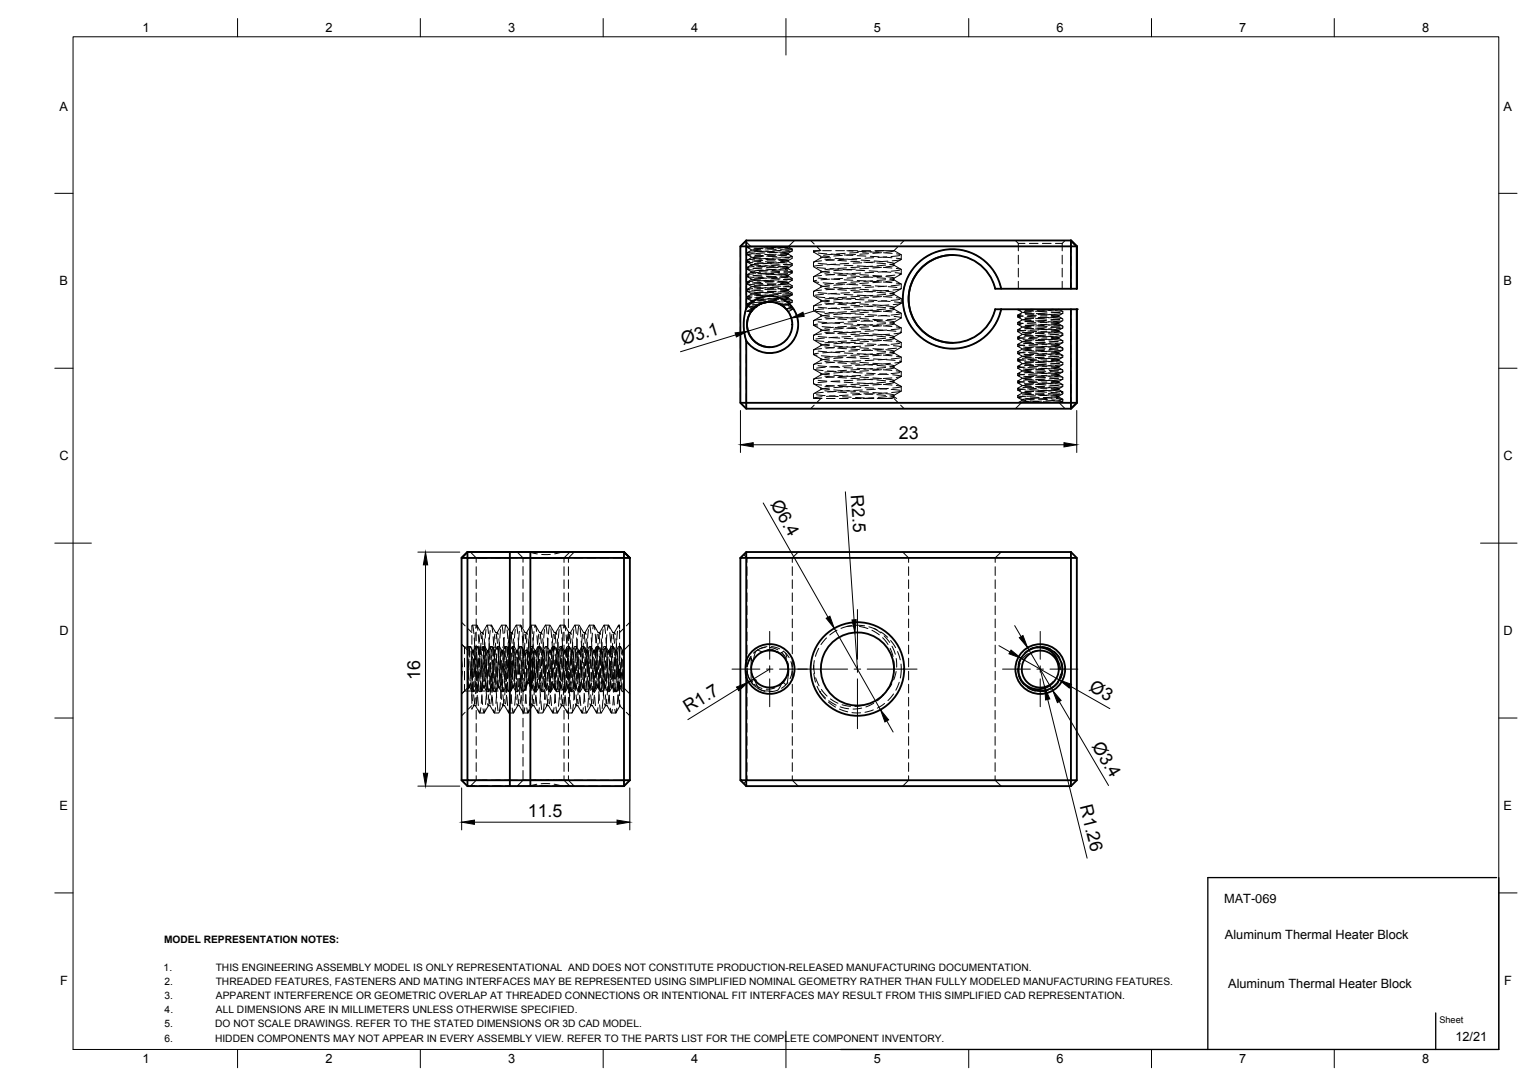
ISO-10303-21;
HEADER;
/* Generated by software containing ST-Developer
 * from STEP Tools, Inc. (www.steptools.com) 
 */

FILE_DESCRIPTION(
/* description */ ('CAx-IF Rec.Pracs.---Representation and Presentation of Product Manufa
cturing Information (PMI)---4.0---2014-10-13'),
/* implementation_level */ '2;1');

FILE_NAME(
/* name */ 'Aluminum Thermal Heater Block.step',
/* time_stamp */ '2026-10-24T15:08:39-07:00',
/* author */ (''),
/* organization */ (''),
/* preprocessor_version */ 'ST-DEVELOPER v20.2',
/* originating_system */ 'Autodesk Translation Framework v15.17.0.0',
/* authorisation */ '');

FILE_SCHEMA (('AP242_MANAGED_MODEL_BASED_3D_ENGINEERING_MIM_LF { 1 0 10303 442 2 1 4 }'));
ENDSEC;

DATA;
#10=MECHANICAL_DESIGN_GEOMETRIC_PRESENTATION_REPRESENTATION('',(#829),#50081);
#96=B_SPLINE_SURFACE_WITH_KNOTS('',3,3,((#29778,#29779,#29780,#29781,#29782,
#29783,#29784,#29785,#29786,#29787,#29788,#29789,#29790,#29791,#29792,#29793,
#29794,#29795,#29796,#29797,#29798,#29799,#29800,#29801,#29802,#29803,#29804,
#29805,#29806,#29807,#29808,#29809,#29810,#29811,#29812,#29813,#29814,#29815,
#29816,#29817,#29818,#29819,#29820,#29821,#29822,#29823,#29824,#29825,#29826,
#29827,#29828,#29829,#29830,#29831,#29832,#29833,#29834,#29835,#29836,#29837,
#29838,#29839,#29840,#29841,#29842,#29843,#29844,#29845,#29846,#29847,#29848,
#29849,#29850,#29851,#29852,#29853,#29854,#29855,#29856,#29857,#29858,#29859,
#29860,#29861,#29862),(#29863,#29864,#29865,#29866,#29867,#29868,#29869,
#29870,#29871,#29872,#29873,#29874,#29875,#29876,#29877,#29878,#29879,#29880,
#29881,#29882,#29883,#29884,#29885,#29886,#29887,#29888,#29889,#29890,#29891,
#29892,#29893,#29894,#29895,#29896,#29897,#29898,#29899,#29900,#29901,#29902,
#29903,#29904,#29905,#29906,#29907,#29908,#29909,#29910,#29911,#29912,#29913,
#29914,#29915,#29916,#29917,#29918,#29919,#29920,#29921,#29922,#29923,#29924,
#29925,#29926,#29927,#29928,#29929,#29930,#29931,#29932,#29933,#29934,#29935,
#29936,#29937,#29938,#29939,#29940,#29941,#29942,#29943,#29944,#29945,#29946,
#29947),(#29948,#29949,#29950,#29951,#29952,#29953,#29954,#29955,#29956,
#29957,#29958,#29959,#29960,#29961,#29962,#29963,#29964,#29965,#29966,#29967,
#29968,#29969,#29970,#29971,#29972,#29973,#29974,#29975,#29976,#29977,#29978,
#29979,#29980,#29981,#29982,#29983,#29984,#29985,#29986,#29987,#29988,#29989,
#29990,#29991,#29992,#29993,#29994,#29995,#29996,#29997,#29998,#29999,#30000,
#30001,#30002,#30003,#30004,#30005,#30006,#30007,#30008,#30009,#30010,#30011,
#30012,#30013,#30014,#30015,#30016,#30017,#30018,#30019,#30020,#30021,#30022,
#30023,#30024,#30025,#30026,#30027,#30028,#30029,#30030,#30031,#30032),
(#30033,#30034,#30035,#30036,#30037,#30038,#30039,#30040,#30041,#30042,
#30043,#30044,#30045,#30046,#30047,#30048,#30049,#30050,#30051,#30052,#30053,
#30054,#30055,#30056,#30057,#30058,#30059,#30060,#30061,#30062,#30063,#30064,
#30065,#30066,#30067,#30068,#30069,#30070,#30071,#30072,#30073,#30074,#30075,
#30076,#30077,#30078,#30079,#30080,#30081,#30082,#30083,#30084,#30085,#30086,
#30087,#30088,#30089,#30090,#30091,#30092,#30093,#30094,#30095,#30096,#30097,
#30098,#30099,#30100,#30101,#30102,#30103,#30104,#30105,#30106,#30107,#30108,
#30109,#30110,#30111,#30112,#30113,#30114,#30115,#30116,#30117)),
 .UNSPECIFIED.,.F.,.F.,.F.,(4,4),(4,1,1,1,1,1,1,1,1,1,1,1,1,1,1,1,1,1,1,
1,1,1,1,1,1,1,1,1,1,1,1,1,1,1,1,1,1,1,1,1,1,1,1,1,1,1,1,1,1,1,1,1,1,1,1,
1,1,1,1,1,1,1,1,1,1,1,1,1,1,1,1,1,1,1,1,1,1,1,1,1,1,1,4),(-0.000229032876373949,
0.0325052131810458),(10.2100639933856,11.2101668347381,12.2101575453093,
13.2101482558806,14.2101389664519,15.2101296770232,16.2101203875945,17.2101110981658,
18.2101018087371,19.2100925193084,20.2100832298797,21.210073940451,22.2100646510223,
23.2100553615935,24.2100460721648,25.2100367827361,26.2100274933074,27.2100182038787,
28.21000891445,29.2099996250213,30.2099903355926,31.2099810461639,32.2099717567352,
33.2099624673065,34.2099531778778,35.209943888449,36.2099345990203,37.2099253095916,
38.2099160201629,39.2099067307342,40.2098974413055,41.2098881518768,42.2098788624481,
43.2098695730194,44.2098602835907,45.209850994162,46.2098417047333,47.2098324153045,
48.2098231258758,49.2098138364471,50.2098045470184,51.2097952575897,52.209785968161,
53.2097766787323,54.2097673893036,55.2097580998749,56.2097488104462,57.2097395210175,
58.2097302315887,59.20972094216,60.2097116527313,61.2097023633026,62.2096930738739,
63.2096837844452,64.2096744950165,65.2096652055878,66.2096559161591,67.2096466267304,
68.2096373373017,69.209628047873,70.2096187584443,71.2096094690155,72.2096001795868,
73.2095908901581,74.2095816007294,75.2095723113007,76.209563021872,77.2095537324433,
78.2095444430146,79.2095351535859,80.2095258641572,81.2095165747285,82.2095072852998,
83.209497995871,84.2094887064423,85.2094794170136,86.2094701275849,87.2094608381562,
88.2094515487275,89.2094422592988,90.2094329698701,91.2094236804414,92.2094929101791),
 .UNSPECIFIED.);
#97=B_SPLINE_SURFACE_WITH_KNOTS('',3,3,((#30146,#30147,#30148,#30149,#30150,
#30151,#30152,#30153,#30154,#30155,#30156,#30157,#30158,#30159,#30160,#30161,
#30162,#30163,#30164,#30165,#30166,#30167,#30168,#30169,#30170,#30171,#30172,
#30173,#30174,#30175,#30176,#30177,#30178,#30179,#30180,#30181,#30182,#30183,
#30184,#30185,#30186,#30187,#30188,#30189,#30190,#30191,#30192,#30193,#30194,
#30195,#30196,#30197,#30198,#30199,#30200,#30201,#30202,#30203,#30204,#30205,
#30206,#30207,#30208,#30209,#30210,#30211,#30212,#30213,#30214,#30215,#30216,
#30217,#30218,#30219,#30220,#30221,#30222,#30223,#30224,#30225,#30226,#30227,
#30228,#30229,#30230),(#30231,#30232,#30233,#30234,#30235,#30236,#30237,
#30238,#30239,#30240,#30241,#30242,#30243,#30244,#30245,#30246,#30247,#30248,
#30249,#30250,#30251,#30252,#30253,#30254,#30255,#30256,#30257,#30258,#30259,
#30260,#30261,#30262,#30263,#30264,#30265,#30266,#30267,#30268,#30269,#30270,
#30271,#30272,#30273,#30274,#30275,#30276,#30277,#30278,#30279,#30280,#30281,
#30282,#30283,#30284,#30285,#30286,#30287,#30288,#30289,#30290,#30291,#30292,
#30293,#30294,#30295,#30296,#30297,#30298,#30299,#30300,#30301,#30302,#30303,
#30304,#30305,#30306,#30307,#30308,#30309,#30310,#30311,#30312,#30313,#30314,
#30315),(#30316,#30317,#30318,#30319,#30320,#30321,#30322,#30323,#30324,
#30325,#30326,#30327,#30328,#30329,#30330,#30331,#30332,#30333,#30334,#30335,
#30336,#30337,#30338,#30339,#30340,#30341,#30342,#30343,#30344,#30345,#30346,
#30347,#30348,#30349,#30350,#30351,#30352,#30353,#30354,#30355,#30356,#30357,
#30358,#30359,#30360,#30361,#30362,#30363,#30364,#30365,#30366,#30367,#30368,
#30369,#30370,#30371,#30372,#30373,#30374,#30375,#30376,#30377,#30378,#30379,
#30380,#30381,#30382,#30383,#30384,#30385,#30386,#30387,#30388,#30389,#30390,
#30391,#30392,#30393,#30394,#30395,#30396,#30397,#30398,#30399,#30400),
(#30401,#30402,#30403,#30404,#30405,#30406,#30407,#30408,#30409,#30410,
#30411,#30412,#30413,#30414,#30415,#30416,#30417,#30418,#30419,#30420,#30421,
#30422,#30423,#30424,#30425,#30426,#30427,#30428,#30429,#30430,#30431,#30432,
#30433,#30434,#30435,#30436,#30437,#30438,#30439,#30440,#30441,#30442,#30443,
#30444,#30445,#30446,#30447,#30448,#30449,#30450,#30451,#30452,#30453,#30454,
#30455,#30456,#30457,#30458,#30459,#30460,#30461,#30462,#30463,#30464,#30465,
#30466,#30467,#30468,#30469,#30470,#30471,#30472,#30473,#30474,#30475,#30476,
#30477,#30478,#30479,#30480,#30481,#30482,#30483,#30484,#30485)),
 .UNSPECIFIED.,.F.,.F.,.F.,(4,4),(4,1,1,1,1,1,1,1,1,1,1,1,1,1,1,1,1,1,1,
1,1,1,1,1,1,1,1,1,1,1,1,1,1,1,1,1,1,1,1,1,1,1,1,1,1,1,1,1,1,1,1,1,1,1,1,
1,1,1,1,1,1,1,1,1,1,1,1,1,1,1,1,1,1,1,1,1,1,1,1,1,1,1,4),(-0.000337093536336005,
0.0325391625776436),(13.6871942222869,14.6873814867633,15.6873721973346,
16.6873629079059,17.6873536184772,18.6873443290484,19.6873350396197,20.687325750191,
21.6873164607623,22.6873071713336,23.6872978819049,24.6872885924762,25.6872793030475,
26.6872700136188,27.6872607241901,28.6872514347614,29.6872421453326,30.6872328559039,
31.6872235664752,32.6872142770465,33.6872049876178,34.6871956981891,35.6871864087604,
36.6871771193317,37.687167829903,38.6871585404743,39.6871492510456,40.6871399616169,
41.6871306721881,42.6871213827594,43.6871120933307,44.687102803902,45.6870935144733,
46.6870842250446,47.6870749356159,48.6870656461872,49.6870563567585,50.6870470673298,
51.6870377779011,52.6870284884724,53.6870191990436,54.6870099096149,55.6870006201862,
56.6869913307575,57.6869820413288,58.6869727519001,59.6869634624714,60.6869541730427,
61.686944883614,62.6869355941853,63.6869263047566,64.6869170153279,65.6869077258991,
66.6868984364704,67.6868891470417,68.686879857613,69.6868705681843,70.6868612787556,
71.6868519893269,72.6868426998982,73.6868334104695,74.6868241210408,75.6868148316121,
76.6868055421834,77.6867962527546,78.6867869633259,79.6867776738972,80.6867683844685,
81.6867590950398,82.6867498056111,83.6867405161824,84.6867312267537,85.686721937325,
86.6867126478963,87.6867033584676,88.6866940690389,89.6866847796101,90.6866754901814,
91.6866662007527,92.686656911324,93.6866476218953,94.6866383324666,95.6868551020536),
 .UNSPECIFIED.);
#98=B_SPLINE_SURFACE_WITH_KNOTS('',3,3,((#30688,#30689,#30690,#30691,#30692,
#30693,#30694,#30695,#30696,#30697,#30698,#30699,#30700,#30701,#30702,#30703,
#30704,#30705,#30706,#30707,#30708,#30709,#30710,#30711,#30712,#30713,#30714,
#30715,#30716,#30717,#30718,#30719,#30720,#30721,#30722,#30723,#30724,#30725,
#30726,#30727,#30728,#30729,#30730,#30731,#30732,#30733,#30734,#30735,#30736,
#30737,#30738,#30739,#30740,#30741,#30742,#30743,#30744,#30745,#30746,#30747,
#30748,#30749,#30750,#30751,#30752,#30753,#30754,#30755,#30756),(#30757,
#30758,#30759,#30760,#30761,#30762,#30763,#30764,#30765,#30766,#30767,#30768,
#30769,#30770,#30771,#30772,#30773,#30774,#30775,#30776,#30777,#30778,#30779,
#30780,#30781,#30782,#30783,#30784,#30785,#30786,#30787,#30788,#30789,#30790,
#30791,#30792,#30793,#30794,#30795,#30796,#30797,#30798,#30799,#30800,#30801,
#30802,#30803,#30804,#30805,#30806,#30807,#30808,#30809,#30810,#30811,#30812,
#30813,#30814,#30815,#30816,#30817,#30818,#30819,#30820,#30821,#30822,#30823,
#30824,#30825),(#30826,#30827,#30828,#30829,#30830,#30831,#30832,#30833,
#30834,#30835,#30836,#30837,#30838,#30839,#30840,#30841,#30842,#30843,#30844,
#30845,#30846,#30847,#30848,#30849,#30850,#30851,#30852,#30853,#30854,#30855,
#30856,#30857,#30858,#30859,#30860,#30861,#30862,#30863,#30864,#30865,#30866,
#30867,#30868,#30869,#30870,#30871,#30872,#30873,#30874,#30875,#30876,#30877,
#30878,#30879,#30880,#30881,#30882,#30883,#30884,#30885,#30886,#30887,#30888,
#30889,#30890,#30891,#30892,#30893,#30894),(#30895,#30896,#30897,#30898,
#30899,#30900,#30901,#30902,#30903,#30904,#30905,#30906,#30907,#30908,#30909,
#30910,#30911,#30912,#30913,#30914,#30915,#30916,#30917,#30918,#30919,#30920,
#30921,#30922,#30923,#30924,#30925,#30926,#30927,#30928,#30929,#30930,#30931,
#30932,#30933,#30934,#30935,#30936,#30937,#30938,#30939,#30940,#30941,#30942,
#30943,#30944,#30945,#30946,#30947,#30948,#30949,#30950,#30951,#30952,#30953,
#30954,#30955,#30956,#30957,#30958,#30959,#30960,#30961,#30962,#30963)),
 .UNSPECIFIED.,.F.,.F.,.F.,(4,4),(4,1,1,1,1,1,1,1,1,1,1,1,1,1,1,1,1,1,1,
1,1,1,1,1,1,1,1,1,1,1,1,1,1,1,1,1,1,1,1,1,1,1,1,1,1,1,1,1,1,1,1,1,1,1,1,
1,1,1,1,1,1,1,1,1,1,1,4),(-0.000882682909917588,0.0581163152088491),(13.8937860366664,
14.8831634638169,15.8721630239192,16.8611625840214,17.8501621441237,18.8391617042259,
19.8281612643282,20.8171608244304,21.8061603845326,22.7951599446349,23.7841595047371,
24.7731590648394,25.7621586249416,26.7511581850439,27.7401577451461,28.7291573052483,
29.7181568653506,30.7071564254528,31.6961559855551,32.6851555456573,33.6741551057596,
34.6631546658618,35.652154225964,36.6411537860663,37.6301533461685,38.6191529062708,
39.608152466373,40.5971520264753,41.5861515865775,42.5751511466798,43.564150706782,
44.5531502668842,45.5421498269865,46.5311493870887,47.520148947191,48.5091485072932,
49.4981480673955,50.4871476274977,51.4761471875999,52.4651467477022,53.4541463078044,
54.4431458679067,55.4321454280089,56.4211449881112,57.4101445482134,58.3991441083156,
59.3881436684179,60.3771432285201,61.3661427886224,62.3551423487246,63.3441419088269,
64.3331414689291,65.3221410290313,66.3111405891336,67.3001401492358,68.2891397093381,
69.2781392694403,70.2671388295426,71.2561383896448,72.245137949747,73.2341375098493,
74.2231370699515,75.2121366300538,76.201136190156,77.1901357502583,78.1791353103605,
79.1681348704628),.UNSPECIFIED.);
#99=B_SPLINE_SURFACE_WITH_KNOTS('',3,3,((#31557,#31558,#31559,#31560,#31561,
#31562,#31563,#31564,#31565,#31566,#31567,#31568,#31569,#31570,#31571,#31572,
#31573,#31574,#31575,#31576,#31577,#31578,#31579,#31580,#31581,#31582,#31583,
#31584,#31585,#31586,#31587,#31588,#31589,#31590,#31591,#31592,#31593,#31594,
#31595,#31596,#31597,#31598,#31599,#31600,#31601,#31602,#31603,#31604,#31605,
#31606,#31607,#31608,#31609,#31610,#31611,#31612,#31613,#31614,#31615,#31616,
#31617,#31618,#31619,#31620,#31621,#31622,#31623,#31624,#31625),(#31626,
#31627,#31628,#31629,#31630,#31631,#31632,#31633,#31634,#31635,#31636,#31637,
#31638,#31639,#31640,#31641,#31642,#31643,#31644,#31645,#31646,#31647,#31648,
#31649,#31650,#31651,#31652,#31653,#31654,#31655,#31656,#31657,#31658,#31659,
#31660,#31661,#31662,#31663,#31664,#31665,#31666,#31667,#31668,#31669,#31670,
#31671,#31672,#31673,#31674,#31675,#31676,#31677,#31678,#31679,#31680,#31681,
#31682,#31683,#31684,#31685,#31686,#31687,#31688,#31689,#31690,#31691,#31692,
#31693,#31694),(#31695,#31696,#31697,#31698,#31699,#31700,#31701,#31702,
#31703,#31704,#31705,#31706,#31707,#31708,#31709,#31710,#31711,#31712,#31713,
#31714,#31715,#31716,#31717,#31718,#31719,#31720,#31721,#31722,#31723,#31724,
#31725,#31726,#31727,#31728,#31729,#31730,#31731,#31732,#31733,#31734,#31735,
#31736,#31737,#31738,#31739,#31740,#31741,#31742,#31743,#31744,#31745,#31746,
#31747,#31748,#31749,#31750,#31751,#31752,#31753,#31754,#31755,#31756,#31757,
#31758,#31759,#31760,#31761,#31762,#31763),(#31764,#31765,#31766,#31767,
#31768,#31769,#31770,#31771,#31772,#31773,#31774,#31775,#31776,#31777,#31778,
#31779,#31780,#31781,#31782,#31783,#31784,#31785,#31786,#31787,#31788,#31789,
#31790,#31791,#31792,#31793,#31794,#31795,#31796,#31797,#31798,#31799,#31800,
#31801,#31802,#31803,#31804,#31805,#31806,#31807,#31808,#31809,#31810,#31811,
#31812,#31813,#31814,#31815,#31816,#31817,#31818,#31819,#31820,#31821,#31822,
#31823,#31824,#31825,#31826,#31827,#31828,#31829,#31830,#31831,#31832)),
 .UNSPECIFIED.,.F.,.F.,.F.,(4,4),(4,1,1,1,1,1,1,1,1,1,1,1,1,1,1,1,1,1,1,
1,1,1,1,1,1,1,1,1,1,1,1,1,1,1,1,1,1,1,1,1,1,1,1,1,1,1,1,1,1,1,1,1,1,1,1,
1,1,1,1,1,1,1,1,1,1,1,4),(-0.000390001319482014,0.0587333122782212),(10.2099729995397,
11.199175684269,12.1881752443713,13.1771748044735,14.1661743645758,15.155173924678,
16.1441734847802,17.1331730448825,18.1221726049847,19.111172165087,20.1001717251892,
21.0891712852915,22.0781708453937,23.0671704054959,24.0561699655982,25.0451695257004,
26.0341690858027,27.0231686459049,28.0121682060072,29.0011677661094,29.9901673262116,
30.9791668863139,31.9681664464161,32.9571660065184,33.9461655666206,34.9351651267229,
35.9241646868251,36.9131642469273,37.9021638070296,38.8911633671318,39.8801629272341,
40.8691624873363,41.8581620474386,42.8471616075408,43.836161167643,44.8251607277453,
45.8141602878475,46.8031598479498,47.792159408052,48.7811589681543,49.7701585282565,
50.7591580883588,51.748157648461,52.7371572085632,53.7261567686655,54.7151563287677,
55.70415588887,56.6931554489722,57.6821550090744,58.6711545691767,59.6601541292789,
60.6491536893812,61.6381532494834,62.6271528095857,63.6161523696879,64.6051519297902,
65.5941514898924,66.5831510499946,67.5721506100969,68.5611501701991,69.5501497303014,
70.5391492904036,71.5281488505059,72.5171484106081,73.5061479707103,74.4951475308126,
75.484582158383),.UNSPECIFIED.);
#100=B_SPLINE_SURFACE_WITH_KNOTS('',3,3,((#33783,#33784,#33785,#33786,#33787,
#33788,#33789,#33790,#33791,#33792,#33793,#33794,#33795,#33796,#33797,#33798,
#33799,#33800,#33801,#33802,#33803,#33804,#33805,#33806,#33807,#33808,#33809,
#33810,#33811,#33812,#33813,#33814,#33815,#33816,#33817,#33818,#33819,#33820,
#33821,#33822,#33823,#33824,#33825,#33826,#33827,#33828,#33829,#33830,#33831,
#33832,#33833,#33834,#33835,#33836),(#33837,#33838,#33839,#33840,#33841,
#33842,#33843,#33844,#33845,#33846,#33847,#33848,#33849,#33850,#33851,#33852,
#33853,#33854,#33855,#33856,#33857,#33858,#33859,#33860,#33861,#33862,#33863,
#33864,#33865,#33866,#33867,#33868,#33869,#33870,#33871,#33872,#33873,#33874,
#33875,#33876,#33877,#33878,#33879,#33880,#33881,#33882,#33883,#33884,#33885,
#33886,#33887,#33888,#33889,#33890),(#33891,#33892,#33893,#33894,#33895,
#33896,#33897,#33898,#33899,#33900,#33901,#33902,#33903,#33904,#33905,#33906,
#33907,#33908,#33909,#33910,#33911,#33912,#33913,#33914,#33915,#33916,#33917,
#33918,#33919,#33920,#33921,#33922,#33923,#33924,#33925,#33926,#33927,#33928,
#33929,#33930,#33931,#33932,#33933,#33934,#33935,#33936,#33937,#33938,#33939,
#33940,#33941,#33942,#33943,#33944),(#33945,#33946,#33947,#33948,#33949,
#33950,#33951,#33952,#33953,#33954,#33955,#33956,#33957,#33958,#33959,#33960,
#33961,#33962,#33963,#33964,#33965,#33966,#33967,#33968,#33969,#33970,#33971,
#33972,#33973,#33974,#33975,#33976,#33977,#33978,#33979,#33980,#33981,#33982,
#33983,#33984,#33985,#33986,#33987,#33988,#33989,#33990,#33991,#33992,#33993,
#33994,#33995,#33996,#33997,#33998)),.UNSPECIFIED.,.F.,.F.,.F.,(4,4),(4,
1,1,1,1,1,1,1,1,1,1,1,1,1,1,1,1,1,1,1,1,1,1,1,1,1,1,1,1,1,1,1,1,1,1,1,1,
1,1,1,1,1,1,1,1,1,1,1,1,1,1,4),(-0.000427176962040987,0.0325519917386635),
(13.6872368315967,14.6740326940116,15.6606746118312,16.6473165296507,17.6339584474703,
18.6206003652899,19.6072422831094,20.593884200929,21.5805261187486,22.5671680365682,
23.5538099543877,24.5404518722073,25.5270937900269,26.5137357078464,27.500377625666,
28.4870195434856,29.4736614613051,30.4603033791247,31.4469452969443,32.4335872147639,
33.4202291325834,34.406871050403,35.3935129682226,36.3801548860421,37.3667968038617,
38.3534387216813,39.3400806395008,40.3267225573204,41.31336447514,42.3000063929596,
43.2866483107791,44.2732902285987,45.2599321464183,46.2465740642378,47.2332159820574,
48.219857899877,49.2064998176965,50.1931417355161,51.1797836533357,52.1664255711553,
53.1530674889748,54.1397094067944,55.126351324614,56.1129932424335,57.0996351602531,
58.0862770780727,59.0729189958922,60.0595609137118,61.0462028315314,62.032844749351,
63.0194866671705,64.0063577917107),.UNSPECIFIED.);
#101=B_SPLINE_SURFACE_WITH_KNOTS('',3,3,((#34172,#34173,#34174,#34175,#34176,
#34177,#34178,#34179,#34180,#34181,#34182,#34183,#34184,#34185,#34186,#34187,
#34188,#34189,#34190,#34191,#34192,#34193,#34194,#34195,#34196,#34197,#34198,
#34199,#34200,#34201,#34202,#34203,#34204,#34205,#34206,#34207,#34208,#34209,
#34210,#34211,#34212,#34213,#34214,#34215,#34216,#34217,#34218,#34219,#34220,
#34221,#34222,#34223,#34224,#34225),(#34226,#34227,#34228,#34229,#34230,
#34231,#34232,#34233,#34234,#34235,#34236,#34237,#34238,#34239,#34240,#34241,
#34242,#34243,#34244,#34245,#34246,#34247,#34248,#34249,#34250,#34251,#34252,
#34253,#34254,#34255,#34256,#34257,#34258,#34259,#34260,#34261,#34262,#34263,
#34264,#34265,#34266,#34267,#34268,#34269,#34270,#34271,#34272,#34273,#34274,
#34275,#34276,#34277,#34278,#34279),(#34280,#34281,#34282,#34283,#34284,
#34285,#34286,#34287,#34288,#34289,#34290,#34291,#34292,#34293,#34294,#34295,
#34296,#34297,#34298,#34299,#34300,#34301,#34302,#34303,#34304,#34305,#34306,
#34307,#34308,#34309,#34310,#34311,#34312,#34313,#34314,#34315,#34316,#34317,
#34318,#34319,#34320,#34321,#34322,#34323,#34324,#34325,#34326,#34327,#34328,
#34329,#34330,#34331,#34332,#34333),(#34334,#34335,#34336,#34337,#34338,
#34339,#34340,#34341,#34342,#34343,#34344,#34345,#34346,#34347,#34348,#34349,
#34350,#34351,#34352,#34353,#34354,#34355,#34356,#34357,#34358,#34359,#34360,
#34361,#34362,#34363,#34364,#34365,#34366,#34367,#34368,#34369,#34370,#34371,
#34372,#34373,#34374,#34375,#34376,#34377,#34378,#34379,#34380,#34381,#34382,
#34383,#34384,#34385,#34386,#34387)),.UNSPECIFIED.,.F.,.F.,.F.,(4,4),(4,
1,1,1,1,1,1,1,1,1,1,1,1,1,1,1,1,1,1,1,1,1,1,1,1,1,1,1,1,1,1,1,1,1,1,1,1,
1,1,1,1,1,1,1,1,1,1,1,1,1,1,4),(-0.000290371553175226,0.0325162600682668),
(10.2100759344954,11.2038007070197,12.1974252898726,13.1910498727256,14.1846744555785,
15.1782990384314,16.1719236212843,17.1655482041372,18.1591727869901,19.152797369843,
20.146421952696,21.1400465355489,22.1336711184018,23.1272957012547,24.1209202841076,
25.1145448669605,26.1081694498134,27.1017940326664,28.0954186155193,29.0890431983722,
30.0826677812251,31.076292364078,32.0699169469309,33.0635415297839,34.0571661126368,
35.0507906954897,36.0444152783426,37.0380398611955,38.0316644440484,39.0252890269013,
40.0189136097543,41.0125381926072,42.0061627754601,42.999787358313,43.9934119411659,
44.9870365240188,45.9806611068718,46.9742856897247,47.9679102725776,48.9615348554305,
49.9551594382834,50.9487840211363,51.9424086039892,52.9360331868422,53.9296577696951,
54.923282352548,55.9169069354009,56.9105315182538,57.9041561011067,58.8977806839596,
59.8914052668126,60.8850348774998),.UNSPECIFIED.);
#102=B_SPLINE_SURFACE_WITH_KNOTS('',3,3,((#34609,#34610,#34611,#34612,#34613),
(#34614,#34615,#34616,#34617,#34618),(#34619,#34620,#34621,#34622,#34623),
(#34624,#34625,#34626,#34627,#34628)),.UNSPECIFIED.,.F.,.F.,.F.,(4,4),(4,
1,4),(0.,0.032160890827504),(68.4560911973857,69.0589356637105,69.6617801300352),
 .UNSPECIFIED.);
#103=B_SPLINE_SURFACE_WITH_KNOTS('',3,3,((#34647,#34648,#34649,#34650,#34651),
(#34652,#34653,#34654,#34655,#34656),(#34657,#34658,#34659,#34660,#34661),
(#34662,#34663,#34664,#34665,#34666)),.UNSPECIFIED.,.F.,.F.,.F.,(4,4),(4,
1,4),(-9.07170059861442E-6,0.0322908342399317),(61.7440410216514,62.7372907531955,
63.7305404920565),.UNSPECIFIED.);
#104=B_SPLINE_SURFACE_WITH_KNOTS('',3,3,((#34693,#34694,#34695,#34696,#34697),
(#34698,#34699,#34700,#34701,#34702),(#34703,#34704,#34705,#34706,#34707),
(#34708,#34709,#34710,#34711,#34712)),.UNSPECIFIED.,.F.,.F.,.F.,(4,4),(4,
1,4),(-0.000103109978180118,0.0323481470425964),(64.9669593015238,65.8588193203942,
66.7505475116691),.UNSPECIFIED.);
#105=B_SPLINE_SURFACE_WITH_KNOTS('',3,3,((#34737,#34738,#34739,#34740,#34741),
(#34742,#34743,#34744,#34745,#34746),(#34747,#34748,#34749,#34750,#34751),
(#34752,#34753,#34754,#34755,#34756)),.UNSPECIFIED.,.F.,.F.,.F.,(4,4),(4,
1,4),(0.00156261713707751,0.032191282069214),(65.1886793093356,65.9220033054732,
66.6553273016042),.UNSPECIFIED.);
#204=B_SPLINE_CURVE_WITH_KNOTS('',3,(#18145,#18146,#18147,#18148),
 .UNSPECIFIED.,.F.,.F.,(4,4),(0.971412745929808,0.971526261856752),
 .UNSPECIFIED.);
#205=B_SPLINE_CURVE_WITH_KNOTS('',3,(#18150,#18151,#18152,#18153,#18154,
#18155,#18156,#18157,#18158,#18159),.UNSPECIFIED.,.F.,.F.,(4,3,3,4),(0.,
0.167901694834844,0.56724113492481,0.999999992512719),.UNSPECIFIED.);
#206=B_SPLINE_CURVE_WITH_KNOTS('',3,(#18161,#18162,#18163,#18164,#18165,
#18166),.UNSPECIFIED.,.F.,.F.,(4,2,4),(0.315127929368065,0.328175365228812,
0.354466558811423),.UNSPECIFIED.);
#207=B_SPLINE_CURVE_WITH_KNOTS('',3,(#18168,#18169,#18170,#18171,#18172,
#18173,#18174,#18175,#18176,#18177,#18178,#18179,#18180,#18181,#18182,#18183,
#18184,#18185,#18186,#18187,#18188,#18189,#18190,#18191,#18192,#18193,#18194,
#18195,#18196,#18197,#18198,#18199,#18200,#18201,#18202,#18203,#18204,#18205,
#18206,#18207,#18208,#18209,#18210,#18211,#18212,#18213,#18214,#18215),
 .UNSPECIFIED.,.F.,.F.,(4,2,2,2,2,2,2,2,2,2,2,2,2,2,2,2,2,2,2,2,2,2,2,4),
(0.000119713185355978,0.00575344874658494,0.00971112169393152,0.0122781598323848,
0.0146592854190729,0.0174902469786257,0.0227397139191457,0.0430245441916241,
0.0660773827934058,0.0761631161494674,0.0842516350753493,0.0890477968215787,
0.0934275126674497,0.0991547350761513,0.111968591580187,0.132666811210395,
0.158224662764418,0.163318033350428,0.166132967630979,0.16860703948596,
0.172184160315179,0.182361036453311,0.201361583255606,0.223791868919182),
 .UNSPECIFIED.);
#208=B_SPLINE_CURVE_WITH_KNOTS('',3,(#18216,#18217,#18218,#18219),
 .UNSPECIFIED.,.F.,.F.,(4,4),(-9.40886979550022E-5,-9.99998847734106E-7),
 .UNSPECIFIED.);
#209=B_SPLINE_CURVE_WITH_KNOTS('',3,(#18225,#18226,#18227,#18228),
 .UNSPECIFIED.,.F.,.F.,(4,4),(-4.85633810213992,-4.85633121754184),
 .UNSPECIFIED.);
#210=B_SPLINE_CURVE_WITH_KNOTS('',3,(#18229,#18230,#18231,#18232,#18233,
#18234,#18235,#18236,#18237,#18238,#18239,#18240,#18241,#18242,#18243,#18244,
#18245,#18246,#18247,#18248,#18249,#18250,#18251,#18252,#18253,#18254,#18255,
#18256,#18257,#18258,#18259,#18260,#18261,#18262,#18263,#18264,#18265,#18266,
#18267,#18268,#18269,#18270,#18271,#18272,#18273,#18274,#18275,#18276,#18277,
#18278,#18279,#18280,#18281,#18282,#18283,#18284,#18285,#18286,#18287,#18288,
#18289,#18290,#18291,#18292,#18293,#18294,#18295,#18296,#18297,#18298,#18299,
#18300,#18301,#18302,#18303,#18304,#18305,#18306,#18307,#18308,#18309,#18310,
#18311,#18312,#18313,#18314,#18315,#18316,#18317,#18318,#18319,#18320,#18321,
#18322,#18323,#18324,#18325,#18326,#18327,#18328,#18329,#18330,#18331,#18332,
#18333,#18334,#18335,#18336,#18337,#18338,#18339,#18340,#18341,#18342,#18343,
#18344,#18345,#18346,#18347,#18348,#18349,#18350,#18351,#18352,#18353,#18354,
#18355,#18356,#18357,#18358,#18359,#18360,#18361,#18362,#18363,#18364,#18365,
#18366,#18367,#18368,#18369,#18370,#18371,#18372,#18373,#18374,#18375,#18376,
#18377,#18378,#18379,#18380,#18381,#18382,#18383,#18384,#18385,#18386,#18387,
#18388,#18389,#18390,#18391,#18392,#18393,#18394,#18395,#18396,#18397,#18398,
#18399,#18400,#18401,#18402,#18403,#18404,#18405,#18406),.UNSPECIFIED.,
 .F.,.F.,(4,2,2,2,2,2,2,2,2,2,2,2,2,2,2,2,2,2,2,2,2,2,2,2,2,2,2,2,2,2,2,
2,2,2,2,2,2,2,2,2,2,2,2,2,2,2,2,2,2,2,2,2,2,2,2,2,2,2,2,2,2,2,2,2,2,2,2,
2,2,2,2,2,2,2,2,2,2,2,2,2,2,2,2,2,2,2,2,2,4),(0.000141208970641106,0.00260421869732101,
0.0052276655840623,0.0097768460544778,0.0172305119182923,0.0501220173560818,
0.0664236905796941,0.0757300526936879,0.0791631109294421,0.0815747821003626,
0.0843414713693197,0.0894007964463044,0.122158036354821,0.138557390784882,
0.149876449259462,0.155175782700374,0.159350568636847,0.164184987943546,
0.172678480141147,0.210890365945431,0.227969106547551,0.232065738371256,
0.234603525100323,0.23716172683167,0.241335891636054,0.25882343157927,0.286510199887536,
0.301740206595418,0.307600734640189,0.311888589272734,0.316468780859696,
0.323892113808258,0.358076836795881,0.373771160545672,0.382869904577255,
0.386278215195521,0.388683195388731,0.391441676684064,0.396518214189327,
0.426670009264769,0.451576415664413,0.459372629966599,0.464001457786102,
0.468219921708977,0.473710730334942,0.485788376105022,0.504690750023019,
0.533932313828317,0.53873116378046,0.541406392559831,0.543848174084512,
0.547461433203641,0.558234193736316,0.579315768765851,0.605461131396945,
0.613275807184344,0.617943501828802,0.622217509627598,0.627912405532227,
0.641771644016302,0.664748194881735,0.686924115465114,0.692149336246089,
0.694936696052987,0.697413109346304,0.700989607490205,0.711057887758149,
0.72977222339771,0.757407061188366,0.76510902159049,0.769781938977176,0.77411278768263,
0.779969035677471,0.794784284402865,0.820580861292412,0.8410739972508,0.845308006048228,
0.847872631386642,0.850264924059376,0.853976226329157,0.867138706639604,
0.899855434061717,0.916853095757379,0.922877344557088,0.926610466523709,
0.930734370267285,0.936631753567681,0.953829720348217,0.971412745929808),
 .UNSPECIFIED.);
#211=B_SPLINE_CURVE_WITH_KNOTS('',3,(#18407,#18408,#18409,#18410,#18411,
#18412,#18413,#18414,#18415,#18416,#18417,#18418,#18419,#18420,#18421,#18422,
#18423,#18424,#18425,#18426,#18427,#18428,#18429,#18430,#18431,#18432,#18433,
#18434,#18435,#18436,#18437,#18438,#18439,#18440,#18441,#18442,#18443,#18444,
#18445,#18446,#18447,#18448,#18449,#18450,#18451,#18452,#18453,#18454,#18455,
#18456,#18457,#18458,#18459,#18460,#18461,#18462,#18463,#18464,#18465,#18466,
#18467,#18468,#18469,#18470,#18471,#18472,#18473,#18474,#18475,#18476,#18477,
#18478,#18479,#18480,#18481,#18482,#18483,#18484,#18485,#18486,#18487,#18488,
#18489,#18490,#18491,#18492,#18493,#18494,#18495,#18496,#18497,#18498,#18499,
#18500,#18501,#18502,#18503,#18504,#18505,#18506,#18507,#18508,#18509,#18510,
#18511,#18512,#18513,#18514,#18515,#18516,#18517,#18518,#18519,#18520,#18521,
#18522,#18523,#18524,#18525,#18526,#18527,#18528,#18529,#18530,#18531,#18532,
#18533,#18534,#18535,#18536,#18537,#18538,#18539,#18540,#18541,#18542,#18543,
#18544,#18545,#18546,#18547,#18548,#18549,#18550,#18551,#18552,#18553,#18554,
#18555,#18556,#18557,#18558,#18559,#18560,#18561,#18562,#18563,#18564,#18565,
#18566,#18567,#18568,#18569,#18570,#18571,#18572,#18573,#18574,#18575,#18576,
#18577,#18578,#18579,#18580,#18581,#18582,#18583,#18584,#18585,#18586,#18587,
#18588),.UNSPECIFIED.,.F.,.F.,(4,2,2,2,2,2,2,2,2,2,2,2,2,2,2,2,2,2,2,2,
2,2,2,2,2,2,2,2,2,2,2,2,2,2,2,2,2,2,2,2,2,2,2,2,2,2,2,2,2,2,2,2,2,2,2,2,
2,2,2,2,2,2,2,2,2,2,2,2,2,2,2,2,2,2,2,2,2,2,2,2,2,2,2,2,2,2,2,2,2,2,4),
(-0.971391456537255,-0.971350475017715,-0.94591226166657,-0.939055866602481,
-0.934491943525297,-0.929966522537624,-0.923315457172628,-0.900084828443717,
-0.866675788733297,-0.861483715642629,-0.858667284068134,-0.856156444610882,
-0.852480155304097,-0.841678563536531,-0.82054319420312,-0.79533261802684,
-0.787491045820371,-0.782733466408728,-0.77832103124467,-0.772342363335511,
-0.75698856882546,-0.728964770759938,-0.712339354105396,-0.708142242501503,
-0.705532704686271,-0.702880771961631,-0.698485355783003,-0.674022702995305,
-0.642599533278312,-0.634880128685733,-0.630145861839832,-0.625722256150309,
-0.619676109637291,-0.603761730423759,-0.5733448179666,-0.564910522641159,
-0.557601689880697,-0.55443107439597,-0.551970146896551,-0.548875717294742,
-0.542206024288379,-0.532494999382091,-0.489582880438121,-0.482087767216936,
-0.477401905795565,-0.472964832662002,-0.466804632427164,-0.449814264601177,
-0.413424403576693,-0.405535496779586,-0.402459473341899,-0.399951900345286,
-0.397132042878921,-0.391921343895885,-0.372654164363047,-0.336263006736024,
-0.329122575864086,-0.324502881571398,-0.320018727171346,-0.313602331443732,
-0.29388634728559,-0.276304617435784,-0.256570434034097,-0.251340125257597,
-0.24851417463144,-0.245996946416581,-0.242316540835892,-0.231540604020166,
-0.210486510775074,-0.185387242102097,-0.177555587523125,-0.172793530995205,
-0.16836913555747,-0.162360818143053,-0.146824797563933,-0.118104728439308,
-0.102309888146275,-0.098139487777396,-0.0955356246830923,-0.0929006792526596,
-0.088522539861798,-0.0830553365089054,-0.070707876555459,-0.0556129729315022,
-0.0325113603607354,-0.0247369510017717,-0.0200127871468392,-0.0158546275414271,
-0.0115824295604963,-0.00654733946174566,-9.40886979550022E-5),
 .UNSPECIFIED.);
#212=B_SPLINE_CURVE_WITH_KNOTS('',3,(#18593,#18594,#18595,#18596,#18597,
#18598,#18599,#18600,#18601,#18602,#18603,#18604,#18605,#18606,#18607,#18608,
#18609,#18610,#18611,#18612,#18613,#18614,#18615,#18616,#18617,#18618,#18619,
#18620,#18621,#18622,#18623,#18624,#18625,#18626,#18627,#18628,#18629,#18630,
#18631,#18632,#18633,#18634,#18635,#18636,#18637,#18638,#18639,#18640,#18641,
#18642,#18643,#18644,#18645,#18646,#18647,#18648,#18649,#18650,#18651,#18652,
#18653,#18654,#18655,#18656,#18657,#18658,#18659,#18660,#18661,#18662,#18663,
#18664,#18665,#18666,#18667,#18668,#18669,#18670,#18671,#18672,#18673,#18674,
#18675,#18676,#18677,#18678,#18679,#18680,#18681,#18682,#18683,#18684,#18685,
#18686,#18687,#18688,#18689,#18690,#18691,#18692,#18693,#18694,#18695,#18696,
#18697,#18698,#18699,#18700,#18701,#18702,#18703,#18704,#18705,#18706,#18707,
#18708,#18709,#18710,#18711,#18712,#18713,#18714,#18715,#18716,#18717,#18718,
#18719,#18720,#18721,#18722,#18723,#18724,#18725,#18726,#18727,#18728,#18729,
#18730,#18731,#18732,#18733,#18734,#18735,#18736,#18737,#18738,#18739,#18740,
#18741,#18742,#18743,#18744,#18745,#18746,#18747,#18748,#18749,#18750,#18751,
#18752,#18753,#18754,#18755,#18756,#18757,#18758,#18759,#18760,#18761,#18762,
#18763,#18764,#18765,#18766,#18767,#18768),.UNSPECIFIED.,.F.,.F.,(4,2,2,
2,2,2,2,2,2,2,2,2,2,2,2,2,2,2,2,2,2,2,2,2,2,2,2,2,2,2,2,2,2,2,2,2,2,2,2,
2,2,2,2,2,2,2,2,2,2,2,2,2,2,2,2,2,2,2,2,2,2,2,2,2,2,2,2,2,2,2,2,2,2,2,2,
2,2,2,2,2,2,2,2,2,2,2,2,4),(-4.85633121754184,-4.85213065139609,-4.84647712007667,
-4.81509163858284,-4.79825979897682,-4.78876865709538,-4.78530539628214,
-4.78288273583215,-4.78011349846824,-4.7750701610028,-4.74952354545192,
-4.72855908723541,-4.71538188389384,-4.70978571060111,-4.70552965445536,
-4.70082677238956,-4.69281250170212,-4.65374878230526,-4.63651598370295,
-4.63240505707741,-4.62985974897014,-4.62730253249263,-4.62313232718254,
-4.60581215907345,-4.57782671807124,-4.56249583090281,-4.55661704711339,
-4.55232213524437,-4.54774021309657,-4.54032700092237,-4.50611548905706,
-4.4904787062145,-4.48139560604128,-4.47798324594874,-4.47556663890993,
-4.47276988568106,-4.46759538793662,-4.4469975552687,-4.42839427299879,
-4.41579147273591,-4.40632672287472,-4.40134419610195,-4.39712653939579,
-4.39196322116091,-4.38149899293316,-4.34576805751086,-4.3291871500724,
-4.32511116833149,-4.32257420413104,-4.32001020944753,-4.3158074141098,
-4.29765351873152,-4.27033522323949,-4.2551758391028,-4.24931760071498,
-4.24502565608104,-4.24043587806352,-4.23298424974857,-4.1991058388011,
-4.18330012692505,-4.17699819205573,-4.17214266234621,-4.16944123140104,
-4.1670201152808,-4.1640022471072,-4.15612700531233,-4.11979209381665,-4.10217771943166,
-4.0960492225731,-4.09171332297588,-4.08774491599307,-4.08121543145688,
-4.06038638190995,-4.03660661272028,-4.0217184107034,-4.01774498588615,
-4.01522918083307,-4.01264060239549,-4.00832142166615,-3.98491873872065,
-3.96283719571124,-3.94786173772201,-3.94202651256228,-3.93773842295176,
-3.93314082421309,-3.92564856185857,-3.89212701756681,-3.88485527042599),
 .UNSPECIFIED.);
#213=B_SPLINE_CURVE_WITH_KNOTS('',3,(#18770,#18771,#18772,#18773,#18774,
#18775,#18776,#18777,#18778,#18779,#18780,#18781,#18782,#18783,#18784,#18785,
#18786,#18787,#18788,#18789,#18790,#18791,#18792,#18793,#18794,#18795,#18796,
#18797,#18798,#18799,#18800,#18801,#18802,#18803,#18804,#18805,#18806,#18807,
#18808,#18809,#18810,#18811,#18812,#18813,#18814,#18815,#18816,#18817,#18818,
#18819,#18820,#18821,#18822,#18823,#18824,#18825,#18826,#18827,#18828,#18829,
#18830,#18831,#18832,#18833,#18834,#18835,#18836,#18837,#18838,#18839,#18840,
#18841,#18842,#18843,#18844,#18845,#18846,#18847,#18848,#18849,#18850,#18851,
#18852,#18853,#18854,#18855,#18856,#18857,#18858,#18859,#18860,#18861,#18862,
#18863,#18864,#18865,#18866,#18867,#18868,#18869,#18870,#18871,#18872,#18873,
#18874,#18875,#18876,#18877,#18878,#18879,#18880,#18881,#18882,#18883,#18884,
#18885,#18886,#18887,#18888,#18889,#18890,#18891,#18892,#18893,#18894,#18895,
#18896,#18897,#18898,#18899,#18900,#18901,#18902,#18903,#18904,#18905,#18906,
#18907,#18908,#18909,#18910,#18911,#18912,#18913,#18914,#18915,#18916,#18917,
#18918,#18919,#18920,#18921,#18922,#18923,#18924,#18925,#18926,#18927,#18928,
#18929,#18930,#18931,#18932,#18933,#18934,#18935,#18936,#18937,#18938,#18939,
#18940,#18941,#18942,#18943,#18944,#18945,#18946,#18947,#18948,#18949),
 .UNSPECIFIED.,.F.,.F.,(4,2,2,2,2,2,2,2,2,2,2,2,2,2,2,2,2,2,2,2,2,2,2,2,
2,2,2,2,2,2,2,2,2,2,2,2,2,2,2,2,2,2,2,2,2,2,2,2,2,2,2,2,2,2,2,2,2,2,2,2,
2,2,2,2,2,2,2,2,2,2,2,2,2,2,2,2,2,2,2,2,2,2,2,2,2,2,2,2,2,4),(-1.94269089166418,
-1.93517126631823,-1.93043333031223,-1.92786163297422,-1.92553536015628,
-1.92280532619892,-1.91803394431714,-1.89257796006248,-1.87521637487989,
-1.85925975941574,-1.85320984431279,-1.84878693253339,-1.84405669275704,
-1.83635192095474,-1.80474817087353,-1.78807814579666,-1.77861330164555,
-1.77509630832447,-1.77260867024126,-1.76971426813013,-1.76413130798493,
-1.72451055249351,-1.70709282269508,-1.70088554182812,-1.69643807008872,
-1.69176164519176,-1.6843267070496,-1.65018390868158,-1.6349011240992,-1.62868924094152,
-1.62386396573735,-1.62112286042163,-1.61860796391698,-1.61476212732756,
-1.60325377303154,-1.57221947927429,-1.55461691378427,-1.54839093462721,
-1.54394024355143,-1.5392693116814,-1.53186285436495,-1.4974924177766,-1.47704377309018,
-1.47170592584779,-1.46886008183724,-1.46635918549734,-1.46332036842669,
-1.45569326796168,-1.41897825334754,-1.40193593124306,-1.39576718039066,
-1.39132592330984,-1.38663716530924,-1.3791401304918,-1.34060260362163,
-1.32827031598642,-1.32279955547753,-1.31841370662874,-1.31576482604718,
-1.31315484570357,-1.30895356582117,-1.29223604561974,-1.26426876913352,
-1.24892766355139,-1.24295068925588,-1.23853883800795,-1.2337812834758,
-1.22593814368876,-1.20005736734272,-1.17945799774462,-1.16880260208862,
-1.16514274803746,-1.1626344563469,-1.15981042358652,-1.15458141811861,
-1.13486316357308,-1.11599121466708,-1.09728664369118,-1.09095635205127,
-1.08648786296795,-1.08184677873542,-1.07459311863954,-1.03907910966406,
-1.01933714810872,-1.01407451481946,-1.0112436859667,-1.00873791278509,
-1.00567541865444,-0.999413749447903,-0.971391456537255),.UNSPECIFIED.);
#214=B_SPLINE_CURVE_WITH_KNOTS('',3,(#18950,#18951,#18952,#18953),
 .UNSPECIFIED.,.F.,.F.,(4,4),(-5.03931041703063E-5,-9.99999999955958E-7),
 .UNSPECIFIED.);
#215=B_SPLINE_CURVE_WITH_KNOTS('',3,(#18958,#18959,#18960,#18961,#18962,
#18963,#18964,#18965,#18966,#18967,#18968,#18969,#18970,#18971,#18972,#18973,
#18974,#18975,#18976,#18977,#18978,#18979,#18980,#18981,#18982,#18983,#18984,
#18985,#18986,#18987,#18988,#18989,#18990,#18991,#18992,#18993,#18994,#18995,
#18996,#18997,#18998,#18999,#19000,#19001,#19002,#19003,#19004,#19005,#19006,
#19007,#19008,#19009,#19010,#19011,#19012,#19013,#19014,#19015,#19016,#19017,
#19018,#19019,#19020,#19021,#19022,#19023,#19024,#19025,#19026,#19027,#19028,
#19029,#19030,#19031,#19032,#19033,#19034,#19035,#19036,#19037,#19038,#19039,
#19040,#19041,#19042,#19043,#19044,#19045,#19046,#19047,#19048,#19049,#19050,
#19051,#19052,#19053,#19054,#19055,#19056,#19057,#19058,#19059,#19060,#19061,
#19062,#19063,#19064,#19065,#19066,#19067,#19068,#19069,#19070,#19071,#19072,
#19073,#19074,#19075,#19076,#19077,#19078,#19079,#19080,#19081,#19082,#19083,
#19084,#19085,#19086,#19087,#19088,#19089,#19090,#19091,#19092,#19093,#19094,
#19095,#19096,#19097,#19098,#19099,#19100,#19101,#19102,#19103,#19104,#19105,
#19106,#19107,#19108,#19109,#19110,#19111,#19112,#19113,#19114,#19115,#19116,
#19117,#19118,#19119,#19120,#19121,#19122,#19123,#19124,#19125,#19126,#19127,
#19128,#19129,#19130,#19131,#19132,#19133,#19134,#19135,#19136,#19137,#19138,
#19139,#19140,#19141),.UNSPECIFIED.,.F.,.F.,(4,2,2,2,2,2,2,2,2,2,2,2,2,
2,2,2,2,2,2,2,2,2,2,2,2,2,2,2,2,2,2,2,2,2,2,2,2,2,2,2,2,2,2,2,2,2,2,2,2,
2,2,2,2,2,2,2,2,2,2,2,2,2,2,2,2,2,2,2,2,2,2,2,2,2,2,2,2,2,2,2,2,2,2,2,2,
2,2,2,2,2,2,4),(-3.88485527042599,-3.87612942688473,-3.86692044470073,-3.86349153731901,
-3.86107257062718,-3.85828415396544,-3.85314986936548,-3.83333871713199,
-3.81620582124791,-3.79554569255171,-3.78915634087622,-3.78477394437684,
-3.78033504307713,-3.77364604115463,-3.74852033650871,-3.72943267851357,
-3.71450137835232,-3.71052510579754,-3.70800873290492,-3.70542091489492,
-3.70110519033777,-3.67776277543455,-3.65576783747023,-3.64067702214714,
-3.63482764500726,-3.6305374713829,-3.62594527333001,-3.61847969068087,
-3.58472537830717,-3.56885372918825,-3.55968859064669,-3.55626545207974,
-3.55384732491795,-3.55105601839559,-3.54590777953046,-3.52577729066484,
-3.50121160951107,-3.4868336778872,-3.48107453324816,-3.4767977861641,-3.47217062463026,
-3.464530214041,-3.4265206417358,-3.41369232636088,-3.40567341917178,-3.40241026570776,
-3.40001061219079,-3.39712333543128,-3.39133091879335,-3.35149730986139,
-3.3340332722328,-3.3279203483318,-3.32358760248186,-3.31961685512853,-3.31307117766192,
-3.29189576157376,-3.26853402696514,-3.25362519952796,-3.24965080394012,
-3.24713502918839,-3.2445471729515,-3.24023032986175,-3.216862172777,-3.19482835978413,
-3.17979514314729,-3.17395332523438,-3.16966470088453,-3.16507048997968,
-3.15759303466847,-3.12395452658673,-3.10802504654718,-3.09884021816107,
-3.09541476698086,-3.09299655139007,-3.09020699420807,-3.0850660896511,
-3.06508406113471,-3.04741826210348,-3.03394630531244,-3.0240292898885,
-3.01896370630131,-3.01474788399437,-3.00967462757103,-3.00003076781016,
-2.96340500896624,-2.94664413792194,-2.94255877751648,-2.94001993078873,
-2.93745851883094,-2.93326652107717,-2.91540016853139,-2.91349531428362),
 .UNSPECIFIED.);
#216=B_SPLINE_CURVE_WITH_KNOTS('',3,(#19142,#19143,#19144,#19145,#19146,
#19147,#19148,#19149,#19150,#19151,#19152,#19153,#19154,#19155,#19156,#19157,
#19158,#19159,#19160,#19161,#19162,#19163,#19164,#19165,#19166,#19167,#19168,
#19169,#19170,#19171,#19172,#19173,#19174,#19175,#19176,#19177,#19178,#19179,
#19180,#19181,#19182,#19183,#19184,#19185,#19186,#19187,#19188,#19189,#19190,
#19191,#19192,#19193,#19194,#19195,#19196,#19197,#19198,#19199,#19200,#19201,
#19202,#19203,#19204,#19205,#19206,#19207,#19208,#19209,#19210,#19211,#19212,
#19213,#19214,#19215,#19216,#19217,#19218,#19219,#19220,#19221,#19222,#19223,
#19224,#19225,#19226,#19227,#19228,#19229,#19230,#19231,#19232,#19233,#19234,
#19235,#19236,#19237,#19238,#19239,#19240,#19241,#19242,#19243,#19244,#19245,
#19246,#19247,#19248,#19249,#19250,#19251,#19252,#19253,#19254,#19255,#19256,
#19257,#19258,#19259,#19260,#19261,#19262,#19263,#19264,#19265,#19266,#19267,
#19268,#19269,#19270,#19271,#19272,#19273,#19274,#19275,#19276,#19277,#19278,
#19279,#19280,#19281,#19282,#19283,#19284,#19285,#19286,#19287,#19288,#19289,
#19290,#19291,#19292,#19293,#19294,#19295,#19296,#19297,#19298,#19299,#19300,
#19301,#19302,#19303,#19304,#19305,#19306,#19307,#19308,#19309,#19310,#19311,
#19312,#19313),.UNSPECIFIED.,.F.,.F.,(4,2,2,2,2,2,2,2,2,2,2,2,2,2,2,2,2,
2,2,2,2,2,2,2,2,2,2,2,2,2,2,2,2,2,2,2,2,2,2,2,2,2,2,2,2,2,2,2,2,2,2,2,2,
2,2,2,2,2,2,2,2,2,2,2,2,2,2,2,2,2,2,2,2,2,2,2,2,2,2,2,2,2,2,2,2,4),(-0.971153636545791,
-0.971008594948987,-0.965153140353171,-0.95076796891759,-0.926253312146383,
-0.90671530802577,-0.901494145309361,-0.89867202134374,-0.896163631368954,
-0.892501243608833,-0.881821284397918,-0.861131733116912,-0.835352323870838,
-0.827509082887044,-0.822751871248581,-0.818340630311989,-0.812364916031061,
-0.797028470229962,-0.769069200644485,-0.752372464055914,-0.748172865866162,
-0.745563418770317,-0.742914593343789,-0.738527914593733,-0.713956050207449,
-0.682628402926648,-0.674902030268896,-0.670168151700236,-0.665748074128256,
-0.659711984422174,-0.643865552001454,-0.613741869417596,-0.599615662445248,
-0.595543574305058,-0.593215185351513,-0.590611055995399,-0.586436796558227,
-0.569165018086564,-0.529000858285284,-0.52183672145698,-0.517213947677662,
-0.512735529760769,-0.506342893017696,-0.486899844471605,-0.462578022509873,
-0.447258910048538,-0.443111883548401,-0.440769822998353,-0.438181882272539,
-0.434086121713075,-0.418245765591886,-0.394401111842103,-0.375077375664371,
-0.368594007728611,-0.364144264275441,-0.359553818730779,-0.352556450278034,
-0.323932613112025,-0.296283664564022,-0.291322307551835,-0.288553280531884,
-0.286023139790771,-0.282230708438604,-0.27030305615395,-0.244409759413656,
-0.222958751252185,-0.216306730914958,-0.212233208575315,-0.207751323681161,
-0.201340042475556,-0.181673786527202,-0.164031378728836,-0.144274319040584,
-0.139042083772736,-0.136217773264899,-0.133710255969495,-0.130053059538382,
-0.119418783112649,-0.0988954692710536,-0.0728956763044899,-0.0650518898003542,
-0.0602946576044903,-0.0558835931377834,-0.0499084241794123,-0.0345755390114698,
-5.03931041703063E-5),.UNSPECIFIED.);
#217=B_SPLINE_CURVE_WITH_KNOTS('',3,(#19318,#19319,#19320,#19321,#19322,
#19323,#19324,#19325,#19326,#19327,#19328,#19329,#19330,#19331,#19332,#19333,
#19334,#19335,#19336,#19337,#19338,#19339,#19340,#19341,#19342,#19343,#19344,
#19345,#19346,#19347,#19348,#19349,#19350,#19351,#19352,#19353,#19354,#19355,
#19356,#19357,#19358,#19359,#19360,#19361,#19362,#19363,#19364,#19365,#19366,
#19367,#19368,#19369,#19370,#19371,#19372,#19373,#19374,#19375,#19376,#19377,
#19378,#19379,#19380,#19381,#19382,#19383,#19384,#19385,#19386,#19387,#19388,
#19389,#19390,#19391,#19392,#19393,#19394,#19395,#19396,#19397,#19398,#19399,
#19400,#19401,#19402,#19403,#19404,#19405,#19406,#19407,#19408,#19409,#19410,
#19411,#19412,#19413,#19414,#19415,#19416,#19417,#19418,#19419,#19420,#19421,
#19422,#19423,#19424,#19425,#19426,#19427,#19428,#19429,#19430,#19431,#19432,
#19433,#19434,#19435,#19436,#19437,#19438,#19439,#19440,#19441,#19442,#19443,
#19444,#19445,#19446,#19447,#19448,#19449,#19450,#19451,#19452,#19453,#19454,
#19455,#19456,#19457,#19458,#19459,#19460,#19461,#19462,#19463,#19464,#19465,
#19466,#19467,#19468,#19469,#19470,#19471,#19472,#19473,#19474,#19475,#19476,
#19477,#19478,#19479,#19480,#19481,#19482,#19483,#19484,#19485,#19486,#19487,
#19488,#19489,#19490,#19491,#19492,#19493,#19494,#19495,#19496,#19497,#19498,
#19499),.UNSPECIFIED.,.F.,.F.,(4,2,2,2,2,2,2,2,2,2,2,2,2,2,2,2,2,2,2,2,
2,2,2,2,2,2,2,2,2,2,2,2,2,2,2,2,2,2,2,2,2,2,2,2,2,2,2,2,2,2,2,2,2,2,2,2,
2,2,2,2,2,2,2,2,2,2,2,2,2,2,2,2,2,2,2,2,2,2,2,2,2,2,2,2,2,2,2,2,2,2,4),
(-2.91349531428362,-2.88785921300174,-2.8726430027449,-2.86677863205918,
-2.86248643922693,-2.85790029096159,-2.85046367156569,-2.81646981931229,
-2.8007280660255,-2.79160863757645,-2.78819166947628,-2.78577453314058,
-2.78298032492328,-2.7778177001423,-2.75740712949668,-2.73825152738121,
-2.72583812859598,-2.71647441260755,-2.71151088112635,-2.70729248773251,
-2.70210703845323,-2.69390586646746,-2.6591339369195,-2.64588606824007,
-2.63769869396671,-2.63441089253566,-2.63200904157476,-2.62913865956645,
-2.6234339484568,-2.58348277115152,-2.56600629696093,-2.55989253487532,
-2.55555995071342,-2.55158985421312,-2.54504643819555,-2.52390841910659,
-2.50029087033371,-2.49029362580967,-2.48351409579007,-2.480449193245,-2.4780605078139,
-2.47501214793163,-2.46832900078042,-2.45915292464736,-2.42810789893616,
-2.41232853260371,-2.40625822001906,-2.40197600471217,-2.39746852318833,
-2.39042469203808,-2.38200394689515,-2.36369363346378,-2.33336593040561,
-2.32867955052637,-2.32601391858675,-2.3235491164382,-2.31983572683312,
-2.30811366746104,-2.28309948628011,-2.2599663128295,-2.25335383883438,
-2.24893029326256,-2.24453614668166,-2.23807947644657,-2.21642727345666,
-2.19829989391596,-2.17894872278306,-2.17472001156547,-2.1721509942611,
-2.16961971164294,-2.16556936904969,-2.14944123261186,-2.12563610681186,
-2.10603499553312,-2.09958972783228,-2.09563623816902,-2.09128861274927,
-2.08508808823211,-2.06670303492164,-2.04752070148475,-2.027147259442,-2.02198742240317,
-2.01919398856709,-2.01677702398121,-2.01335958053459,-2.00423504373367,
-1.98847734663213,-1.95449285532475,-1.94705346079759,-1.94246711155014,
-1.94225105833858),.UNSPECIFIED.);
#218=B_SPLINE_CURVE_WITH_KNOTS('',3,(#19500,#19501,#19502,#19503,#19504,
#19505,#19506,#19507,#19508,#19509,#19510,#19511,#19512,#19513,#19514,#19515,
#19516,#19517,#19518,#19519,#19520,#19521,#19522,#19523,#19524,#19525,#19526,
#19527,#19528,#19529,#19530,#19531,#19532,#19533,#19534,#19535,#19536,#19537,
#19538,#19539,#19540,#19541,#19542,#19543,#19544,#19545,#19546,#19547,#19548,
#19549,#19550,#19551,#19552,#19553,#19554,#19555,#19556,#19557,#19558,#19559,
#19560,#19561,#19562,#19563,#19564,#19565,#19566,#19567,#19568,#19569,#19570,
#19571,#19572,#19573,#19574,#19575,#19576,#19577,#19578,#19579,#19580,#19581,
#19582,#19583,#19584,#19585,#19586,#19587,#19588,#19589,#19590,#19591,#19592,
#19593,#19594,#19595,#19596,#19597,#19598,#19599,#19600,#19601,#19602,#19603,
#19604,#19605,#19606,#19607,#19608,#19609,#19610,#19611,#19612,#19613,#19614,
#19615,#19616,#19617,#19618,#19619,#19620,#19621,#19622,#19623,#19624,#19625,
#19626,#19627,#19628,#19629,#19630,#19631,#19632,#19633,#19634,#19635,#19636,
#19637,#19638,#19639,#19640,#19641,#19642,#19643,#19644,#19645,#19646,#19647,
#19648,#19649,#19650,#19651,#19652,#19653,#19654,#19655,#19656,#19657,#19658,
#19659,#19660,#19661,#19662,#19663,#19664,#19665,#19666,#19667,#19668,#19669,
#19670,#19671,#19672,#19673),.UNSPECIFIED.,.F.,.F.,(4,2,2,2,2,2,2,2,2,2,
2,2,2,2,2,2,2,2,2,2,2,2,2,2,2,2,2,2,2,2,2,2,2,2,2,2,2,2,2,2,2,2,2,2,2,2,
2,2,2,2,2,2,2,2,2,2,2,2,2,2,2,2,2,2,2,2,2,2,2,2,2,2,2,2,2,2,2,2,2,2,2,2,
2,2,2,2,4),(-1.94245618738083,-1.93666604794167,-1.90204794308009,-1.89466971332662,
-1.89000414570624,-1.88555010505709,-1.87930511456366,-1.86150959565628,
-1.84248742044491,-1.82190397686627,-1.81663235642541,-1.81379978161942,
-1.8112944826846,-1.80765376515567,-1.79716872592755,-1.77718374838492,
-1.75044607779919,-1.74260114083196,-1.73784309629813,-1.73343120666949,
-1.72745480759043,-1.71211797648903,-1.68416231528133,-1.66745337302565,
-1.6632526590439,-1.6606427107058,-1.65799358232213,-1.65360673403587,-1.64813392266078,
-1.63579470820685,-1.59724524016339,-1.58974619776021,-1.58505694537765,
-1.58061575981501,-1.57444797141161,-1.55741343123057,-1.52073045017774,
-1.51309191974478,-1.51005139105216,-1.50755014135901,-1.50470548247491,
-1.49937336423293,-1.4789803418051,-1.44449618557995,-1.43710156101452,
-1.43243304053073,-1.42798123994456,-1.42174793734908,-1.40406750826335,
-1.38483827982886,-1.36431858492595,-1.35905146718736,-1.35621995243168,
-1.35371459476435,-1.35007240956499,-1.33957267411533,-1.31953415473493,
-1.29287412174753,-1.28502968466071,-1.28027201711475,-1.2758605236468,
-1.26988473431397,-1.25454998511729,-1.22659974312072,-1.20988862582101,
-1.20568810136917,-1.20307834315922,-1.20042948546114,-1.19604321065498,
-1.17138803697016,-1.14015161558894,-1.13241791790184,-1.12768236692295,
-1.12326253877635,-1.11722967994469,-1.10141348586324,-1.07142877420758,
-1.05714431415319,-1.05306015150634,-1.05072945077579,-1.048127766341,-1.04396593742351,
-1.02694592560699,-0.988307700660695,-0.980210340516297,-0.97540285891718,
-0.971153636545791),.UNSPECIFIED.);
#219=B_SPLINE_CURVE_WITH_KNOTS('',3,(#19678,#19679,#19680,#19681,#19682,
#19683,#19684,#19685,#19686,#19687,#19688,#19689,#19690,#19691,#19692,#19693,
#19694,#19695,#19696,#19697,#19698,#19699,#19700,#19701,#19702,#19703,#19704,
#19705,#19706,#19707,#19708,#19709,#19710,#19711,#19712,#19713,#19714,#19715,
#19716,#19717,#19718,#19719,#19720,#19721,#19722,#19723,#19724,#19725,#19726,
#19727,#19728,#19729,#19730,#19731,#19732,#19733,#19734,#19735,#19736,#19737,
#19738,#19739,#19740,#19741,#19742,#19743,#19744,#19745,#19746,#19747,#19748,
#19749,#19750,#19751,#19752,#19753,#19754,#19755,#19756,#19757,#19758,#19759,
#19760,#19761,#19762,#19763,#19764,#19765,#19766,#19767,#19768,#19769,#19770,
#19771,#19772,#19773,#19774,#19775,#19776,#19777,#19778,#19779,#19780,#19781,
#19782,#19783,#19784,#19785,#19786,#19787,#19788,#19789,#19790,#19791,#19792,
#19793,#19794,#19795,#19796,#19797,#19798,#19799,#19800,#19801,#19802,#19803,
#19804,#19805,#19806,#19807,#19808,#19809,#19810,#19811,#19812,#19813,#19814,
#19815,#19816,#19817,#19818,#19819,#19820,#19821,#19822,#19823,#19824,#19825,
#19826,#19827,#19828,#19829,#19830,#19831,#19832,#19833,#19834,#19835,#19836,
#19837,#19838,#19839,#19840,#19841,#19842,#19843,#19844,#19845,#19846,#19847,
#19848,#19849,#19850,#19851,#19852,#19853,#19854,#19855),.UNSPECIFIED.,
 .F.,.F.,(4,2,2,2,2,2,2,2,2,2,2,2,2,2,2,2,2,2,2,2,2,2,2,2,2,2,2,2,2,2,2,
2,2,2,2,2,2,2,2,2,2,2,2,2,2,2,2,2,2,2,2,2,2,2,2,2,2,2,2,2,2,2,2,2,2,2,2,
2,2,2,2,2,2,2,2,2,2,2,2,2,2,2,2,2,2,2,2,2,4),(-1.94225105833858,-1.93817574801027,
-1.93231411518889,-1.91711500751957,-1.88963102947338,-1.87172412036913,
-1.86753138927278,-1.8649700191301,-1.86243177847413,-1.8583481593741,-1.84161793735377,
-1.80515530132293,-1.795380257346,-1.79028208426469,-1.78606669827375,-1.78102681224781,
-1.77124795889596,-1.73973914369167,-1.719912592923,-1.71477931531364,-1.71199154432955,
-1.70957320869571,-1.70614527105133,-1.69693999447017,-1.68095029460128,
-1.64740248617903,-1.63991313286521,-1.6353168705613,-1.63102976626463,
-1.6251954438425,-1.61021784625178,-1.58816155316777,-1.56478150171211,
-1.56046398562556,-1.55787617832783,-1.55536095068415,-1.5513880750123,
-1.53649964166235,-1.51269756471832,-1.49188165487078,-1.48535372135347,
-1.48138635901469,-1.47705172621421,-1.47092519036825,-1.45331554879081,
-1.41749445323066,-1.40922488689507,-1.40584696409475,-1.40343514035856,
-1.400620134993,-1.39519912177293,-1.38788544959407,-1.3670881388276,-1.34080726817211,
-1.33301890460348,-1.32836274674951,-1.32409675309266,-1.31840930426554,
-1.30456333433945,-1.2816664608601,-1.25919555634037,-1.25404859301556,
-1.25125790778109,-1.24884029374826,-1.24541780555451,-1.23625448984316,
-1.22038566594815,-1.1866117703993,-1.17914796741874,-1.17455678542318,
-1.17026754163774,-1.1644193812063,-1.14932995360108,-1.12226165345558,
-1.10383073725108,-1.09962093371131,-1.09705596718609,-1.09452113217626,
-1.09045361213551,-1.07401965479348,-1.0457268751906,-1.0300686358062,-1.02400990891724,
-1.01972965461697,-1.01521888392003,-1.00815824775775,-0.98876999730182,
-0.971774429615847,-0.971085382281135),.UNSPECIFIED.);
#220=B_SPLINE_CURVE_WITH_KNOTS('',3,(#19856,#19857,#19858,#19859,#19860,
#19861,#19862,#19863,#19864,#19865,#19866,#19867,#19868,#19869,#19870,#19871,
#19872,#19873,#19874,#19875,#19876,#19877,#19878,#19879,#19880,#19881,#19882,
#19883,#19884,#19885,#19886,#19887,#19888,#19889,#19890,#19891,#19892,#19893,
#19894,#19895,#19896,#19897,#19898,#19899,#19900,#19901,#19902,#19903,#19904,
#19905,#19906,#19907,#19908,#19909,#19910,#19911,#19912,#19913,#19914,#19915,
#19916,#19917,#19918,#19919,#19920,#19921,#19922,#19923,#19924,#19925,#19926,
#19927,#19928,#19929,#19930,#19931,#19932,#19933,#19934,#19935,#19936,#19937,
#19938,#19939,#19940,#19941,#19942,#19943,#19944,#19945,#19946,#19947,#19948,
#19949,#19950,#19951,#19952,#19953,#19954,#19955,#19956,#19957,#19958,#19959,
#19960,#19961,#19962,#19963,#19964,#19965,#19966,#19967,#19968,#19969,#19970,
#19971,#19972,#19973,#19974,#19975,#19976,#19977,#19978,#19979,#19980,#19981,
#19982,#19983,#19984,#19985,#19986,#19987,#19988,#19989,#19990,#19991,#19992,
#19993,#19994,#19995,#19996,#19997,#19998,#19999,#20000,#20001,#20002,#20003,
#20004,#20005,#20006,#20007,#20008,#20009,#20010,#20011,#20012,#20013,#20014,
#20015,#20016,#20017,#20018,#20019,#20020,#20021,#20022,#20023,#20024,#20025,
#20026,#20027,#20028,#20029,#20030,#20031,#20032,#20033,#20034,#20035),
 .UNSPECIFIED.,.F.,.F.,(4,2,2,2,2,2,2,2,2,2,2,2,2,2,2,2,2,2,2,2,2,2,2,2,
2,2,2,2,2,2,2,2,2,2,2,2,2,2,2,2,2,2,2,2,2,2,2,2,2,2,2,2,2,2,2,2,2,2,2,2,
2,2,2,2,2,2,2,2,2,2,2,2,2,2,2,2,2,2,2,2,2,2,2,2,2,2,2,2,2,4),(-2.91390510725203,
-2.90506916989555,-2.88772673429663,-2.8835480860879,-2.8809423704627,-2.87861359182467,
-2.87454254971778,-2.86044734758774,-2.83026176834386,-2.81439641115966,
-2.80835642733313,-2.80393451095304,-2.79919960570182,-2.79147369713496,
-2.76012189440003,-2.73557156460837,-2.73118505816924,-2.72853566313497,
-2.7259250364792,-2.72172250438345,-2.70499398005282,-2.67702817031134,
-2.66168584902575,-2.65570787327748,-2.65129512960579,-2.64653646712782,
-2.63869114627471,-2.6126222420344,-2.59215471299504,-2.58153453166287,
-2.57787815246974,-2.5753700689154,-2.57254382937296,-2.56730509631592,
-2.54736467729883,-2.52861598188627,-2.50999173565466,-2.50366784824209,
-2.49919992865341,-2.49455609451121,-2.48729097506967,-2.45184326922799,
-2.4371964058279,-2.42844302550073,-2.42535639556814,-2.42284501514053,
-2.420028027468,-2.41483495373192,-2.3957295454715,-2.35910993658772,-2.35200981835196,
-2.34739843873784,-2.3429095787987,-2.33646386555045,-2.31638148401164,
-2.29909437824261,-2.27944481753455,-2.27421846504341,-2.27139486389236,
-2.26888614771493,-2.26522465745816,-2.25455806149966,-2.23392189313628,
-2.2080583944128,-2.20021292232938,-2.19545449055155,-2.19104220230369,
-2.18506520124496,-2.16972638699072,-2.14176573463677,-2.12505839436397,
-2.12085745960638,-2.11824731279366,-2.11559791678661,-2.11121051920109,
-2.10573695657757,-2.09339565663989,-2.05484541326446,-2.04734518869667,
-2.04265542025411,-2.03821389526489,-2.03204588294094,-2.01501288953075,
-1.97834784318526,-1.970691107395,-1.9676476134136,-1.96514559019334,-1.96230241920289,
-1.95697850885554,-1.94245618738083),.UNSPECIFIED.);
#221=B_SPLINE_CURVE_WITH_KNOTS('',3,(#20041,#20042,#20043,#20044),
 .UNSPECIFIED.,.F.,.F.,(4,4),(0.971411654023308,0.971463527532095),
 .UNSPECIFIED.);
#222=B_SPLINE_CURVE_WITH_KNOTS('',3,(#20045,#20046,#20047,#20048,#20049,
#20050,#20051,#20052,#20053,#20054,#20055,#20056,#20057,#20058,#20059,#20060,
#20061,#20062,#20063,#20064,#20065,#20066,#20067,#20068,#20069,#20070,#20071,
#20072,#20073,#20074,#20075,#20076,#20077,#20078,#20079,#20080,#20081,#20082,
#20083,#20084,#20085,#20086,#20087,#20088,#20089,#20090,#20091,#20092,#20093,
#20094,#20095,#20096,#20097,#20098,#20099,#20100,#20101,#20102,#20103,#20104,
#20105,#20106,#20107,#20108,#20109,#20110,#20111,#20112,#20113,#20114,#20115,
#20116,#20117,#20118,#20119,#20120,#20121,#20122,#20123,#20124,#20125,#20126,
#20127,#20128,#20129,#20130,#20131,#20132,#20133,#20134,#20135,#20136,#20137,
#20138,#20139,#20140,#20141,#20142,#20143,#20144,#20145,#20146,#20147,#20148,
#20149,#20150,#20151,#20152,#20153,#20154,#20155,#20156,#20157,#20158,#20159,
#20160,#20161,#20162,#20163,#20164,#20165,#20166,#20167,#20168,#20169,#20170,
#20171,#20172,#20173,#20174,#20175,#20176,#20177,#20178,#20179,#20180,#20181,
#20182,#20183,#20184,#20185,#20186,#20187,#20188,#20189,#20190,#20191,#20192,
#20193,#20194,#20195,#20196,#20197,#20198,#20199,#20200,#20201,#20202,#20203,
#20204,#20205,#20206,#20207,#20208,#20209,#20210,#20211,#20212,#20213,#20214,
#20215,#20216,#20217,#20218,#20219,#20220,#20221,#20222,#20223,#20224,#20225,
#20226,#20227,#20228),.UNSPECIFIED.,.F.,.F.,(4,2,2,2,2,2,2,2,2,2,2,2,2,
2,2,2,2,2,2,2,2,2,2,2,2,2,2,2,2,2,2,2,2,2,2,2,2,2,2,2,2,2,2,2,2,2,2,2,2,
2,2,2,2,2,2,2,2,2,2,2,2,2,2,2,2,2,2,2,2,2,2,2,2,2,2,2,2,2,2,2,2,2,2,2,2,
2,2,2,2,2,2,4),(-0.971085382281135,-0.952017792902401,-0.946887432167989,
-0.944100295124911,-0.941681821236157,-0.938252749983855,-0.929038611127879,
-0.913023210440452,-0.879523662738073,-0.872029045202164,-0.867431756175606,
-0.863145118166893,-0.857313684147572,-0.842359088763997,-0.820286139752394,
-0.796894438362392,-0.79257632409696,-0.789988405026593,-0.787473312643114,
-0.783501009954662,-0.768620603544608,-0.744673319203854,-0.723979872911306,
-0.717458520787705,-0.713492309834453,-0.709156757727181,-0.703024669862699,
-0.685358114282465,-0.65359169314679,-0.642232113050811,-0.638459384428977,
-0.636008118489447,-0.633371235784275,-0.628821535758767,-0.623041560473158,
-0.609403794671107,-0.573020454850763,-0.565176371485666,-0.560509312757121,
-0.556247032331601,-0.550585160075782,-0.536923941376815,-0.514576124664695,
-0.491216671566923,-0.486125177869648,-0.48334636199671,-0.48092577991027,
-0.477480959993249,-0.468144152881925,-0.451770477933558,-0.418925052205649,
-0.411361974473767,-0.406751108100979,-0.402470006324611,-0.396674683919592,
-0.382006200663234,-0.356452120365438,-0.336009594444376,-0.331774337944482,
-0.329204078843861,-0.326674365941362,-0.322630720333002,-0.306612701948914,
-0.280508397917966,-0.277886164043204,-0.262211200634713,-0.25615115654366,
-0.251870919348402,-0.247360986889347,-0.24030345927568,-0.209476177528243,
-0.183985304908225,-0.178943418322464,-0.176175112575443,-0.173751473514796,
-0.170285537214507,-0.160782937797474,-0.143915852684806,-0.111923197089701,
-0.104281902724935,-0.0996552709832551,-0.0953797221880297,-0.0896232712769271,
-0.0752578316239034,-0.0628013904956974,-0.0323914044481022,-0.0260414146726733,
-0.0230517243937155,-0.0206616239994298,-0.0183163031974911,-0.0151902078220476,
-1.00000003733225E-6),.UNSPECIFIED.);
#223=B_SPLINE_CURVE_WITH_KNOTS('',3,(#20229,#20230,#20231,#20232,#20233,
#20234,#20235,#20236,#20237,#20238,#20239,#20240,#20241,#20242,#20243,#20244,
#20245,#20246,#20247,#20248,#20249,#20250,#20251,#20252,#20253,#20254,#20255,
#20256,#20257,#20258,#20259,#20260,#20261,#20262,#20263,#20264,#20265,#20266,
#20267,#20268,#20269,#20270,#20271,#20272,#20273,#20274,#20275,#20276,#20277,
#20278,#20279,#20280,#20281,#20282,#20283,#20284,#20285,#20286,#20287,#20288,
#20289,#20290,#20291,#20292,#20293,#20294,#20295,#20296,#20297,#20298,#20299,
#20300,#20301,#20302,#20303,#20304,#20305,#20306,#20307,#20308,#20309,#20310,
#20311,#20312,#20313,#20314,#20315,#20316,#20317,#20318,#20319,#20320,#20321,
#20322,#20323,#20324,#20325,#20326,#20327,#20328,#20329,#20330,#20331,#20332,
#20333,#20334,#20335,#20336,#20337,#20338,#20339,#20340,#20341,#20342,#20343,
#20344,#20345,#20346,#20347,#20348,#20349,#20350,#20351,#20352,#20353,#20354,
#20355,#20356,#20357,#20358,#20359,#20360,#20361,#20362,#20363,#20364,#20365,
#20366,#20367,#20368,#20369,#20370,#20371,#20372,#20373,#20374,#20375,#20376,
#20377,#20378,#20379,#20380,#20381,#20382,#20383,#20384,#20385,#20386,#20387,
#20388,#20389,#20390,#20391,#20392,#20393,#20394,#20395,#20396,#20397,#20398,
#20399,#20400,#20401,#20402,#20403,#20404,#20405,#20406,#20407,#20408),
 .UNSPECIFIED.,.F.,.F.,(4,2,2,2,2,2,2,2,2,2,2,2,2,2,2,2,2,2,2,2,2,2,2,2,
2,2,2,2,2,2,2,2,2,2,2,2,2,2,2,2,2,2,2,2,2,2,2,2,2,2,2,2,2,2,2,2,2,2,2,2,
2,2,2,2,2,2,2,2,2,2,2,2,2,2,2,2,2,2,2,2,2,2,2,2,2,2,2,2,2,4),(-3.88535150283469,
-3.88206035453889,-3.87607707548919,-3.87166257690228,-3.86690391205419,
-3.85906272704095,-3.83357894725827,-3.8126953004503,-3.80533831202851,
-3.799868786755,-3.7969956088574,-3.79450114210205,-3.79149892792447,-3.78410652161969,
-3.74710213544244,-3.73001793708437,-3.72384423113077,-3.71940166878453,
-3.71471352987746,-3.70722203056161,-3.66863710155652,-3.65631546398605,
-3.65084729615386,-3.64646290060631,-3.64381421307235,-3.64120384542324,
-3.63700107334225,-3.62025719321828,-3.59230640344088,-3.57696863223177,
-3.57099186417255,-3.56657992282527,-3.56182207196605,-3.55397804374203,
-3.52719836237098,-3.50725743768062,-3.49678493994851,-3.49314572741337,
-3.4906405877451,-3.4878070449491,-3.4825315902463,-3.46189736598215,-3.44288580097196,
-3.42509991143467,-3.41885501071075,-3.41440051324379,-3.40973401626855,
-3.40235319539531,-3.36553066063845,-3.34709456543,-3.34197757082293,-3.33917592150492,
-3.33668712098327,-3.33359093629159,-3.32549151930023,-3.2986392514912,
-3.27555184356393,-3.2678827313774,-3.26315915128797,-3.2587326127178,-3.25266185931445,
-3.23774973729583,-3.23323840101226,-3.20883007852156,-3.19271533485041,
-3.18860248720295,-3.18601043490097,-3.18367043807317,-3.179537537448,-3.16449543019859,
-3.13514329638442,-3.11946714048323,-3.11344962767322,-3.10903138551789,
-3.10428867036823,-3.09652209350788,-3.06579020797141,-3.04160158508689,
-3.03672543278749,-3.03397344902604,-3.03146333981517,-3.02764630109747,
-3.01643596510118,-2.9869759230571,-2.96777260568876,-2.96139797963505,
-2.95692138561248,-2.95229144896243,-2.94509696895192,-2.91390510725203),
 .UNSPECIFIED.);
#224=B_SPLINE_CURVE_WITH_KNOTS('',3,(#20414,#20415,#20416,#20417,#20418,
#20419,#20420,#20421,#20422,#20423,#20424,#20425,#20426,#20427,#20428,#20429,
#20430,#20431,#20432),.UNSPECIFIED.,.F.,.F.,(4,3,3,3,3,3,4),(3.11344365898459E-7,
0.0233011787387913,0.320469476292411,0.5,0.51186353466473,0.820469476292293,
0.999999999999359),.UNSPECIFIED.);
#225=B_SPLINE_CURVE_WITH_KNOTS('',3,(#20435,#20436,#20437,#20438,#20439,
#20440,#20441,#20442,#20443,#20444,#20445,#20446,#20447,#20448,#20449,#20450,
#20451,#20452,#20453,#20454,#20455,#20456,#20457,#20458,#20459,#20460,#20461,
#20462,#20463,#20464,#20465,#20466,#20467,#20468,#20469,#20470,#20471,#20472,
#20473,#20474,#20475,#20476,#20477,#20478,#20479,#20480,#20481,#20482,#20483,
#20484,#20485,#20486,#20487,#20488,#20489,#20490,#20491,#20492,#20493,#20494,
#20495,#20496,#20497,#20498,#20499,#20500,#20501,#20502,#20503,#20504,#20505,
#20506,#20507,#20508,#20509,#20510,#20511,#20512,#20513,#20514,#20515,#20516,
#20517,#20518,#20519,#20520,#20521,#20522,#20523,#20524,#20525,#20526,#20527,
#20528,#20529,#20530,#20531,#20532),.UNSPECIFIED.,.F.,.F.,(4,2,2,2,2,2,
2,2,2,2,2,2,2,2,2,2,2,2,2,2,2,2,2,2,2,2,2,2,2,2,2,2,2,2,2,2,2,2,2,2,2,2,
2,2,2,2,2,2,4),(8.62633731758881E-5,0.00489546330344884,0.0142706318016333,
0.0445460973104298,0.0630467411669007,0.0693037770110129,0.0736989523517897,
0.0782406243222035,0.0852821894467348,0.124802990275626,0.141850628688387,
0.145989670920605,0.148576444505331,0.151175121296076,0.155488466861705,
0.178558908054217,0.202019090751898,0.216034749297213,0.221750471086131,
0.226027220615217,0.230685578642636,0.238453950532035,0.269014666080015,
0.293684353627655,0.298770656815782,0.301546549909239,0.303950704394756,
0.307358580056001,0.316538424984634,0.33249230058845,0.366143481626674,
0.373591277326783,0.378150253498505,0.38239241413236,0.388145658930972,
0.402721932626938,0.427956648573111,0.447476517083816,0.452584570366893,
0.455349803213659,0.457753117029615,0.46114906629338,0.470153889756483,
0.485582082471485,0.520062889397207,0.52737915856892,0.531908116637689,
0.534920387016673,0.537782073242468),.UNSPECIFIED.);
#226=B_SPLINE_CURVE_WITH_KNOTS('',3,(#20538,#20539,#20540,#20541),
 .UNSPECIFIED.,.F.,.F.,(4,4),(0.971382721880866,0.971517849456709),
 .UNSPECIFIED.);
#227=B_SPLINE_CURVE_WITH_KNOTS('',3,(#20543,#20544,#20545,#20546,#20547,
#20548,#20549,#20550,#20551,#20552),.UNSPECIFIED.,.F.,.F.,(4,3,3,4),(0.,
0.0931868878003157,0.613406353066145,0.999999999998996),.UNSPECIFIED.);
#228=B_SPLINE_CURVE_WITH_KNOTS('',3,(#20555,#20556,#20557,#20558,#20559,
#20560,#20561,#20562,#20563,#20564,#20565,#20566,#20567,#20568,#20569,#20570,
#20571,#20572,#20573,#20574,#20575,#20576,#20577,#20578,#20579,#20580,#20581,
#20582,#20583,#20584,#20585,#20586,#20587,#20588,#20589,#20590,#20591,#20592,
#20593,#20594,#20595,#20596,#20597,#20598,#20599,#20600,#20601,#20602,#20603,
#20604,#20605,#20606,#20607,#20608,#20609,#20610,#20611,#20612,#20613,#20614,
#20615,#20616,#20617,#20618,#20619,#20620,#20621,#20622,#20623,#20624,#20625,
#20626,#20627,#20628,#20629,#20630,#20631,#20632,#20633,#20634,#20635,#20636,
#20637,#20638,#20639,#20640,#20641,#20642),.UNSPECIFIED.,.F.,.F.,(4,2,2,
2,2,2,2,2,2,2,2,2,2,2,2,2,2,2,2,2,2,2,2,2,2,2,2,2,2,2,2,2,2,2,2,2,2,2,2,
2,2,2,2,4),(0.000234844493040472,0.00146418424371738,0.00341290155910423,
0.0105235842651047,0.0435947675953836,0.0652403380488386,0.0713326511653109,
0.074496898121553,0.0768442786627634,0.0797918452300767,0.0848443214240282,
0.108994234681365,0.135616401151146,0.143099789849741,0.148157384505868,
0.150240790666415,0.15174083621689,0.153383032157199,0.156222550817788,
0.167533662195587,0.198103239830759,0.219661864304074,0.224625012836271,
0.227533567510446,0.229855712185375,0.232992693500092,0.239052101197498,
0.260684547479627,0.281545102252944,0.300695542025709,0.30380988239119,
0.305520791106776,0.306959059118639,0.308816983437047,0.312803153697811,
0.329751614485091,0.363453134506496,0.376029122449674,0.380247298277758,
0.382972843708573,0.385398498336505,0.38792367207521,0.391442636254487,
0.395910794425901),.UNSPECIFIED.);
#229=B_SPLINE_CURVE_WITH_KNOTS('',3,(#20648,#20649,#20650,#20651),
 .UNSPECIFIED.,.F.,.F.,(4,4),(3.88500542880906,3.88507765274843),
 .UNSPECIFIED.);
#230=B_SPLINE_CURVE_WITH_KNOTS('',3,(#20652,#20653,#20654,#20655,#20656,
#20657,#20658,#20659,#20660,#20661,#20662,#20663,#20664,#20665,#20666,#20667,
#20668,#20669,#20670,#20671,#20672,#20673,#20674,#20675,#20676,#20677,#20678,
#20679,#20680,#20681,#20682,#20683,#20684,#20685,#20686,#20687,#20688,#20689,
#20690,#20691,#20692,#20693,#20694,#20695,#20696,#20697,#20698,#20699,#20700,
#20701,#20702,#20703,#20704,#20705,#20706,#20707,#20708,#20709,#20710,#20711,
#20712,#20713,#20714,#20715,#20716,#20717,#20718,#20719,#20720,#20721,#20722,
#20723,#20724,#20725,#20726,#20727,#20728,#20729,#20730,#20731,#20732,#20733,
#20734,#20735,#20736,#20737,#20738,#20739,#20740,#20741,#20742,#20743,#20744,
#20745,#20746,#20747,#20748,#20749,#20750,#20751,#20752,#20753,#20754,#20755,
#20756,#20757,#20758,#20759,#20760,#20761,#20762,#20763,#20764,#20765,#20766,
#20767,#20768,#20769,#20770,#20771,#20772,#20773,#20774,#20775,#20776,#20777,
#20778,#20779,#20780,#20781,#20782,#20783,#20784,#20785,#20786,#20787,#20788,
#20789,#20790,#20791,#20792,#20793,#20794,#20795,#20796,#20797,#20798,#20799,
#20800,#20801,#20802,#20803,#20804,#20805,#20806,#20807,#20808,#20809,#20810,
#20811,#20812,#20813,#20814,#20815,#20816,#20817,#20818,#20819,#20820,#20821,
#20822,#20823,#20824,#20825,#20826,#20827,#20828,#20829,#20830,#20831,#20832,
#20833,#20834,#20835,#20836,#20837,#20838,#20839,#20840,#20841,#20842,#20843),
 .UNSPECIFIED.,.F.,.F.,(4,2,2,2,2,2,2,2,2,2,2,2,2,2,2,2,2,2,2,2,2,2,2,2,
2,2,2,2,2,2,2,2,2,2,2,2,2,2,2,2,2,2,2,2,2,2,2,2,2,2,2,2,2,2,2,2,2,2,2,2,
2,2,2,2,2,2,2,2,2,2,2,2,2,2,2,2,2,2,2,2,2,2,2,2,2,2,2,2,2,2,2,2,2,2,2,4),
(0.00010723938499698,0.0325187247414615,0.0544725371139445,0.0575983339188545,
0.0592871541663569,0.0607260986265854,0.0625764159723312,0.0666114580245643,
0.0972489748726172,0.118039938923406,0.12618621984718,0.132455473259296,
0.135619249056975,0.138173003785047,0.141108191615718,0.146128011407001,
0.174150022420611,0.194280527218451,0.209426783900504,0.212355910959386,
0.214005042652508,0.21545781729891,0.217386535260743,0.221663145687393,
0.245868482680921,0.278894239275846,0.286186917169818,0.28954662742067,
0.292125179215272,0.294953054612662,0.299590347161342,0.316186033500614,
0.34553556872939,0.362165930058378,0.366122194262503,0.367978103843899,
0.369411413612714,0.371105569223375,0.37420224477463,0.393833070494413,
0.413307470118417,0.437728930353591,0.442639641342819,0.445508952404061,
0.448048188735129,0.451250327337316,0.45779269776308,0.485741215041162,
0.516986055850625,0.520572071624079,0.522376012929019,0.523836159716188,
0.525393711857864,0.527903595431521,0.536715860065318,0.553860138012039,
0.590528931316358,0.596098825485749,0.599429046958941,0.602017534001131,
0.604845373079938,0.609457924076973,0.62757698180739,0.648156752284447,
0.650779948621628,0.672976630071433,0.676122126760828,0.677846444242693,
0.679171577048668,0.681015609814576,0.6847506784207,0.70807317152071,0.743124756883826,
0.748635715824495,0.751966549153858,0.754578867291662,0.757457772803745,
0.762213915144583,0.781977740838373,0.801561242789734,0.824507170834108,
0.828405954858497,0.830497849884236,0.831950627934779,0.833445295207564,
0.835868352091489,0.844813610434875,0.86262868468981,0.900453538272329,
0.906603066920837,0.909641785046459,0.912060551520529,0.914800836309468,
0.919501233589327,0.942373104456299,0.971382721880866),.UNSPECIFIED.);
#231=B_SPLINE_CURVE_WITH_KNOTS('',3,(#20845,#20846,#20847,#20848),
 .UNSPECIFIED.,.F.,.F.,(4,4),(0.395910794425901,0.395980603577569),
 .UNSPECIFIED.);
#232=B_SPLINE_CURVE_WITH_KNOTS('',3,(#20849,#20850,#20851,#20852,#20853,
#20854,#20855,#20856,#20857,#20858,#20859,#20860,#20861,#20862,#20863,#20864,
#20865,#20866,#20867,#20868,#20869,#20870,#20871,#20872,#20873,#20874,#20875,
#20876,#20877,#20878,#20879,#20880,#20881,#20882,#20883,#20884,#20885,#20886,
#20887,#20888,#20889,#20890,#20891,#20892,#20893,#20894,#20895,#20896,#20897,
#20898,#20899,#20900,#20901,#20902,#20903,#20904,#20905,#20906,#20907,#20908,
#20909,#20910,#20911,#20912,#20913,#20914,#20915,#20916,#20917,#20918,#20919,
#20920,#20921,#20922,#20923,#20924,#20925,#20926,#20927,#20928,#20929,#20930,
#20931,#20932,#20933,#20934,#20935,#20936,#20937,#20938,#20939,#20940,#20941,
#20942,#20943,#20944,#20945,#20946,#20947,#20948,#20949,#20950,#20951,#20952,
#20953,#20954,#20955,#20956,#20957,#20958,#20959,#20960,#20961,#20962,#20963,
#20964,#20965,#20966,#20967,#20968,#20969,#20970,#20971,#20972,#20973,#20974,
#20975,#20976,#20977,#20978,#20979,#20980,#20981,#20982,#20983,#20984,#20985,
#20986,#20987,#20988,#20989,#20990,#20991,#20992,#20993,#20994,#20995,#20996,
#20997,#20998,#20999,#21000,#21001,#21002,#21003,#21004,#21005,#21006,#21007,
#21008,#21009,#21010,#21011,#21012,#21013,#21014,#21015,#21016,#21017,#21018,
#21019,#21020,#21021,#21022,#21023,#21024,#21025,#21026,#21027,#21028,#21029,
#21030,#21031,#21032,#21033,#21034,#21035,#21036,#21037,#21038,#21039,#21040),
 .UNSPECIFIED.,.F.,.F.,(4,2,2,2,2,2,2,2,2,2,2,2,2,2,2,2,2,2,2,2,2,2,2,2,
2,2,2,2,2,2,2,2,2,2,2,2,2,2,2,2,2,2,2,2,2,2,2,2,2,2,2,2,2,2,2,2,2,2,2,2,
2,2,2,2,2,2,2,2,2,2,2,2,2,2,2,2,2,2,2,2,2,2,2,2,2,2,2,2,2,2,2,2,2,2,2,4),
(9.9999999796755E-7,0.02519092473315,0.0564025880721698,0.0616559800192072,
0.0637316023650858,0.0651999446191349,0.0668019206662103,0.0694848898638641,
0.0790681216699718,0.106175768478792,0.133394245650913,0.138446429899689,
0.141377475176916,0.143960024998273,0.147202921781375,0.153568097338929,
0.186356224183761,0.205581266730133,0.21191672535024,0.216378598227054,
0.218339147871063,0.21980092101262,0.221473877686754,0.224398440116991,
0.237776146358797,0.262138962502371,0.285564999976058,0.291850582258868,
0.295032065258697,0.297605155500909,0.300568549248421,0.305652693250769,
0.333568857700026,0.365169152721188,0.37060678651047,0.372720564963444,
0.374201757311434,0.37579470633124,0.378441810170241,0.387657508910769,
0.415010559853812,0.442351829245785,0.447395093832823,0.450317863305526,
0.452891051892687,0.456119141701659,0.462658796258345,0.491880569723409,
0.513956596191244,0.520786495528479,0.525501565918187,0.527499328014449,
0.528961232216845,0.530605175812081,0.533480768351148,0.545499219654417,
0.57085035850078,0.594754734797463,0.601100471141146,0.604293562160237,
0.606867200090937,0.609821509125751,0.614866065499073,0.642774862253483,
0.674390605975228,0.679796159409505,0.681906034592995,0.683387469654588,
0.684984439363804,0.687644949509465,0.696985810657996,0.724241673081108,
0.751521510367138,0.756566267650658,0.759491226758494,0.762067194953283,
0.765299977278521,0.771637877409102,0.804989965384699,0.824039851195637,
0.830341354740278,0.834782709217647,0.836734785574818,0.838191394415411,
0.839860934758488,0.842777098139197,0.856042009909667,0.880505979313697,
0.903992705973529,0.910285138291514,0.913466804443258,0.916038436588451,
0.918998346673348,0.924071971441916,0.952345120658601,0.971257865379087),
 .UNSPECIFIED.);
#233=B_SPLINE_CURVE_WITH_KNOTS('',3,(#21045,#21046,#21047,#21048,#21049,
#21050,#21051,#21052,#21053,#21054,#21055,#21056,#21057,#21058,#21059,#21060,
#21061,#21062,#21063,#21064,#21065,#21066,#21067,#21068,#21069,#21070,#21071,
#21072,#21073,#21074,#21075,#21076,#21077,#21078,#21079,#21080,#21081,#21082,
#21083,#21084,#21085,#21086,#21087,#21088,#21089,#21090,#21091,#21092,#21093,
#21094,#21095,#21096,#21097,#21098,#21099,#21100,#21101,#21102,#21103,#21104,
#21105,#21106,#21107,#21108,#21109,#21110,#21111,#21112,#21113,#21114,#21115,
#21116,#21117,#21118,#21119,#21120,#21121,#21122,#21123,#21124,#21125,#21126,
#21127,#21128,#21129,#21130,#21131,#21132,#21133,#21134,#21135,#21136,#21137,
#21138,#21139,#21140,#21141,#21142,#21143,#21144,#21145,#21146,#21147,#21148,
#21149,#21150,#21151,#21152,#21153,#21154,#21155,#21156,#21157,#21158,#21159,
#21160,#21161,#21162,#21163,#21164,#21165,#21166,#21167,#21168,#21169,#21170,
#21171,#21172,#21173,#21174,#21175,#21176,#21177,#21178,#21179,#21180,#21181,
#21182,#21183,#21184,#21185,#21186,#21187,#21188,#21189,#21190,#21191,#21192,
#21193,#21194,#21195,#21196,#21197,#21198,#21199,#21200,#21201,#21202,#21203,
#21204,#21205,#21206,#21207,#21208,#21209,#21210,#21211,#21212,#21213,#21214,
#21215,#21216,#21217,#21218,#21219,#21220,#21221,#21222,#21223,#21224,#21225,
#21226,#21227,#21228,#21229,#21230,#21231,#21232,#21233,#21234,#21235,#21236,
#21237,#21238,#21239,#21240,#21241,#21242,#21243,#21244,#21245,#21246,#21247,
#21248,#21249,#21250),.UNSPECIFIED.,.F.,.F.,(4,2,2,2,2,2,2,2,2,2,2,2,2,
2,2,2,2,2,2,2,2,2,2,2,2,2,2,2,2,2,2,2,2,2,2,2,2,2,2,2,2,2,2,2,2,2,2,2,2,
2,2,2,2,2,2,2,2,2,2,2,2,2,2,2,2,2,2,2,2,2,2,2,2,2,2,2,2,2,2,2,2,2,2,2,2,
2,2,2,2,2,2,2,2,2,2,2,2,2,2,2,2,2,4),(2.91363847548873,2.92846992430067,
2.9350037570659,2.93822435847139,2.9407892795551,2.94370003308178,2.94871529797709,
2.97539590091814,3.00163345244596,3.01244030335717,3.01522552220558,3.01684535898034,
3.01830721705526,3.0203326637322,3.02523830887129,3.0324500724466,3.05703095222732,
3.08310147634826,3.0896067236805,3.09282193493012,3.09538651111843,3.09830111136425,
3.10333388046192,3.13064857064572,3.15794469573232,3.16727920182255,3.16993216976661,
3.1715230771442,3.17299676052353,3.17509224043723,3.18044210440504,3.21188177216223,
3.24014375118115,3.24514046985061,3.24807586495119,3.25063824712196,3.25382388106003,
3.26017575008762,3.28422343262169,3.30985634038819,3.32152127499904,3.32436726635071,
3.32600045416016,3.32745808321209,3.32945562095726,3.33419227433353,3.3410696018987,
3.36347202072606,3.39225530415368,3.39878904836501,3.40200957470853,3.40457441166448,
3.40748503655207,3.41249997330323,3.43916916861822,3.46538510161361,3.47622728940209,
3.47901516489793,3.4806355529561,3.48209722001825,3.48412136315025,3.48901874827911,
3.49621381119142,3.52067755869478,3.5492957521086,3.55432286424874,3.55726513610132,
3.55982690613964,3.56300319099291,3.56930697945768,3.59296538608811,3.61778457682974,
3.63059294607692,3.63347815776497,3.63513682593029,3.6365890294428,3.63854103762135,
3.64300479014127,3.64935395955308,3.66869093849567,3.70156201422261,3.70793168799658,
3.71116385984767,3.71373107656037,3.71663708756684,3.72162556090924,3.74736062303953,
3.77185899830765,3.78512965865827,3.7880391861883,3.78970331034777,3.79100705499865,
3.79285973693038,3.79678624329087,3.81312212407598,3.84374498333481,3.85947673479073,
3.86404209704228,3.8668545262212,3.86932980156745,3.87183462723816,3.87508034379017,
3.88500542880906),.UNSPECIFIED.);
#234=B_SPLINE_CURVE_WITH_KNOTS('',3,(#21251,#21252,#21253,#21254,#21255,
#21256,#21257,#21258,#21259,#21260,#21261,#21262,#21263,#21264,#21265,#21266,
#21267,#21268,#21269,#21270,#21271,#21272,#21273,#21274,#21275,#21276,#21277,
#21278,#21279,#21280,#21281,#21282,#21283,#21284,#21285,#21286,#21287,#21288,
#21289,#21290,#21291,#21292,#21293,#21294,#21295,#21296,#21297,#21298,#21299,
#21300,#21301,#21302,#21303,#21304,#21305,#21306,#21307,#21308,#21309,#21310,
#21311,#21312,#21313,#21314,#21315,#21316,#21317,#21318,#21319,#21320,#21321,
#21322,#21323,#21324,#21325,#21326,#21327,#21328,#21329,#21330,#21331,#21332,
#21333,#21334,#21335,#21336,#21337,#21338,#21339,#21340,#21341,#21342,#21343,
#21344,#21345,#21346,#21347,#21348,#21349,#21350,#21351,#21352,#21353,#21354,
#21355,#21356,#21357,#21358,#21359,#21360,#21361,#21362,#21363,#21364,#21365,
#21366,#21367,#21368,#21369,#21370,#21371,#21372,#21373,#21374,#21375,#21376,
#21377,#21378,#21379,#21380,#21381,#21382,#21383,#21384,#21385,#21386,#21387,
#21388,#21389,#21390,#21391,#21392,#21393,#21394,#21395,#21396,#21397,#21398,
#21399,#21400,#21401,#21402,#21403,#21404,#21405,#21406,#21407,#21408,#21409,
#21410,#21411,#21412,#21413,#21414,#21415,#21416,#21417,#21418,#21419,#21420,
#21421,#21422,#21423,#21424,#21425,#21426,#21427,#21428,#21429,#21430,#21431,
#21432,#21433,#21434,#21435,#21436,#21437,#21438,#21439,#21440,#21441,#21442,
#21443,#21444,#21445,#21446,#21447,#21448,#21449,#21450,#21451,#21452,#21453,
#21454,#21455,#21456,#21457,#21458,#21459,#21460,#21461,#21462),
 .UNSPECIFIED.,.F.,.F.,(4,2,2,2,2,2,2,2,2,2,2,2,2,2,2,2,2,2,2,2,2,2,2,2,
2,2,2,2,2,2,2,2,2,2,2,2,2,2,2,2,2,2,2,2,2,2,2,2,2,2,2,2,2,2,2,2,2,2,2,2,
2,2,2,2,2,2,2,2,2,2,2,2,2,2,2,2,2,2,2,2,2,2,2,2,2,2,2,2,2,2,2,2,2,2,2,2,
2,2,2,2,2,2,2,2,2,4),(0.971257865379087,0.976325255804158,0.983962143761288,
0.989081685200867,0.991146399765066,0.99261935824194,0.994233295168095,
0.996971799670707,1.00719264491218,1.03382143376433,1.06072456082819,1.06575934219924,
1.06868220348836,1.07125851377223,1.07449464533364,1.08084868505782,1.11382997239657,
1.13312526446993,1.13947228778614,1.14393769368611,1.14589414297634,1.14735147273487,
1.14901894796997,1.15192538747999,1.16499881532324,1.18959666054105,1.21314384227968,
1.21944408532782,1.22262751146473,1.2251995459957,1.22815880142242,1.23322854545502,
1.26117681299847,1.28541740127014,1.29309564335376,1.29823548258234,1.30030352534595,
1.30177710840145,1.30338965782822,1.30612209305398,1.31627369360075,1.34295132762344,
1.36988319406742,1.3749184436539,1.37784123349403,1.38041727164373,1.38365277619851,
1.39022157974486,1.41718262529436,1.43761462950057,1.4467480392036,1.45257091166774,
1.45474111922433,1.45623301281079,1.45780793621372,1.46036929416519,1.46871670971107,
1.49670760690703,1.52442176842347,1.52947730490398,1.53240441272288,1.53497984635921,
1.53820873780349,1.54474325694021,1.57440412199197,1.59611513982899,1.60288557410263,
1.60757094423572,1.60956493398379,1.61102707837854,1.6126738835161,1.61556337358936,
1.62773580619324,1.65296815940903,1.67681172019271,1.68314856102598,1.68633903496989,
1.68891140214184,1.69186514390001,1.69691082539189,1.72637566256953,1.75012648343322,
1.75722108995571,1.76207137141689,1.7640927858228,1.76555890720528,1.76719213379559,
1.77001927648233,1.78130188580457,1.80716753299769,1.83132094388323,1.8376958511454,
1.84089374947813,1.84344303646357,1.84638287376466,1.85136668970763,1.8749379239436,
1.90357094345627,1.91133048358001,1.91650982504854,1.91858400109638,1.92005855538232,
1.92166844916331,1.92438899032147,1.93440366827172,1.94248326667345),
 .UNSPECIFIED.);
#235=B_SPLINE_CURVE_WITH_KNOTS('',3,(#21467,#21468,#21469,#21470,#21471,
#21472,#21473,#21474,#21475,#21476,#21477,#21478,#21479,#21480,#21481,#21482,
#21483,#21484,#21485,#21486,#21487,#21488,#21489,#21490,#21491,#21492,#21493,
#21494,#21495,#21496,#21497,#21498,#21499,#21500,#21501,#21502,#21503,#21504,
#21505,#21506,#21507,#21508,#21509,#21510,#21511,#21512,#21513,#21514,#21515,
#21516,#21517,#21518,#21519,#21520,#21521,#21522,#21523,#21524,#21525,#21526,
#21527,#21528,#21529,#21530,#21531,#21532,#21533,#21534,#21535,#21536,#21537,
#21538,#21539,#21540,#21541,#21542,#21543,#21544,#21545,#21546,#21547,#21548,
#21549,#21550,#21551,#21552,#21553,#21554,#21555,#21556,#21557,#21558,#21559,
#21560,#21561,#21562,#21563,#21564,#21565,#21566,#21567,#21568,#21569,#21570,
#21571,#21572,#21573,#21574,#21575,#21576,#21577,#21578,#21579,#21580,#21581,
#21582,#21583,#21584,#21585,#21586,#21587,#21588,#21589,#21590,#21591,#21592,
#21593,#21594,#21595,#21596,#21597,#21598,#21599,#21600,#21601,#21602,#21603,
#21604,#21605,#21606,#21607,#21608,#21609,#21610,#21611,#21612,#21613,#21614,
#21615,#21616,#21617,#21618,#21619,#21620,#21621,#21622,#21623,#21624,#21625,
#21626,#21627,#21628,#21629,#21630,#21631,#21632,#21633,#21634,#21635,#21636,
#21637,#21638,#21639,#21640,#21641,#21642,#21643,#21644,#21645,#21646,#21647,
#21648,#21649,#21650,#21651,#21652,#21653,#21654,#21655,#21656,#21657,#21658,
#21659,#21660,#21661,#21662),.UNSPECIFIED.,.F.,.F.,(4,2,2,2,2,2,2,2,2,2,
2,2,2,2,2,2,2,2,2,2,2,2,2,2,2,2,2,2,2,2,2,2,2,2,2,2,2,2,2,2,2,2,2,2,2,2,
2,2,2,2,2,2,2,2,2,2,2,2,2,2,2,2,2,2,2,2,2,2,2,2,2,2,2,2,2,2,2,2,2,2,2,2,
2,2,2,2,2,2,2,2,2,2,2,2,2,2,2,4),(1.94237495036772,1.94253659913532,1.96409512683097,
2.00185039429317,2.0072586395656,2.01057432072849,2.01314890224053,2.01600255190526,
2.02075328911474,2.04114311351225,2.07026986901385,2.08457089645924,2.0875358103584,
2.089212075023,2.09051427689846,2.09234999246578,2.09618267534226,2.11170077327053,
2.1463471246293,2.15949757954353,2.16380268412224,2.16656053774036,2.16916704368215,
2.17270340883202,2.18101782407163,2.21205172661935,2.23707904544012,2.24138069583305,
2.24328263050384,2.24473185985878,2.24639852132983,2.24940039746432,2.26626634298567,
2.30086647801091,2.31406497738209,2.31837520819215,2.32113413029699,2.32374008464055,
2.32727325957176,2.33556834130142,2.36658614775378,2.37409716642295,2.39346041401075,
2.39657274435135,2.3982819605469,2.39972478476211,2.40159520321101,2.40561167478547,
2.42274234098753,2.45259378397755,2.46808790924334,2.47266585788397,2.47548226344961,
2.47806656224483,2.48145729271481,2.48891506478013,2.52223743771716,2.54620570782123,
2.55051754289015,2.55242128098498,2.55387074274075,2.55553632041342,2.55853310653489,
2.57525885906144,2.60941671689506,2.62309673387811,2.62746093204471,2.63023140313683,
2.63283224823109,2.63633371488541,2.64443661403982,2.65588413690852,2.68792724786295,
2.70280799359832,2.7058031157615,2.70748619407393,2.70878744058801,2.71061374550297,
2.71439734538039,2.71950183861378,2.73292586816594,2.76378702805817,2.77762347194152,
2.78200417146369,2.78477825376355,2.7873777403833,2.79087008666148,2.79891783028213,
2.81025920809249,2.85435907783433,2.85927960557419,2.86137154585917,2.8628299232549,
2.86441724114062,2.86705430920708,2.87730208617024,2.89973667215865,2.91363847548873),
 .UNSPECIFIED.);
#236=B_SPLINE_CURVE_WITH_KNOTS('',3,(#21663,#21664,#21665,#21666,#21667,
#21668,#21669,#21670,#21671,#21672,#21673,#21674,#21675,#21676,#21677,#21678,
#21679,#21680,#21681,#21682,#21683,#21684,#21685,#21686,#21687,#21688,#21689,
#21690,#21691,#21692,#21693,#21694,#21695,#21696,#21697,#21698,#21699,#21700,
#21701,#21702,#21703,#21704,#21705,#21706,#21707,#21708,#21709,#21710,#21711,
#21712,#21713,#21714,#21715,#21716,#21717,#21718,#21719,#21720,#21721,#21722,
#21723,#21724,#21725,#21726,#21727,#21728,#21729,#21730,#21731,#21732,#21733,
#21734,#21735,#21736,#21737,#21738,#21739,#21740,#21741,#21742,#21743,#21744,
#21745,#21746,#21747,#21748,#21749,#21750,#21751,#21752,#21753,#21754,#21755,
#21756,#21757,#21758,#21759,#21760,#21761,#21762,#21763,#21764,#21765,#21766,
#21767,#21768,#21769,#21770,#21771,#21772,#21773,#21774,#21775,#21776,#21777,
#21778,#21779,#21780,#21781,#21782,#21783,#21784,#21785,#21786,#21787,#21788,
#21789,#21790,#21791,#21792,#21793,#21794,#21795,#21796,#21797,#21798,#21799,
#21800,#21801,#21802,#21803,#21804,#21805,#21806,#21807,#21808,#21809,#21810,
#21811,#21812,#21813,#21814,#21815,#21816,#21817,#21818,#21819,#21820,#21821,
#21822,#21823,#21824,#21825,#21826,#21827,#21828,#21829,#21830,#21831,#21832,
#21833,#21834,#21835,#21836,#21837,#21838,#21839,#21840,#21841,#21842,#21843,
#21844,#21845,#21846,#21847,#21848,#21849,#21850,#21851,#21852,#21853,#21854),
 .UNSPECIFIED.,.F.,.F.,(4,2,2,2,2,2,2,2,2,2,2,2,2,2,2,2,2,2,2,2,2,2,2,2,
2,2,2,2,2,2,2,2,2,2,2,2,2,2,2,2,2,2,2,2,2,2,2,2,2,2,2,2,2,2,2,2,2,2,2,2,
2,2,2,2,2,2,2,2,2,2,2,2,2,2,2,2,2,2,2,2,2,2,2,2,2,2,2,2,2,2,2,2,2,2,2,4),
(1.94248326667345,1.96117665740519,1.98816504256082,1.99320162058116,1.99612460892992,
1.99870048343877,2.00193533306056,2.00850120578587,2.03655542175966,2.06771854393334,
2.07164915893847,2.0735082861722,2.07481795786207,2.07649179774937,2.07942661952704,
2.09305774849087,2.12273754222689,2.14324551837807,2.14801575984335,2.1508815844196,
2.15346768045551,2.15679921380833,2.16223641388999,2.19981682681802,2.22354290357223,
2.22671240585986,2.22841923764114,2.22986984164467,2.23173234044536,2.23578707225683,
2.26622254667201,2.2933523159578,2.3008638056891,2.30427292507808,2.30686922497771,
2.3096969583169,2.31428990536329,2.32981317854939,2.35920713380074,2.37670650875656,
2.38077052850205,2.38265470246385,2.38410446174985,2.38581823259845,2.3889308611405,
2.40784497213815,2.42811084607846,2.45191551434548,2.45690495479881,2.45984622762602,
2.46239562403442,2.46559218242204,2.47195923437794,2.49604705419999,2.52177327221965,
2.53328053947546,2.53612345368896,2.53776022181072,2.53922544786543,2.54124004219528,
2.54604822331266,2.55305860625372,2.5762630771683,2.60389479596131,2.61049225390588,
2.61373341419378,2.6163101613531,2.61922970599601,2.62424902270143,2.65060109391575,
2.67627533764175,2.6878578450532,2.69070588165652,2.69234379956564,2.69380874096683,
2.69582114787963,2.70061587377952,2.70759963272315,2.73063282106473,2.75851724987628,
2.76509364286982,2.76833083185051,2.77090729639272,2.77382959338312,2.77886148434049,
2.80564165610537,2.83205906085926,2.84259257456498,2.84536381605995,2.84698499897824,
2.84845557525342,2.85050428204258,2.85552140797899,2.86294891921168,2.8890095558369,
2.91380463577067),.UNSPECIFIED.);
#237=B_SPLINE_CURVE_WITH_KNOTS('',3,(#21859,#21860,#21861,#21862,#21863,
#21864,#21865,#21866,#21867,#21868,#21869,#21870,#21871,#21872,#21873,#21874,
#21875,#21876,#21877,#21878,#21879,#21880,#21881,#21882,#21883,#21884,#21885,
#21886,#21887,#21888,#21889,#21890,#21891,#21892,#21893,#21894,#21895,#21896,
#21897,#21898,#21899,#21900,#21901,#21902,#21903,#21904,#21905,#21906,#21907,
#21908,#21909,#21910,#21911,#21912,#21913,#21914,#21915,#21916,#21917,#21918,
#21919,#21920,#21921,#21922,#21923,#21924,#21925,#21926,#21927,#21928,#21929,
#21930,#21931,#21932,#21933,#21934,#21935,#21936,#21937,#21938,#21939,#21940,
#21941,#21942,#21943,#21944,#21945,#21946,#21947,#21948,#21949,#21950,#21951,
#21952,#21953,#21954,#21955,#21956,#21957,#21958,#21959,#21960,#21961,#21962,
#21963,#21964,#21965,#21966,#21967,#21968,#21969,#21970,#21971,#21972,#21973,
#21974,#21975,#21976,#21977,#21978,#21979,#21980,#21981,#21982,#21983,#21984,
#21985,#21986,#21987,#21988,#21989,#21990,#21991,#21992,#21993,#21994,#21995,
#21996,#21997,#21998,#21999,#22000,#22001,#22002,#22003,#22004,#22005,#22006,
#22007,#22008,#22009,#22010,#22011,#22012,#22013,#22014,#22015,#22016,#22017,
#22018,#22019,#22020,#22021,#22022,#22023,#22024,#22025,#22026,#22027,#22028,
#22029,#22030,#22031,#22032,#22033,#22034,#22035,#22036,#22037,#22038,#22039,
#22040,#22041,#22042,#22043,#22044,#22045,#22046,#22047,#22048,#22049,#22050,
#22051,#22052,#22053,#22054,#22055,#22056,#22057,#22058,#22059,#22060,#22061,
#22062,#22063,#22064,#22065,#22066,#22067,#22068),.UNSPECIFIED.,.F.,.F.,
(4,2,2,2,2,2,2,2,2,2,2,2,2,2,2,2,2,2,2,2,2,2,2,2,2,2,2,2,2,2,2,2,2,2,2,
2,2,2,2,2,2,2,2,2,2,2,2,2,2,2,2,2,2,2,2,2,2,2,2,2,2,2,2,2,2,2,2,2,2,2,2,
2,2,2,2,2,2,2,2,2,2,2,2,2,2,2,2,2,2,2,2,2,2,2,2,2,2,2,2,2,2,2,2,2,4),(0.971210180410019,
0.975261496742874,0.994106600701588,1.00036348073205,1.00477761980553,1.00671997089861,
1.00817010981954,1.00983255736165,1.01273618767421,1.0259100314029,1.0504498676663,
1.07397609471919,1.08026287570202,1.08343533175024,1.08599624542203,1.08893999017788,
1.09397570919052,1.12202624026933,1.14693303345406,1.15419233059721,1.15912123074284,
1.16115031821869,1.16261261461269,1.16423052028552,1.16700740171044,1.17770986578371,
1.20400122857697,1.23070963420215,1.23572486237741,1.23863541531787,1.24120005999134,
1.24442018203644,1.25073707171717,1.28428643785143,1.30321538549088,1.30948801878196,
1.31391047558128,1.31585427836146,1.31730458836495,1.31896618149448,1.32186606227585,
1.3349682287126,1.35955862079213,1.38310789328704,1.38939753379382,1.39257054218465,
1.39513148348492,1.39807479955747,1.40310864322361,1.4307536621768,1.4559890974859,
1.46329538543929,1.46824769886415,1.47028056604288,1.47174345287426,1.47335964406156,
1.47612871113095,1.48673168299265,1.51309345768745,1.53984307456524,1.54485944724831,
1.5477702359569,1.55033483416101,1.55355455965989,1.56008489558888,1.58923968240741,
1.61136492567873,1.61819731087374,1.6229105589393,1.6249041105827,1.62636102715067,
1.62799578613998,1.63085002457584,1.64265032168548,1.66816463731992,1.69443121625562,
1.69943344183427,1.70234117507355,1.70490614626822,1.70813042531729,1.71446771173402,
1.7476058422646,1.76681768522387,1.77314302695158,1.7775932495274,1.77954187616466,
1.78099275340665,1.78265151394907,1.78553900513351,1.79840826385534,1.8231625868599,
1.84678694267006,1.85308585862446,1.85626064287922,1.85882165581355,1.86176355651798,
1.86679126908261,1.89487302921753,1.9151291232248,1.93011630653898,1.93304191434742,
1.93469215616608,1.93614501112256,1.9380747945384,1.94237495036772),
 .UNSPECIFIED.);
#238=B_SPLINE_CURVE_WITH_KNOTS('',3,(#22069,#22070,#22071,#22072,#22073,
#22074,#22075,#22076,#22077,#22078,#22079,#22080,#22081,#22082,#22083,#22084,
#22085,#22086,#22087,#22088,#22089,#22090,#22091,#22092,#22093,#22094,#22095,
#22096,#22097,#22098,#22099,#22100,#22101,#22102,#22103,#22104,#22105,#22106,
#22107,#22108,#22109,#22110,#22111,#22112,#22113,#22114,#22115,#22116,#22117,
#22118,#22119,#22120,#22121,#22122,#22123,#22124,#22125,#22126,#22127,#22128,
#22129,#22130,#22131,#22132,#22133,#22134,#22135,#22136,#22137,#22138,#22139,
#22140,#22141,#22142,#22143,#22144,#22145,#22146,#22147,#22148,#22149,#22150,
#22151,#22152,#22153,#22154,#22155,#22156,#22157,#22158,#22159,#22160,#22161,
#22162,#22163,#22164,#22165,#22166,#22167,#22168,#22169,#22170,#22171,#22172,
#22173,#22174,#22175,#22176,#22177,#22178,#22179,#22180,#22181,#22182,#22183,
#22184,#22185,#22186,#22187,#22188,#22189,#22190,#22191,#22192,#22193,#22194,
#22195,#22196,#22197,#22198,#22199,#22200,#22201,#22202,#22203,#22204,#22205,
#22206,#22207,#22208,#22209,#22210,#22211,#22212,#22213,#22214,#22215,#22216,
#22217,#22218,#22219,#22220,#22221,#22222,#22223,#22224,#22225,#22226,#22227,
#22228,#22229,#22230,#22231,#22232,#22233,#22234,#22235,#22236,#22237,#22238,
#22239,#22240,#22241,#22242,#22243,#22244,#22245,#22246,#22247,#22248,#22249,
#22250,#22251,#22252,#22253,#22254,#22255,#22256,#22257,#22258,#22259,#22260,
#22261,#22262,#22263,#22264,#22265,#22266,#22267,#22268,#22269,#22270,#22271,
#22272,#22273,#22274,#22275,#22276),.UNSPECIFIED.,.F.,.F.,(4,2,2,2,2,2,
2,2,2,2,2,2,2,2,2,2,2,2,2,2,2,2,2,2,2,2,2,2,2,2,2,2,2,2,2,2,2,2,2,2,2,2,
2,2,2,2,2,2,2,2,2,2,2,2,2,2,2,2,2,2,2,2,2,2,2,2,2,2,2,2,2,2,2,2,2,2,2,2,
2,2,2,2,2,2,2,2,2,2,2,2,2,2,2,2,2,2,2,2,2,2,2,2,2,4),(2.91380463577067,
2.91558023577488,2.92062618130808,2.92358031518007,2.92615316906034,2.92934443437629,
2.93568344900227,2.95954075360705,2.98479097068585,2.99696999021269,2.99986041191154,
3.00150760920297,3.00296999809474,3.00496417752987,3.00964942673475,3.01641857102645,
3.03812103479389,3.06777817344399,3.07431287501553,3.07754216346911,3.08011806219389,
3.08304585813898,3.08810297454847,3.11583112608264,3.14383779454734,3.15219383664496,
3.15475651621168,3.15633193330948,3.15782406349889,3.15999422601928,3.16581474348366,
3.17494123920076,3.19534119474881,3.2247871699429,3.22983373040736,3.23278812485231,
3.23536114588621,3.23855254101388,3.24489154816366,3.26874694409867,3.2939915060906,
3.30618175967733,3.30907300811698,3.31072045347557,3.31218290329949,3.31417694970153,
3.31886092905509,3.32562744274242,3.34731280902575,3.37699643245793,3.38353122196624,
3.38676065989535,3.38933672597844,3.39226476385495,3.39732243112552,3.42506105053049,
3.45308458564713,3.46142151175627,3.46398219524387,3.46555724141491,3.46704975444102,
3.4692215408972,3.47505284053578,3.48420296014097,3.50471598674893,3.53160979281116,
3.53814656226339,3.54137648854507,3.54395272173579,3.54688071057921,3.55193767871528,
3.57963815438586,3.60759427639966,3.61602233692538,3.61859310767078,3.62017042739307,
3.62166173713894,3.62382690372044,3.62961127745315,3.63865749737499,3.65867039064899,
3.68862288924594,3.6936796302642,3.69663652616528,3.69920964962001,3.70239848356632,
3.70872322063626,3.73246006604158,3.75745128468574,3.77001147430507,3.77288766811954,
3.77454856513064,3.77600784250254,3.77797724530373,3.7825158637303,3.78900141758038,
3.80905589589399,3.8409627958709,3.84736024583427,3.85060579078563,3.85318354678195,
3.8561015952899,3.86111163008662,3.8852916424057),.UNSPECIFIED.);
#239=B_SPLINE_CURVE_WITH_KNOTS('',3,(#22282,#22283,#22284,#22285),
 .UNSPECIFIED.,.F.,.F.,(4,4),(4.85639440324075,4.85640163643273),
 .UNSPECIFIED.);
#240=B_SPLINE_CURVE_WITH_KNOTS('',3,(#22286,#22287,#22288,#22289,#22290,
#22291,#22292,#22293,#22294,#22295,#22296,#22297,#22298,#22299,#22300,#22301,
#22302,#22303,#22304,#22305,#22306,#22307,#22308,#22309,#22310,#22311,#22312,
#22313,#22314,#22315,#22316,#22317,#22318,#22319,#22320,#22321,#22322,#22323,
#22324,#22325,#22326,#22327,#22328,#22329,#22330,#22331,#22332,#22333,#22334,
#22335,#22336,#22337,#22338,#22339,#22340,#22341,#22342,#22343,#22344,#22345,
#22346,#22347,#22348,#22349,#22350,#22351,#22352,#22353,#22354,#22355,#22356,
#22357,#22358,#22359,#22360,#22361,#22362,#22363,#22364,#22365,#22366,#22367,
#22368,#22369,#22370,#22371,#22372,#22373,#22374,#22375,#22376,#22377,#22378,
#22379,#22380,#22381,#22382,#22383,#22384,#22385,#22386,#22387,#22388,#22389,
#22390,#22391,#22392,#22393,#22394,#22395,#22396,#22397,#22398,#22399,#22400,
#22401,#22402,#22403,#22404,#22405,#22406,#22407,#22408,#22409,#22410,#22411,
#22412,#22413,#22414,#22415,#22416,#22417,#22418,#22419,#22420,#22421,#22422,
#22423,#22424,#22425,#22426,#22427,#22428,#22429,#22430,#22431,#22432,#22433,
#22434,#22435,#22436,#22437,#22438,#22439,#22440,#22441,#22442,#22443,#22444,
#22445,#22446,#22447,#22448,#22449,#22450,#22451,#22452,#22453,#22454,#22455,
#22456,#22457,#22458,#22459,#22460,#22461,#22462,#22463,#22464,#22465,#22466,
#22467,#22468,#22469,#22470,#22471,#22472,#22473,#22474,#22475,#22476,#22477,
#22478,#22479,#22480,#22481,#22482,#22483,#22484,#22485,#22486,#22487,#22488,
#22489,#22490,#22491),.UNSPECIFIED.,.F.,.F.,(4,2,2,2,2,2,2,2,2,2,2,2,2,
2,2,2,2,2,2,2,2,2,2,2,2,2,2,2,2,2,2,2,2,2,2,2,2,2,2,2,2,2,2,2,2,2,2,2,2,
2,2,2,2,2,2,2,2,2,2,2,2,2,2,2,2,2,2,2,2,2,2,2,2,2,2,2,2,2,2,2,2,2,2,2,2,
2,2,2,2,2,2,2,2,2,2,2,2,2,2,2,2,2,4),(1.00000000494344E-6,0.00175834446107242,
0.00351802001987414,0.00623450174180225,0.0104376497705416,0.0234537311842529,
0.033898526851978,0.0645977440181031,0.0720635796929351,0.0770950285300956,
0.0791406606262912,0.0806056574754419,0.0822163658602987,0.0849601410301629,
0.0953115684528038,0.121859723686488,0.148720086995578,0.153739794934463,
0.156651398638247,0.159216050547573,0.162434960064653,0.168960487834963,
0.195674234885171,0.219731334588504,0.226865921249746,0.231732405192923,
0.233751370289202,0.235212128255905,0.236834755579364,0.239633104491153,
0.250618548081526,0.27671048144492,0.30330343132107,0.308315483056487,0.311225410308613,
0.3137902267606,0.317011527069953,0.323549707391378,0.350329584820988,0.374317103293988,
0.381441183857816,0.38630236009672,0.388320431739015,0.389781028990109,
0.391404020031621,0.394204129618682,0.40521408987298,0.431287981028016,
0.457870299532301,0.46288195733698,0.465791762509731,0.468356534692227,
0.471577863725021,0.47790053528438,0.511340996447652,0.530345024962821,
0.536631749548814,0.54106165361766,0.543006768903625,0.544457249350533,
0.546118107239259,0.549014709269728,0.562054105165321,0.586689174060207,
0.612485916210867,0.61747369057303,0.620378390903898,0.622943889064307,
0.626173110657204,0.632534154233901,0.665129884854871,0.684723479931867,
0.69111909137914,0.695606264981013,0.697561349841379,0.699013076849338,
0.700668273634879,0.703539939567172,0.716118155241525,0.741079167566029,
0.764799965387285,0.771110959475979,0.774288168938421,0.776849423654191,
0.779789718702168,0.784810029171743,0.811053635071867,0.837445112522644,
0.844911333075698,0.849942907812285,0.851988500992957,0.853453437771141,
0.855064044559905,0.857807574679856,0.868157479231774,0.894705142478403,
0.921564687368944,0.926584169790405,0.929495638051399,0.932060167909693,
0.935278920587192,0.941589134389271,0.971210180410019),.UNSPECIFIED.);
#241=B_SPLINE_CURVE_WITH_KNOTS('',3,(#22493,#22494,#22495,#22496,#22497,
#22498,#22499,#22500,#22501,#22502,#22503,#22504,#22505,#22506,#22507,#22508,
#22509,#22510,#22511,#22512,#22513,#22514,#22515,#22516,#22517,#22518,#22519,
#22520,#22521,#22522,#22523,#22524,#22525,#22526,#22527,#22528,#22529,#22530,
#22531,#22532,#22533,#22534,#22535,#22536,#22537,#22538,#22539,#22540,#22541,
#22542,#22543,#22544,#22545,#22546,#22547,#22548,#22549,#22550,#22551,#22552,
#22553,#22554,#22555,#22556,#22557,#22558,#22559,#22560,#22561,#22562,#22563,
#22564,#22565,#22566,#22567,#22568,#22569,#22570,#22571,#22572,#22573,#22574,
#22575,#22576,#22577,#22578,#22579,#22580,#22581,#22582,#22583,#22584,#22585,
#22586,#22587,#22588,#22589,#22590,#22591,#22592,#22593,#22594,#22595,#22596,
#22597,#22598,#22599,#22600,#22601,#22602,#22603,#22604,#22605,#22606,#22607,
#22608,#22609,#22610,#22611,#22612,#22613,#22614,#22615,#22616,#22617,#22618,
#22619,#22620,#22621,#22622,#22623,#22624,#22625,#22626,#22627,#22628,#22629,
#22630,#22631,#22632,#22633,#22634,#22635,#22636,#22637,#22638,#22639,#22640,
#22641,#22642,#22643,#22644,#22645,#22646,#22647,#22648,#22649,#22650,#22651,
#22652,#22653,#22654,#22655,#22656,#22657,#22658,#22659,#22660,#22661,#22662,
#22663,#22664,#22665,#22666,#22667,#22668,#22669,#22670,#22671,#22672,#22673,
#22674,#22675,#22676,#22677,#22678,#22679,#22680,#22681,#22682,#22683,#22684,
#22685,#22686,#22687,#22688,#22689,#22690,#22691,#22692,#22693,#22694,#22695,
#22696),.UNSPECIFIED.,.F.,.F.,(4,2,2,2,2,2,2,2,2,2,2,2,2,2,2,2,2,2,2,2,
2,2,2,2,2,2,2,2,2,2,2,2,2,2,2,2,2,2,2,2,2,2,2,2,2,2,2,2,2,2,2,2,2,2,2,2,
2,2,2,2,2,2,2,2,2,2,2,2,2,2,2,2,2,2,2,2,2,2,2,2,2,2,2,2,2,2,2,2,2,2,2,2,
2,2,2,2,2,2,2,2,2,4),(3.8852916424057,3.88712357187435,3.91216947743994,
3.9246531922623,3.92752492741152,3.92918482502709,3.93064436526573,3.93261565580514,
3.93716512981121,3.94367145555473,3.96384219122548,3.99558822905864,4.00199128771823,
4.00523801162481,4.00781591189297,4.01073328057202,4.01574000778422,4.04164490123671,
4.06648872724025,4.07925380133357,4.08214462365852,4.0838088761948,4.08526743828527,
4.08723096949413,4.09173541682024,4.09815558014516,4.11784667598959,4.15026463169926,
4.15664360145686,4.15988541073684,4.16246288824127,4.16538348918838,4.17040520475659,
4.19679595052899,4.222532884249,4.23404070996666,4.23688433896004,4.23852159625695,
4.2399873173006,4.24200266999815,4.24681301802354,4.25382686470911,4.27704643474919,
4.30467621364325,4.31127680073499,4.31451920909085,4.31709681847175,4.32001720133888,
4.32503760590402,4.35137965262185,4.37702892191618,4.38866251591199,4.39151463310466,
4.39315377350226,4.39461898862488,4.3966306520774,4.40141849033875,4.40838787240894,
4.4313225042054,4.45936782852854,4.46593563184901,4.46917181948658,4.47174894438843,
4.47467355033144,4.47971340721548,4.50673000075536,4.53353739410063,4.54354954777129,
4.54627087031369,4.54788144324439,4.54935680320084,4.55143235107923,4.55661641116771,
4.5643834559937,4.59306964624377,4.61658370856067,4.62156784010452,4.62450869290741,
4.62705936322379,4.63025965359842,4.63664157293854,4.6608390061161,4.68671506922212,
4.69799859720205,4.7008269822907,4.70246101537498,4.70392793678638,4.70595054604866,
4.71080417987074,4.71790343977355,4.7416770470004,4.77112603927686,4.77616935104553,
4.77912353385828,4.78169738759916,4.78489113496757,4.79123933425002,4.81516140348468,
4.85043472705162,4.85462041813607,4.85590572853124,4.85697161330123),
 .UNSPECIFIED.);
#242=B_SPLINE_CURVE_WITH_KNOTS('',3,(#22697,#22698,#22699,#22700),
 .UNSPECIFIED.,.F.,.F.,(4,4),(9.99999999028984E-7,8.68074318044454E-6),
 .UNSPECIFIED.);
#243=B_SPLINE_CURVE_WITH_KNOTS('',3,(#22705,#22706,#22707,#22708,#22709,
#22710,#22711,#22712,#22713,#22714,#22715,#22716,#22717,#22718,#22719,#22720,
#22721,#22722,#22723,#22724,#22725,#22726,#22727,#22728,#22729,#22730,#22731,
#22732,#22733,#22734,#22735,#22736,#22737,#22738,#22739,#22740,#22741,#22742,
#22743,#22744,#22745,#22746,#22747,#22748,#22749,#22750,#22751,#22752,#22753,
#22754,#22755,#22756,#22757,#22758,#22759,#22760,#22761,#22762,#22763,#22764,
#22765,#22766,#22767,#22768,#22769,#22770,#22771,#22772,#22773,#22774,#22775,
#22776,#22777,#22778,#22779,#22780,#22781,#22782,#22783,#22784,#22785,#22786,
#22787,#22788,#22789,#22790,#22791,#22792,#22793,#22794,#22795,#22796,#22797,
#22798,#22799,#22800,#22801,#22802,#22803,#22804,#22805,#22806,#22807,#22808,
#22809,#22810,#22811,#22812,#22813,#22814,#22815,#22816,#22817,#22818,#22819,
#22820,#22821,#22822,#22823,#22824,#22825,#22826,#22827,#22828,#22829,#22830,
#22831,#22832,#22833,#22834,#22835,#22836,#22837,#22838,#22839,#22840,#22841,
#22842,#22843,#22844,#22845,#22846,#22847,#22848,#22849,#22850,#22851,#22852,
#22853,#22854,#22855,#22856,#22857,#22858,#22859,#22860,#22861,#22862,#22863,
#22864,#22865,#22866,#22867,#22868,#22869,#22870,#22871,#22872,#22873,#22874,
#22875,#22876,#22877,#22878,#22879,#22880,#22881,#22882,#22883,#22884,#22885,
#22886,#22887,#22888,#22889,#22890,#22891,#22892,#22893,#22894,#22895,#22896,
#22897,#22898,#22899,#22900,#22901,#22902),.UNSPECIFIED.,.F.,.F.,(4,2,2,
2,2,2,2,2,2,2,2,2,2,2,2,2,2,2,2,2,2,2,2,2,2,2,2,2,2,2,2,2,2,2,2,2,2,2,2,
2,2,2,2,2,2,2,2,2,2,2,2,2,2,2,2,2,2,2,2,2,2,2,2,2,2,2,2,2,2,2,2,2,2,2,2,
2,2,2,2,2,2,2,2,2,2,2,2,2,2,2,2,2,2,2,2,2,2,2,4),(3.88489243871108,3.92114843911136,
3.92656013571019,3.92987713707966,3.9324522733762,3.93530605983754,3.94005588503002,
3.96041815001304,3.98933486616674,4.0038601255331,4.00684130011541,4.0085214093387,
4.00982332137784,4.01165439266635,4.01546184708096,4.03076426927921,4.0647053273136,
4.07865001671835,4.0830424625509,4.08581931758763,4.08841818411302,4.09190477054171,
4.09991638662898,4.11118802125539,4.15410919928886,4.15999890960721,4.16223883309563,
4.16359119989388,4.16509950099853,4.1673728664512,4.17400499664583,4.18502877768122,
4.2168562802777,4.23287953530137,4.23747879974249,4.2403003640074,4.24288419227716,
4.24626673441922,4.25367470103365,4.28282408075351,4.31122782526017,4.31537292236307,
4.31727616889885,4.31872594402144,4.32039269555107,4.32339348619826,4.34020867853257,
4.37462871920109,4.38803614840836,4.39237002355832,4.3951345729966,4.39773917536513,
4.4012601394897,4.40947670781103,4.44044145439295,4.46571228666464,4.47000530883829,
4.47190607237417,4.47335552999937,4.47502377836822,4.47803160834316,4.49504339424672,
4.53021274530603,4.5428371012365,4.54708648986297,4.54983303028564,4.5524462630988,
4.55601933802338,4.56455681225543,4.57685363467972,4.59718156069749,4.59922542152331,
4.62206633515296,4.62520700258585,4.62692277842189,4.62836538728244,4.63022812195892,
4.63420181190906,4.65094177479742,4.68039786180168,4.69666885651923,4.70129560173763,
4.70412304087402,4.70670510908676,4.71007502098321,4.71741242970433,4.74190433180067,
4.77076194799688,4.77804793297946,4.78047846486467,4.78202057229202,4.78352409031177,
4.78577440122295,4.79222657592678,4.80281629548545,4.83856415593349,4.8506049365565,
4.85389406752718,4.85639440324075),.UNSPECIFIED.);
#244=B_SPLINE_CURVE_WITH_KNOTS('',3,(#22903,#22904,#22905,#22906,#22907,
#22908,#22909,#22910,#22911,#22912,#22913,#22914,#22915,#22916,#22917,#22918,
#22919,#22920,#22921,#22922,#22923,#22924,#22925,#22926,#22927,#22928,#22929,
#22930,#22931,#22932,#22933,#22934,#22935,#22936,#22937,#22938,#22939,#22940,
#22941,#22942,#22943,#22944,#22945,#22946,#22947,#22948,#22949,#22950,#22951,
#22952,#22953,#22954,#22955,#22956,#22957,#22958,#22959,#22960,#22961,#22962,
#22963,#22964,#22965,#22966,#22967,#22968,#22969,#22970,#22971,#22972,#22973,
#22974,#22975,#22976,#22977,#22978,#22979,#22980,#22981,#22982,#22983,#22984,
#22985,#22986,#22987,#22988,#22989,#22990,#22991,#22992,#22993,#22994,#22995,
#22996,#22997,#22998,#22999,#23000,#23001,#23002,#23003,#23004,#23005,#23006,
#23007,#23008,#23009,#23010,#23011,#23012,#23013,#23014,#23015,#23016,#23017,
#23018,#23019,#23020,#23021,#23022,#23023,#23024,#23025,#23026,#23027,#23028,
#23029,#23030,#23031,#23032,#23033,#23034,#23035,#23036,#23037,#23038,#23039,
#23040,#23041,#23042,#23043,#23044,#23045,#23046,#23047,#23048,#23049,#23050,
#23051,#23052,#23053,#23054,#23055,#23056,#23057,#23058,#23059,#23060,#23061,
#23062,#23063,#23064,#23065,#23066,#23067,#23068,#23069,#23070,#23071,#23072,
#23073,#23074,#23075,#23076,#23077,#23078,#23079,#23080,#23081,#23082,#23083,
#23084,#23085,#23086,#23087,#23088,#23089,#23090,#23091,#23092,#23093,#23094,
#23095,#23096,#23097,#23098,#23099,#23100,#23101,#23102,#23103,#23104,#23105,
#23106),.UNSPECIFIED.,.F.,.F.,(4,2,2,2,2,2,2,2,2,2,2,2,2,2,2,2,2,2,2,2,
2,2,2,2,2,2,2,2,2,2,2,2,2,2,2,2,2,2,2,2,2,2,2,2,2,2,2,2,2,2,2,2,2,2,2,2,
2,2,2,2,2,2,2,2,2,2,2,2,2,2,2,2,2,2,2,2,2,2,2,2,2,2,2,2,2,2,2,2,2,2,2,2,
2,2,2,2,2,2,2,2,2,4),(8.68074318044454E-6,0.000834621271518507,0.00173280952585111,
0.00355963114514543,0.00791244521117191,0.0325924078649119,0.0637082748297012,
0.0720437098184778,0.0755925001490042,0.0782098340002669,0.0809808938060275,
0.0853107618666323,0.0985894049359075,0.133103219096935,0.149958024574866,
0.152968375369957,0.154641256738511,0.156097219500549,0.158010376055546,
0.162348137750859,0.185507039412247,0.206264126190896,0.218221226988665,
0.226593471511632,0.230148455544655,0.232766982559044,0.235536212871401,
0.239856756378913,0.25304641563528,0.287648468173131,0.304528149240935,
0.307539607759378,0.309212814345661,0.310668864453939,0.312581885754515,
0.316918317418711,0.340081690107502,0.360840544904464,0.372798664169237,
0.381171621812575,0.384726908647325,0.38734565869906,0.390115124885162,
0.394436036402009,0.40762681910747,0.442231818934014,0.459112937757,0.462124652781375,
0.463798001885804,0.465254176015673,0.467167360261257,0.471504161288867,
0.494669506996137,0.515430130015401,0.527389267783587,0.535762938582636,
0.539318528241047,0.54193750134877,0.544707203430572,0.549028482995861,
0.562220389314955,0.596828336624423,0.613710893310983,0.6167228648631,0.618396356497941,
0.619852654660281,0.621766001865311,0.626103172289309,0.649270491527636,
0.670032883382867,0.681993039275234,0.690367423053537,0.693923315522988,
0.696542511699596,0.699312449710978,0.703634097419727,0.716827128039619,
0.751438022523362,0.768322017045462,0.77133424514177,0.773007879318091,
0.774464301523692,0.776377811703755,0.780715351566238,0.803884647951786,
0.824648813439459,0.83660998283435,0.844985077253225,0.84854127216841,0.851160691368128,
0.853930865465378,0.858252881988832,0.871447042964835,0.906060879208404,
0.922946310159948,0.925958794766932,0.92763257148505,0.929089117746588,
0.931002790934689,0.935340700377612,0.958512009723332,0.971370657581808),
 .UNSPECIFIED.);
#245=B_SPLINE_CURVE_WITH_KNOTS('',3,(#23111,#23112,#23113,#23114,#23115,
#23116,#23117,#23118,#23119,#23120,#23121,#23122,#23123,#23124,#23125,#23126,
#23127,#23128,#23129,#23130,#23131,#23132,#23133,#23134,#23135,#23136,#23137,
#23138,#23139,#23140,#23141,#23142,#23143,#23144,#23145,#23146,#23147,#23148,
#23149,#23150,#23151,#23152,#23153,#23154,#23155,#23156,#23157,#23158,#23159,
#23160,#23161,#23162,#23163,#23164,#23165,#23166,#23167,#23168,#23169,#23170,
#23171,#23172,#23173,#23174,#23175,#23176,#23177,#23178,#23179,#23180,#23181,
#23182,#23183,#23184,#23185,#23186,#23187,#23188,#23189,#23190,#23191,#23192,
#23193,#23194,#23195,#23196,#23197,#23198,#23199,#23200,#23201,#23202,#23203,
#23204,#23205,#23206,#23207,#23208,#23209,#23210,#23211,#23212,#23213,#23214,
#23215,#23216,#23217,#23218,#23219,#23220,#23221,#23222,#23223,#23224,#23225,
#23226,#23227,#23228,#23229,#23230,#23231,#23232,#23233,#23234,#23235,#23236,
#23237,#23238,#23239,#23240,#23241,#23242,#23243,#23244,#23245,#23246,#23247,
#23248,#23249,#23250,#23251,#23252,#23253,#23254,#23255,#23256,#23257,#23258,
#23259,#23260,#23261,#23262,#23263,#23264,#23265,#23266,#23267,#23268,#23269,
#23270,#23271,#23272,#23273,#23274,#23275,#23276,#23277,#23278,#23279,#23280,
#23281,#23282,#23283,#23284,#23285,#23286,#23287,#23288,#23289,#23290,#23291,
#23292,#23293,#23294,#23295,#23296,#23297,#23298,#23299,#23300,#23301,#23302,
#23303,#23304,#23305,#23306,#23307,#23308,#23309,#23310,#23311,#23312,#23313,
#23314,#23315,#23316),.UNSPECIFIED.,.F.,.F.,(4,2,2,2,2,2,2,2,2,2,2,2,2,
2,2,2,2,2,2,2,2,2,2,2,2,2,2,2,2,2,2,2,2,2,2,2,2,2,2,2,2,2,2,2,2,2,2,2,2,
2,2,2,2,2,2,2,2,2,2,2,2,2,2,2,2,2,2,2,2,2,2,2,2,2,2,2,2,2,2,2,2,2,2,2,2,
2,2,2,2,2,2,2,2,2,2,2,2,2,2,2,2,2,4),(2.91352716392038,2.92212482027256,
2.92488138764063,2.92649497879777,2.92795908418521,2.92999858455716,2.93499109717784,
2.94237726532148,2.96818478069313,2.99507394356249,3.00012399632293,3.00307121175156,
3.00563220930499,3.00880097969311,3.01506754852075,3.03842966858025,3.06259523178947,
3.07632777435279,3.07926015573891,3.08092925845763,3.08223289030545,3.08407972677961,
3.08796964960132,3.1039746164507,3.13269775760315,3.15037353985382,3.15509602948967,
3.15794397369396,3.16052054463653,3.16384885099863,3.17095682835366,3.18055687794074,
3.20869358513345,3.23056715658777,3.23369639205691,3.23540958465394,3.23685236330121,
3.23871833615166,3.24270962649622,3.25960832398754,3.28922482092507,3.30519699361634,
3.30979756053083,3.31261925958587,3.31520277733571,3.31858428265464,3.32598734138549,
3.35770729684018,3.38341822677389,3.38770008357308,3.38959880091261,3.39104793077835,
3.39271726118508,3.3957304577294,3.41289943203876,3.44881449936663,3.46069966978749,
3.46486506607815,3.46759374421344,3.47021659919886,3.47384592631169,3.4827415395113,
3.49576147876501,3.51516429080594,3.52239732713388,3.53986462762231,3.54293413492266,
3.5446340214246,3.54607824345045,3.54796252885003,3.55205267116827,3.56985834260623,
3.60009683927851,3.61466321470322,3.61912480443844,3.62191651849675,3.62450968858381,
3.62795903241982,3.63575110225162,3.66165840818371,3.69307743509823,3.69704507335354,
3.69890662198317,3.70034907840885,3.70206560451353,3.70530197039488,3.7305938442555,
3.76612759885566,3.7722999426448,3.77549042435448,3.77805296650026,3.78098446292431,
3.7860964208165,3.81786535163903,3.84752243315254,3.851214243834,3.85305254609228,
3.85452929175845,3.85608352634331,3.85856979805513,3.86711179078751,3.88340845438037,
3.88489243871108),.UNSPECIFIED.);
#246=B_SPLINE_CURVE_WITH_KNOTS('',3,(#23317,#23318,#23319,#23320,#23321,
#23322,#23323,#23324,#23325,#23326,#23327,#23328,#23329,#23330,#23331,#23332,
#23333,#23334,#23335,#23336,#23337,#23338,#23339,#23340,#23341,#23342,#23343,
#23344,#23345,#23346,#23347,#23348,#23349,#23350,#23351,#23352,#23353,#23354,
#23355,#23356,#23357,#23358,#23359,#23360,#23361,#23362,#23363,#23364,#23365,
#23366,#23367,#23368,#23369,#23370,#23371,#23372,#23373,#23374,#23375,#23376,
#23377,#23378,#23379,#23380,#23381,#23382,#23383,#23384,#23385,#23386,#23387,
#23388,#23389,#23390,#23391,#23392,#23393,#23394,#23395,#23396,#23397,#23398,
#23399,#23400,#23401,#23402,#23403,#23404,#23405,#23406,#23407,#23408,#23409,
#23410,#23411,#23412,#23413,#23414,#23415,#23416,#23417,#23418,#23419,#23420,
#23421,#23422,#23423,#23424,#23425,#23426,#23427,#23428,#23429,#23430,#23431,
#23432,#23433,#23434,#23435,#23436,#23437,#23438,#23439,#23440,#23441,#23442,
#23443,#23444,#23445,#23446,#23447,#23448,#23449,#23450,#23451,#23452,#23453,
#23454,#23455,#23456,#23457,#23458,#23459,#23460,#23461,#23462,#23463,#23464,
#23465,#23466,#23467,#23468,#23469,#23470,#23471,#23472,#23473,#23474,#23475,
#23476,#23477,#23478,#23479,#23480,#23481,#23482,#23483,#23484,#23485,#23486,
#23487,#23488,#23489,#23490,#23491,#23492,#23493,#23494,#23495,#23496,#23497,
#23498,#23499,#23500,#23501,#23502,#23503,#23504,#23505,#23506,#23507,#23508,
#23509,#23510,#23511,#23512,#23513,#23514,#23515,#23516,#23517,#23518,#23519,
#23520,#23521,#23522,#23523,#23524),.UNSPECIFIED.,.F.,.F.,(4,2,2,2,2,2,
2,2,2,2,2,2,2,2,2,2,2,2,2,2,2,2,2,2,2,2,2,2,2,2,2,2,2,2,2,2,2,2,2,2,2,2,
2,2,2,2,2,2,2,2,2,2,2,2,2,2,2,2,2,2,2,2,2,2,2,2,2,2,2,2,2,2,2,2,2,2,2,2,
2,2,2,2,2,2,2,2,2,2,2,2,2,2,2,2,2,2,2,2,2,2,2,2,2,4),(0.971370657581808,
0.979277997018167,0.991240131328745,0.999615911644618,1.00317240498867,
1.00579204656183,1.00856245817241,1.01288485015418,1.02608020317924,1.06069692285973,
1.07758377455686,1.08059651512142,1.08227043426922,1.08372710462119,1.08564094103095,
1.08997922122614,1.11315291153842,1.13392121614515,1.1458838133258,1.15426002370785,
1.15781677380067,1.160436630868,1.16320729453397,1.16753013023196,1.18072731093024,
1.21534631004211,1.23223441952737,1.23524741014308,1.23692147045425,1.23837826515267,
1.2402922668557,1.24463092960056,1.26781085042781,1.28858663131252,1.30054445182912,
1.30891842181223,1.31247499335924,1.31509499395538,1.31786606135251,1.32219005327595,
1.33539569764978,1.37001066950027,1.38689833174362,1.38991151043589,1.39158569855271,
1.3930426201776,1.3949568087112,1.39929597709156,1.42253064686139,1.44337485726503,
1.46128708260616,1.46589493885138,1.46872704178241,1.47132420297448,1.47467246407102,
1.48028947067604,1.49259957033701,1.52517775118101,1.53629503838642,1.54297152385403,
1.5452571055728,1.54677288788755,1.54813185940556,1.55038322408958,1.5563084996177,
1.58629649017889,1.61508764045441,1.62017044177064,1.62310462820691,1.62568116343352,
1.62890465720159,1.63540425449226,1.66676551929197,1.68724691320141,1.69380937879914,
1.69838812140855,1.70036480117645,1.7018253970308,1.70348317868293,1.70634427066025,
1.71860735344789,1.7438013255651,1.76763481318485,1.77397276408173,1.77716480931454,
1.77973891734645,1.78269517899748,1.78774645505725,1.81781380738918,1.84111733777395,
1.84814571851921,1.85296342916564,1.85498032773697,1.85644658375467,1.85808378736496,
1.86092591854467,1.87240512350821,1.898155388249,1.92455457964085,1.92957734258209,
1.93249866801996,1.9350768592819,1.93831966467421,1.94318075099866),
 .UNSPECIFIED.);
#247=B_SPLINE_CURVE_WITH_KNOTS('',3,(#23529,#23530,#23531,#23532,#23533,
#23534,#23535,#23536,#23537,#23538,#23539,#23540,#23541,#23542,#23543,#23544,
#23545,#23546,#23547,#23548,#23549,#23550,#23551,#23552,#23553,#23554,#23555,
#23556,#23557,#23558,#23559,#23560,#23561,#23562,#23563,#23564,#23565,#23566,
#23567,#23568,#23569,#23570,#23571,#23572,#23573,#23574,#23575,#23576,#23577,
#23578,#23579,#23580,#23581,#23582,#23583,#23584,#23585,#23586,#23587,#23588,
#23589,#23590,#23591,#23592,#23593,#23594,#23595,#23596,#23597,#23598,#23599,
#23600,#23601,#23602,#23603,#23604,#23605,#23606,#23607,#23608,#23609,#23610,
#23611,#23612,#23613,#23614,#23615,#23616,#23617,#23618,#23619,#23620,#23621,
#23622,#23623,#23624,#23625,#23626,#23627,#23628,#23629,#23630,#23631,#23632,
#23633,#23634,#23635,#23636,#23637,#23638,#23639,#23640,#23641,#23642,#23643,
#23644,#23645,#23646,#23647,#23648,#23649,#23650,#23651,#23652,#23653,#23654,
#23655,#23656,#23657,#23658,#23659,#23660,#23661,#23662,#23663,#23664,#23665,
#23666,#23667,#23668,#23669,#23670,#23671,#23672,#23673,#23674,#23675,#23676,
#23677,#23678,#23679,#23680,#23681,#23682,#23683,#23684,#23685,#23686,#23687,
#23688,#23689,#23690,#23691,#23692,#23693,#23694,#23695,#23696,#23697,#23698,
#23699,#23700,#23701,#23702,#23703,#23704,#23705,#23706,#23707,#23708,#23709,
#23710,#23711,#23712,#23713,#23714,#23715,#23716,#23717,#23718,#23719,#23720,
#23721,#23722,#23723,#23724,#23725,#23726),.UNSPECIFIED.,.F.,.F.,(4,2,2,
2,2,2,2,2,2,2,2,2,2,2,2,2,2,2,2,2,2,2,2,2,2,2,2,2,2,2,2,2,2,2,2,2,2,2,2,
2,2,2,2,2,2,2,2,2,2,2,2,2,2,2,2,2,2,2,2,2,2,2,2,2,2,2,2,2,2,2,2,2,2,2,2,
2,2,2,2,2,2,2,2,2,2,2,2,2,2,2,2,2,2,2,2,2,2,2,4),(1.94227575636339,1.94606012199988,
1.97571217536218,1.9926199053659,1.99661156625058,1.9984773157092,1.99991972840137,
2.00163227418584,2.00475978212231,2.02651431365555,2.0547111591379,2.06431910950835,
2.0714315889137,2.07476020351083,2.07733627674735,2.08018292812399,2.08490150537415,
2.10251977375633,2.13129096851807,2.1473191074588,2.15121114362269,2.15305812141286,
2.15436150135844,2.15602982093617,2.15895976721434,2.17265670682989,2.19682333204858,
2.22017979226211,2.22644504745562,2.22961311231055,2.23217352947465,2.23512006630898,
2.24016892342347,2.2681614449127,2.29967791704117,2.30510960970925,2.30721706388844,
2.30869254398128,2.31027832891169,2.31290910232146,2.32201267224442,2.34945384016924,
2.37685147897525,2.38188510879577,2.38479950338163,2.38736348806987,2.3905774129512,
2.39707808220417,2.42788725642536,2.45597234416596,2.45977444644796,2.46163928365593,
2.46298912404641,2.46449959847563,2.46678475879825,2.47351408996637,2.48477781593115,
2.51870532238233,2.53265700246679,2.53704967634984,2.53982626438683,2.54242459771294,
2.54591003562909,2.55391700887379,2.56518046371741,2.60799697087485,2.61396822429828,
2.61621926782982,2.61757353405862,2.61907907482276,2.62134002742006,2.62787659692171,
2.63866956121232,2.65850129791815,2.68592481999823,2.69095996101765,2.69390377005905,
2.69646498309967,2.69963812421213,2.70592729348022,2.72947099415938,2.75403918440645,
2.76720130642072,2.77010472802123,2.77176724079776,2.77321758637382,2.77516038021447,
2.77957628986106,2.78583571601702,2.80469402736594,2.83832679364759,2.84463853199626,
2.84785782733945,2.8504226814839,2.85333440283375,2.85835401052689,2.8851860636777,
2.91168153582172,2.91352716392038),.UNSPECIFIED.);
#248=B_SPLINE_CURVE_WITH_KNOTS('',3,(#23727,#23728,#23729,#23730,#23731,
#23732,#23733,#23734,#23735,#23736,#23737,#23738,#23739,#23740,#23741,#23742,
#23743,#23744,#23745,#23746,#23747,#23748,#23749,#23750,#23751,#23752,#23753,
#23754,#23755,#23756,#23757,#23758,#23759,#23760,#23761,#23762,#23763,#23764,
#23765,#23766,#23767,#23768,#23769,#23770,#23771,#23772,#23773,#23774,#23775,
#23776,#23777,#23778,#23779,#23780,#23781,#23782,#23783,#23784,#23785,#23786,
#23787,#23788,#23789,#23790,#23791,#23792,#23793,#23794,#23795,#23796,#23797,
#23798,#23799,#23800,#23801,#23802,#23803,#23804,#23805,#23806,#23807,#23808,
#23809,#23810,#23811,#23812,#23813,#23814,#23815,#23816,#23817,#23818,#23819,
#23820,#23821,#23822,#23823,#23824,#23825,#23826,#23827,#23828,#23829,#23830,
#23831,#23832,#23833,#23834,#23835,#23836,#23837,#23838,#23839,#23840,#23841,
#23842,#23843,#23844,#23845,#23846,#23847,#23848,#23849,#23850,#23851,#23852,
#23853,#23854,#23855,#23856,#23857,#23858,#23859,#23860,#23861,#23862,#23863,
#23864,#23865,#23866,#23867,#23868,#23869,#23870,#23871,#23872,#23873,#23874,
#23875,#23876,#23877,#23878,#23879,#23880,#23881,#23882,#23883,#23884,#23885,
#23886,#23887,#23888,#23889,#23890,#23891,#23892,#23893,#23894,#23895,#23896,
#23897,#23898,#23899,#23900,#23901,#23902,#23903,#23904,#23905,#23906,#23907,
#23908,#23909,#23910,#23911,#23912,#23913,#23914,#23915,#23916,#23917,#23918,
#23919,#23920,#23921,#23922,#23923,#23924,#23925,#23926),.UNSPECIFIED.,
 .F.,.F.,(4,2,2,2,2,2,2,2,2,2,2,2,2,2,2,2,2,2,2,2,2,2,2,2,2,2,2,2,2,2,2,
2,2,2,2,2,2,2,2,2,2,2,2,2,2,2,2,2,2,2,2,2,2,2,2,2,2,2,2,2,2,2,2,2,2,2,2,
2,2,2,2,2,2,2,2,2,2,2,2,2,2,2,2,2,2,2,2,2,2,2,2,2,2,2,2,2,2,2,2,4),(1.94318075099866,
1.9449198072812,1.97261890963837,1.995819569099,2.00283190549208,2.00764146870455,
2.00965699748318,2.01112302858771,2.01276084670494,2.01560588362152,2.02712858789808,
2.05284750938481,2.07922886835664,2.084251023186,2.08717218475555,2.08975034447495,
2.09299326121901,2.09937520817257,2.13180342803993,2.15151755490416,2.15794295301821,
2.16245013482104,2.16441445003703,2.16587341224631,2.16753794281071,2.17042882170992,
2.18318705438527,2.20802840266903,2.2316957167679,2.23801297545379,2.24120091700669,
2.24377468137401,2.24673381322601,2.25179809407889,2.27867666689431,2.30450972255293,
2.31190868164312,2.3169119821349,2.31895909220625,2.32042997518728,2.32205311836209,
2.32483100450179,2.33543647401551,2.36180396000936,2.38622062984978,2.39262988999964,
2.39583578896418,2.39838725763012,2.40132496488738,2.40629390495854,2.42926122870977,
2.44732319463312,2.46934237407034,2.47248260926525,2.47420309487407,2.47565308593321,
2.47753050985365,2.48155472198726,2.49867808379253,2.52854028639414,2.54404881676014,
2.5486422113095,2.55147112582103,2.55406911058441,2.55748131859959,2.56500325592232,
2.59290053350538,2.62255713928356,2.62625668649689,2.62810130433826,2.62958451847937,
2.63114787730473,2.63365357108196,2.6423172607276,2.65897037247993,2.69609350093568,
2.70158344086033,2.70489551112571,2.70748754357272,2.71033742021486,2.71502821410594,
2.73417146660743,2.75406843857191,2.76100701961687,2.77879231342716,2.78187970926978,
2.7835884278339,2.7850397121151,2.78693338415877,2.79104542149832,2.80897942182484,
2.83958118453618,2.85373662015413,2.85816367452865,2.86095677927945,2.8635672107077,
2.8670640619128,2.87507746271276,2.88633861573731,2.91507246461277),
 .UNSPECIFIED.);
#249=B_SPLINE_CURVE_WITH_KNOTS('',3,(#23931,#23932,#23933,#23934,#23935,
#23936,#23937,#23938,#23939,#23940,#23941,#23942,#23943,#23944,#23945,#23946,
#23947,#23948,#23949,#23950,#23951,#23952,#23953,#23954,#23955,#23956,#23957,
#23958,#23959,#23960,#23961,#23962,#23963,#23964,#23965,#23966,#23967,#23968,
#23969,#23970,#23971,#23972,#23973,#23974,#23975,#23976,#23977,#23978,#23979,
#23980,#23981,#23982,#23983,#23984,#23985,#23986,#23987,#23988,#23989,#23990,
#23991,#23992,#23993,#23994,#23995,#23996,#23997,#23998,#23999,#24000,#24001,
#24002,#24003,#24004,#24005,#24006,#24007,#24008,#24009,#24010,#24011,#24012,
#24013,#24014,#24015,#24016,#24017,#24018,#24019,#24020,#24021,#24022,#24023,
#24024,#24025,#24026,#24027,#24028,#24029,#24030,#24031,#24032,#24033,#24034,
#24035,#24036,#24037,#24038,#24039,#24040,#24041,#24042,#24043,#24044,#24045,
#24046,#24047,#24048,#24049,#24050,#24051,#24052,#24053,#24054,#24055,#24056,
#24057,#24058,#24059,#24060,#24061,#24062,#24063,#24064,#24065,#24066,#24067,
#24068,#24069,#24070,#24071,#24072,#24073,#24074,#24075,#24076,#24077,#24078,
#24079,#24080,#24081,#24082,#24083,#24084,#24085,#24086,#24087,#24088,#24089,
#24090,#24091,#24092,#24093,#24094,#24095,#24096,#24097,#24098,#24099,#24100,
#24101,#24102,#24103,#24104,#24105,#24106,#24107,#24108,#24109,#24110,#24111,
#24112,#24113,#24114,#24115,#24116,#24117,#24118,#24119,#24120,#24121,#24122,
#24123,#24124,#24125,#24126,#24127,#24128,#24129,#24130,#24131,#24132,#24133,
#24134,#24135,#24136),.UNSPECIFIED.,.F.,.F.,(4,2,2,2,2,2,2,2,2,2,2,2,2,
2,2,2,2,2,2,2,2,2,2,2,2,2,2,2,2,2,2,2,2,2,2,2,2,2,2,2,2,2,2,2,2,2,2,2,2,
2,2,2,2,2,2,2,2,2,2,2,2,2,2,2,2,2,2,2,2,2,2,2,2,2,2,2,2,2,2,2,2,2,2,2,2,
2,2,2,2,2,2,2,2,2,2,2,2,2,2,2,2,2,4),(0.971183928329439,0.981978580297393,
0.989401327859789,0.992785759167962,0.995369105059563,0.998188251475987,
1.00277924958466,1.01865391345551,1.04834270021461,1.06528631472166,1.06928197282649,
1.07114847611538,1.07259095302642,1.07430295771319,1.07742799586797,1.09844372534886,
1.12721199756066,1.13691361258339,1.1440783144175,1.14741644304352,1.14999370968088,
1.15283547035284,1.15753132624397,1.17476253752569,1.20373062134106,1.21995788358913,
1.22387281787572,1.22572414150184,1.22702802935362,1.22869344022834,1.23161051040303,
1.24504973305628,1.26939901029108,1.29283771105136,1.2991132856649,1.30228338606068,
1.30484395024269,1.30778900397799,1.31283121134815,1.33961809664802,1.3655305769501,
1.37293124013626,1.3779303025948,1.37997059421145,1.3814345791128,1.38304728676066,
1.38580079242375,1.39621252604107,1.42270758721816,1.44953498976916,1.45455321926251,
1.45746426532755,1.46002860389898,1.46324735662422,1.46955835223679,1.50320419867449,
1.52206384330452,1.52832323121067,1.53273860156304,1.53468106903922,1.53613111878725,
1.53779326134986,1.54069592290172,1.55385477169786,1.57840233772069,1.60193104480362,
1.608217850225,1.61139014617916,1.61395084962223,1.61689426353616,1.6219291953336,
1.64858043756649,1.67461357454576,1.68203078476091,1.68703802966729,1.68907962577979,
1.6905438152654,1.69215593941916,1.69490680327333,1.70528653442309,1.73180419716634,
1.75864494565876,1.76366352646318,1.76657463884147,1.76913895430266,1.77235756962026,
1.7788829580155,1.80844893503423,1.83025608883817,1.84035003586668,1.84297447876203,
1.8445588313716,1.84601816219907,1.8481168146456,1.85202908873096,1.87630100960411,
1.90932997566341,1.91673698068668,1.9201186061708,1.92270155659123,1.92552198879771,
1.93011900053472,1.94227575636339),.UNSPECIFIED.);
#250=B_SPLINE_CURVE_WITH_KNOTS('',3,(#24137,#24138,#24139,#24140,#24141,
#24142,#24143,#24144,#24145,#24146,#24147,#24148,#24149,#24150,#24151,#24152,
#24153,#24154,#24155,#24156,#24157,#24158,#24159,#24160,#24161,#24162,#24163,
#24164,#24165,#24166,#24167,#24168,#24169,#24170,#24171,#24172,#24173,#24174,
#24175,#24176,#24177,#24178,#24179,#24180,#24181,#24182,#24183,#24184,#24185,
#24186,#24187,#24188,#24189,#24190,#24191,#24192,#24193,#24194,#24195,#24196,
#24197,#24198,#24199,#24200,#24201,#24202,#24203,#24204,#24205,#24206,#24207,
#24208,#24209,#24210,#24211,#24212,#24213,#24214,#24215,#24216,#24217,#24218,
#24219,#24220,#24221,#24222,#24223,#24224,#24225,#24226,#24227,#24228,#24229,
#24230,#24231,#24232,#24233,#24234,#24235,#24236,#24237,#24238,#24239,#24240,
#24241,#24242,#24243,#24244,#24245,#24246,#24247,#24248,#24249,#24250,#24251,
#24252,#24253,#24254,#24255,#24256,#24257,#24258,#24259,#24260,#24261,#24262,
#24263,#24264,#24265,#24266,#24267,#24268,#24269,#24270,#24271,#24272,#24273,
#24274,#24275,#24276,#24277,#24278,#24279,#24280,#24281,#24282,#24283,#24284,
#24285,#24286,#24287,#24288,#24289,#24290,#24291,#24292,#24293,#24294,#24295,
#24296,#24297,#24298,#24299,#24300,#24301,#24302,#24303,#24304,#24305,#24306,
#24307,#24308,#24309,#24310,#24311,#24312,#24313,#24314,#24315,#24316,#24317,
#24318,#24319,#24320,#24321,#24322,#24323,#24324,#24325,#24326,#24327,#24328,
#24329,#24330,#24331,#24332,#24333,#24334,#24335,#24336,#24337,#24338,#24339,
#24340,#24341,#24342),.UNSPECIFIED.,.F.,.F.,(4,2,2,2,2,2,2,2,2,2,2,2,2,
2,2,2,2,2,2,2,2,2,2,2,2,2,2,2,2,2,2,2,2,2,2,2,2,2,2,2,2,2,2,2,2,2,2,2,2,
2,2,2,2,2,2,2,2,2,2,2,2,2,2,2,2,2,2,2,2,2,2,2,2,2,2,2,2,2,2,2,2,2,2,2,2,
2,2,2,2,2,2,2,2,2,2,2,2,2,2,2,2,2,4),(2.91507246461277,2.92892983330798,
2.93509516237109,2.93738075274632,2.93874615004116,2.9402548103543,2.94250567280783,
2.94891181939204,2.95937704315373,2.97925187709222,3.00715373703291,3.01220125260113,
3.01515682255433,3.01773123803996,3.02092484345554,3.02726988664468,3.05115966669676,
3.07646309735543,3.08860236958841,3.09148728571456,3.09313389401542,3.09459758556087,
3.09659602088827,3.10130229099896,3.10811100018298,3.13004117415034,3.15943372786153,
3.16597586600442,3.16920776061695,3.17178525325416,3.17471433998824,3.17977234704304,
3.20743104356605,3.2353054443965,3.24386354716294,3.24644888360228,3.24802988722588,
3.24952022680718,3.25167754879362,3.2574029546012,3.26631794597162,3.28782523526673,
3.31655396307781,3.32159623887981,3.32455075938561,3.32712547601933,3.33032103230054,
3.33667535866395,3.36063851848362,3.38609251563041,3.39802302667916,3.40089441631143,
3.40253815581299,3.4040027933226,3.40600728005715,3.41074914141098,3.41762725967811,
3.43998152481581,3.4688258990976,3.47537357560256,3.47860667661035,3.48118443786163,
3.48411308533695,3.48916842141634,3.51670823744944,3.54437765586336,3.55321480934177,
3.55582832848231,3.55741560488964,3.55890269654982,3.56104216523377,3.56664439771152,
3.57529149614558,3.61293861000869,3.62723795007889,3.63168110210604,3.63447809538465,
3.6370878703782,3.64057731917508,3.64854387446908,3.67413671680118,3.70566659648351,
3.70958395400686,3.71144846979611,3.71290030663004,3.71460820413436,3.71777868320359,
3.74141412036115,3.77914121269257,3.78456775338773,3.78789767369664,3.79048541141279,
3.79335600238358,3.79814120537275,3.81885920918604,3.84727462794304,3.86191504451675,
3.8649107962956,3.86659923341252,3.86790791402729,3.86974956384311,3.87358361220623,
3.88714619154448),.UNSPECIFIED.);
#251=B_SPLINE_CURVE_WITH_KNOTS('',3,(#24347,#24348,#24349,#24350,#24351,
#24352,#24353,#24354,#24355,#24356,#24357,#24358,#24359,#24360,#24361,#24362,
#24363,#24364,#24365,#24366,#24367,#24368,#24369,#24370,#24371,#24372,#24373,
#24374,#24375,#24376,#24377,#24378,#24379,#24380,#24381,#24382,#24383,#24384,
#24385,#24386,#24387,#24388,#24389,#24390,#24391,#24392,#24393,#24394,#24395,
#24396,#24397,#24398,#24399,#24400,#24401,#24402,#24403,#24404,#24405,#24406,
#24407,#24408,#24409,#24410,#24411,#24412,#24413,#24414,#24415,#24416,#24417,
#24418,#24419,#24420,#24421,#24422,#24423,#24424,#24425,#24426,#24427,#24428,
#24429,#24430,#24431,#24432,#24433,#24434,#24435,#24436,#24437,#24438,#24439,
#24440,#24441,#24442,#24443,#24444,#24445,#24446,#24447,#24448,#24449,#24450,
#24451,#24452,#24453,#24454,#24455,#24456,#24457,#24458,#24459,#24460,#24461,
#24462,#24463,#24464,#24465,#24466,#24467,#24468,#24469,#24470,#24471,#24472,
#24473,#24474,#24475,#24476,#24477,#24478,#24479,#24480,#24481,#24482,#24483,
#24484,#24485,#24486,#24487,#24488,#24489,#24490,#24491,#24492,#24493,#24494,
#24495,#24496,#24497,#24498,#24499,#24500,#24501,#24502,#24503,#24504,#24505,
#24506,#24507,#24508,#24509,#24510,#24511,#24512,#24513,#24514,#24515,#24516,
#24517,#24518,#24519,#24520,#24521,#24522,#24523,#24524,#24525,#24526,#24527,
#24528,#24529,#24530,#24531,#24532,#24533,#24534,#24535,#24536,#24537,#24538,
#24539,#24540,#24541,#24542,#24543,#24544),.UNSPECIFIED.,.F.,.F.,(4,2,2,
2,2,2,2,2,2,2,2,2,2,2,2,2,2,2,2,2,2,2,2,2,2,2,2,2,2,2,2,2,2,2,2,2,2,2,2,
2,2,2,2,2,2,2,2,2,2,2,2,2,2,2,2,2,2,2,2,2,2,2,2,2,2,2,2,2,2,2,2,2,2,2,2,
2,2,2,2,2,2,2,2,2,2,2,2,2,2,2,2,2,2,2,2,2,2,2,4),(3.71760032817636E-5,0.03278469583082,
0.0563587893830542,0.0626514284411906,0.0658249701322316,0.0683858821371772,
0.0713286585911362,0.076360324979787,0.104235625211231,0.129287446885874,
0.136567454309088,0.14150664053465,0.14353735177536,0.144999865587911,0.146616953652437,
0.14939025023695,0.160047601256219,0.186335777941661,0.21309429534276,0.218110799715376,
0.221021565072916,0.223586083497252,0.226805630064309,0.233120032288051,
0.266710715841159,0.285610033406775,0.29187701324973,0.296296447900073,
0.298239683289246,0.299689884604605,0.301351715648585,0.304252789441236,
0.317379142574959,0.341951324916222,0.365491869975665,0.371780313659773,
0.374953024573585,0.377513869636035,0.380457233485767,0.385491551727468,
0.413050494466129,0.433138625376172,0.443690163139714,0.450125285100344,
0.452372961858122,0.45387560991684,0.455417750302452,0.457849845984146,
0.465152245768651,0.493970927540239,0.52215374812209,0.527206346535803,
0.530124787872092,0.532688246223326,0.535896107075785,0.542365392150518,
0.574187251074119,0.594329771245847,0.600824054159274,0.605362724250848,
0.607326610242817,0.608779387211021,0.610429520813941,0.613279257986403,
0.625509127753051,0.65071582067813,0.676814107350653,0.681811034053337,
0.684717556421354,0.687282572938134,0.690508395188122,0.696853581806874,
0.729811182356325,0.749147142434869,0.75549531249463,0.75995749671615,0.761908156281899,
0.763359235798578,0.765016722442816,0.767898791347565,0.78066927847836,
0.805491972683465,0.829147458303651,0.835450100375146,0.838625531888373,
0.841186490164272,0.844127694061621,0.849152646406451,0.877892520150095,
0.899429983843141,0.908320310967609,0.91402784059735,0.916175851308233,
0.917658770030781,0.919230297849247,0.921796432067453,0.930249207011913,
0.958170814870202,0.971183928329439),.UNSPECIFIED.);
#252=B_SPLINE_CURVE_WITH_KNOTS('',3,(#24546,#24547,#24548,#24549,#24550,
#24551,#24552,#24553,#24554,#24555,#24556,#24557,#24558,#24559,#24560,#24561,
#24562,#24563,#24564,#24565,#24566,#24567,#24568,#24569,#24570,#24571,#24572,
#24573,#24574,#24575,#24576,#24577,#24578,#24579,#24580,#24581,#24582,#24583,
#24584,#24585,#24586,#24587,#24588,#24589,#24590,#24591,#24592,#24593,#24594,
#24595,#24596,#24597,#24598,#24599,#24600,#24601,#24602,#24603,#24604,#24605,
#24606,#24607,#24608,#24609,#24610,#24611,#24612,#24613,#24614,#24615,#24616,
#24617,#24618,#24619,#24620,#24621,#24622,#24623,#24624,#24625,#24626,#24627,
#24628,#24629,#24630,#24631,#24632,#24633,#24634,#24635,#24636,#24637,#24638,
#24639,#24640,#24641,#24642,#24643,#24644,#24645,#24646,#24647,#24648,#24649,
#24650,#24651,#24652,#24653,#24654,#24655,#24656,#24657,#24658,#24659,#24660,
#24661,#24662,#24663,#24664,#24665,#24666,#24667,#24668,#24669,#24670,#24671,
#24672,#24673,#24674,#24675,#24676,#24677,#24678,#24679,#24680,#24681,#24682,
#24683,#24684,#24685,#24686,#24687,#24688,#24689,#24690,#24691,#24692,#24693,
#24694,#24695,#24696,#24697,#24698,#24699,#24700,#24701,#24702,#24703,#24704,
#24705,#24706,#24707,#24708,#24709,#24710,#24711,#24712,#24713,#24714,#24715,
#24716,#24717,#24718,#24719,#24720,#24721,#24722,#24723,#24724,#24725,#24726,
#24727,#24728,#24729,#24730,#24731,#24732,#24733,#24734,#24735,#24736,#24737),
 .UNSPECIFIED.,.F.,.F.,(4,2,2,2,2,2,2,2,2,2,2,2,2,2,2,2,2,2,2,2,2,2,2,2,
2,2,2,2,2,2,2,2,2,2,2,2,2,2,2,2,2,2,2,2,2,2,2,2,2,2,2,2,2,2,2,2,2,2,2,2,
2,2,2,2,2,2,2,2,2,2,2,2,2,2,2,2,2,2,2,2,2,2,2,2,2,2,2,2,2,2,2,2,2,2,2,4),
(3.88714619154448,3.88904047763074,3.92337707087601,3.9368685887607,3.94122442248375,
3.94400268807385,3.94662023297175,3.95015903961425,3.95842150992048,3.9895133701466,
4.01460583942679,4.01891333637113,4.02082217862764,4.02227867611456,4.02395672416928,
4.02698696700417,4.04435119938023,4.07304469944747,4.09081410353643,4.09555711310022,
4.09841863245391,4.1010084819,4.104355632429,4.11151234509875,4.12118754014292,
4.14971225519636,4.17108501371657,4.1742229054481,4.17594309641775,4.17739347450226,
4.17927221962773,4.18330219246631,4.200473585041,4.24287590994943,4.24908514021146,
4.25229262490926,4.25486811507121,4.25781388016512,4.26295004203676,4.29561457726858,
4.3242485980522,4.32843094909298,4.33031747457891,4.3317714145387,4.33346382172003,
4.33656145173604,4.35621865732663,4.38705124106428,4.40094664754376,4.40534698166918,
4.40813472222598,4.41074807879151,4.41426101332378,4.42236778024624,4.43380701886507,
4.47005956901946,4.48118795456977,4.48400603333332,4.48563818755824,4.48710643820127,
4.48913502877977,4.4940224392307,4.50118789742162,4.52539359298118,4.55432540624771,
4.55936779294089,4.56232242904433,4.56489727676177,4.56809303498626,4.57444789680388,
4.59841400940972,4.62387283079741,4.63579905187722,4.63867026231687,4.64031401309601,
4.6417787417417,4.64378346337462,4.6485263765485,4.65540643329968,4.67777163423897,
4.70653285405691,4.71312691302682,4.71636902005457,4.7189476972708,4.72187068583609,
4.72689912781784,4.75344411101109,4.77944225728865,4.79060484515618,4.79342549850228,
4.79505827166498,4.79652644920787,4.79855406078582,4.80343496672445,4.81058731918367,
4.85928900080305),.UNSPECIFIED.);
#253=B_SPLINE_CURVE_WITH_KNOTS('',3,(#24738,#24739,#24740,#24741),
 .UNSPECIFIED.,.F.,.F.,(4,4),(9.99997534344612E-7,6.60003561536544E-5),
 .UNSPECIFIED.);
#254=B_SPLINE_CURVE_WITH_KNOTS('',3,(#24747,#24748,#24749,#24750,#24751,
#24752,#24753,#24754,#24755,#24756,#24757,#24758,#24759,#24760,#24761,#24762,
#24763,#24764,#24765,#24766,#24767,#24768,#24769,#24770,#24771,#24772,#24773,
#24774,#24775,#24776,#24777,#24778,#24779,#24780,#24781,#24782,#24783,#24784,
#24785,#24786,#24787,#24788,#24789,#24790,#24791,#24792,#24793,#24794,#24795,
#24796,#24797,#24798,#24799,#24800,#24801,#24802,#24803,#24804,#24805,#24806,
#24807,#24808,#24809,#24810,#24811,#24812,#24813,#24814,#24815,#24816,#24817,
#24818,#24819,#24820,#24821,#24822,#24823,#24824,#24825,#24826,#24827,#24828,
#24829,#24830,#24831,#24832,#24833,#24834,#24835,#24836,#24837,#24838,#24839,
#24840,#24841,#24842,#24843,#24844,#24845,#24846,#24847,#24848,#24849,#24850,
#24851,#24852,#24853,#24854,#24855,#24856,#24857,#24858,#24859,#24860,#24861,
#24862,#24863,#24864,#24865,#24866,#24867,#24868,#24869,#24870,#24871,#24872,
#24873,#24874,#24875,#24876,#24877,#24878,#24879,#24880,#24881,#24882,#24883,
#24884,#24885,#24886,#24887,#24888,#24889,#24890,#24891,#24892,#24893,#24894,
#24895,#24896,#24897,#24898,#24899,#24900,#24901,#24902,#24903,#24904,#24905,
#24906,#24907,#24908,#24909,#24910,#24911,#24912,#24913,#24914,#24915,#24916,
#24917,#24918,#24919,#24920,#24921,#24922,#24923,#24924,#24925,#24926,#24927,
#24928,#24929,#24930,#24931,#24932,#24933,#24934,#24935,#24936,#24937,#24938,
#24939,#24940,#24941,#24942,#24943,#24944,#24945,#24946,#24947,#24948,#24949,
#24950,#24951,#24952),.UNSPECIFIED.,.F.,.F.,(4,2,2,2,2,2,2,2,2,2,2,2,2,
2,2,2,2,2,2,2,2,2,2,2,2,2,2,2,2,2,2,2,2,2,2,2,2,2,2,2,2,2,2,2,2,2,2,2,2,
2,2,2,2,2,2,2,2,2,2,2,2,2,2,2,2,2,2,2,2,2,2,2,2,2,2,2,2,2,2,2,2,2,2,2,2,
2,2,2,2,2,2,2,2,2,2,2,2,2,2,2,2,2,4),(0.971367835775262,0.998094173292414,
1.00234894763263,1.00424292364808,1.00569151645768,1.0073638562606,1.01039123684256,
1.0279810237121,1.05685453782617,1.07423204822755,1.07893735022615,1.08178157454706,
1.08435900800789,1.08769441721048,1.09484145362972,1.10451150391608,1.13307180573538,
1.1543984102362,1.15752541889822,1.15923809480626,1.16068088479313,1.16254744345115,
1.16654201582585,1.18347064374707,1.21311749279739,1.22906455797877,1.2336443704587,
1.23646155281658,1.23904632060158,1.2424373094354,1.24989413459048,1.27995385018521,
1.30733551430408,1.31114376790517,1.31301029331827,1.31436075156709,1.31587118764701,
1.3181549947914,1.3248707199154,1.33609963139502,1.36992386303947,1.38401729741264,
1.38842559341184,1.39120597995782,1.39380369474847,1.3972819409031,1.405243118424,
1.41641823676776,1.43639857184088,1.46182641650173,1.46611565634774,1.46801566557311,
1.4694649343276,1.47113341770954,1.47414276131796,1.49120327700166,1.52659441990255,
1.53899136783934,1.54321564207803,1.54595669417189,1.54857245185579,1.55216136662084,
1.56079950410705,1.57329785567181,1.59340544813696,1.59873477391159,1.61820286507637,
1.62131736843421,1.62302724251528,1.62447027973268,1.62634052994438,1.63035503934253,
1.64746448333872,1.67729620266772,1.69283846121881,1.6974212522254,1.70023902479084,
1.70282352002554,1.70621296503973,1.71366139995885,1.74124779457326,1.77136409510874,
1.77541529414148,1.77727250381039,1.77871713316958,1.78041405223617,1.78355711624091,
1.8060218451321,1.84431851969616,1.8506303939869,1.85384970621829,1.85641454876322,
1.85932623019209,1.86434570090037,1.89117383312301,1.9181079716179,1.92818047252751,
1.93090284163963,1.93250893244155,1.93389341514821,1.93534591863205,1.93827964096405,
1.942706406208),.UNSPECIFIED.);
#255=B_SPLINE_CURVE_WITH_KNOTS('',3,(#24953,#24954,#24955,#24956),
 .UNSPECIFIED.,.F.,.F.,(4,4),(9.99999999419236E-7,3.71760032817636E-5),
 .UNSPECIFIED.);
#256=B_SPLINE_CURVE_WITH_KNOTS('',3,(#24957,#24958,#24959,#24960,#24961,
#24962,#24963,#24964,#24965,#24966,#24967,#24968,#24969,#24970,#24971,#24972,
#24973,#24974,#24975,#24976,#24977,#24978,#24979,#24980,#24981,#24982,#24983,
#24984,#24985,#24986,#24987,#24988,#24989,#24990,#24991,#24992,#24993,#24994,
#24995,#24996,#24997,#24998,#24999,#25000,#25001,#25002,#25003,#25004,#25005,
#25006,#25007,#25008,#25009,#25010,#25011,#25012,#25013,#25014,#25015,#25016,
#25017,#25018,#25019,#25020,#25021,#25022,#25023,#25024,#25025,#25026,#25027,
#25028,#25029,#25030,#25031,#25032,#25033,#25034,#25035,#25036,#25037,#25038,
#25039,#25040,#25041,#25042,#25043,#25044,#25045,#25046,#25047,#25048,#25049,
#25050,#25051,#25052,#25053,#25054,#25055,#25056,#25057,#25058,#25059,#25060,
#25061,#25062,#25063,#25064,#25065,#25066,#25067,#25068,#25069,#25070,#25071,
#25072,#25073,#25074,#25075,#25076,#25077,#25078,#25079,#25080,#25081,#25082,
#25083,#25084,#25085,#25086,#25087,#25088,#25089,#25090,#25091,#25092,#25093,
#25094,#25095,#25096,#25097,#25098,#25099,#25100,#25101,#25102,#25103,#25104,
#25105,#25106,#25107,#25108,#25109,#25110,#25111,#25112,#25113,#25114,#25115,
#25116,#25117,#25118,#25119,#25120,#25121,#25122,#25123,#25124,#25125,#25126,
#25127,#25128,#25129,#25130,#25131,#25132,#25133,#25134,#25135,#25136,#25137,
#25138,#25139,#25140,#25141,#25142,#25143,#25144,#25145,#25146,#25147,#25148,
#25149,#25150,#25151,#25152,#25153,#25154,#25155,#25156,#25157,#25158,#25159,
#25160,#25161,#25162,#25163,#25164),.UNSPECIFIED.,.F.,.F.,(4,2,2,2,2,2,
2,2,2,2,2,2,2,2,2,2,2,2,2,2,2,2,2,2,2,2,2,2,2,2,2,2,2,2,2,2,2,2,2,2,2,2,
2,2,2,2,2,2,2,2,2,2,2,2,2,2,2,2,2,2,2,2,2,2,2,2,2,2,2,2,2,2,2,2,2,2,2,2,
2,2,2,2,2,2,2,2,2,2,2,2,2,2,2,2,2,2,2,2,2,2,2,2,2,4),(6.60003561536544E-5,
0.00509830578563299,0.00890644455873718,0.0114573845437381,0.0139160719651195,
0.0166825861635177,0.0209902987440654,0.03409017582065,0.06647418236722,
0.0855619923175944,0.0886430328165784,0.0903311055533978,0.091784398664254,
0.0936739598411391,0.0978782754695145,0.126226386619866,0.155161429625844,
0.162710920271129,0.166126662272053,0.168723817356241,0.171548394241512,
0.176126966844707,0.191492877015373,0.221017561224163,0.238563349854191,
0.242632337087529,0.244517393684056,0.245967181396833,0.247680210037605,
0.250789645678147,0.269555154245992,0.275533038578283,0.295550048962192,
0.308110048280513,0.316786121216338,0.320390074735872,0.323016989327633,
0.325770124806536,0.330014283483755,0.342493432290207,0.377791613484175,
0.389347911648222,0.396200583625539,0.398507288812623,0.400026918185239,
0.401381414683244,0.403610987263217,0.409390832399151,0.439483463495319,
0.468315318180592,0.473396399885783,0.476329237391912,0.478904384337202,
0.482125877371935,0.488620531468662,0.520005940590206,0.540444721812987,
0.546997989771674,0.551571281623472,0.553546348169862,0.555005980228067,
0.556662802150842,0.559522898669054,0.571801619368723,0.596966847608817,
0.620780331464314,0.627113507706498,0.630303211074365,0.632875448740539,
0.6358295739681,0.640877203440268,0.668402643247623,0.693707307415768,0.701029982043089,
0.705994512268106,0.708034513594095,0.709503487799869,0.71112810789276,
0.713915700554983,0.724659913984999,0.750915277546541,0.773322479339483,
0.781000187291292,0.784438529645841,0.787039108445138,0.78985409882879,
0.794387348770099,0.809587693452398,0.839289818077307,0.856898933691147,
0.860975159422045,0.862861819644608,0.864312320386488,0.866025869928257,
0.86913446506561,0.887814613287093,0.908797117278246,0.930370431045197,
0.936416771622968,0.93955066073554,0.941872105170914,0.944781910516068,
0.949752290371324,0.971346799428905),.UNSPECIFIED.);
#257=B_SPLINE_CURVE_WITH_KNOTS('',3,(#25170,#25171,#25172,#25173,#25174,
#25175,#25176,#25177,#25178,#25179,#25180,#25181,#25182,#25183,#25184,#25185,
#25186,#25187,#25188),.UNSPECIFIED.,.F.,.F.,(4,3,3,3,3,3,4),(1.57402034594183E-7,
0.0101506090236634,0.320442688740482,0.5,0.505274663924246,0.820442688740574,
0.999999999999516),.UNSPECIFIED.);
#258=B_SPLINE_CURVE_WITH_KNOTS('',3,(#25191,#25192,#25193,#25194,#25195,
#25196,#25197,#25198,#25199,#25200,#25201,#25202,#25203,#25204,#25205,#25206,
#25207,#25208,#25209,#25210,#25211,#25212,#25213,#25214,#25215,#25216,#25217,
#25218,#25219,#25220,#25221,#25222,#25223,#25224,#25225,#25226,#25227,#25228,
#25229,#25230,#25231,#25232,#25233,#25234,#25235,#25236,#25237,#25238,#25239,
#25240,#25241,#25242,#25243,#25244,#25245,#25246,#25247,#25248,#25249,#25250,
#25251,#25252,#25253,#25254,#25255,#25256,#25257,#25258,#25259,#25260,#25261,
#25262,#25263,#25264,#25265,#25266,#25267,#25268,#25269,#25270,#25271,#25272,
#25273,#25274,#25275,#25276,#25277,#25278,#25279,#25280,#25281,#25282,#25283,
#25284,#25285,#25286,#25287,#25288,#25289,#25290,#25291,#25292,#25293,#25294,
#25295,#25296,#25297,#25298,#25299,#25300),.UNSPECIFIED.,.F.,.F.,(4,2,2,
2,2,2,2,2,2,2,2,2,2,2,2,2,2,2,2,2,2,2,2,2,2,2,2,2,2,2,2,2,2,2,2,2,2,2,2,
2,2,2,2,2,2,2,2,2,2,2,2,2,2,2,4),(8.76930096496887E-5,0.00220428059398837,
0.00568383013496389,0.0303307759043643,0.0544825665568798,0.063817873399979,
0.0708027036708884,0.0741337354038329,0.0767392742264438,0.0796478823154546,
0.0845440334456498,0.104800038983582,0.134919545680411,0.142817236007138,
0.148073965356983,0.150185389521897,0.151687239457442,0.153309199107319,
0.156069872786612,0.166411689581759,0.192839035181447,0.219552369491333,
0.224570259786848,0.227485132444039,0.230055393280623,0.233285060518315,
0.239845606163803,0.268990206379869,0.299238582945375,0.302920325304879,
0.304754474096283,0.306227569333834,0.307766498216407,0.310225728504426,
0.318639456612004,0.334585704901009,0.373007914352284,0.378319946253382,
0.381589915132521,0.38413613061569,0.386965017071062,0.391688725824432,
0.412112790855365,0.440792353930564,0.455795390053634,0.45877543143784,
0.460443509871959,0.461736058117411,0.463548094120491,0.467275124240861,
0.492660976406284,0.527829958215341,0.533497363632991,0.535909822943192,
0.537775768622803),.UNSPECIFIED.);
#259=B_SPLINE_CURVE_WITH_KNOTS('',3,(#25306,#25307,#25308,#25309,#25310,
#25311,#25312,#25313,#25314,#25315,#25316,#25317,#25318,#25319,#25320,#25321,
#25322,#25323,#25324,#25325,#25326,#25327,#25328,#25329,#25330),
 .UNSPECIFIED.,.F.,.F.,(4,3,3,3,3,3,3,3,4),(0.,0.157792862860784,0.25,0.402378442421338,
0.5,0.652378442421304,0.75,0.907792862860534,1.),.UNSPECIFIED.);
#260=B_SPLINE_CURVE_WITH_KNOTS('',3,(#25332,#25333,#25334,#25335),
 .UNSPECIFIED.,.F.,.F.,(4,4),(0.155689172965689,0.175303809248541),
 .UNSPECIFIED.);
#261=B_SPLINE_CURVE_WITH_KNOTS('',3,(#25336,#25337,#25338,#25339,#25340,
#25341,#25342,#25343,#25344,#25345,#25346,#25347,#25348,#25349,#25350,#25351,
#25352,#25353),.UNSPECIFIED.,.F.,.F.,(4,2,2,2,2,2,2,2,4),(0.000250941785903305,
0.151853795676273,0.25,0.396282804485723,0.5,0.646282804485731,0.75,0.901853795676217,
1.),.UNSPECIFIED.);
#262=B_SPLINE_CURVE_WITH_KNOTS('',3,(#25358,#25359,#25360,#25361,#25362,
#25363,#25364,#25365,#25366,#25367,#25368,#25369,#25370,#25371,#25372,#25373,
#25374,#25375,#25376,#25377,#25378,#25379,#25380,#25381,#25382,#25383,#25384,
#25385,#25386,#25387,#25388,#25389,#25390,#25391),.UNSPECIFIED.,.F.,.F.,
(4,2,2,2,2,2,2,2,2,2,2,2,2,2,2,2,4),(0.,0.109988325501573,0.125,0.23296026575946,
0.25,0.358354397029719,0.375,0.483378945338423,0.5,0.608294453235343,0.625,
0.733345732989897,0.75,0.857948705197813,0.875,0.984973198402819,1.),
 .UNSPECIFIED.);
#263=B_SPLINE_CURVE_WITH_KNOTS('',3,(#25392,#25393,#25394,#25395,#25396,
#25397,#25398,#25399,#25400,#25401,#25402,#25403,#25404,#25405,#25406,#25407,
#25408,#25409,#25410,#25411,#25412,#25413,#25414,#25415,#25416,#25417,#25418,
#25419,#25420,#25421,#25422,#25423,#25424,#25425,#25426,#25427,#25428,#25429,
#25430,#25431,#25432,#25433,#25434,#25435,#25436,#25437,#25438,#25439,#25440),
 .UNSPECIFIED.,.F.,.F.,(4,3,3,3,3,3,3,3,3,3,3,3,3,3,3,3,4),(0.,0.109983686962011,
0.125,0.232957075765626,0.25,0.358356399835469,0.375,0.48333605083713,0.5,
0.608336050836012,0.625,0.733356399835935,0.75,0.857957075765578,0.875,
0.984983686958202,1.),.UNSPECIFIED.);
#264=B_SPLINE_CURVE_WITH_KNOTS('',3,(#25445,#25446,#25447,#25448,#25449,
#25450,#25451,#25452,#25453,#25454,#25455,#25456,#25457,#25458,#25459,#25460,
#25461,#25462,#25463,#25464,#25465,#25466,#25467,#25468,#25469,#25470,#25471,
#25472,#25473,#25474,#25475,#25476,#25477,#25478,#25479,#25480,#25481,#25482,
#25483,#25484,#25485,#25486,#25487,#25488,#25489,#25490,#25491,#25492,#25493,
#25494,#25495,#25496,#25497,#25498,#25499,#25500,#25501,#25502,#25503,#25504,
#25505,#25506,#25507,#25508,#25509,#25510,#25511,#25512,#25513,#25514,#25515,
#25516,#25517,#25518,#25519,#25520,#25521,#25522,#25523,#25524,#25525,#25526,
#25527,#25528,#25529,#25530,#25531,#25532,#25533,#25534,#25535,#25536,#25537,
#25538,#25539,#25540,#25541,#25542,#25543,#25544,#25545,#25546,#25547,#25548,
#25549,#25550,#25551,#25552,#25553,#25554,#25555,#25556,#25557,#25558,#25559,
#25560,#25561,#25562,#25563,#25564,#25565,#25566,#25567,#25568,#25569,#25570,
#25571,#25572,#25573,#25574,#25575,#25576,#25577,#25578,#25579,#25580,#25581,
#25582,#25583,#25584,#25585,#25586,#25587,#25588,#25589,#25590,#25591,#25592,
#25593,#25594,#25595,#25596,#25597,#25598,#25599,#25600,#25601,#25602,#25603,
#25604,#25605,#25606),.UNSPECIFIED.,.F.,.F.,(4,2,2,2,2,2,2,2,2,2,2,2,2,
2,2,2,2,2,2,2,2,2,2,2,2,2,2,2,2,2,2,2,2,2,2,2,2,2,2,2,2,2,2,2,2,2,2,2,2,
2,2,2,2,2,2,2,2,2,2,2,2,2,2,2,2,2,2,2,2,2,2,2,2,2,2,2,2,2,2,2,4),(-0.796526705481827,
-0.787640941015784,-0.784969985598708,-0.782706384755367,-0.780066614844884,
-0.775590151703796,-0.752801998234308,-0.73096932875452,-0.724386701502598,
-0.71991097401508,-0.715876616314145,-0.709260547728906,-0.681773468829423,
-0.665143928783108,-0.660440991667095,-0.657755123073246,-0.655160601070774,
-0.650908753296221,-0.627054474899414,-0.608279469465114,-0.600484027535724,
-0.595786471325523,-0.591384813002343,-0.585256042011791,-0.554279156357543,
-0.538493813991255,-0.534598057960354,-0.532069788794442,-0.52927476598896,
-0.524020352992956,-0.500326602124289,-0.481261567992463,-0.474440690591909,
-0.469922950426694,-0.465399475628605,-0.458546529915877,-0.440686428309571,
-0.425391380671531,-0.413012908116307,-0.409308093122338,-0.406810597119231,
-0.403936202063164,-0.398260952268314,-0.39025630621729,-0.358566344318047,
-0.350503878294458,-0.345757258247316,-0.341376223416114,-0.335384734570859,
-0.317516357450394,-0.293206087121349,-0.286391165134631,-0.283319629305644,
-0.281106856460015,-0.277898786226338,-0.270189289902916,-0.257367379611346,
-0.230930817331304,-0.224189463729992,-0.220135590777724,-0.215681118104049,
-0.209220088675575,-0.186443729527482,-0.164265495805742,-0.159845809532047,
-0.157217849351324,-0.154571289264464,-0.150060852240392,-0.135115780808072,
-0.104662437121048,-0.0984557913681036,-0.0940863041535525,-0.0894270559394841,
-0.0818344157323819,-0.0609587772238571,-0.0392274395486936,-0.0347847589950281,
-0.032152190913683,-0.0295111793780467,-0.0250260607396291,0.),
 .UNSPECIFIED.);
#265=B_SPLINE_CURVE_WITH_KNOTS('',3,(#25607,#25608,#25609,#25610,#25611,
#25612,#25613,#25614,#25615,#25616,#25617,#25618,#25619,#25620,#25621,#25622,
#25623,#25624,#25625,#25626,#25627,#25628,#25629,#25630,#25631,#25632,#25633,
#25634,#25635,#25636,#25637,#25638,#25639,#25640,#25641,#25642,#25643,#25644,
#25645,#25646,#25647,#25648,#25649,#25650,#25651,#25652,#25653,#25654,#25655),
 .UNSPECIFIED.,.F.,.F.,(4,3,3,3,3,3,3,3,3,3,3,3,3,3,3,3,4),(0.,0.110009589359278,
0.125,0.232983376003898,0.25,0.358382691626032,0.375,0.483362296118791,
0.5,0.60836229611875,0.625,0.733382691626039,0.75,0.857983376004365,0.875,
0.985009589359391,1.),.UNSPECIFIED.);
#266=B_SPLINE_CURVE_WITH_KNOTS('',3,(#25660,#25661,#25662,#25663,#25664,
#25665,#25666,#25667,#25668,#25669,#25670,#25671,#25672,#25673,#25674,#25675,
#25676,#25677,#25678,#25679,#25680,#25681,#25682,#25683,#25684,#25685,#25686,
#25687,#25688,#25689,#25690,#25691,#25692,#25693,#25694,#25695,#25696,#25697,
#25698,#25699,#25700,#25701,#25702,#25703,#25704,#25705,#25706,#25707,#25708,
#25709,#25710,#25711,#25712,#25713,#25714,#25715,#25716,#25717,#25718,#25719,
#25720,#25721,#25722,#25723,#25724,#25725,#25726,#25727,#25728,#25729,#25730,
#25731,#25732,#25733,#25734,#25735,#25736,#25737,#25738,#25739,#25740,#25741,
#25742,#25743,#25744,#25745,#25746,#25747,#25748,#25749,#25750,#25751,#25752,
#25753,#25754,#25755,#25756,#25757,#25758,#25759,#25760,#25761,#25762,#25763,
#25764,#25765,#25766,#25767,#25768,#25769,#25770,#25771,#25772,#25773,#25774,
#25775,#25776,#25777,#25778,#25779,#25780,#25781,#25782,#25783,#25784,#25785,
#25786,#25787,#25788,#25789,#25790,#25791,#25792,#25793,#25794,#25795,#25796,
#25797,#25798,#25799,#25800,#25801,#25802,#25803,#25804,#25805,#25806,#25807,
#25808,#25809,#25810,#25811,#25812,#25813),.UNSPECIFIED.,.F.,.F.,(4,2,2,
2,2,2,2,2,2,2,2,2,2,2,2,2,2,2,2,2,2,2,2,2,2,2,2,2,2,2,2,2,2,2,2,2,2,2,2,
2,2,2,2,2,2,2,2,2,2,2,2,2,2,2,2,2,2,2,2,2,2,2,2,2,2,2,2,2,2,2,2,2,2,2,2,
2,4),(-0.796626433927326,-0.793640581520238,-0.785620283949,-0.75568028508624,
-0.74255056199915,-0.738714547085683,-0.73620663770818,-0.733360336449524,
-0.727905815584501,-0.702584421545849,-0.683830192055982,-0.677728192881519,
-0.673303483107345,-0.668540221178598,-0.660520256434299,-0.630581497681404,
-0.617452316442157,-0.613616460357274,-0.61110865492475,-0.608262471886745,
-0.602808178121058,-0.577487851267826,-0.558734374603957,-0.552632627560487,
-0.548208101052797,-0.543445036838665,-0.535425406142308,-0.505487886405355,
-0.492359247875895,-0.488523550523903,-0.486015848759443,-0.483169782763419,
-0.477715712637789,-0.452396403724468,-0.433643743522045,-0.42754224966276,
-0.423117905796551,-0.418355037238492,-0.410335733214807,-0.380399452822331,
-0.367271365456845,-0.363435827135068,-0.360928229209102,-0.358082281479942,
-0.352628437398602,-0.327310173459904,-0.308558292665218,-0.30245705240812,
-0.298032892820156,-0.293270223102979,-0.285251255457627,-0.255316218204372,
-0.242188661692694,-0.238353282169347,-0.235845788770509,-0.232999961134182,
-0.227546351013326,-0.202229260735234,-0.183477996658464,-0.177377005022688,
-0.172953028529602,-0.168190558605416,-0.160171934513209,-0.130238130612887,
-0.11711111636167,-0.113275894959867,-0.110768503919532,-0.107922787699957,
-0.102469385145431,-0.0771530864554135,-0.0584029324467546,-0.0523021985126006,
-0.0478784013394972,-0.043116116880782,-0.0350977835281825,-0.00516521924404225,
-1.00000002178913E-6),.UNSPECIFIED.);
#267=B_SPLINE_CURVE_WITH_KNOTS('',3,(#25814,#25815,#25816,#25817,#25818,
#25819,#25820,#25821,#25822,#25823,#25824,#25825,#25826,#25827,#25828,#25829,
#25830,#25831,#25832,#25833,#25834,#25835,#25836,#25837,#25838,#25839,#25840,
#25841,#25842,#25843,#25844,#25845,#25846,#25847,#25848,#25849,#25850,#25851,
#25852,#25853,#25854,#25855,#25856,#25857,#25858,#25859,#25860,#25861,#25862),
 .UNSPECIFIED.,.F.,.F.,(4,3,3,3,3,3,3,3,3,3,3,3,3,3,3,3,4),(0.,0.109981554777347,
0.125,0.232954910826536,0.25,0.358354235590002,0.375,0.483333890418085,
0.5,0.608333890420568,0.625,0.73335423558997,0.75,0.857954910826484,0.875,
0.984981554779499,1.),.UNSPECIFIED.);
#268=B_SPLINE_CURVE_WITH_KNOTS('',3,(#25867,#25868,#25869,#25870,#25871,
#25872,#25873,#25874,#25875,#25876,#25877,#25878,#25879,#25880,#25881,#25882,
#25883,#25884,#25885,#25886,#25887,#25888,#25889,#25890,#25891,#25892,#25893,
#25894,#25895,#25896,#25897,#25898,#25899,#25900,#25901,#25902,#25903,#25904,
#25905,#25906,#25907,#25908,#25909,#25910,#25911,#25912,#25913,#25914,#25915,
#25916,#25917,#25918,#25919,#25920,#25921,#25922,#25923,#25924,#25925,#25926,
#25927,#25928,#25929,#25930,#25931,#25932,#25933,#25934,#25935,#25936,#25937,
#25938,#25939,#25940,#25941,#25942,#25943,#25944,#25945,#25946,#25947,#25948,
#25949,#25950,#25951,#25952,#25953,#25954,#25955,#25956,#25957,#25958,#25959,
#25960,#25961,#25962,#25963,#25964,#25965,#25966,#25967,#25968,#25969,#25970,
#25971,#25972,#25973,#25974,#25975,#25976,#25977,#25978,#25979,#25980,#25981,
#25982,#25983,#25984,#25985,#25986,#25987,#25988,#25989,#25990,#25991,#25992,
#25993,#25994,#25995,#25996,#25997,#25998,#25999,#26000,#26001,#26002,#26003,
#26004,#26005,#26006,#26007,#26008,#26009,#26010,#26011,#26012,#26013,#26014,
#26015,#26016,#26017,#26018,#26019,#26020),.UNSPECIFIED.,.F.,.F.,(4,2,2,
2,2,2,2,2,2,2,2,2,2,2,2,2,2,2,2,2,2,2,2,2,2,2,2,2,2,2,2,2,2,2,2,2,2,2,2,
2,2,2,2,2,2,2,2,2,2,2,2,2,2,2,2,2,2,2,2,2,2,2,2,2,2,2,2,2,2,2,2,2,2,2,2,
2,4),(-1.59344183207227,-1.5631015427112,-1.55534294381678,-1.55062716576884,
-1.54617987037097,-1.53993408148607,-1.51654561466502,-1.49445274621809,
-1.49001106992231,-1.4873650768753,-1.48469019848849,-1.48010649463389,
-1.46467298378037,-1.43511927646285,-1.42875749255833,-1.42433622713228,
-1.41966731840556,-1.41216025549249,-1.38170451660708,-1.36811341680057,
-1.36427989319193,-1.36177198004572,-1.35892372442787,-1.35346089649308,
-1.32802390503159,-1.30938174237699,-1.30328092048709,-1.29885564348651,
-1.29409048430771,-1.28606396015132,-1.25612283918375,-1.24299539285905,
-1.23915898984057,-1.23665070166086,-1.23380382118636,-1.22834784155515,
-1.20301380936049,-1.18426530506198,-1.17816246981553,-1.17373704793275,
-1.1689729236065,-1.16095125641983,-1.13100764563381,-1.1178767335622,-1.11404026314902,
-1.11153204316617,-1.10868537408301,-1.10323011271367,-1.07790468242545,
-1.05914900274413,-1.05304625632506,-1.04862099392943,-1.04385712734113,
-1.03583611901101,-1.00589361659963,-0.992762836478716,-0.988926501716389,
-0.986418381926754,-0.983571840315769,-0.978116855299387,-0.952793247609392,
-0.934037529225433,-0.927935018739069,-0.923509937172587,-0.918746274075594,
-0.910725631441768,-0.880784356481209,-0.867654076886061,-0.863817898541952,
-0.861309882207993,-0.85846345937844,-0.853008705277776,-0.827686223767837,
-0.808931201282278,-0.80282894179811,-0.798404043147548,-0.796626433927326),
 .UNSPECIFIED.);
#269=B_SPLINE_CURVE_WITH_KNOTS('',3,(#26021,#26022,#26023,#26024,#26025,
#26026,#26027,#26028,#26029,#26030,#26031,#26032,#26033,#26034,#26035,#26036,
#26037,#26038,#26039,#26040,#26041,#26042,#26043,#26044,#26045,#26046,#26047,
#26048,#26049,#26050,#26051,#26052,#26053,#26054,#26055,#26056,#26057,#26058,
#26059,#26060,#26061,#26062,#26063,#26064,#26065,#26066,#26067,#26068,#26069),
 .UNSPECIFIED.,.F.,.F.,(4,3,3,3,3,3,3,3,3,3,3,3,3,3,3,3,4),(0.,0.109981188115351,
0.125,0.232954538531684,0.25,0.358353863414904,0.375,0.48333351890363,0.5,
0.608333518903562,0.625,0.733353863414284,0.75,0.857954538531691,0.875,
0.984981188108003,1.),.UNSPECIFIED.);
#270=B_SPLINE_CURVE_WITH_KNOTS('',3,(#26074,#26075,#26076,#26077,#26078,
#26079,#26080,#26081,#26082,#26083,#26084,#26085,#26086,#26087,#26088,#26089,
#26090,#26091,#26092,#26093,#26094,#26095,#26096,#26097,#26098,#26099,#26100,
#26101,#26102,#26103,#26104,#26105,#26106,#26107,#26108,#26109,#26110,#26111,
#26112,#26113,#26114,#26115,#26116,#26117,#26118,#26119,#26120,#26121,#26122,
#26123,#26124,#26125,#26126,#26127,#26128,#26129,#26130,#26131,#26132,#26133,
#26134,#26135,#26136,#26137,#26138,#26139,#26140,#26141,#26142,#26143,#26144,
#26145,#26146,#26147,#26148,#26149,#26150,#26151,#26152,#26153,#26154,#26155,
#26156,#26157,#26158,#26159,#26160,#26161,#26162,#26163,#26164,#26165,#26166,
#26167,#26168,#26169,#26170,#26171,#26172,#26173,#26174,#26175,#26176,#26177,
#26178,#26179,#26180,#26181,#26182,#26183,#26184,#26185,#26186,#26187,#26188,
#26189,#26190,#26191,#26192,#26193,#26194,#26195,#26196,#26197,#26198,#26199,
#26200,#26201,#26202,#26203,#26204,#26205,#26206,#26207,#26208,#26209,#26210,
#26211,#26212,#26213,#26214,#26215,#26216,#26217,#26218,#26219,#26220,#26221,
#26222,#26223,#26224,#26225,#26226,#26227,#26228,#26229,#26230,#26231,#26232,
#26233,#26234,#26235,#26236,#26237,#26238,#26239,#26240,#26241,#26242,#26243,
#26244,#26245),.UNSPECIFIED.,.F.,.F.,(4,2,2,2,2,2,2,2,2,2,2,2,2,2,2,2,2,
2,2,2,2,2,2,2,2,2,2,2,2,2,2,2,2,2,2,2,2,2,2,2,2,2,2,2,2,2,2,2,2,2,2,2,2,
2,2,2,2,2,2,2,2,2,2,2,2,2,2,2,2,2,2,2,2,2,2,2,2,2,2,2,2,2,2,2,2,4),(-2.3902143501497,
-2.38554194577431,-2.37447330888417,-2.36950293640176,-2.36547360999595,
-2.36290730182847,-2.36012121013131,-2.3549810250734,-2.33114463532179,
-2.31204084732371,-2.30519157752972,-2.30064291951131,-2.29607627997444,
-2.28912645358936,-2.26886526315001,-2.25201845896579,-2.24578010835845,
-2.24101853522758,-2.23830773888958,-2.23569266117793,-2.23140494962123,
-2.2077432918209,-2.18555443767192,-2.1793330561332,-2.17488984483387,-2.17016681139977,
-2.16236723224184,-2.13072108025255,-2.12242046362916,-2.11659236808856,
-2.11367617722163,-2.11116241447302,-2.10745463890786,-2.09595699927284,
-2.07195583167083,-2.06287276797988,-2.0554987540172,-2.05085433544024,
-2.04641828763313,-2.03996521998969,-2.01108021899938,-1.99944540031978,
-1.99432996199589,-1.99021365590509,-1.98763133580489,-1.98487279251223,
-1.97987276871724,-1.95588491249837,-1.93671199725028,-1.92985340205595,
-1.92530300165537,-1.92073795328766,-1.91379742170667,-1.88949057636316,
-1.8697685298415,-1.86536422909586,-1.86272586726691,-1.86004288106547,
-1.8554188677267,-1.83975708712326,-1.82010937990871,-1.80812066085723,
-1.80270299401605,-1.79834900762235,-1.79320692548309,-1.78303650531064,
-1.75443173353944,-1.7466634593118,-1.74109683931642,-1.73822895069798,
-1.73572809115556,-1.73194035125851,-1.71955185148558,-1.68969650166847,
-1.68112832509411,-1.67626353586041,-1.67186991134657,-1.66610863690228,
-1.65182484725151,-1.62135953938078,-1.61589392031055,-1.61304501981348,
-1.6105371549527,-1.60670451035262,-1.59365382166334,-1.59344183207227),
 .UNSPECIFIED.);
#271=B_SPLINE_CURVE_WITH_KNOTS('',3,(#26246,#26247,#26248,#26249,#26250,
#26251,#26252,#26253,#26254,#26255,#26256,#26257,#26258,#26259,#26260,#26261,
#26262,#26263,#26264,#26265,#26266,#26267,#26268,#26269,#26270,#26271,#26272,
#26273,#26274,#26275,#26276,#26277,#26278,#26279,#26280,#26281,#26282,#26283,
#26284,#26285,#26286,#26287,#26288,#26289,#26290,#26291,#26292,#26293,#26294),
 .UNSPECIFIED.,.F.,.F.,(4,3,3,3,3,3,3,3,3,3,3,3,3,3,3,3,4),(0.,0.110009462588615,
0.125,0.232983247289302,0.25,0.358382562953094,0.375,0.483362167673359,
0.5,0.60836216767328,0.625,0.733382562953116,0.75,0.857983247290714,0.875,
0.985009462590842,1.),.UNSPECIFIED.);
#272=B_SPLINE_CURVE_WITH_KNOTS('',3,(#26300,#26301,#26302,#26303,#26304,
#26305,#26306,#26307,#26308,#26309,#26310,#26311,#26312,#26313,#26314,#26315,
#26316,#26317,#26318,#26319,#26320,#26321,#26322,#26323,#26324),
 .UNSPECIFIED.,.F.,.F.,(4,3,3,3,3,3,3,3,4),(0.,0.125,0.25,0.375,0.5,0.625,
0.75,0.875,1.),.UNSPECIFIED.);
#273=B_SPLINE_CURVE_WITH_KNOTS('',3,(#26327,#26328,#26329,#26330,#26331,
#26332,#26333,#26334,#26335,#26336,#26337,#26338,#26339,#26340,#26341,#26342,
#26343,#26344,#26345,#26346,#26347,#26348,#26349,#26350,#26351,#26352,#26353,
#26354,#26355,#26356,#26357,#26358,#26359,#26360,#26361,#26362,#26363,#26364,
#26365,#26366,#26367,#26368,#26369,#26370,#26371,#26372,#26373,#26374,#26375),
 .UNSPECIFIED.,.F.,.F.,(4,3,3,3,3,3,3,3,3,3,3,3,3,3,3,3,4),(0.,0.109988800771746,
0.125,0.232962268129454,0.25,0.358361590536211,0.375,0.483341232350794,
0.5,0.608341232350757,0.625,0.733361590536065,0.75,0.857962268128102,0.875,
0.984988800771637,0.999999856346085),.UNSPECIFIED.);
#274=B_SPLINE_CURVE_WITH_KNOTS('',3,(#26381,#26382,#26383,#26384,#26385,
#26386,#26387,#26388,#26389,#26390,#26391,#26392,#26393,#26394,#26395,#26396,
#26397,#26398,#26399,#26400,#26401,#26402,#26403,#26404,#26405),
 .UNSPECIFIED.,.F.,.F.,(4,3,3,3,3,3,3,3,4),(0.,0.148099938408352,0.25,0.392428578596628,
0.5,0.642428578596597,0.75,0.898099938408575,1.),.UNSPECIFIED.);
#275=B_SPLINE_CURVE_WITH_KNOTS('',3,(#26408,#26409,#26410,#26411,#26412,
#26413,#26414,#26415,#26416,#26417,#26418,#26419,#26420,#26421,#26422,#26423,
#26424,#26425,#26426,#26427,#26428,#26429,#26430,#26431,#26432),
 .UNSPECIFIED.,.F.,.F.,(4,3,3,3,3,3,3,3,4),(0.,0.125,0.25,0.375,0.5,0.625,
0.75,0.875,1.),.UNSPECIFIED.);
#276=B_SPLINE_CURVE_WITH_KNOTS('',3,(#26437,#26438,#26439,#26440,#26441,
#26442,#26443,#26444,#26445,#26446,#26447,#26448,#26449,#26450,#26451,#26452,
#26453,#26454,#26455,#26456,#26457,#26458,#26459,#26460,#26461,#26462,#26463,
#26464,#26465,#26466,#26467,#26468,#26469,#26470,#26471,#26472,#26473,#26474,
#26475,#26476,#26477,#26478,#26479,#26480,#26481,#26482,#26483,#26484,#26485),
 .UNSPECIFIED.,.F.,.F.,(4,3,3,3,3,3,3,3,3,3,3,3,3,3,3,3,4),(0.,0.109988656217671,
0.125,0.232962121355374,0.25,0.358361443808927,0.375,0.483341085883086,
0.5,0.608341085883097,0.625,0.733361443808902,0.75,0.85796212135537,0.875,
0.984988656217777,1.),.UNSPECIFIED.);
#277=B_SPLINE_CURVE_WITH_KNOTS('',3,(#26486,#26487,#26488,#26489,#26490,
#26491,#26492,#26493,#26494,#26495,#26496,#26497,#26498,#26499,#26500,#26501,
#26502,#26503,#26504,#26505,#26506,#26507,#26508,#26509,#26510,#26511,#26512,
#26513,#26514,#26515,#26516,#26517,#26518,#26519,#26520,#26521,#26522,#26523,
#26524,#26525,#26526,#26527,#26528,#26529,#26530,#26531,#26532,#26533,#26534),
 .UNSPECIFIED.,.F.,.F.,(4,3,3,3,3,3,3,3,3,3,3,3,3,3,3,3,4),(0.,0.110665262381513,
0.125,0.232406990370153,0.25,0.354480944471444,0.375,0.4375,0.5,0.5625,
0.625,0.743596242461822,0.75,0.849347812241323,0.875,0.967457627501634,
1.),.UNSPECIFIED.);
#278=B_SPLINE_CURVE_WITH_KNOTS('',3,(#26539,#26540,#26541,#26542,#26543,
#26544,#26545,#26546,#26547,#26548,#26549,#26550,#26551,#26552,#26553,#26554,
#26555,#26556,#26557,#26558,#26559,#26560,#26561,#26562,#26563,#26564,#26565,
#26566,#26567,#26568,#26569,#26570,#26571,#26572,#26573,#26574,#26575,#26576,
#26577,#26578,#26579,#26580,#26581,#26582,#26583,#26584,#26585,#26586,#26587),
 .UNSPECIFIED.,.F.,.F.,(4,3,3,3,3,3,3,3,3,3,3,3,3,3,3,3,4),(0.,0.110008283622672,
0.125,0.232982050215023,0.25,0.358381366264466,0.375,0.483360973100441,
0.5,0.608360973100499,0.625,0.733381366264475,0.75,0.857982050215031,0.875,
0.985008283625021,1.),.UNSPECIFIED.);
#279=B_SPLINE_CURVE_WITH_KNOTS('',3,(#26588,#26589,#26590,#26591,#26592,
#26593,#26594,#26595,#26596,#26597,#26598,#26599,#26600,#26601,#26602,#26603,
#26604,#26605,#26606,#26607,#26608,#26609,#26610,#26611,#26612,#26613,#26614,
#26615,#26616,#26617,#26618,#26619,#26620,#26621,#26622,#26623,#26624,#26625,
#26626,#26627,#26628,#26629,#26630,#26631,#26632,#26633,#26634,#26635,#26636),
 .UNSPECIFIED.,.F.,.F.,(4,3,3,3,3,3,3,3,3,3,3,3,3,3,3,3,4),(0.,0.109995624518602,
0.125,0.232969196690076,0.25,0.358368516873247,0.375,0.483348146433747,
0.5,0.60834814643373,0.625,0.733368516873222,0.75,0.857969196690087,0.875,
0.984995624518607,1.),.UNSPECIFIED.);
#280=B_SPLINE_CURVE_WITH_KNOTS('',3,(#26641,#26642,#26643,#26644,#26645,
#26646,#26647,#26648,#26649,#26650,#26651,#26652,#26653,#26654,#26655,#26656,
#26657,#26658,#26659,#26660,#26661,#26662,#26663,#26664,#26665,#26666,#26667,
#26668,#26669,#26670,#26671,#26672,#26673,#26674,#26675,#26676,#26677,#26678,
#26679,#26680,#26681,#26682,#26683,#26684,#26685,#26686,#26687,#26688,#26689),
 .UNSPECIFIED.,.F.,.F.,(4,3,3,3,3,3,3,3,3,3,3,3,3,3,3,3,4),(0.,0.109988095064951,
0.125,0.232961551582756,0.25,0.35836087421893,0.375,0.483340517301036,0.5,
0.608340517300975,0.625,0.733360874218944,0.75,0.857961551582776,0.875,
0.984988095064888,1.),.UNSPECIFIED.);
#281=B_SPLINE_CURVE_WITH_KNOTS('',3,(#26690,#26691,#26692,#26693,#26694,
#26695,#26696,#26697,#26698,#26699,#26700,#26701,#26702,#26703,#26704,#26705,
#26706,#26707,#26708,#26709,#26710,#26711,#26712,#26713,#26714,#26715,#26716,
#26717,#26718,#26719,#26720,#26721,#26722,#26723,#26724,#26725,#26726,#26727,
#26728,#26729,#26730,#26731,#26732,#26733,#26734,#26735,#26736,#26737,#26738),
 .UNSPECIFIED.,.F.,.F.,(4,3,3,3,3,3,3,3,3,3,3,3,3,3,3,3,4),(0.,0.110003210421414,
0.125,0.232976899099387,0.25,0.358376216809013,0.375,0.483355832748265,
0.5,0.608355832752626,0.625,0.733376216808992,0.75,0.857976899101109,0.875,
0.98500321042069,1.),.UNSPECIFIED.);
#282=B_SPLINE_CURVE_WITH_KNOTS('',3,(#26743,#26744,#26745,#26746,#26747,
#26748,#26749,#26750,#26751,#26752,#26753,#26754,#26755,#26756,#26757,#26758,
#26759,#26760,#26761,#26762,#26763,#26764,#26765,#26766,#26767,#26768,#26769,
#26770,#26771,#26772,#26773,#26774,#26775,#26776),.UNSPECIFIED.,.F.,.F.,
(4,2,2,2,2,2,2,2,2,2,2,2,2,2,2,2,4),(0.,0.109985596045135,0.125,0.23295933697955,
0.25,0.358356487411939,0.375,0.483342521801201,0.5,0.608357003630201,0.625,
0.733317144881367,0.75,0.857951550631935,0.875,0.984974973868141,1.),
 .UNSPECIFIED.);
#283=B_SPLINE_CURVE_WITH_KNOTS('',3,(#26777,#26778,#26779,#26780,#26781,
#26782,#26783,#26784,#26785,#26786,#26787,#26788,#26789,#26790,#26791,#26792,
#26793,#26794,#26795,#26796,#26797,#26798,#26799,#26800,#26801,#26802,#26803,
#26804,#26805,#26806,#26807,#26808,#26809,#26810,#26811,#26812,#26813,#26814,
#26815,#26816,#26817,#26818,#26819,#26820,#26821,#26822,#26823,#26824,#26825,
#26826,#26827,#26828,#26829,#26830,#26831,#26832,#26833,#26834,#26835,#26836,
#26837,#26838,#26839,#26840,#26841,#26842,#26843,#26844,#26845,#26846),
 .UNSPECIFIED.,.F.,.F.,(4,3,3,3,3,3,3,3,3,3,3,3,3,3,3,3,3,3,3,3,3,3,3,4),
(0.,0.0586198091601681,0.0625,0.125,0.1875,0.25,0.3125,0.375,0.40625,0.4375,
0.46875,0.484375,0.48828125,0.5,0.515625,0.53125,0.5625,0.625,0.6875,0.75,
0.858448953897341,0.875,0.984200206485096,1.),.UNSPECIFIED.);
#284=B_SPLINE_CURVE_WITH_KNOTS('',3,(#26851,#26852,#26853,#26854,#26855,
#26856,#26857,#26858,#26859,#26860,#26861,#26862,#26863,#26864,#26865,#26866,
#26867,#26868,#26869,#26870,#26871,#26872,#26873,#26874,#26875,#26876,#26877,
#26878,#26879,#26880,#26881,#26882,#26883,#26884,#26885,#26886,#26887,#26888,
#26889,#26890,#26891,#26892,#26893,#26894,#26895,#26896,#26897,#26898,#26899),
 .UNSPECIFIED.,.F.,.F.,(4,3,3,3,3,3,3,3,3,3,3,3,3,3,3,3,4),(0.,0.109997341214618,
0.125,0.23297093975572,0.25,0.35837025937904,0.375,0.483349885857099,0.5,
0.608349885857203,0.625,0.733370259379004,0.75,0.857970939755706,0.875,
0.984997341214533,1.),.UNSPECIFIED.);
#285=B_SPLINE_CURVE_WITH_KNOTS('',3,(#26900,#26901,#26902,#26903,#26904,
#26905,#26906,#26907,#26908,#26909,#26910,#26911,#26912,#26913,#26914,#26915,
#26916,#26917,#26918,#26919,#26920,#26921,#26922,#26923,#26924,#26925,#26926,
#26927,#26928,#26929,#26930,#26931,#26932,#26933,#26934,#26935,#26936,#26937,
#26938,#26939,#26940,#26941,#26942,#26943,#26944,#26945,#26946,#26947,#26948),
 .UNSPECIFIED.,.F.,.F.,(4,3,3,3,3,3,3,3,3,3,3,3,3,3,3,3,4),(0.,0.109983123479305,
0.125,0.23295650362664,0.25,0.358355827880222,0.375,0.483335479892581,0.5,
0.608335479892553,0.625,0.733355827880202,0.75,0.857956503626664,0.875,
0.984983123479114,1.),.UNSPECIFIED.);
#286=B_SPLINE_CURVE_WITH_KNOTS('',3,(#26953,#26954,#26955,#26956,#26957,
#26958,#26959,#26960,#26961,#26962,#26963,#26964,#26965,#26966,#26967,#26968,
#26969,#26970,#26971,#26972,#26973,#26974,#26975,#26976,#26977,#26978,#26979,
#26980,#26981,#26982,#26983,#26984,#26985,#26986,#26987,#26988,#26989,#26990,
#26991,#26992,#26993,#26994,#26995,#26996,#26997,#26998,#26999,#27000,#27001),
 .UNSPECIFIED.,.F.,.F.,(4,3,3,3,3,3,3,3,3,3,3,3,3,3,3,3,4),(0.,0.109997882182062,
0.125,0.232971489029442,0.25,0.358370808476237,0.375,0.48335043398321,0.5,
0.608350433983159,0.625,0.733370808476259,0.75,0.857971489029473,0.875,
0.984997882181992,1.),.UNSPECIFIED.);
#287=B_SPLINE_CURVE_WITH_KNOTS('',3,(#27002,#27003,#27004,#27005,#27006,
#27007,#27008,#27009,#27010,#27011,#27012,#27013,#27014,#27015,#27016,#27017,
#27018,#27019,#27020,#27021,#27022,#27023,#27024,#27025,#27026,#27027,#27028,
#27029,#27030,#27031,#27032,#27033,#27034,#27035,#27036,#27037,#27038,#27039,
#27040,#27041,#27042,#27043,#27044,#27045,#27046,#27047,#27048,#27049,#27050),
 .UNSPECIFIED.,.F.,.F.,(4,3,3,3,3,3,3,3,3,3,3,3,3,3,3,3,4),(0.,0.110006491219228,
0.125,0.232980230285482,0.25,0.358379546919392,0.375,0.483359156973627,
0.5,0.608359156973173,0.625,0.733379546920954,0.75,0.857980230285446,0.875,
0.985006491219265,1.),.UNSPECIFIED.);
#288=B_SPLINE_CURVE_WITH_KNOTS('',3,(#27055,#27056,#27057,#27058,#27059,
#27060,#27061,#27062,#27063,#27064,#27065,#27066,#27067,#27068,#27069,#27070,
#27071,#27072,#27073,#27074,#27075,#27076,#27077,#27078,#27079,#27080,#27081,
#27082,#27083,#27084,#27085,#27086,#27087,#27088,#27089,#27090,#27091,#27092,
#27093,#27094,#27095,#27096,#27097,#27098,#27099,#27100,#27101,#27102,#27103,
#27104,#27105,#27106,#27107,#27108,#27109,#27110,#27111,#27112,#27113,#27114,
#27115),.UNSPECIFIED.,.F.,.F.,(4,3,3,3,3,3,3,3,3,3,3,3,3,3,3,3,3,3,3,3,
4),(0.,0.109229796985621,0.125,0.233476713981996,0.25,0.3125,0.375,0.4375,
0.46875,0.484375,0.5,0.515625,0.53125,0.5625,0.625,0.6875,0.75,0.833497889959173,
0.875,0.9375,1.),.UNSPECIFIED.);
#289=B_SPLINE_CURVE_WITH_KNOTS('',3,(#27116,#27117,#27118,#27119,#27120,
#27121,#27122,#27123,#27124,#27125,#27126,#27127,#27128,#27129,#27130,#27131,
#27132,#27133,#27134,#27135,#27136,#27137,#27138,#27139,#27140,#27141,#27142,
#27143,#27144,#27145,#27146,#27147,#27148,#27149,#27150,#27151,#27152,#27153,
#27154,#27155,#27156,#27157,#27158,#27159,#27160,#27161,#27162,#27163,#27164),
 .UNSPECIFIED.,.F.,.F.,(4,3,3,3,3,3,3,3,3,3,3,3,3,3,3,3,4),(0.,0.109993207336737,
0.125,0.232966742381088,0.25,0.35836606335207,0.375,0.48334569725311,0.5,
0.608345697254482,0.625,0.733366063352394,0.75,0.8579667423811,0.875,0.984993207336734,
1.),.UNSPECIFIED.);
#290=B_SPLINE_CURVE_WITH_KNOTS('',3,(#27169,#27170,#27171,#27172,#27173,
#27174,#27175,#27176,#27177,#27178,#27179,#27180,#27181,#27182,#27183,#27184,
#27185,#27186,#27187,#27188,#27189,#27190,#27191,#27192,#27193,#27194,#27195,
#27196,#27197,#27198,#27199,#27200,#27201,#27202,#27203,#27204,#27205,#27206,
#27207,#27208,#27209,#27210,#27211,#27212,#27213,#27214,#27215,#27216,#27217),
 .UNSPECIFIED.,.F.,.F.,(4,3,3,3,3,3,3,3,3,3,3,3,3,3,3,3,4),(0.,0.109987471059102,
0.125,0.232960917994534,0.25,0.358360240830988,0.375,0.483339885033845,
0.5,0.608339885033874,0.625,0.733360240831014,0.75,0.857960917994191,0.875,
0.984987471059085,1.),.UNSPECIFIED.);
#291=B_SPLINE_CURVE_WITH_KNOTS('',3,(#27218,#27219,#27220,#27221,#27222,
#27223,#27224,#27225,#27226,#27227,#27228,#27229,#27230,#27231,#27232,#27233,
#27234,#27235,#27236,#27237,#27238,#27239,#27240,#27241,#27242,#27243,#27244,
#27245,#27246,#27247,#27248,#27249,#27250,#27251,#27252,#27253,#27254,#27255,
#27256,#27257,#27258,#27259,#27260,#27261,#27262,#27263),.UNSPECIFIED.,
 .F.,.F.,(4,3,3,3,3,3,3,3,3,3,3,3,3,3,3,4),(0.,0.109411056806016,0.125,
0.233524594880298,0.25,0.361851047408981,0.375,0.467122237965085,0.5,0.625,
0.729792305576865,0.75,0.85487283082487,0.875,0.978749428137399,1.),
 .UNSPECIFIED.);
#292=B_SPLINE_CURVE_WITH_KNOTS('',3,(#27268,#27269,#27270,#27271,#27272,
#27273,#27274,#27275,#27276,#27277,#27278,#27279,#27280,#27281,#27282,#27283,
#27284,#27285,#27286,#27287,#27288,#27289,#27290,#27291,#27292,#27293,#27294,
#27295,#27296,#27297,#27298,#27299,#27300,#27301,#27302,#27303,#27304,#27305,
#27306,#27307,#27308,#27309,#27310,#27311,#27312,#27313,#27314,#27315,#27316),
 .UNSPECIFIED.,.F.,.F.,(4,3,3,3,3,3,3,3,3,3,3,3,3,3,3,3,4),(0.,0.110008212483426,
0.125,0.232981977989281,0.25,0.358381294058765,0.375,0.48336090102248,0.5,
0.608360901022441,0.625,0.733381294058795,0.75,0.857981977986097,0.875,
0.985008212482492,1.),.UNSPECIFIED.);
#293=B_SPLINE_CURVE_WITH_KNOTS('',3,(#27317,#27318,#27319,#27320,#27321,
#27322,#27323,#27324,#27325,#27326,#27327,#27328,#27329,#27330,#27331,#27332,
#27333,#27334,#27335,#27336,#27337,#27338,#27339,#27340,#27341,#27342,#27343,
#27344,#27345,#27346,#27347,#27348,#27349,#27350,#27351,#27352,#27353,#27354,
#27355,#27356,#27357,#27358,#27359,#27360,#27361,#27362,#27363,#27364,#27365),
 .UNSPECIFIED.,.F.,.F.,(4,3,3,3,3,3,3,3,3,3,3,3,3,3,3,3,4),(0.,0.109994646065219,
0.125,0.232968203208124,0.25,0.35836752370985,0.375,0.483347155027715,0.5,
0.608347155027694,0.625,0.733367523710364,0.75,0.857968203208095,0.875,
0.984994646065316,1.),.UNSPECIFIED.);
#294=B_SPLINE_CURVE_WITH_KNOTS('',3,(#27370,#27371,#27372,#27373,#27374,
#27375,#27376,#27377,#27378,#27379,#27380,#27381,#27382,#27383,#27384,#27385,
#27386,#27387,#27388,#27389,#27390,#27391,#27392,#27393,#27394,#27395,#27396,
#27397,#27398,#27399,#27400,#27401,#27402,#27403,#27404,#27405,#27406,#27407,
#27408,#27409,#27410,#27411,#27412,#27413,#27414,#27415,#27416,#27417,#27418),
 .UNSPECIFIED.,.F.,.F.,(4,3,3,3,3,3,3,3,3,3,3,3,3,3,3,3,4),(0.,0.109989675774911,
0.125,0.232963156575604,0.25,0.358362478695303,0.375,0.483342118938395,
0.5,0.608342118938392,0.625,0.733362478695318,0.75,0.857963156572259,0.875,
0.984989675774944,1.),.UNSPECIFIED.);
#295=B_SPLINE_CURVE_WITH_KNOTS('',3,(#27419,#27420,#27421,#27422,#27423,
#27424,#27425,#27426,#27427,#27428,#27429,#27430,#27431,#27432,#27433,#27434,
#27435,#27436,#27437,#27438,#27439,#27440,#27441,#27442,#27443,#27444,#27445,
#27446,#27447,#27448,#27449,#27450,#27451,#27452,#27453,#27454,#27455,#27456,
#27457,#27458,#27459,#27460,#27461,#27462,#27463,#27464,#27465,#27466,#27467),
 .UNSPECIFIED.,.F.,.F.,(4,3,3,3,3,3,3,3,3,3,3,3,3,3,3,3,4),(0.,0.110004858025113,
0.125,0.232978572010577,0.25,0.358377889178609,0.375,0.483357502162731,
0.5,0.608357502162803,0.625,0.73337788917867,0.75,0.857978572010549,0.875,
0.985004858024923,1.),.UNSPECIFIED.);
#296=B_SPLINE_CURVE_WITH_KNOTS('',3,(#27473,#27474,#27475,#27476,#27477,
#27478,#27479,#27480,#27481,#27482,#27483,#27484,#27485,#27486,#27487,#27488,
#27489,#27490,#27491,#27492,#27493,#27494,#27495,#27496,#27497),
 .UNSPECIFIED.,.F.,.F.,(4,3,3,3,3,3,3,3,4),(0.,0.125,0.25,0.375,0.5,0.625,
0.75,0.875,1.),.UNSPECIFIED.);
#297=B_SPLINE_CURVE_WITH_KNOTS('',3,(#27500,#27501,#27502,#27503,#27504,
#27505,#27506,#27507,#27508,#27509,#27510,#27511,#27512,#27513,#27514,#27515,
#27516,#27517,#27518,#27519,#27520,#27521,#27522,#27523,#27524,#27525,#27526,
#27527,#27528,#27529,#27530,#27531,#27532,#27533,#27534,#27535,#27536,#27537,
#27538,#27539,#27540,#27541,#27542,#27543,#27544,#27545,#27546,#27547,#27548),
 .UNSPECIFIED.,.F.,.F.,(4,3,3,3,3,3,3,3,3,3,3,3,3,3,3,3,4),(1.05676601839088E-5,
0.110007241592374,0.125,0.232970353736968,0.25,0.358369673547411,0.375,
0.483349301063305,0.5,0.60834930106321,0.625,0.733369673548882,0.75,0.857970353739919,
0.875,0.98499676406314,1.),.UNSPECIFIED.);
#298=B_SPLINE_CURVE_WITH_KNOTS('',3,(#27550,#27551,#27552,#27553,#27554,
#27555,#27556,#27557,#27558,#27559,#27560,#27561,#27562,#27563,#27564,#27565,
#27566,#27567,#27568,#27569,#27570,#27571,#27572,#27573,#27574,#27575,#27576,
#27577,#27578,#27579,#27580,#27581,#27582,#27583),.UNSPECIFIED.,.F.,.F.,
(4,2,2,2,2,2,2,2,2,2,2,2,2,2,2,2,4),(0.,0.1099839788089,0.125,0.232958793615559,
0.25,0.358357719328499,0.375,0.483320936683858,0.5,0.608394468603398,0.625,
0.733299780434519,0.75,0.857953179030985,0.875,0.984975935865878,1.),
 .UNSPECIFIED.);
#299=B_SPLINE_CURVE_WITH_KNOTS('',3,(#27584,#27585,#27586,#27587,#27588,
#27589,#27590,#27591,#27592,#27593,#27594,#27595,#27596,#27597,#27598,#27599,
#27600,#27601,#27602,#27603,#27604,#27605,#27606,#27607,#27608,#27609,#27610,
#27611,#27612,#27613,#27614,#27615,#27616,#27617,#27618,#27619,#27620,#27621,
#27622,#27623,#27624,#27625,#27626,#27627,#27628,#27629,#27630,#27631,#27632),
 .UNSPECIFIED.,.F.,.F.,(4,3,3,3,3,3,3,3,3,3,3,3,3,3,3,3,4),(0.,0.109981115336569,
0.125,0.232954464634818,0.25,0.358353789540815,0.375,0.483333445161142,
0.5,0.608333445161148,0.625,0.733353789541188,0.75,0.857954464634781,0.875,
0.984981115336604,1.),.UNSPECIFIED.);
#300=B_SPLINE_CURVE_WITH_KNOTS('',3,(#27634,#27635,#27636,#27637,#27638,
#27639,#27640,#27641,#27642,#27643,#27644,#27645,#27646,#27647,#27648,#27649,
#27650,#27651,#27652,#27653,#27654,#27655,#27656,#27657,#27658,#27659,#27660,
#27661,#27662,#27663,#27664,#27665,#27666,#27667,#27668,#27669,#27670,#27671,
#27672,#27673,#27674,#27675,#27676,#27677,#27678,#27679,#27680,#27681,#27682,
#27683,#27684,#27685,#27686,#27687,#27688,#27689,#27690,#27691,#27692,#27693,
#27694,#27695,#27696,#27697,#27698,#27699,#27700,#27701,#27702,#27703,#27704,
#27705,#27706,#27707,#27708,#27709,#27710,#27711,#27712,#27713,#27714,#27715,
#27716,#27717,#27718,#27719,#27720,#27721,#27722,#27723,#27724,#27725,#27726,
#27727,#27728,#27729,#27730,#27731,#27732,#27733,#27734,#27735,#27736,#27737,
#27738,#27739,#27740,#27741,#27742,#27743,#27744,#27745,#27746,#27747,#27748,
#27749,#27750,#27751,#27752,#27753,#27754,#27755,#27756,#27757,#27758,#27759,
#27760,#27761,#27762,#27763,#27764,#27765,#27766,#27767,#27768,#27769,#27770,
#27771,#27772,#27773,#27774,#27775,#27776,#27777,#27778,#27779,#27780,#27781,
#27782,#27783,#27784,#27785,#27786,#27787,#27788,#27789,#27790,#27791,#27792,
#27793,#27794,#27795,#27796,#27797,#27798,#27799,#27800,#27801,#27802,#27803,
#27804,#27805),.UNSPECIFIED.,.F.,.F.,(4,2,2,2,2,2,2,2,2,2,2,2,2,2,2,2,2,
2,2,2,2,2,2,2,2,2,2,2,2,2,2,2,2,2,2,2,2,2,2,2,2,2,2,2,2,2,2,2,2,2,2,2,2,
2,2,2,2,2,2,2,2,2,2,2,2,2,2,2,2,2,2,2,2,2,2,2,2,2,2,2,2,2,2,2,2,4),(-3.18698728124793,
-3.18221150041198,-3.17770115961186,-3.17351534682041,-3.16794534503497,
-3.15510289974664,-3.14041186020985,-3.12656711296006,-3.12093142351134,
-3.11650988030342,-3.11386727450745,-3.11118717587842,-3.10657791508633,
-3.08620123136938,-3.06968503536365,-3.06202460328115,-3.05550292678536,
-3.05101124207204,-3.04692417253542,-3.04012330120204,-3.014050467194,-3.00106332653079,
-2.99562143285543,-2.99131261770304,-2.98869354071747,-2.98598864056323,
-2.98125503114169,-2.95697590185544,-2.9376706591066,-2.93079521268944,
-2.92624246073123,-2.92168170266288,-2.91476142321413,-2.89012631427218,
-2.87634138783952,-2.87071936786336,-2.86630615065774,-2.86366633762864,
-2.86098581479334,-2.8563731997087,-2.84113361751968,-2.82481174903563,
-2.81000401317442,-2.80424557943887,-2.79986443220269,-2.79494715004204,
-2.78633314665999,-2.75567772970282,-2.74774096640098,-2.74209068126568,
-2.7392071999634,-2.73668320320541,-2.73290562150034,-2.72063041979193,
-2.69068302951113,-2.68209322477362,-2.67722480156804,-2.67283260709197,
-2.6670800611951,-2.65287898102453,-2.62264197141188,-2.6169720173207,-2.61408498279469,
-2.61156230645776,-2.60779316367471,-2.59562470690211,-2.57223410085811,
-2.56324261321821,-2.5559217426326,-2.55128725491093,-2.54684510531043,
-2.54035402504735,-2.51174648636987,-2.4999883969495,-2.49266513269346,
-2.48949927524476,-2.48702287507504,-2.48375590382051,-2.47631287383972,
-2.44835612981682,-2.43877060704842,-2.43110978873152,-2.42641227829457,
-2.42200605065057,-2.41574067915496,-2.3902143501497),.UNSPECIFIED.);
#301=B_SPLINE_CURVE_WITH_KNOTS('',3,(#27806,#27807,#27808,#27809,#27810,
#27811,#27812,#27813,#27814,#27815,#27816,#27817,#27818,#27819,#27820,#27821,
#27822,#27823,#27824,#27825,#27826,#27827,#27828,#27829,#27830,#27831,#27832,
#27833,#27834,#27835,#27836,#27837,#27838,#27839,#27840,#27841,#27842,#27843,
#27844,#27845,#27846,#27847,#27848,#27849,#27850,#27851,#27852,#27853,#27854),
 .UNSPECIFIED.,.F.,.F.,(4,3,3,3,3,3,3,3,3,3,3,3,3,3,3,3,4),(0.,0.109984428745348,
0.125,0.232957828943971,0.25,0.358357152774683,0.375,0.483336802439457,
0.5,0.608336802440611,0.625,0.733357152772898,0.75,0.857957828943944,0.875,
0.984984428745393,1.),.UNSPECIFIED.);
#302=B_SPLINE_CURVE_WITH_KNOTS('',2,(#27983,#27984,#27985),
 .UNSPECIFIED.,.F.,.F.,(3,3),(0.,0.115758369027897),.UNSPECIFIED.);
#303=B_SPLINE_CURVE_WITH_KNOTS('',3,(#27997,#27998,#27999,#28000),
 .UNSPECIFIED.,.F.,.F.,(4,4),(0.,1.),.UNSPECIFIED.);
#304=B_SPLINE_CURVE_WITH_KNOTS('',3,(#28021,#28022,#28023,#28024,#28025,
#28026,#28027,#28028,#28029,#28030,#28031,#28032,#28033,#28034,#28035,#28036,
#28037,#28038,#28039,#28040,#28041,#28042,#28043,#28044,#28045),
 .UNSPECIFIED.,.F.,.F.,(4,3,3,3,3,3,3,3,4),(-0.226770318913044,-0.176070092740286,
-0.141340884398364,-0.125369866567527,-0.0941292001496635,-0.0702859439456138,
-0.0114755323037468,-0.00261123297662246,0.),.UNSPECIFIED.);
#305=B_SPLINE_CURVE_WITH_KNOTS('',3,(#28046,#28047,#28048,#28049,#28050,
#28051,#28052,#28053,#28054,#28055,#28056,#28057,#28058,#28059,#28060,#28061,
#28062,#28063,#28064,#28065,#28066,#28067,#28068,#28069,#28070,#28071,#28072,
#28073),.UNSPECIFIED.,.F.,.F.,(4,3,3,3,3,3,3,3,3,4),(-0.528419249915466,
-0.3824987601112,-0.313797789423033,-0.236578270306934,-0.180178655007884,
-0.091691640876666,-0.0576929606469953,-0.03032436788477,-0.00320462674544752,
-0.0001765620571701),.UNSPECIFIED.);
#306=B_SPLINE_CURVE_WITH_KNOTS('',3,(#28079,#28080,#28081,#28082),
 .UNSPECIFIED.,.F.,.F.,(4,4),(0.,1.),.UNSPECIFIED.);
#307=B_SPLINE_CURVE_WITH_KNOTS('',3,(#28104,#28105,#28106,#28107,#28108,
#28109,#28110,#28111,#28112,#28113,#28114,#28115,#28116,#28117,#28118,#28119,
#28120,#28121,#28122,#28123,#28124,#28125,#28126,#28127,#28128,#28129,#28130,
#28131,#28132,#28133,#28134,#28135,#28136,#28137,#28138,#28139,#28140,#28141,
#28142,#28143,#28144,#28145,#28146,#28147,#28148,#28149,#28150,#28151,#28152),
 .UNSPECIFIED.,.F.,.F.,(4,3,3,3,3,3,3,3,3,3,3,3,3,3,3,3,4),(0.,0.0927497600106301,
0.125,0.216040635762613,0.25,0.34137739623301,0.375,0.466360239331372,0.5,
0.591360239331263,0.625,0.716377396232998,0.75,0.841040635762724,0.875,
0.967749760010667,1.),.UNSPECIFIED.);
#308=B_SPLINE_CURVE_WITH_KNOTS('',3,(#28154,#28155,#28156,#28157,#28158,
#28159,#28160,#28161,#28162,#28163,#28164,#28165,#28166,#28167,#28168,#28169,
#28170,#28171,#28172,#28173,#28174,#28175,#28176,#28177,#28178,#28179,#28180,
#28181,#28182,#28183,#28184,#28185,#28186,#28187,#28188,#28189,#28190,#28191,
#28192,#28193,#28194,#28195,#28196,#28197,#28198,#28199,#28200,#28201,#28202),
 .UNSPECIFIED.,.F.,.F.,(4,3,3,3,3,3,3,3,3,3,3,3,3,3,3,3,4),(0.,0.0927530928142782,
0.125,0.216044019764289,0.25,0.341380779151096,0.375,0.466363616262366,
0.5,0.591363616262178,0.625,0.716380779151037,0.75,0.841044019764313,0.875,
0.967753092814524,1.),.UNSPECIFIED.);
#309=B_SPLINE_CURVE_WITH_KNOTS('',3,(#28204,#28205,#28206,#28207,#28208,
#28209,#28210,#28211,#28212,#28213,#28214,#28215,#28216,#28217,#28218,#28219,
#28220,#28221,#28222,#28223,#28224,#28225,#28226,#28227,#28228,#28229,#28230,
#28231,#28232,#28233,#28234,#28235,#28236,#28237,#28238,#28239,#28240,#28241,
#28242,#28243,#28244,#28245,#28246,#28247,#28248,#28249,#28250,#28251,#28252),
 .UNSPECIFIED.,.F.,.F.,(4,3,3,3,3,3,3,3,3,3,3,3,3,3,3,3,4),(0.,0.0927719347706172,
0.125,0.216063151119803,0.25,0.341399904362238,0.375,0.466382707642218,
0.5,0.591382707642052,0.625,0.716399904361949,0.75,0.841063151120002,0.875,
0.967771934770454,1.),.UNSPECIFIED.);
#310=B_SPLINE_CURVE_WITH_KNOTS('',3,(#28254,#28255,#28256,#28257,#28258,
#28259,#28260,#28261,#28262,#28263,#28264,#28265,#28266,#28267,#28268,#28269,
#28270,#28271,#28272,#28273,#28274,#28275,#28276,#28277,#28278,#28279,#28280,
#28281,#28282,#28283,#28284,#28285,#28286,#28287,#28288,#28289,#28290,#28291,
#28292,#28293,#28294,#28295,#28296,#28297,#28298,#28299,#28300,#28301,#28302,
#28303,#28304,#28305,#28306,#28307,#28308,#28309,#28310,#28311,#28312,#28313,
#28314,#28315,#28316,#28317,#28318,#28319,#28320,#28321,#28322,#28323,#28324,
#28325,#28326,#28327,#28328,#28329,#28330,#28331,#28332,#28333,#28334,#28335,
#28336,#28337,#28338,#28339,#28340,#28341,#28342,#28343,#28344,#28345,#28346,
#28347,#28348,#28349,#28350,#28351,#28352,#28353,#28354,#28355,#28356,#28357,
#28358,#28359,#28360,#28361,#28362,#28363,#28364,#28365,#28366,#28367,#28368,
#28369,#28370,#28371,#28372,#28373,#28374,#28375,#28376,#28377),
 .UNSPECIFIED.,.F.,.F.,(4,3,3,3,3,3,3,3,3,3,3,3,3,3,3,3,3,3,3,3,3,3,3,3,
3,3,3,3,3,3,3,3,3,3,3,3,3,3,3,3,3,4),(0.,0.0468270325633607,0.0625,0.064586021838547,
0.11912898254499,0.125,0.168623487537581,0.1875,0.25,0.3125,0.323789195493357,
0.375,0.4375,0.46875,0.484375,0.4921875,0.5,0.515625,0.53125,0.5625,0.625,
0.636035971190133,0.65625,0.6875,0.703125,0.71875,0.734375,0.741588067961916,
0.746426043014038,0.748801135923832,0.75216626473836,0.756085815752169,
0.764372920225663,0.78125,0.796875,0.8125,0.84375,0.875,0.92634083787367,
0.9375,0.995557989972811,1.),.UNSPECIFIED.);
#311=B_SPLINE_CURVE_WITH_KNOTS('',3,(#28379,#28380,#28381,#28382,#28383,
#28384,#28385,#28386,#28387,#28388,#28389,#28390,#28391,#28392,#28393,#28394,
#28395,#28396,#28397,#28398,#28399,#28400,#28401,#28402,#28403,#28404,#28405,
#28406,#28407,#28408,#28409,#28410,#28411,#28412,#28413,#28414,#28415,#28416,
#28417,#28418,#28419,#28420,#28421,#28422,#28423,#28424,#28425,#28426,#28427),
 .UNSPECIFIED.,.F.,.F.,(4,3,3,3,3,3,3,3,3,3,3,3,3,3,3,3,4),(0.,0.0927574051465889,
0.125,0.21604839833824,0.25,0.341385156321511,0.375,0.46636798568725,0.5,
0.591367985687259,0.625,0.716385156321534,0.75,0.841048398338404,0.875,
0.967757405146268,1.),.UNSPECIFIED.);
#312=B_SPLINE_CURVE_WITH_KNOTS('',3,(#28429,#28430,#28431,#28432,#28433,
#28434,#28435,#28436,#28437,#28438,#28439,#28440,#28441,#28442,#28443,#28444,
#28445,#28446,#28447,#28448,#28449,#28450,#28451,#28452,#28453,#28454,#28455,
#28456,#28457,#28458,#28459,#28460,#28461,#28462,#28463,#28464,#28465,#28466,
#28467,#28468,#28469,#28470,#28471,#28472,#28473,#28474,#28475,#28476,#28477),
 .UNSPECIFIED.,.F.,.F.,(4,3,3,3,3,3,3,3,3,3,3,3,3,3,3,3,4),(0.,0.0927663738152036,
0.125,0.21605750476053,0.25,0.341394259819506,0.375,0.466377073081152,0.5,
0.591377073081215,0.625,0.716394259819437,0.75,0.841057504760613,0.875,
0.967766373815486,1.),.UNSPECIFIED.);
#313=B_SPLINE_CURVE_WITH_KNOTS('',3,(#28479,#28480,#28481,#28482,#28483,
#28484,#28485,#28486,#28487,#28488,#28489,#28490,#28491,#28492,#28493,#28494,
#28495,#28496,#28497,#28498,#28499,#28500,#28501,#28502,#28503,#28504,#28505,
#28506,#28507,#28508,#28509,#28510,#28511,#28512),.UNSPECIFIED.,.F.,.F.,
(4,2,2,2,2,2,2,2,2,2,2,2,2,2,2,2,4),(0.,0.0927498161032601,0.125,0.216043543384793,
0.25,0.3413826281949,0.375,0.466317384484732,0.5,0.591468261682124,0.625,
0.716305724457278,0.75,0.841042047534153,0.875,0.967746874834895,1.),
 .UNSPECIFIED.);
#314=B_SPLINE_CURVE_WITH_KNOTS('',3,(#28514,#28515,#28516,#28517,#28518,
#28519,#28520,#28521,#28522,#28523,#28524,#28525,#28526,#28527,#28528,#28529,
#28530,#28531,#28532,#28533,#28534,#28535,#28536,#28537,#28538,#28539,#28540,
#28541,#28542,#28543,#28544,#28545,#28546,#28547,#28548,#28549,#28550,#28551,
#28552,#28553,#28554,#28555,#28556,#28557,#28558,#28559,#28560,#28561,#28562),
 .UNSPECIFIED.,.F.,.F.,(4,3,3,3,3,3,3,3,3,3,3,3,3,3,3,3,4),(0.,0.0927616901918672,
0.125,0.216052749201994,0.25,0.341389505789046,0.375,0.466372327459579,
0.5,0.591372327459986,0.625,0.716389505788987,0.75,0.841052749202119,0.875,
0.967761690191907,1.),.UNSPECIFIED.);
#315=B_SPLINE_CURVE_WITH_KNOTS('',3,(#28564,#28565,#28566,#28567,#28568,
#28569,#28570,#28571,#28572,#28573,#28574,#28575,#28576,#28577,#28578,#28579,
#28580,#28581,#28582,#28583,#28584,#28585,#28586,#28587,#28588,#28589,#28590,
#28591,#28592,#28593,#28594,#28595,#28596,#28597,#28598,#28599,#28600,#28601,
#28602,#28603,#28604,#28605,#28606,#28607,#28608,#28609,#28610,#28611,#28612),
 .UNSPECIFIED.,.F.,.F.,(4,3,3,3,3,3,3,3,3,3,3,3,3,3,3,3,4),(0.,0.0927693846977541,
0.125,0.216060561884735,0.25,0.341397315960308,0.375,0.466380123817375,
0.5,0.591380123817283,0.625,0.716397315960319,0.75,0.841060561884845,0.875,
0.967769384698343,1.),.UNSPECIFIED.);
#316=B_SPLINE_CURVE_WITH_KNOTS('',3,(#28614,#28615,#28616,#28617,#28618,
#28619,#28620,#28621,#28622,#28623,#28624,#28625,#28626,#28627,#28628,#28629,
#28630,#28631,#28632,#28633,#28634,#28635,#28636,#28637,#28638,#28639,#28640,
#28641,#28642,#28643,#28644,#28645,#28646,#28647,#28648,#28649,#28650),
 .UNSPECIFIED.,.F.,.F.,(4,3,3,3,3,3,3,3,3,3,3,3,4),(-0.157708230401766,
-0.138862257038452,-0.126648343324981,-0.119614872623337,-0.113538993032145,
-0.106944773722366,-0.0982823459339201,-0.0786512255255752,-0.0450114713913922,
-0.0124390832211188,-0.00494329693926847,-0.00231862606359825,0.),
 .UNSPECIFIED.);
#317=B_SPLINE_CURVE_WITH_KNOTS('',3,(#28654,#28655,#28656,#28657,#28658,
#28659,#28660,#28661,#28662,#28663,#28664,#28665,#28666),.UNSPECIFIED.,
 .F.,.F.,(4,3,3,3,4),(4.17257076022422E-7,0.41302767210967,0.5,0.913027257516351,
1.),.UNSPECIFIED.);
#318=B_SPLINE_CURVE_WITH_KNOTS('',3,(#28668,#28669,#28670,#28671,#28672,
#28673,#28674,#28675,#28676,#28677,#28678,#28679,#28680,#28681,#28682,#28683,
#28684,#28685,#28686,#28687,#28688,#28689,#28690,#28691,#28692,#28693,#28694,
#28695,#28696,#28697,#28698,#28699,#28700,#28701,#28702,#28703,#28704,#28705,
#28706,#28707,#28708,#28709,#28710,#28711,#28712,#28713,#28714,#28715,#28716),
 .UNSPECIFIED.,.F.,.F.,(4,3,3,3,3,3,3,3,3,3,3,3,3,3,3,3,4),(0.,0.0927564231352309,
0.125,0.216045703373452,0.25,0.341377418388321,0.375,0.466406748023344,
0.5,0.591313174398933,0.625,0.71637725021057,0.75,0.841035152620575,0.875,
0.967742717294513,1.),.UNSPECIFIED.);
#319=B_SPLINE_CURVE_WITH_KNOTS('',3,(#28718,#28719,#28720,#28721,#28722,
#28723,#28724,#28725,#28726,#28727,#28728,#28729,#28730,#28731,#28732,#28733,
#28734,#28735,#28736,#28737,#28738,#28739,#28740,#28741,#28742,#28743,#28744,
#28745,#28746,#28747,#28748,#28749,#28750,#28751,#28752,#28753,#28754,#28755,
#28756,#28757,#28758,#28759,#28760,#28761,#28762,#28763,#28764,#28765,#28766),
 .UNSPECIFIED.,.F.,.F.,(4,3,3,3,3,3,3,3,3,3,3,3,3,3,3,3,4),(0.,0.0927584978174006,
0.125,0.21604950779295,0.25,0.341386265420333,0.375,0.466369092823765,0.5,
0.591369092823743,0.625,0.716386265420279,0.75,0.841049507793065,0.875,
0.967758497817597,1.),.UNSPECIFIED.);
#320=B_SPLINE_CURVE_WITH_KNOTS('',3,(#28768,#28769,#28770,#28771,#28772,
#28773,#28774,#28775,#28776,#28777,#28778,#28779,#28780,#28781,#28782,#28783,
#28784,#28785,#28786,#28787,#28788,#28789,#28790,#28791,#28792,#28793,#28794,
#28795,#28796,#28797,#28798,#28799,#28800,#28801,#28802,#28803,#28804,#28805,
#28806,#28807,#28808,#28809,#28810,#28811,#28812,#28813,#28814,#28815,#28816),
 .UNSPECIFIED.,.F.,.F.,(4,3,3,3,3,3,3,3,3,3,3,3,3,3,3,3,4),(0.,0.0927642788375456,
0.125,0.21605537760672,0.25,0.341392133349299,0.375,0.466374950372504,0.5,
0.59137495037261,0.625,0.716392133349448,0.75,0.841055377606904,0.875,0.967764278837053,
1.),.UNSPECIFIED.);
#321=B_SPLINE_CURVE_WITH_KNOTS('',3,(#28818,#28819,#28820,#28821,#28822,
#28823,#28824,#28825,#28826,#28827,#28828,#28829,#28830,#28831,#28832,#28833,
#28834,#28835,#28836,#28837,#28838,#28839,#28840,#28841,#28842,#28843,#28844,
#28845,#28846,#28847,#28848,#28849,#28850,#28851,#28852,#28853,#28854,#28855,
#28856,#28857,#28858,#28859,#28860,#28861,#28862,#28863,#28864,#28865,#28866),
 .UNSPECIFIED.,.F.,.F.,(4,3,3,3,3,3,3,3,3,3,3,3,3,3,3,3,4),(0.,0.0928180932521736,
0.125,0.215969156459661,0.25,0.341016499097481,0.375,0.469480461922614,
0.5,0.58699659830702,0.625,0.7167307792291,0.75,0.841380676583067,0.875,
0.968438688021389,1.),.UNSPECIFIED.);
#322=B_SPLINE_CURVE_WITH_KNOTS('',3,(#28868,#28869,#28870,#28871,#28872,
#28873,#28874,#28875,#28876,#28877,#28878,#28879,#28880,#28881,#28882,#28883,
#28884,#28885,#28886,#28887,#28888,#28889,#28890,#28891,#28892,#28893,#28894,
#28895,#28896,#28897,#28898,#28899,#28900,#28901,#28902,#28903,#28904,#28905,
#28906,#28907,#28908,#28909,#28910,#28911,#28912,#28913,#28914,#28915,#28916),
 .UNSPECIFIED.,.F.,.F.,(4,3,3,3,3,3,3,3,3,3,3,3,3,3,3,3,4),(0.,0.0927640659933894,
0.125,0.216055161493703,0.25,0.341391917305785,0.375,0.466374734710861,
0.5,0.591374734710935,0.625,0.716391917305873,0.75,0.841055161493749,0.875,
0.967764065993903,1.),.UNSPECIFIED.);
#323=B_SPLINE_CURVE_WITH_KNOTS('',3,(#28918,#28919,#28920,#28921,#28922,
#28923,#28924,#28925,#28926,#28927,#28928,#28929,#28930,#28931,#28932,#28933,
#28934,#28935,#28936,#28937,#28938,#28939,#28940,#28941,#28942,#28943,#28944,
#28945,#28946,#28947,#28948,#28949,#28950,#28951,#28952,#28953,#28954,#28955,
#28956,#28957,#28958,#28959,#28960,#28961,#28962,#28963,#28964,#28965,#28966),
 .UNSPECIFIED.,.F.,.F.,(4,3,3,3,3,3,3,3,3,3,3,3,3,3,3,3,4),(0.,0.0927585881876831,
0.125,0.216049599551051,0.25,0.341386357148991,0.375,0.466369184390078,
0.5,0.591369184389981,0.625,0.716386357148919,0.75,0.841049599551146,0.875,
0.967758588187543,1.),.UNSPECIFIED.);
#324=B_SPLINE_CURVE_WITH_KNOTS('',3,(#28968,#28969,#28970,#28971,#28972,
#28973,#28974,#28975,#28976,#28977,#28978,#28979,#28980,#28981,#28982,#28983,
#28984,#28985,#28986,#28987,#28988,#28989,#28990,#28991,#28992,#28993,#28994,
#28995,#28996,#28997,#28998,#28999,#29000,#29001,#29002,#29003,#29004,#29005,
#29006,#29007,#29008,#29009,#29010,#29011,#29012,#29013,#29014,#29015,#29016,
#29017,#29018,#29019,#29020,#29021,#29022,#29023,#29024,#29025,#29026,#29027,
#29028,#29029,#29030,#29031,#29032,#29033,#29034,#29035,#29036,#29037,#29038,
#29039,#29040,#29041,#29042,#29043,#29044,#29045,#29046,#29047,#29048,#29049,
#29050,#29051,#29052,#29053,#29054,#29055,#29056,#29057,#29058,#29059,#29060,
#29061,#29062,#29063,#29064,#29065,#29066,#29067),.UNSPECIFIED.,.F.,.F.,
(4,3,3,3,3,3,3,3,3,3,3,3,3,3,3,3,3,3,3,3,3,3,3,3,3,3,3,3,3,3,3,3,3,4),(0.,
0.0939730383414856,0.0972745498842664,0.125,0.1875,0.25,0.254701161761956,
0.3125,0.375,0.40625,0.412096773522505,0.4375,0.46875,0.484375,0.4921875,
0.5,0.50390625,0.5078125,0.515625,0.53125,0.5625,0.59375,0.625,0.648660762160911,
0.6875,0.75,0.8125,0.815195003357837,0.875,0.929951775124377,0.932307451240959,
0.9375,0.989835529327015,1.),.UNSPECIFIED.);
#325=B_SPLINE_CURVE_WITH_KNOTS('',3,(#29069,#29070,#29071,#29072,#29073,
#29074,#29075,#29076,#29077,#29078,#29079,#29080,#29081,#29082,#29083,#29084,
#29085,#29086,#29087,#29088,#29089,#29090,#29091,#29092,#29093,#29094,#29095,
#29096,#29097,#29098,#29099,#29100,#29101,#29102,#29103,#29104,#29105,#29106,
#29107,#29108,#29109,#29110,#29111,#29112,#29113,#29114,#29115,#29116,#29117),
 .UNSPECIFIED.,.F.,.F.,(4,3,3,3,3,3,3,3,3,3,3,3,3,3,3,3,4),(0.,0.0927704812620034,
0.125,0.216061675289301,0.25,0.341398429006514,0.375,0.466381234895823,
0.5,0.591381234895582,0.625,0.716398429006577,0.75,0.841061675289124,0.875,
0.967770481262084,1.),.UNSPECIFIED.);
#326=B_SPLINE_CURVE_WITH_KNOTS('',3,(#29119,#29120,#29121,#29122,#29123,
#29124,#29125,#29126,#29127,#29128,#29129,#29130,#29131,#29132,#29133,#29134,
#29135,#29136,#29137,#29138,#29139,#29140,#29141,#29142,#29143,#29144,#29145,
#29146,#29147,#29148,#29149,#29150,#29151,#29152,#29153,#29154,#29155,#29156,
#29157,#29158,#29159,#29160,#29161,#29162,#29163,#29164,#29165,#29166,#29167),
 .UNSPECIFIED.,.F.,.F.,(4,3,3,3,3,3,3,3,3,3,3,3,3,3,3,3,4),(0.,0.092754524514728,
0.125,0.216045473457587,0.25,0.34138223237852,0.375,0.466365066918033,0.5,
0.591365066918176,0.625,0.716382232378618,0.75,0.841045473457608,0.875,
0.967754524515514,1.),.UNSPECIFIED.);
#327=B_SPLINE_CURVE_WITH_KNOTS('',3,(#29168,#29169,#29170,#29171,#29172,
#29173,#29174,#29175,#29176,#29177,#29178,#29179,#29180,#29181,#29182,#29183,
#29184,#29185,#29186,#29187,#29188,#29189,#29190,#29191,#29192,#29193,#29194,
#29195,#29196,#29197,#29198,#29199,#29200,#29201,#29202,#29203,#29204,#29205,
#29206,#29207,#29208,#29209,#29210,#29211,#29212,#29213,#29214,#29215,#29216),
 .UNSPECIFIED.,.F.,.F.,(4,3,3,3,3,3,3,3,3,3,3,3,3,3,3,3,4),(0.,0.106472604170083,
0.125,0.229954011808637,0.25,0.35528007535872,0.375,0.4802448705967,0.5,
0.605244870596807,0.625,0.730280075360275,0.75,0.854954011808786,0.875,
0.98147260417198,1.),.UNSPECIFIED.);
#328=B_SPLINE_CURVE_WITH_KNOTS('',3,(#29217,#29218,#29219,#29220,#29221,
#29222,#29223,#29224,#29225,#29226,#29227,#29228,#29229,#29230,#29231,#29232,
#29233,#29234,#29235,#29236,#29237,#29238,#29239,#29240,#29241,#29242,#29243,
#29244,#29245,#29246,#29247,#29248,#29249,#29250,#29251,#29252,#29253,#29254,
#29255,#29256,#29257,#29258,#29259,#29260,#29261,#29262,#29263,#29264,#29265),
 .UNSPECIFIED.,.F.,.F.,(4,3,3,3,3,3,3,3,3,3,3,3,3,3,3,3,4),(0.,0.0927744783480364,
0.125,0.216065733758611,0.25,0.341402486168678,0.375,0.466385284884496,
0.5,0.591385284884159,0.625,0.716402486168833,0.75,0.841065733758618,0.875,
0.967774478348059,1.),.UNSPECIFIED.);
#329=B_SPLINE_CURVE_WITH_KNOTS('',3,(#29270,#29271,#29272,#29273,#29274,
#29275,#29276,#29277,#29278,#29279,#29280,#29281,#29282,#29283,#29284,#29285),
 .UNSPECIFIED.,.F.,.F.,(4,3,3,3,3,4),(-0.529687579579074,-0.331590427453144,
-0.219920121605962,-0.150766908575684,-0.0882648636903197,0.),
 .UNSPECIFIED.);
#330=B_SPLINE_CURVE_WITH_KNOTS('',3,(#29286,#29287,#29288,#29289,#29290,
#29291,#29292,#29293,#29294,#29295,#29296,#29297,#29298,#29299,#29300,#29301,
#29302,#29303,#29304),.UNSPECIFIED.,.F.,.F.,(4,3,3,3,3,3,4),(-0.425594667631933,
-0.326610996136396,-0.263194447999632,-0.22762732464086,-0.156642940697186,
-0.119119097859436,-0.000122244586405741),.UNSPECIFIED.);
#331=B_SPLINE_CURVE_WITH_KNOTS('',3,(#29306,#29307,#29308,#29309,#29310,
#29311,#29312,#29313,#29314,#29315,#29316,#29317,#29318,#29319,#29320,#29321,
#29322,#29323,#29324,#29325,#29326,#29327,#29328,#29329,#29330),
 .UNSPECIFIED.,.F.,.F.,(4,3,3,3,3,3,3,3,4),(-0.188664084190461,-0.152061353030785,
-0.128429664012943,-0.115458621871108,-0.0964653635667077,-0.0843255862211543,
-0.0416444979807187,-0.00599163753997056,0.),.UNSPECIFIED.);
#332=B_SPLINE_CURVE_WITH_KNOTS('',3,(#29331,#29332,#29333,#29334,#29335,
#29336,#29337,#29338,#29339,#29340,#29341,#29342,#29343,#29344,#29345,#29346,
#29347,#29348,#29349,#29350,#29351,#29352),.UNSPECIFIED.,.F.,.F.,(4,3,3,
3,3,3,3,4),(-0.312582490464858,-0.230760194515857,-0.19070267351417,-0.148937898566855,
-0.112852497416037,-0.0497426635164272,-0.0051444580421514,-0.000153083505448296),
 .UNSPECIFIED.);
#333=B_SPLINE_CURVE_WITH_KNOTS('',3,(#29372,#29373,#29374,#29375),
 .UNSPECIFIED.,.F.,.F.,(4,4),(0.537775768622803,0.537783217741629),
 .UNSPECIFIED.);
#334=B_SPLINE_CURVE_WITH_KNOTS('',3,(#29376,#29377,#29378,#29379,#29380,
#29381,#29382,#29383,#29384,#29385,#29386,#29387,#29388,#29389,#29390,#29391,
#29392,#29393,#29394,#29395,#29396,#29397,#29398,#29399,#29400,#29401,#29402,
#29403,#29404,#29405,#29406,#29407,#29408,#29409,#29410,#29411,#29412,#29413,
#29414,#29415,#29416,#29417,#29418,#29419,#29420,#29421,#29422,#29423,#29424,
#29425,#29426,#29427,#29428,#29429,#29430,#29431,#29432,#29433,#29434,#29435,
#29436,#29437,#29438,#29439,#29440,#29441,#29442,#29443,#29444,#29445,#29446,
#29447,#29448,#29449,#29450,#29451,#29452,#29453,#29454,#29455,#29456,#29457,
#29458,#29459,#29460,#29461,#29462,#29463,#29464,#29465,#29466,#29467,#29468,
#29469,#29470,#29471,#29472,#29473,#29474,#29475,#29476,#29477,#29478,#29479,
#29480,#29481,#29482,#29483,#29484,#29485,#29486,#29487,#29488,#29489,#29490,
#29491,#29492,#29493,#29494,#29495,#29496,#29497,#29498,#29499,#29500,#29501,
#29502,#29503,#29504,#29505,#29506,#29507,#29508,#29509,#29510,#29511,#29512,
#29513,#29514,#29515,#29516,#29517,#29518,#29519,#29520,#29521,#29522,#29523,
#29524,#29525,#29526,#29527,#29528,#29529,#29530,#29531,#29532,#29533,#29534,
#29535,#29536,#29537,#29538,#29539,#29540,#29541,#29542,#29543,#29544,#29545,
#29546,#29547,#29548,#29549,#29550,#29551,#29552,#29553,#29554,#29555,#29556,
#29557,#29558,#29559,#29560,#29561,#29562,#29563,#29564,#29565,#29566,#29567,
#29568,#29569,#29570,#29571,#29572,#29573,#29574,#29575),.UNSPECIFIED.,
 .F.,.F.,(4,2,2,2,2,2,2,2,2,2,2,2,2,2,2,2,2,2,2,2,2,2,2,2,2,2,2,2,2,2,2,
2,2,2,2,2,2,2,2,2,2,2,2,2,2,2,2,2,2,2,2,2,2,2,2,2,2,2,2,2,2,2,2,2,2,2,2,
2,2,2,2,2,2,2,2,2,2,2,2,2,2,2,2,2,2,2,2,2,2,2,2,2,2,2,2,2,2,2,2,4),(9.99999999815765E-7,
0.00248984042910974,0.00561629617446753,0.0121505941808296,0.0438670508689377,
0.0636585190425291,0.0732302639569316,0.0758178509753012,0.077398537873236,
0.0788665251219267,0.08100030653153,0.0862126925358243,0.129907811692407,
0.141218827496,0.149251312086533,0.152742148855637,0.155342482793766,0.15811933761236,
0.162508433617683,0.176408600881536,0.207278298350196,0.225317859375305,
0.229432767972491,0.231321325149154,0.232765166695651,0.234459828153989,
0.237510479782257,0.254272786683191,0.262028243731876,0.281367431819593,
0.294532997169395,0.303498302270635,0.307135984844374,0.30975812507255,
0.312480066164869,0.316623123308372,0.32834715694087,0.364471526036297,
0.380291775425887,0.384158484259675,0.385999655135213,0.387301916129383,
0.388973360713079,0.391915906101928,0.405858359578526,0.429859743425932,
0.453147683202867,0.459406094113763,0.462573915587413,0.465135685236222,
0.468085519691301,0.473144478384027,0.501090709371585,0.521197818454051,
0.53636743591904,0.539302624890517,0.540955700493059,0.542408832475035,
0.544336594881267,0.548611971336903,0.571807280426291,0.592595049163689,
0.610579334485302,0.615178136700596,0.617999412220788,0.620582974606797,
0.623908305821585,0.629473657635745,0.665762139295943,0.682938890144216,
0.691756005977596,0.694268762485516,0.695828724746857,0.697301533320525,
0.699125290134432,0.703657331174639,0.748249961533015,0.75961599685998,
0.767677212752748,0.771171716058845,0.773771451873097,0.77620897017638,
0.780277868989691,0.791420660087405,0.82814652339523,0.844065228409776,
0.847944836739026,0.849789541995181,0.851092821102683,0.852763168663429,
0.855701021110849,0.869548363739972,0.89361605863966,0.919124215601457,
0.92410332658099,0.92700652159823,0.929572811348499,0.932805875765826,0.939183891755464,
0.971367835775262),.UNSPECIFIED.);
#335=B_SPLINE_CURVE_WITH_KNOTS('',3,(#29576,#29577,#29578,#29579,#29580,
#29581,#29582,#29583,#29584,#29585,#29586,#29587,#29588,#29589,#29590,#29591,
#29592,#29593,#29594,#29595,#29596,#29597,#29598,#29599,#29600,#29601,#29602,
#29603,#29604,#29605,#29606,#29607,#29608,#29609,#29610,#29611,#29612,#29613,
#29614,#29615,#29616,#29617,#29618,#29619,#29620,#29621,#29622,#29623,#29624,
#29625,#29626,#29627,#29628,#29629,#29630,#29631,#29632,#29633,#29634,#29635,
#29636,#29637,#29638,#29639,#29640,#29641,#29642,#29643,#29644,#29645,#29646,
#29647,#29648,#29649,#29650,#29651,#29652,#29653,#29654,#29655,#29656,#29657,
#29658,#29659,#29660,#29661,#29662,#29663,#29664,#29665,#29666,#29667,#29668,
#29669,#29670,#29671,#29672,#29673,#29674,#29675,#29676,#29677,#29678,#29679,
#29680,#29681,#29682,#29683,#29684,#29685,#29686,#29687,#29688,#29689,#29690,
#29691,#29692,#29693,#29694,#29695,#29696,#29697,#29698,#29699,#29700,#29701,
#29702,#29703,#29704,#29705,#29706,#29707,#29708,#29709,#29710,#29711,#29712,
#29713,#29714,#29715,#29716,#29717,#29718,#29719,#29720,#29721,#29722,#29723,
#29724,#29725,#29726,#29727,#29728,#29729,#29730,#29731,#29732,#29733,#29734,
#29735,#29736,#29737,#29738,#29739,#29740,#29741,#29742,#29743,#29744,#29745,
#29746,#29747,#29748,#29749,#29750,#29751,#29752,#29753,#29754,#29755,#29756,
#29757,#29758,#29759,#29760,#29761,#29762,#29763,#29764,#29765,#29766,#29767,
#29768,#29769,#29770,#29771,#29772,#29773,#29774,#29775,#29776,#29777),
 .UNSPECIFIED.,.F.,.F.,(4,2,2,2,2,2,2,2,2,2,2,2,2,2,2,2,2,2,2,2,2,2,2,2,
2,2,2,2,2,2,2,2,2,2,2,2,2,2,2,2,2,2,2,2,2,2,2,2,2,2,2,2,2,2,2,2,2,2,2,2,
2,2,2,2,2,2,2,2,2,2,2,2,2,2,2,2,2,2,2,2,2,2,2,2,2,2,2,2,2,2,2,2,2,2,2,2,
2,2,2,2,4),(0.971346799428905,0.971393807723292,1.00248341395968,1.01353394040873,
1.01634507260716,1.01797506879581,1.01944139297462,1.02146845289682,1.02635989237911,
1.03353697284982,1.05784397528317,1.08664086907653,1.09167811617992,1.09462850001616,
1.09719882336612,1.10038783299113,1.10672505869199,1.1305881102961,1.1558491195431,
1.16802449405939,1.17090891968254,1.17255390322787,1.17401592605357,1.17601090279887,
1.18070182549438,1.18748175325983,1.20924226483471,1.23888227027299,1.24542305047163,
1.2486545037329,1.25123175338879,1.25416069957369,1.25921891469424,1.28695703721142,
1.31500785019909,1.32328028209969,1.32583578429263,1.32741103473521,1.32891094151386,
1.33109984015253,1.33701466447982,1.3463446509391,1.36734901133354,1.39560911445701,
1.40064758494378,1.40360463071679,1.40618467363479,1.40939112042748,1.41578264892817,
1.4400019745184,1.46593835726208,1.47718972238715,1.48001583436438,1.48164936741866,
1.48310707516813,1.48511120146793,1.48991414039928,1.49692632679696,1.52017464631029,
1.5480883158423,1.55467124583728,1.55789628881885,1.56045551001211,1.56334972438136,
1.56831028187733,1.59351167928391,1.60966700083135,1.63145055180715,1.6345771526172,
1.63628830128374,1.63773585107037,1.63961237947638,1.6436244231757,1.66060259999796,
1.69020088389503,1.70640405493955,1.71104625692704,1.71389500144778,1.71650470961001,
1.71992322841228,1.72742402960879,1.75269629251805,1.78351522487468,1.7883188449285,
1.79020759590426,1.79171760304882,1.79332027787656,1.79587382904581,1.80459989585764,
1.82143880069531,1.85626652138392,1.86181256634905,1.8652032056099,1.86783345108478,
1.87074782342507,1.87560101473461,1.89663034549709,1.92531077105376,1.93825773548782,
1.94103475003504,1.94279591973499),.UNSPECIFIED.);
#336=B_SPLINE_CURVE_WITH_KNOTS('',3,(#30118,#30119,#30120,#30121,#30122,
#30123,#30124,#30125,#30126,#30127,#30128,#30129,#30130,#30131,#30132,#30133,
#30134,#30135,#30136,#30137,#30138,#30139,#30140,#30141,#30142,#30143,#30144,
#30145),.UNSPECIFIED.,.F.,.F.,(4,3,3,3,3,3,3,3,3,4),(0.,0.0461567016013966,
0.10481637338886,0.141987909893012,0.148065501794539,0.187793278496004,
0.22417637037208,0.275733961853634,0.32759864266339,0.331419002748183),
 .UNSPECIFIED.);
#337=B_SPLINE_CURVE_WITH_KNOTS('',3,(#30486,#30487,#30488,#30489,#30490,
#30491,#30492,#30493,#30494,#30495,#30496,#30497,#30498,#30499,#30500,#30501,
#30502,#30503,#30504,#30505,#30506,#30507,#30508,#30509,#30510),
 .UNSPECIFIED.,.F.,.F.,(4,3,3,3,3,3,3,3,4),(0.,0.0451591013560227,0.0863053370931954,
0.114402431924666,0.128866540493028,0.15651567637735,0.208426240523224,
0.23219202465052,0.233592218228785),.UNSPECIFIED.);
#338=B_SPLINE_CURVE_WITH_KNOTS('',3,(#30515,#30516,#30517,#30518,#30519,
#30520,#30521),.UNSPECIFIED.,.F.,.F.,(4,3,4),(-0.0356563315348787,-0.0168385637965097,
-6.00712216046093E-6),.UNSPECIFIED.);
#339=B_SPLINE_CURVE_WITH_KNOTS('',3,(#30523,#30524,#30525,#30526),
 .UNSPECIFIED.,.F.,.F.,(4,4),(0.0706728850407956,0.0856518761238354),
 .UNSPECIFIED.);
#340=B_SPLINE_CURVE_WITH_KNOTS('',3,(#30528,#30529,#30530,#30531,#30532,
#30533),.UNSPECIFIED.,.F.,.F.,(4,2,4),(-0.0693808026657025,-0.0346741578608072,
-9.99911564922296E-7),.UNSPECIFIED.);
#341=B_SPLINE_CURVE_WITH_KNOTS('',3,(#30535,#30536,#30537,#30538,#30539,
#30540),.UNSPECIFIED.,.F.,.F.,(4,2,4),(0.220967788015232,0.232496868866944,
0.26115278337561),.UNSPECIFIED.);
#342=B_SPLINE_CURVE_WITH_KNOTS('',3,(#30541,#30542,#30543,#30544,#30545,
#30546,#30547,#30548,#30549,#30550,#30551,#30552,#30553,#30554,#30555,#30556,
#30557,#30558,#30559,#30560,#30561,#30562,#30563,#30564),.UNSPECIFIED.,
 .F.,.F.,(4,2,2,2,2,2,2,2,2,2,2,4),(-0.0545071100794137,-0.0346117647175132,
-0.0288940964902406,-0.027947926335196,-0.0276921717992136,-0.0275391564768281,
-0.0274029213244984,-0.0272315883107351,-0.0268910373658706,-0.02438570236167,
-0.0184895448929481,-0.000174302815414135),.UNSPECIFIED.);
#343=B_SPLINE_CURVE_WITH_KNOTS('',3,(#30566,#30567,#30568,#30569,#30570,
#30571),.UNSPECIFIED.,.F.,.F.,(4,2,4),(-0.0566586033688786,-0.0284132480267369,
-0.000146512503515223),.UNSPECIFIED.);
#344=B_SPLINE_CURVE_WITH_KNOTS('',3,(#30573,#30574,#30575,#30576,#30577,
#30578),.UNSPECIFIED.,.F.,.F.,(4,2,4),(0.296274329747878,0.305955146920116,
0.308739916339329),.UNSPECIFIED.);
#345=B_SPLINE_CURVE_WITH_KNOTS('',3,(#30580,#30581,#30582,#30583,#30584,
#30585,#30586),.UNSPECIFIED.,.F.,.F.,(4,3,4),(-0.0322922670327419,-0.0168989031257184,
0.),.UNSPECIFIED.);
#346=B_SPLINE_CURVE_WITH_KNOTS('',3,(#30590,#30591,#30592,#30593,#30594,
#30595),.UNSPECIFIED.,.F.,.F.,(4,2,4),(-0.0526090819005489,-0.0263046029830051,
-9.9999999843628E-7),.UNSPECIFIED.);
#347=B_SPLINE_CURVE_WITH_KNOTS('',3,(#30599,#30600,#30601,#30602,#30603,
#30604,#30605,#30606),.UNSPECIFIED.,.F.,.F.,(4,2,2,4),(-0.0944036996742436,
-0.0771433030461012,-0.0485319215546893,0.),.UNSPECIFIED.);
#348=B_SPLINE_CURVE_WITH_KNOTS('',3,(#30610,#30611,#30612,#30613,#30614,
#30615,#30616),.UNSPECIFIED.,.F.,.F.,(4,3,4),(-0.0357121223372438,-0.0174889920223166,
0.),.UNSPECIFIED.);
#349=B_SPLINE_CURVE_WITH_KNOTS('',3,(#30618,#30619,#30620,#30621),
 .UNSPECIFIED.,.F.,.F.,(4,4),(0.,0.997468283692927),.UNSPECIFIED.);
#350=B_SPLINE_CURVE_WITH_KNOTS('',3,(#30622,#30623,#30624,#30625,#30626,
#30627,#30628,#30629,#30630,#30631,#30632,#30633,#30634,#30635,#30636,#30637,
#30638,#30639,#30640,#30641,#30642,#30643,#30644,#30645,#30646,#30647,#30648,
#30649),.UNSPECIFIED.,.F.,.F.,(4,2,2,2,2,2,2,2,2,2,2,2,2,4),(-0.125771117028632,
-0.0864552223641016,-0.0678485902550579,-0.0594428399644161,-0.0575924114249427,
-0.0571183863442095,-0.0568468165768063,-0.0566394520287764,-0.0563729061938286,
-0.0559085649950657,-0.0539526314959845,-0.0456980560831236,-0.0292561698449011,
0.),.UNSPECIFIED.);
#351=B_SPLINE_CURVE_WITH_KNOTS('',3,(#30651,#30652,#30653,#30654,#30655,
#30656,#30657),.UNSPECIFIED.,.F.,.F.,(4,3,4),(-0.0385164580871794,-0.0188401674254162,
0.),.UNSPECIFIED.);
#352=B_SPLINE_CURVE_WITH_KNOTS('',3,(#30661,#30662,#30663,#30664,#30665,
#30666,#30667),.UNSPECIFIED.,.F.,.F.,(4,3,4),(-0.0626263501111082,-0.0313079089847344,
-0.000161268437901824),.UNSPECIFIED.);
#353=B_SPLINE_CURVE_WITH_KNOTS('',3,(#30669,#30670,#30671,#30672),
 .UNSPECIFIED.,.F.,.F.,(4,4),(0.754529901247614,0.766860984898717),
 .UNSPECIFIED.);
#354=B_SPLINE_CURVE_WITH_KNOTS('',3,(#30674,#30675,#30676,#30677,#30678,
#30679,#30680),.UNSPECIFIED.,.F.,.F.,(4,3,4),(-0.0311458227321188,-0.0161494601786653,
0.),.UNSPECIFIED.);
#355=B_SPLINE_CURVE_WITH_KNOTS('',3,(#30965,#30966,#30967,#30968,#30969,
#30970,#30971,#30972,#30973,#30974,#30975,#30976,#30977,#30978,#30979,#30980,
#30981,#30982,#30983,#30984,#30985,#30986,#30987,#30988,#30989,#30990,#30991,
#30992,#30993,#30994,#30995,#30996,#30997,#30998,#30999,#31000,#31001,#31002,
#31003,#31004,#31005,#31006,#31007,#31008,#31009,#31010,#31011,#31012,#31013),
 .UNSPECIFIED.,.F.,.F.,(4,3,3,3,3,3,3,3,3,3,3,3,3,3,3,3,4),(-0.503648702838972,
-0.478239118516134,-0.425663343805114,-0.419651033765898,-0.414757025337115,
-0.360029409919934,-0.345036067010815,-0.332450646380526,-0.328029406469616,
-0.242050926335671,-0.24008266664698,-0.222356647888336,-0.119796523329524,
-0.115154566521774,-0.11055320579857,-0.0210267271158198,-3.70377469171095E-5),
 .UNSPECIFIED.);
#356=B_SPLINE_CURVE_WITH_KNOTS('',3,(#31015,#31016,#31017,#31018,#31019,
#31020,#31021,#31022,#31023,#31024,#31025,#31026,#31027),.UNSPECIFIED.,
 .F.,.F.,(4,3,3,3,4),(0.,0.304030668972893,0.5,0.804030668972894,0.999999999999386),
 .UNSPECIFIED.);
#357=B_SPLINE_CURVE_WITH_KNOTS('',3,(#31029,#31030,#31031,#31032,#31033,
#31034,#31035,#31036,#31037,#31038,#31039,#31040,#31041,#31042,#31043,#31044,
#31045,#31046,#31047,#31048,#31049,#31050,#31051,#31052,#31053,#31054,#31055,
#31056,#31057,#31058,#31059,#31060,#31061,#31062,#31063,#31064,#31065,#31066,
#31067,#31068,#31069,#31070,#31071,#31072,#31073,#31074,#31075,#31076,#31077),
 .UNSPECIFIED.,.F.,.F.,(4,3,3,3,3,3,3,3,3,3,3,3,3,3,3,3,4),(0.,0.0886407066381885,
0.125,0.212008098936426,0.25,0.337329846599543,0.375,0.462313411756197,
0.5,0.587313411756187,0.625,0.712329846599542,0.75,0.837008098936432,0.875,
0.963640706638148,1.),.UNSPECIFIED.);
#358=B_SPLINE_CURVE_WITH_KNOTS('',3,(#31079,#31080,#31081,#31082,#31083,
#31084,#31085,#31086,#31087,#31088,#31089,#31090,#31091,#31092,#31093,#31094,
#31095,#31096,#31097,#31098,#31099,#31100,#31101,#31102,#31103,#31104,#31105,
#31106,#31107,#31108,#31109,#31110,#31111,#31112,#31113,#31114,#31115,#31116,
#31117,#31118,#31119,#31120,#31121,#31122,#31123,#31124,#31125,#31126,#31127),
 .UNSPECIFIED.,.F.,.F.,(4,3,3,3,3,3,3,3,3,3,3,3,3,3,3,3,4),(0.,0.0886171082475257,
0.125,0.211984138088812,0.25,0.337305893446915,0.375,0.46228950097559,0.5,
0.587289500975586,0.625,0.712305893446908,0.75,0.836984138088813,0.875,
0.963617108247523,1.),.UNSPECIFIED.);
#359=B_SPLINE_CURVE_WITH_KNOTS('',3,(#31129,#31130,#31131,#31132,#31133,
#31134,#31135,#31136,#31137,#31138,#31139,#31140,#31141,#31142,#31143,#31144,
#31145,#31146,#31147,#31148,#31149,#31150,#31151,#31152,#31153,#31154,#31155,
#31156,#31157,#31158,#31159,#31160,#31161,#31162,#31163,#31164,#31165,#31166,
#31167,#31168,#31169,#31170,#31171,#31172,#31173,#31174,#31175,#31176,#31177),
 .UNSPECIFIED.,.F.,.F.,(4,3,3,3,3,3,3,3,3,3,3,3,3,3,3,3,4),(0.,0.088620284495184,
0.125,0.211987363129608,0.25,0.337309117454998,0.375,0.462292719277718,
0.5,0.587292719277716,0.625,0.712309117455,0.75,0.836987363129601,0.875,
0.963620284495189,1.),.UNSPECIFIED.);
#360=B_SPLINE_CURVE_WITH_KNOTS('',3,(#31179,#31180,#31181,#31182,#31183,
#31184,#31185,#31186,#31187,#31188,#31189,#31190,#31191,#31192,#31193,#31194,
#31195,#31196,#31197,#31198,#31199,#31200,#31201,#31202,#31203,#31204,#31205,
#31206,#31207,#31208,#31209,#31210,#31211,#31212,#31213,#31214,#31215,#31216,
#31217,#31218,#31219,#31220,#31221,#31222,#31223,#31224,#31225,#31226,#31227),
 .UNSPECIFIED.,.F.,.F.,(4,3,3,3,3,3,3,3,3,3,3,3,3,3,3,3,4),(0.,0.0886382763954242,
0.125,0.212005631372845,0.25,0.337327379830824,0.375,0.462310949348795,
0.5,0.587310949348818,0.625,0.712327379830809,0.75,0.837005631372844,0.875,
0.963638276395463,1.),.UNSPECIFIED.);
#361=B_SPLINE_CURVE_WITH_KNOTS('',3,(#31229,#31230,#31231,#31232,#31233,
#31234,#31235,#31236,#31237,#31238,#31239,#31240,#31241,#31242,#31243,#31244,
#31245,#31246,#31247,#31248,#31249,#31250,#31251,#31252,#31253,#31254,#31255,
#31256,#31257,#31258,#31259,#31260,#31261,#31262,#31263,#31264,#31265,#31266,
#31267,#31268,#31269,#31270,#31271,#31272,#31273,#31274,#31275,#31276,#31277),
 .UNSPECIFIED.,.F.,.F.,(4,3,3,3,3,3,3,3,3,3,3,3,3,3,3,3,4),(0.,0.0886104150389065,
0.125,0.211978952212712,0.25,0.337305502283307,0.375,0.462245050243597,
0.5,0.587333772189201,0.625,0.712305979497255,0.75,0.836989031823058,0.875,
0.96362351292812,1.),.UNSPECIFIED.);
#362=B_SPLINE_CURVE_WITH_KNOTS('',3,(#31279,#31280,#31281,#31282,#31283,
#31284,#31285,#31286,#31287,#31288,#31289,#31290,#31291,#31292,#31293,#31294,
#31295,#31296,#31297,#31298,#31299,#31300,#31301,#31302,#31303,#31304,#31305,
#31306,#31307,#31308,#31309,#31310,#31311,#31312,#31313,#31314,#31315,#31316,
#31317,#31318,#31319,#31320,#31321,#31322,#31323,#31324,#31325,#31326,#31327),
 .UNSPECIFIED.,.F.,.F.,(4,3,3,3,3,3,3,3,3,3,3,3,3,3,3,3,4),(0.,0.0886243992808492,
0.125,0.211991541122404,0.25,0.337313294108582,0.375,0.462296888540609,
0.5,0.587296888540603,0.625,0.712313294108576,0.75,0.836991541122409,0.875,
0.96362439928086,1.),.UNSPECIFIED.);
#363=B_SPLINE_CURVE_WITH_KNOTS('',3,(#31329,#31330,#31331,#31332,#31333,
#31334,#31335,#31336,#31337,#31338,#31339,#31340,#31341,#31342,#31343,#31344,
#31345,#31346,#31347,#31348,#31349,#31350,#31351,#31352,#31353,#31354,#31355,
#31356,#31357,#31358,#31359,#31360,#31361,#31362,#31363,#31364,#31365,#31366,
#31367,#31368,#31369,#31370,#31371,#31372,#31373,#31374,#31375,#31376,#31377),
 .UNSPECIFIED.,.F.,.F.,(4,3,3,3,3,3,3,3,3,3,3,3,3,3,3,3,4),(0.,0.0886329632205807,
0.125,0.212000236599526,0.25,0.337321986793343,0.375,0.462305565848219,
0.5,0.587305565848244,0.625,0.712321986793333,0.75,0.83700023659952,0.875,
0.963632963220574,1.),.UNSPECIFIED.);
#364=B_SPLINE_CURVE_WITH_KNOTS('',3,(#31379,#31380,#31381,#31382,#31383,
#31384,#31385,#31386,#31387,#31388,#31389,#31390,#31391,#31392,#31393,#31394,
#31395,#31396,#31397,#31398,#31399,#31400,#31401,#31402,#31403,#31404,#31405,
#31406,#31407,#31408,#31409,#31410,#31411,#31412,#31413,#31414,#31415,#31416,
#31417,#31418,#31419,#31420,#31421,#31422,#31423,#31424,#31425,#31426,#31427,
#31428,#31429,#31430,#31431,#31432,#31433,#31434,#31435,#31436,#31437,#31438,
#31439,#31440,#31441,#31442,#31443,#31444,#31445,#31446,#31447,#31448,#31449,
#31450,#31451,#31452,#31453,#31454,#31455,#31456,#31457),.UNSPECIFIED.,
 .F.,.F.,(4,3,3,3,3,3,3,3,3,3,3,3,3,3,3,3,3,3,3,3,3,3,3,3,3,3,4),(0.,0.0888061128071974,
0.103629824354861,0.125,0.211608444540927,0.25,0.261105648823599,0.337106991491099,
0.375,0.418504729011411,0.4375,0.46875,0.484375,0.5,0.515625,0.53125,0.5625,
0.592028433976737,0.625,0.6875,0.75,0.760059091463865,0.831314636644941,
0.875,0.907035057496371,0.948814674685162,1.),.UNSPECIFIED.);
#365=B_SPLINE_CURVE_WITH_KNOTS('',3,(#31459,#31460,#31461,#31462,#31463,
#31464,#31465,#31466,#31467,#31468,#31469,#31470,#31471,#31472,#31473,#31474,
#31475,#31476,#31477,#31478,#31479,#31480,#31481,#31482,#31483,#31484,#31485,
#31486,#31487,#31488,#31489,#31490,#31491,#31492,#31493,#31494,#31495,#31496,
#31497,#31498,#31499,#31500,#31501,#31502,#31503,#31504,#31505,#31506,#31507),
 .UNSPECIFIED.,.F.,.F.,(4,3,3,3,3,3,3,3,3,3,3,3,3,3,3,3,4),(0.,0.0886284882868581,
0.125,0.211995692935443,0.25,0.337317444589203,0.375,0.462301031678349,
0.5,0.587301031678344,0.625,0.712317444589205,0.75,0.836995692935444,0.875,
0.963628488286822,1.),.UNSPECIFIED.);
#366=B_SPLINE_CURVE_WITH_KNOTS('',3,(#31508,#31509,#31510,#31511,#31512,
#31513,#31514,#31515,#31516,#31517,#31518,#31519,#31520,#31521,#31522,#31523,
#31524,#31525,#31526,#31527,#31528,#31529,#31530,#31531,#31532,#31533,#31534,
#31535,#31536,#31537,#31538,#31539,#31540,#31541,#31542,#31543,#31544,#31545,
#31546,#31547,#31548,#31549,#31550,#31551,#31552,#31553,#31554,#31555,#31556),
 .UNSPECIFIED.,.F.,.F.,(4,3,3,3,3,3,3,3,3,3,3,3,3,3,3,3,4),(0.,0.109960626274433,
0.125,0.233606518241178,0.25,0.358908048100772,0.375,0.483868300041721,
0.5,0.608868300041721,0.625,0.733908048100777,0.75,0.858606518241174,0.875,
0.984960626274394,1.),.UNSPECIFIED.);
#367=B_SPLINE_CURVE_WITH_KNOTS('',3,(#31834,#31835,#31836,#31837,#31838,
#31839,#31840,#31841,#31842,#31843,#31844,#31845,#31846,#31847,#31848,#31849,
#31850,#31851,#31852,#31853,#31854,#31855,#31856,#31857,#31858,#31859,#31860,
#31861,#31862,#31863,#31864,#31865,#31866,#31867,#31868,#31869,#31870,#31871,
#31872,#31873,#31874,#31875,#31876,#31877,#31878,#31879,#31880,#31881,#31882),
 .UNSPECIFIED.,.F.,.F.,(4,3,3,3,3,3,3,3,3,3,3,3,3,3,3,3,4),(-0.501724005229533,
-0.472416574319748,-0.414389357077405,-0.407358038783487,-0.400886943772423,
-0.314043010674865,-0.309619504665006,-0.305251689160703,-0.222333474861526,
-0.217225768055783,-0.208375447427435,-0.203501118200736,-0.199345077371566,
-0.101201676292347,-0.096184718783614,-0.017180163401669,0.),
 .UNSPECIFIED.);
#368=B_SPLINE_CURVE_WITH_KNOTS('',3,(#31884,#31885,#31886,#31887,#31888,
#31889,#31890,#31891,#31892,#31893,#31894,#31895,#31896,#31897,#31898,#31899,
#31900,#31901,#31902,#31903,#31904,#31905,#31906,#31907,#31908),
 .UNSPECIFIED.,.F.,.F.,(4,3,3,3,3,3,3,3,4),(0.,0.172429158239796,0.25,0.41907286168834,
0.5,0.669072861688337,0.75,0.922429158239836,0.999999999999765),
 .UNSPECIFIED.);
#369=B_SPLINE_CURVE_WITH_KNOTS('',3,(#31910,#31911,#31912,#31913,#31914,
#31915,#31916,#31917,#31918,#31919,#31920,#31921,#31922,#31923,#31924,#31925,
#31926,#31927,#31928,#31929,#31930,#31931,#31932,#31933,#31934,#31935,#31936,
#31937,#31938,#31939,#31940,#31941,#31942,#31943,#31944,#31945,#31946,#31947,
#31948,#31949,#31950,#31951,#31952,#31953,#31954,#31955,#31956,#31957,#31958,
#31959,#31960,#31961,#31962,#31963,#31964,#31965,#31966,#31967,#31968,#31969,
#31970,#31971,#31972,#31973,#31974,#31975,#31976,#31977,#31978,#31979,#31980,
#31981,#31982,#31983,#31984,#31985,#31986,#31987,#31988,#31989,#31990,#31991,
#31992,#31993,#31994,#31995,#31996,#31997,#31998,#31999,#32000,#32001,#32002,
#32003,#32004,#32005,#32006,#32007,#32008,#32009,#32010,#32011,#32012,#32013,
#32014,#32015,#32016,#32017,#32018,#32019,#32020,#32021,#32022,#32023,#32024,
#32025,#32026,#32027,#32028,#32029,#32030,#32031,#32032,#32033,#32034,#32035,
#32036,#32037,#32038,#32039,#32040,#32041,#32042,#32043,#32044,#32045,#32046,
#32047,#32048,#32049,#32050,#32051,#32052,#32053,#32054,#32055,#32056,#32057,
#32058,#32059,#32060,#32061,#32062,#32063,#32064,#32065,#32066,#32067,#32068,
#32069,#32070,#32071,#32072,#32073,#32074,#32075,#32076,#32077,#32078,#32079,
#32080,#32081,#32082,#32083,#32084,#32085,#32086,#32087,#32088,#32089,#32090,
#32091,#32092,#32093,#32094,#32095,#32096,#32097,#32098,#32099,#32100,#32101,
#32102,#32103,#32104,#32105,#32106,#32107,#32108,#32109,#32110,#32111),
 .UNSPECIFIED.,.F.,.F.,(4,2,2,2,2,2,2,2,2,2,2,2,2,2,2,2,2,2,2,2,2,2,2,2,
2,2,2,2,2,2,2,2,2,2,2,2,2,2,2,2,2,2,2,2,2,2,2,2,2,2,2,2,2,2,2,2,2,2,2,2,
2,2,2,2,2,2,2,2,2,2,2,2,2,2,2,2,2,2,2,2,2,2,2,2,2,2,2,2,2,2,2,2,2,2,2,2,
2,2,2,2,4),(0.000124435018137221,0.01427599667095,0.0243402584564738,0.0301983218783695,
0.0358628192640442,0.0422528806565145,0.0523393192149522,0.0865312582670473,
0.136171966071755,0.160734773100723,0.170657187299706,0.178238857463452,
0.182210202789374,0.185547378691446,0.189861506823648,0.199464405494597,
0.258108251018683,0.311375935039054,0.323142446876579,0.329888503625282,
0.3358138160006,0.343259360311408,0.355110933842989,0.432903026416704,0.457832505183502,
0.472529140837405,0.477657541990267,0.481106345805127,0.484724116078588,
0.490657440458818,0.511293397342995,0.560725822381833,0.59403432898518,
0.608643282163014,0.620455708549381,0.627206506509566,0.633123230873407,
0.640540751689568,0.652311271688271,0.730499159782864,0.76401724395515,
0.772388244729275,0.776515381350157,0.779839988738716,0.784031102655559,
0.792726815870931,0.843911347931676,0.866563405595919,0.894661236322197,
0.9138157939059,0.92192335961171,0.927933113919541,0.934348506148276,0.944544647984111,
0.98350704921781,1.01906819990235,1.06052822829088,1.06941574992997,1.07364670922496,
1.07698254932194,1.0811015062499,1.08937175975122,1.12189836898887,1.20140338238339,
1.21282063103088,1.22014726103616,1.22607532585814,1.23293240138814,1.24518927319071,
1.28493904976871,1.34126667017682,1.36246187645625,1.36844893652607,1.37208155635995,
1.37550091354802,1.38055206013141,1.3948237395594,1.41869783627087,1.49959570793514,
1.51088580859953,1.51814116132588,1.52401511182766,1.53081150366052,1.54295879950415,
1.58227574527781,1.63299918458442,1.65952038956469,1.66588272908685,1.66958353729213,
1.67298028478349,1.67782785422248,1.69042829604107,1.74635120632815,1.79242737219772,
1.8081116244709,1.81564980836978,1.82160777711801,1.82834799265712,1.83538252057036,
1.85275364928988,1.88917416055493),.UNSPECIFIED.);
#370=B_SPLINE_CURVE_WITH_KNOTS('',3,(#32113,#32114,#32115,#32116,#32117,
#32118,#32119,#32120,#32121,#32122,#32123,#32124,#32125,#32126,#32127,#32128,
#32129,#32130,#32131,#32132,#32133,#32134,#32135,#32136,#32137,#32138,#32139,
#32140,#32141,#32142,#32143,#32144,#32145,#32146,#32147,#32148,#32149,#32150,
#32151,#32152,#32153,#32154,#32155,#32156,#32157,#32158,#32159,#32160,#32161,
#32162,#32163,#32164,#32165,#32166,#32167,#32168,#32169,#32170,#32171,#32172,
#32173,#32174,#32175,#32176,#32177,#32178,#32179,#32180,#32181,#32182,#32183,
#32184,#32185,#32186,#32187,#32188,#32189,#32190,#32191,#32192,#32193,#32194,
#32195,#32196,#32197,#32198,#32199,#32200,#32201,#32202,#32203,#32204,#32205,
#32206,#32207,#32208,#32209,#32210,#32211,#32212,#32213,#32214,#32215,#32216,
#32217,#32218,#32219,#32220,#32221,#32222,#32223,#32224,#32225,#32226,#32227,
#32228,#32229,#32230,#32231,#32232,#32233,#32234,#32235,#32236,#32237,#32238,
#32239,#32240,#32241,#32242,#32243,#32244,#32245,#32246,#32247,#32248,#32249,
#32250,#32251,#32252,#32253,#32254,#32255,#32256,#32257,#32258,#32259,#32260,
#32261,#32262,#32263,#32264,#32265,#32266,#32267,#32268,#32269,#32270,#32271,
#32272,#32273,#32274,#32275,#32276,#32277,#32278,#32279,#32280,#32281,#32282,
#32283,#32284,#32285,#32286,#32287,#32288,#32289,#32290,#32291,#32292,#32293,
#32294,#32295,#32296,#32297,#32298,#32299,#32300,#32301,#32302,#32303,#32304,
#32305,#32306,#32307,#32308,#32309,#32310,#32311,#32312,#32313,#32314,#32315,
#32316,#32317,#32318,#32319,#32320,#32321,#32322,#32323,#32324,#32325,#32326,
#32327,#32328,#32329,#32330,#32331,#32332,#32333,#32334,#32335,#32336,#32337,
#32338,#32339,#32340,#32341,#32342,#32343,#32344,#32345,#32346,#32347,#32348,
#32349,#32350,#32351,#32352,#32353,#32354,#32355,#32356,#32357,#32358,#32359,
#32360,#32361,#32362,#32363,#32364,#32365,#32366,#32367,#32368,#32369,#32370,
#32371,#32372,#32373,#32374,#32375,#32376,#32377,#32378,#32379,#32380,#32381,
#32382,#32383,#32384,#32385,#32386,#32387,#32388,#32389,#32390,#32391,#32392,
#32393,#32394,#32395,#32396,#32397,#32398,#32399,#32400,#32401,#32402,#32403,
#32404,#32405,#32406,#32407,#32408,#32409,#32410,#32411,#32412,#32413,#32414,
#32415,#32416,#32417,#32418,#32419,#32420,#32421,#32422,#32423,#32424,#32425,
#32426,#32427,#32428,#32429,#32430,#32431,#32432,#32433,#32434,#32435,#32436,
#32437,#32438,#32439,#32440,#32441,#32442,#32443,#32444,#32445,#32446,#32447,
#32448,#32449,#32450,#32451,#32452,#32453,#32454,#32455,#32456,#32457,#32458,
#32459,#32460,#32461,#32462,#32463,#32464,#32465,#32466,#32467,#32468,#32469,
#32470,#32471,#32472,#32473,#32474,#32475,#32476,#32477,#32478,#32479,#32480,
#32481,#32482,#32483,#32484,#32485,#32486,#32487,#32488,#32489,#32490,#32491,
#32492,#32493,#32494,#32495,#32496,#32497,#32498,#32499,#32500,#32501,#32502,
#32503,#32504,#32505,#32506,#32507,#32508,#32509,#32510,#32511,#32512,#32513,
#32514,#32515,#32516,#32517,#32518,#32519,#32520,#32521,#32522,#32523,#32524,
#32525,#32526,#32527,#32528,#32529,#32530,#32531,#32532,#32533,#32534,#32535,
#32536,#32537,#32538,#32539,#32540,#32541,#32542,#32543,#32544,#32545,#32546,
#32547,#32548,#32549,#32550,#32551,#32552,#32553,#32554,#32555,#32556,#32557,
#32558,#32559,#32560,#32561,#32562,#32563,#32564,#32565,#32566,#32567,#32568,
#32569,#32570,#32571,#32572,#32573,#32574,#32575,#32576,#32577,#32578,#32579,
#32580,#32581,#32582,#32583,#32584,#32585,#32586,#32587,#32588,#32589,#32590,
#32591,#32592,#32593,#32594,#32595,#32596,#32597,#32598,#32599,#32600,#32601,
#32602,#32603,#32604,#32605,#32606,#32607,#32608,#32609,#32610,#32611,#32612,
#32613,#32614,#32615,#32616,#32617,#32618,#32619,#32620,#32621,#32622,#32623,
#32624,#32625,#32626,#32627,#32628,#32629,#32630,#32631,#32632,#32633,#32634,
#32635,#32636,#32637,#32638,#32639,#32640,#32641,#32642,#32643,#32644,#32645,
#32646,#32647,#32648,#32649,#32650,#32651,#32652,#32653,#32654,#32655,#32656,
#32657,#32658,#32659,#32660,#32661,#32662,#32663,#32664,#32665,#32666,#32667,
#32668,#32669,#32670,#32671,#32672,#32673,#32674,#32675,#32676,#32677,#32678,
#32679,#32680,#32681,#32682,#32683,#32684,#32685,#32686,#32687,#32688,#32689,
#32690,#32691,#32692,#32693,#32694,#32695,#32696,#32697,#32698,#32699,#32700,
#32701,#32702,#32703,#32704,#32705,#32706,#32707,#32708,#32709,#32710,#32711,
#32712,#32713,#32714,#32715,#32716,#32717,#32718,#32719,#32720,#32721,#32722,
#32723,#32724,#32725,#32726,#32727,#32728,#32729,#32730,#32731,#32732,#32733,
#32734,#32735,#32736,#32737,#32738,#32739,#32740,#32741,#32742,#32743,#32744,
#32745,#32746,#32747,#32748,#32749,#32750,#32751,#32752,#32753,#32754,#32755,
#32756,#32757,#32758,#32759,#32760,#32761,#32762,#32763,#32764,#32765,#32766,
#32767,#32768,#32769,#32770,#32771,#32772,#32773,#32774,#32775,#32776,#32777,
#32778,#32779,#32780,#32781,#32782,#32783,#32784,#32785,#32786,#32787,#32788,
#32789,#32790,#32791,#32792,#32793,#32794,#32795,#32796,#32797,#32798,#32799,
#32800,#32801,#32802,#32803,#32804,#32805,#32806,#32807,#32808,#32809,#32810,
#32811,#32812,#32813,#32814,#32815,#32816,#32817,#32818,#32819,#32820,#32821,
#32822,#32823,#32824,#32825,#32826,#32827,#32828,#32829,#32830,#32831,#32832,
#32833,#32834,#32835,#32836,#32837,#32838,#32839,#32840,#32841,#32842,#32843,
#32844,#32845,#32846,#32847,#32848,#32849,#32850,#32851,#32852,#32853,#32854,
#32855,#32856,#32857,#32858,#32859,#32860,#32861,#32862,#32863,#32864,#32865,
#32866,#32867,#32868,#32869,#32870,#32871,#32872,#32873,#32874,#32875,#32876,
#32877,#32878,#32879,#32880,#32881,#32882,#32883,#32884,#32885,#32886,#32887,
#32888,#32889,#32890,#32891,#32892,#32893,#32894,#32895,#32896,#32897,#32898,
#32899,#32900,#32901,#32902,#32903,#32904,#32905,#32906,#32907,#32908,#32909,
#32910,#32911,#32912,#32913,#32914,#32915,#32916,#32917,#32918,#32919,#32920,
#32921,#32922,#32923,#32924,#32925,#32926,#32927,#32928,#32929,#32930,#32931,
#32932,#32933,#32934,#32935,#32936,#32937,#32938,#32939,#32940,#32941,#32942,
#32943,#32944,#32945,#32946,#32947,#32948,#32949,#32950,#32951,#32952,#32953,
#32954,#32955,#32956,#32957,#32958,#32959,#32960,#32961,#32962,#32963,#32964,
#32965,#32966,#32967,#32968,#32969,#32970,#32971,#32972,#32973,#32974,#32975,
#32976,#32977,#32978,#32979,#32980,#32981,#32982,#32983,#32984,#32985,#32986,
#32987,#32988,#32989,#32990,#32991,#32992,#32993,#32994,#32995,#32996,#32997,
#32998,#32999,#33000,#33001,#33002,#33003,#33004,#33005,#33006,#33007,#33008,
#33009,#33010,#33011,#33012,#33013,#33014,#33015,#33016,#33017,#33018,#33019,
#33020,#33021,#33022,#33023,#33024,#33025,#33026,#33027,#33028,#33029,#33030,
#33031,#33032,#33033,#33034,#33035,#33036,#33037,#33038,#33039,#33040,#33041,
#33042,#33043,#33044,#33045,#33046,#33047,#33048,#33049,#33050,#33051,#33052,
#33053,#33054,#33055,#33056,#33057,#33058,#33059,#33060,#33061,#33062,#33063,
#33064,#33065,#33066,#33067,#33068),.UNSPECIFIED.,.F.,.F.,(4,2,2,2,2,2,
2,2,2,2,2,2,2,2,2,2,2,2,2,2,2,2,2,2,2,2,2,2,2,2,2,2,2,2,2,2,2,2,2,2,2,2,
2,2,2,2,2,2,2,2,2,2,2,2,2,2,2,2,2,2,2,2,2,2,2,2,2,2,2,2,2,2,2,2,2,2,2,2,
2,2,2,2,2,2,2,2,2,2,2,2,2,2,2,2,2,2,2,2,2,2,2,2,2,2,2,2,2,2,2,2,2,2,2,2,
2,2,2,2,2,2,2,2,2,2,2,2,2,2,2,2,2,2,2,2,2,2,2,2,2,2,2,2,2,2,2,2,2,2,2,2,
2,2,2,2,2,2,2,2,2,2,2,2,2,2,2,2,2,2,2,2,2,2,2,2,2,2,2,2,2,2,2,2,2,2,2,2,
2,2,2,2,2,2,2,2,2,2,2,2,2,2,2,2,2,2,2,2,2,2,2,2,2,2,2,2,2,2,2,2,2,2,2,2,
2,2,2,2,2,2,2,2,2,2,2,2,2,2,2,2,2,2,2,2,2,2,2,2,2,2,2,2,2,2,2,2,2,2,2,2,
2,2,2,2,2,2,2,2,2,2,2,2,2,2,2,2,2,2,2,2,2,2,2,2,2,2,2,2,2,2,2,2,2,2,2,2,
2,2,2,2,2,2,2,2,2,2,2,2,2,2,2,2,2,2,2,2,2,2,2,2,2,2,2,2,2,2,2,2,2,2,2,2,
2,2,2,2,2,2,2,2,2,2,2,2,2,2,2,2,2,2,2,2,2,2,2,2,2,2,2,2,2,2,2,2,2,2,2,2,
2,2,2,2,2,2,2,2,2,2,2,2,2,2,2,2,2,2,2,2,2,2,2,2,2,2,2,2,2,2,2,2,2,2,2,2,
2,2,2,2,2,2,2,2,2,2,2,2,2,2,2,2,2,2,2,2,2,2,2,2,2,2,2,2,2,2,2,2,2,2,2,2,
2,2,2,2,2,2,2,2,2,2,2,2,2,2,2,2,2,2,2,2,2,2,2,2,2,2,2,2,2,2,2,2,2,2,2,2,
2,2,2,4),(-9.44801459109388,-9.38140150084239,-9.34815307375884,-9.3397733122265,
-9.33561663537882,-9.33225378008983,-9.32799071259287,-9.31905658329978,
-9.27397782766007,-9.24605993230467,-9.20678224637513,-9.1945529386011,
-9.18766664830278,-9.18168688299225,-9.17426078843188,-9.16261390842311,
-9.08368022309558,-9.05927549305772,-9.04475201202775,-9.03961331655339,
-9.03613604670442,-9.03245759347394,-9.02637064532016,-9.00451019539947,
-8.93588411286869,-8.90434566150039,-8.89466860785615,-8.88831729461598,
-8.88224542535717,-8.8736928858359,-8.85332759114986,-8.78310118949654,
-8.76072151462188,-8.74701110333882,-8.74197976410823,-8.73852235435341,
-8.73480741534788,-8.72855242072028,-8.7046364214805,-8.65755567876359,
-8.62521788113793,-8.60412035295504,-8.59566826595096,-8.58955328469147,
-8.58391982570317,-8.57469917726005,-8.54986049164039,-8.47731845713547,
-8.46014871667201,-8.44873949200216,-8.44404703344266,-8.44064512482223,
-8.43678423638304,-8.43003418547347,-8.39194149309516,-8.33738491019732,
-8.30878024248757,-8.29939356560362,-8.2931015766456,-8.28698928792847,
-8.27820980996388,-8.25642512952648,-8.19370446365244,-8.1585501145342,
-8.14995636697368,-8.14575783055956,-8.14239510702805,-8.13817473266887,
-8.12946754333187,-8.07793054335651,-8.01670043505502,-8.00452596885187,
-7.99765056798857,-7.99166898523602,-7.98422592414056,-7.97252247708097,
-7.8938738263871,-7.86066075349899,-7.85228450469096,-7.8481280819492,-7.8447645565344,
-7.84049944600987,-7.83155709452065,-7.78904103073035,-7.75156723620115,
-7.72734503233419,-7.71006411934689,-7.7022162165618,-7.69619298907036,
-7.68955971441796,-7.67854030273919,-7.62740450201838,-7.59040136208314,
-7.56980758607235,-7.55685046786673,-7.55192439245928,-7.54848575170843,
-7.54473104830477,-7.53829327360408,-7.51155731942445,-7.44749720694638,
-7.41677671628374,-7.407177054837,-7.40084179059471,-7.39476012119845,-7.38615071257267,
-7.36539298548847,-7.3016527453641,-7.26614649689816,-7.2575143071448,-7.25330835823292,
-7.24994567168884,-7.24573282343006,-7.23706475751706,-7.18359426703734,
-7.12419443906607,-7.11204523107344,-7.10517513772245,-7.0991931209321,
-7.09174292611686,-7.08001483595798,-7.00149021910906,-6.96821193010324,
-6.95982827081709,-6.95567044196668,-6.95230699996828,-6.94804354564547,
-6.93910985791524,-6.89721235634368,-6.86145789766708,-6.83588214896809,
-6.81791848298812,-6.80995505538576,-6.80391646931734,-6.79733806475074,
-6.78657801810568,-6.7431633551587,-6.68926937411523,-6.66657169756683,
-6.66060724504058,-6.65695546532664,-6.65350227022196,-6.64831075722368,
-6.63451424289507,-6.57387958106604,-6.54232854957359,-6.52157245422814,
-6.51317015182879,-6.50706337703936,-6.50141822384321,-6.49213377339782,
-6.46678587097665,-6.3948183166293,-6.37769227248631,-6.36630353578805,
-6.361614120516,-6.35821242681708,-6.35434947101118,-6.34759097047796,-6.30851126663551,
-6.25471179875971,-6.23564945629639,-6.22115493142345,-6.21381420632902,
-6.20783850025273,-6.20088439296461,-6.18867362680956,-6.11716012429545,
-6.08701174843069,-6.07039559609442,-6.06500366536181,-6.06147523455011,
-6.05830466409053,-6.05295693064295,-6.03804938684816,-5.97815387171798,
-5.94704609230536,-5.92648511437095,-5.91811172397377,-5.91200976675774,
-5.90635779694922,-5.89703580185859,-5.87137147078792,-5.79975667049674,
-5.78265802182167,-5.77128223173348,-5.76659484406917,-5.76319339893564,
-5.75932931137846,-5.75256588712318,-5.71199701004625,-5.66088844554639,
-5.64119845058641,-5.62634876688777,-5.61894010707252,-5.61296037015986,
-5.60605860238916,-5.59408810099918,-5.5207853909241,-5.49158442404803,
-5.47529285464654,-5.46993787466782,-5.46641704496184,-5.46323965003657,
-5.4578556422307,-5.44267823903434,-5.38295500572268,-5.35195446670996,
-5.33144085523658,-5.32307442667898,-5.31697353927857,-5.31131976938189,
-5.30198826430322,-5.27624267865937,-5.20471613540599,-5.18762418430387,
-5.17625150321997,-5.17156455165107,-5.16816311014979,-5.16429866479983,
-5.15753386009215,-5.11662493523327,-5.06421146559669,-5.04538448250777,
-5.03102419215982,-5.02370920671893,-5.01773455639421,-5.01075913091909,
-4.99845089379714,-4.92769225407288,-4.8971317583695,-4.88037652093655,
-4.87496884510086,-4.87143705739459,-4.86826914425481,-4.86293608995139,
-4.84813733285144,-4.77216866854091,-4.73955944340199,-4.72978541974077,
-4.72341409763979,-4.71728508030098,-4.70875355879654,-4.68710543773134,
-4.65347547499122,-4.60315876849961,-4.58379643505322,-4.57793785359249,
-4.57430924445518,-4.57079841284659,-4.56549110081198,-4.54960587936143,
-4.52155682535197,-4.45132434035121,-4.4363506246857,-4.42891887753103,
-4.4229380604913,-4.4160543904857,-4.40384010853783,-4.36467212114955,-4.33757975952056,
-4.29152906339711,-4.28263734796421,-4.27838200487283,-4.27501897262567,
-4.27085422934785,-4.26243422825157,-4.22883404607388,-4.15087278503415,
-4.13902768490065,-4.13154376510978,-4.12555963179594,-4.11871426639979,
-4.1066821864288,-4.05578402163054,-4.0009557887622,-3.9873789719632,-3.98222032925095,
-3.97877386492966,-3.97511298574257,-3.96910482641362,-3.94582884713075,
-3.88872202696743,-3.848807165819,-3.83822590455367,-3.83168611880757,-3.82563652149612,
-3.81758907639446,-3.79910978651272,-3.77248623293831,-3.73750593573787,
-3.69336144107036,-3.68655143702741,-3.68267747448146,-3.67927966221325,
-3.67461386659972,-3.66336877846622,-3.6465415708106,-3.57824420478216,
-3.54951724535958,-3.53986461136127,-3.53351924490027,-3.52737604181771,
-3.5187592475767,-3.4964954449991,-3.46136771442216,-3.40722855515764,-3.39283293567694,
-3.38755669924319,-3.38439992223998,-3.38085669982481,-3.37539096646288,
-3.35809885988307,-3.32589683547393,-3.25803333672706,-3.24650315445813,
-3.23911162051876,-3.23313458114653,-3.22622357528891,-3.21387288832576,
-3.17374093045621,-3.14625463864198,-3.10190993516612,-3.09296845260623,
-3.08870425603886,-3.08534170708683,-3.08118683093758,-3.07281463652837,
-3.0396247106185,-2.96091840573627,-2.94922660990018,-2.94178820740471,
-2.93580862945455,-2.92893362897039,-2.91675458596445,-2.87781625765677,
-2.85362489022765,-2.80429910656731,-2.79548804678734,-2.791248784751,-2.7878870466656,
-2.78370969121696,-2.77522088521722,-2.74099827724974,-2.68093558388414,
-2.65633628424758,-2.64714864811203,-2.64152244101963,-2.63540537762009,
-2.62693187525845,-2.60567330503028,-2.57295712586263,-2.52488226036302,
-2.5024526591567,-2.49630814054109,-2.49261812789441,-2.48914957546455,
-2.48405241078808,-2.46984039298301,-2.44621771852627,-2.36533814786787,
-2.35300527788872,-2.34602679532548,-2.34005569729569,-2.33275281606529,
-2.31844241759414,-2.29970098142884,-2.24773828191848,-2.20634305381292,
-2.19958037884252,-2.1957176834768,-2.1923182087446,-2.18763450888408,-2.17627250123387,
-2.15919774392155,-2.08786671937614,-2.06196055820317,-2.05261416807905,
-2.0469599235255,-2.04086504318408,-2.03251865515358,-2.0121182842402,-1.9813665842259,
-1.92209006676937,-1.90635033768349,-1.90089509969131,-1.89770548156087,
-1.89420153180413,-1.88892224122803,-1.87325821023931,-1.84581628823902,
-1.7779310930747,-1.76088496037318,-1.75316391812636,-1.74714289100281,
-1.74051779870824,-1.72952574448648,-1.67165027446578,-1.6141137366604,
-1.60578913268532,-1.6016441560872,-1.59828212067461,-1.59400905741946,
-1.58501730969047,-1.54605340165214,-1.47257568502694,-1.46063697916326,
-1.45374472712599,-1.44776810455151,-1.44035666446211,-1.42547761252992,
-1.36383569034388,-1.31769839126718,-1.30876141342307,-1.30449875439695,
-1.30113711310382,-1.29698298072558,-1.28861115290025,-1.25541379557153,
-1.17675951780695,-1.16506465118156,-1.15762642659685,-1.15164831619072,
-1.1447764563489,-1.13260695447519,-1.07114764691721,-1.01998875394796,
-1.01126783577167,-1.00704633184975,-1.00368552697631,-0.999492905686176,
-0.990922316997083,-0.95595380282485,-0.893758691458273,-0.871447710955773,
-0.862589745951792,-0.856465552584371,-0.850196610590019,-0.840912099766564,
-0.813222167364056,-0.762074718227652,-0.719620316011767,-0.712849558430266,
-0.708985404786666,-0.705586979035008,-0.700907877600257,-0.689571979762603,
-0.672551191841519,-0.601874583043717,-0.575384033983162,-0.565975182833617,
-0.559681425272963,-0.553505877243141,-0.544701971239021,-0.521027315710591,
-0.482266905632647,-0.424787365560533,-0.41646037122685,-0.412315325640752,
-0.408953848625948,-0.404682273267573,-0.395696257012272,-0.356781239752759,
-0.283234093652927,-0.271314841183368,-0.26442753019634,-0.258451515623989,
-0.251036066172714,-0.23613196988513,-0.174482232466516,-0.128424436005239,
-0.11948157411596,-0.115218218598217,-0.111857080207177,-0.107704873064183,
-0.0993408300310918,-0.0662049594753124,-1.00000004543688E-6),
 .UNSPECIFIED.);
#371=B_SPLINE_CURVE_WITH_KNOTS('',3,(#33070,#33071,#33072,#33073,#33074,
#33075,#33076,#33077,#33078,#33079,#33080,#33081,#33082,#33083,#33084,#33085,
#33086,#33087,#33088,#33089,#33090,#33091,#33092,#33093,#33094,#33095,#33096,
#33097,#33098,#33099,#33100,#33101,#33102,#33103,#33104,#33105,#33106,#33107,
#33108,#33109,#33110,#33111,#33112,#33113,#33114,#33115,#33116,#33117,#33118,
#33119,#33120,#33121,#33122,#33123,#33124,#33125,#33126,#33127,#33128,#33129,
#33130,#33131,#33132,#33133,#33134,#33135,#33136,#33137,#33138,#33139,#33140,
#33141,#33142,#33143,#33144,#33145,#33146,#33147,#33148,#33149,#33150,#33151,
#33152,#33153,#33154,#33155,#33156,#33157,#33158,#33159,#33160,#33161,#33162,
#33163,#33164,#33165,#33166,#33167,#33168,#33169,#33170,#33171,#33172,#33173,
#33174,#33175,#33176,#33177,#33178,#33179,#33180,#33181,#33182,#33183,#33184,
#33185,#33186,#33187,#33188,#33189,#33190,#33191,#33192,#33193,#33194,#33195,
#33196,#33197,#33198,#33199,#33200,#33201,#33202,#33203,#33204,#33205,#33206,
#33207,#33208,#33209,#33210,#33211,#33212,#33213,#33214,#33215,#33216,#33217,
#33218,#33219,#33220,#33221,#33222,#33223,#33224,#33225,#33226,#33227,#33228,
#33229,#33230,#33231,#33232,#33233,#33234,#33235,#33236,#33237,#33238,#33239,
#33240,#33241,#33242,#33243,#33244,#33245,#33246,#33247,#33248,#33249,#33250,
#33251,#33252,#33253,#33254,#33255,#33256,#33257,#33258,#33259,#33260,#33261,
#33262,#33263,#33264,#33265,#33266,#33267,#33268,#33269,#33270,#33271,#33272,
#33273,#33274,#33275,#33276,#33277,#33278,#33279,#33280,#33281,#33282,#33283,
#33284,#33285,#33286,#33287,#33288,#33289,#33290,#33291,#33292,#33293,#33294,
#33295,#33296,#33297,#33298,#33299,#33300,#33301,#33302,#33303,#33304,#33305,
#33306,#33307,#33308,#33309,#33310,#33311,#33312,#33313,#33314,#33315,#33316,
#33317,#33318,#33319,#33320,#33321,#33322,#33323,#33324,#33325,#33326,#33327,
#33328,#33329,#33330,#33331,#33332,#33333,#33334,#33335,#33336,#33337,#33338,
#33339,#33340,#33341,#33342,#33343,#33344,#33345,#33346,#33347,#33348,#33349,
#33350,#33351,#33352,#33353,#33354,#33355,#33356,#33357,#33358,#33359,#33360,
#33361,#33362,#33363,#33364,#33365,#33366,#33367,#33368,#33369,#33370,#33371,
#33372,#33373,#33374,#33375,#33376,#33377,#33378,#33379,#33380,#33381,#33382,
#33383,#33384,#33385,#33386,#33387,#33388,#33389,#33390,#33391,#33392,#33393,
#33394,#33395,#33396,#33397,#33398,#33399,#33400,#33401,#33402,#33403,#33404,
#33405,#33406,#33407,#33408,#33409,#33410,#33411,#33412,#33413,#33414,#33415,
#33416,#33417,#33418,#33419,#33420,#33421,#33422,#33423,#33424,#33425,#33426,
#33427,#33428,#33429,#33430,#33431,#33432,#33433,#33434,#33435,#33436,#33437,
#33438,#33439,#33440,#33441,#33442,#33443,#33444,#33445,#33446,#33447,#33448,
#33449,#33450,#33451,#33452,#33453,#33454,#33455,#33456,#33457,#33458,#33459,
#33460,#33461,#33462,#33463,#33464,#33465,#33466,#33467,#33468,#33469,#33470,
#33471,#33472,#33473,#33474,#33475,#33476,#33477,#33478,#33479,#33480,#33481,
#33482,#33483,#33484,#33485,#33486,#33487,#33488,#33489,#33490,#33491,#33492,
#33493,#33494,#33495,#33496,#33497,#33498,#33499,#33500,#33501,#33502,#33503,
#33504,#33505,#33506,#33507,#33508,#33509,#33510,#33511,#33512,#33513,#33514,
#33515,#33516,#33517,#33518,#33519,#33520,#33521,#33522,#33523,#33524,#33525,
#33526,#33527,#33528,#33529,#33530,#33531,#33532,#33533,#33534,#33535,#33536,
#33537,#33538,#33539,#33540,#33541,#33542,#33543,#33544,#33545,#33546,#33547,
#33548,#33549,#33550,#33551,#33552,#33553,#33554,#33555,#33556,#33557,#33558,
#33559,#33560,#33561,#33562,#33563,#33564,#33565,#33566,#33567,#33568,#33569,
#33570,#33571,#33572,#33573,#33574,#33575,#33576,#33577,#33578,#33579,#33580,
#33581,#33582,#33583,#33584,#33585,#33586,#33587,#33588,#33589,#33590,#33591,
#33592,#33593,#33594,#33595,#33596,#33597,#33598,#33599,#33600,#33601,#33602,
#33603,#33604,#33605,#33606,#33607,#33608,#33609,#33610,#33611,#33612,#33613,
#33614,#33615,#33616,#33617,#33618,#33619,#33620,#33621,#33622,#33623,#33624,
#33625,#33626,#33627,#33628,#33629,#33630,#33631,#33632,#33633,#33634,#33635,
#33636,#33637,#33638,#33639,#33640,#33641,#33642,#33643,#33644,#33645),
 .UNSPECIFIED.,.F.,.F.,(4,2,2,2,2,2,2,2,2,2,2,2,2,2,2,2,2,2,2,2,2,2,2,2,
2,2,2,2,2,2,2,2,2,2,2,2,2,2,2,2,2,2,2,2,2,2,2,2,2,2,2,2,2,2,2,2,2,2,2,2,
2,2,2,2,2,2,2,2,2,2,2,2,2,2,2,2,2,2,2,2,2,2,2,2,2,2,2,2,2,2,2,2,2,2,2,2,
2,2,2,2,2,2,2,2,2,2,2,2,2,2,2,2,2,2,2,2,2,2,2,2,2,2,2,2,2,2,2,2,2,2,2,2,
2,2,2,2,2,2,2,2,2,2,2,2,2,2,2,2,2,2,2,2,2,2,2,2,2,2,2,2,2,2,2,2,2,2,2,2,
2,2,2,2,2,2,2,2,2,2,2,2,2,2,2,2,2,2,2,2,2,2,2,2,2,2,2,2,2,2,2,2,2,2,2,2,
2,2,2,2,2,2,2,2,2,2,2,2,2,2,2,2,2,2,2,2,2,2,2,2,2,2,2,2,2,2,2,2,2,2,2,2,
2,2,2,2,2,2,2,2,2,2,2,2,2,2,2,2,2,2,2,2,2,2,2,2,2,2,2,2,2,2,2,2,2,2,2,2,
2,2,2,2,2,2,2,2,2,2,2,4),(-5.66646737981884,-5.65202977713212,-5.64186283566428,
-5.6359415669808,-5.63021907568959,-5.62376470462157,-5.61358008762193,
-5.57889180222527,-5.53149386455273,-5.49696145083533,-5.48843911991611,
-5.48425585305101,-5.48089499215497,-5.47666391120387,-5.46789271648334,
-5.40071699055294,-5.36867042049385,-5.35436837701679,-5.34272537785606,
-5.33596359162933,-5.32997169531042,-5.32236912659647,-5.30645781792764,
-5.23737450623877,-5.20962989004014,-5.19385681219652,-5.18856501589677,
-5.18505883604978,-5.18142915713168,-5.17555884877083,-5.15604763182971,
-5.10584972629597,-5.05770159356469,-5.04570812516265,-5.03887299604999,
-5.03289112831685,-5.02540121392049,-5.01352848728401,-4.93581849064049,
-4.90215156296082,-4.89372632866156,-4.88956187527887,-4.88620063551178,
-4.88194951375378,-4.87307306320735,-4.82732692448115,-4.76865376762382,
-4.75148127709024,-4.74365512824748,-4.7376378501395,-4.7310003805168,-4.71994818150542,
-4.66852054851719,-4.62951266769257,-4.60129393389863,-4.59496694222568,
-4.59123769438089,-4.58782991164676,-4.58287706441957,-4.57060557609999,
-4.49173904485678,-4.45880225807595,-4.4490043152033,-4.44263106136734,
-4.43657894815234,-4.42812272961005,-4.40854861920622,-4.34375606864796,
-4.3171441661649,-4.3017844048574,-4.29654263789846,-4.29304665804954,-4.28940312240255,
-4.28346862934879,-4.2632572406141,-4.21356705024614,-4.18019709557297,
-4.15866449038775,-4.1501530995515,-4.14403081341646,-4.13841492595579,
-4.12927853651629,-4.105048167129,-4.04470564634612,-4.01039232827666,-4.00189477852074,
-3.99771651043792,-3.99435584991646,-3.99012021837193,-3.98132408175168,
-3.93236341124116,-3.90780092781493,-3.86883939843769,-3.85665929536066,
-3.84978546886808,-3.8438079346922,-3.83637340405622,-3.82469047681393,
-3.74602367273248,-3.71286593163613,-3.70449890384632,-3.7003458793686,
-3.6969844451918,-3.69272116041021,-3.68377997677606,-3.63958240022835,
-3.61099131413731,-3.57161724800104,-3.55937711275923,-3.55249046722558,
-3.54651358177317,-3.53909517356085,-3.52746858691514,-3.46075734008769,
-3.42793202837417,-3.41044307007549,-3.40495753887804,-3.40141093651012,
-3.39782991781627,-3.39218425006672,-3.37486457910174,-3.32303508073422,
-3.27388779954679,-3.26188137024388,-3.25504329110571,-3.24906137798557,
-3.24157475642982,-3.22971416504789,-3.15193394422553,-3.11830012773706,
-3.10987838530369,-3.10571446866184,-3.10235302329738,-3.09810083708849,
-3.0892195203075,-3.04360493844914,-3.01611590134675,-2.97690950322173,
-2.96469296457642,-2.95781087128827,-2.95183304806881,-2.94440712878804,
-2.93275592223282,-2.86631148295166,-2.83332018801372,-2.81607802899908,
-2.81044092814242,-2.80686153952506,-2.80331280572969,-2.79781822596739,
-2.78024850318555,-2.74716874247503,-2.68081763348978,-2.66915417275877,
-2.66172465481073,-2.65574652332987,-2.64886692294768,-2.63666254398883,
-2.59754205880952,-2.57075519925782,-2.52445043598243,-2.51552795985129,
-2.51126801152629,-2.50790643096073,-2.50374980368802,-2.49536513270769,
-2.46205548825634,-2.38361345270778,-2.3718762018619,-2.36442564117767,
-2.35844667999993,-2.35158376546011,-2.33945718311512,-2.28112314814783,
-2.2264133737659,-2.21791643273439,-2.21373809305878,-2.21037718609596,
-2.20614101973642,-2.19734305020684,-2.16025938582741,-2.09180103555146,
-2.07549855963712,-2.06779734707669,-2.06177949523892,-2.05514532955771,
-2.04410809581025,-1.98138814047806,-1.9293277717213,-1.92066600566779,
-1.91645582238859,-1.9130949300682,-1.90889077078366,-1.90026122274774,
-1.864755527422,-1.8010049854682,-1.78027906862233,-1.771677803246,-1.76560001299892,
-1.75926718237016,-1.74966792492346,-1.71891115046681,-1.65458661134996,
-1.6282223013374,-1.62182239498349,-1.61807726106605,-1.61463777152781,
-1.60969654482994,-1.59661815542594,-1.5757343467791,-1.53698251164871,
-1.48783016228087,-1.47694154571141,-1.4703389921685,-1.46431314773228,
-1.45641757833719,-1.43883650201319,-1.41401970757328,-1.37742348212445,
-1.33519137293408,-1.3262593361143,-1.32199806356053,-1.31863701205398,
-1.31448306084595,-1.3061102584762,-1.27290050023367,-1.19425650838086,
-1.18255727453901,-1.17511799410073,-1.16914012739284,-1.16226975073057,
-1.15010615416118,-1.0889964529071,-1.0374599219333,-1.02876365735641,-1.02454670641525,
-1.02118490981561,-1.01698498194405,-1.00838295483133,-0.973138996154328,
-0.910123507190809,-0.888702629059718,-0.87998229198576,-0.873881985281281,
-0.867577729458823,-0.858124455948534,-0.828856995839813,-0.778117056820806,
-0.73717460449203,-0.730414977910018,-0.726553195954124,-0.723156579384028,
-0.718477799940821,-0.707126939379542,-0.690070821879275,-0.61894076230909,
-0.592827418822905,-0.583463979045129,-0.57781088894916,-0.571726063796511,
-0.563409669675828,-0.543173184478235,-0.512778117269808,-0.45405516887641,
-0.437429715620349,-0.431868024820915,-0.428660041397706,-0.425178111955145,
-0.420003204802352,-0.405176509138087,-0.379981617743587,-0.320372090636363,
-0.295214332417875,-0.285954937889434,-0.280315707830894,-0.274208218380575,
-0.265791727463636,-0.244923838854528,-0.213104029072987,-0.145572678770187,
-0.136883779871564,-0.132665685856985,-0.129296100761455,-0.1250762439012,
-0.116413307166631,-0.0806871329657728,-0.0158458709233213,-1.00000000013978E-6),
 .UNSPECIFIED.);
#372=B_SPLINE_CURVE_WITH_KNOTS('',3,(#33646,#33647,#33648,#33649,#33650,
#33651,#33652,#33653,#33654,#33655,#33656,#33657,#33658,#33659,#33660,#33661,
#33662,#33663,#33664,#33665,#33666,#33667,#33668,#33669,#33670,#33671,#33672,
#33673,#33674,#33675,#33676,#33677,#33678,#33679,#33680,#33681,#33682,#33683,
#33684,#33685,#33686,#33687,#33688,#33689,#33690,#33691,#33692,#33693,#33694,
#33695,#33696,#33697,#33698,#33699,#33700,#33701,#33702,#33703,#33704,#33705,
#33706,#33707,#33708,#33709,#33710,#33711,#33712,#33713,#33714,#33715,#33716,
#33717,#33718,#33719,#33720,#33721,#33722,#33723,#33724,#33725,#33726,#33727,
#33728,#33729,#33730,#33731,#33732,#33733,#33734,#33735,#33736,#33737,#33738,
#33739,#33740,#33741,#33742,#33743,#33744,#33745,#33746,#33747,#33748,#33749,
#33750,#33751,#33752,#33753,#33754,#33755,#33756,#33757,#33758,#33759,#33760,
#33761,#33762,#33763,#33764,#33765,#33766,#33767,#33768,#33769,#33770,#33771,
#33772,#33773,#33774,#33775),.UNSPECIFIED.,.F.,.F.,(4,2,2,2,2,2,2,2,2,2,
2,2,2,2,2,2,2,2,2,2,2,2,2,2,2,2,2,2,2,2,2,2,2,2,2,2,2,2,2,2,2,2,2,2,2,2,
2,2,2,2,2,2,2,2,2,2,2,2,2,2,2,2,2,2,4),(1.24528113121354E-5,0.028631889083293,
0.0408247356106915,0.045280590035446,0.0485000424796718,0.0517866681795052,
0.0554902755365286,0.0618059384212369,0.0872969915363886,0.130173433480661,
0.162959191226469,0.186192291234085,0.194967556390622,0.201162746958399,
0.206769526698791,0.214297686819927,0.23314806277008,0.296603596769671,
0.331602370103769,0.340207789039151,0.344448021752713,0.347842071702048,
0.352102503717678,0.361032071767464,0.402285316490655,0.437722675474088,
0.463551666330535,0.481609663048884,0.489560110176308,0.495567551977114,
0.502090489839575,0.512706981711773,0.553638735569381,0.608443290521791,
0.633037596026065,0.639303211024447,0.642998592011321,0.646394118103218,
0.651286079343969,0.664335427032788,0.68523798828632,0.723801928508903,
0.773358298195291,0.784093381456232,0.790593287408483,0.796516211751473,
0.804259439528729,0.821393069658049,0.845417609013507,0.883337362202561,
0.888393239049124,0.929780685976583,0.936478787684859,0.940286064788971,
0.943639514542793,0.94823764090924,0.959235542588296,1.01763285273625,1.04597037320218,
1.07375399933964,1.08324582206853,1.08952307352542,1.09514563179514,1.10081989957959,
1.10723007897768),.UNSPECIFIED.);
#373=B_SPLINE_CURVE_WITH_KNOTS('',3,(#33999,#34000,#34001,#34002,#34003,
#34004,#34005),.UNSPECIFIED.,.F.,.F.,(4,1,1,1,4),(0.000143951182684975,
0.249992846908436,0.499984711894009,0.749976576879583,0.999370396581308),
 .UNSPECIFIED.);
#374=B_SPLINE_CURVE_WITH_KNOTS('',3,(#34006,#34007,#34008,#34009,#34010,
#34011,#34012,#34013,#34014,#34015,#34016,#34017,#34018,#34019,#34020,#34021,
#34022,#34023,#34024,#34025,#34026,#34027,#34028,#34029,#34030,#34031,#34032,
#34033,#34034,#34035,#34036,#34037,#34038,#34039,#34040,#34041,#34042,#34043,
#34044,#34045,#34046,#34047,#34048,#34049,#34050,#34051,#34052,#34053,#34054,
#34055,#34056,#34057,#34058,#34059,#34060,#34061,#34062,#34063,#34064,#34065,
#34066,#34067,#34068,#34069,#34070,#34071,#34072,#34073,#34074,#34075,#34076,
#34077,#34078,#34079,#34080,#34081,#34082,#34083,#34084,#34085,#34086,#34087,
#34088,#34089,#34090,#34091,#34092,#34093,#34094,#34095,#34096,#34097,#34098,
#34099,#34100,#34101,#34102,#34103,#34104,#34105,#34106,#34107,#34108,#34109,
#34110,#34111,#34112,#34113,#34114,#34115,#34116,#34117,#34118,#34119,#34120,
#34121,#34122,#34123,#34124,#34125,#34126,#34127,#34128,#34129,#34130,#34131,
#34132,#34133,#34134,#34135,#34136,#34137,#34138,#34139,#34140,#34141,#34142,
#34143,#34144,#34145,#34146,#34147,#34148,#34149,#34150,#34151,#34152,#34153,
#34154,#34155,#34156,#34157,#34158,#34159,#34160,#34161,#34162,#34163,#34164,
#34165,#34166,#34167,#34168,#34169,#34170,#34171),.UNSPECIFIED.,.F.,.F.,
(4,2,2,2,2,2,2,2,2,2,2,2,2,2,2,2,2,2,2,2,2,2,2,2,2,2,2,2,2,2,2,2,2,2,2,
2,2,2,2,2,2,2,2,2,2,2,2,2,2,2,2,2,2,2,2,2,2,2,2,2,2,2,2,2,2,2,2,2,2,2,2,
2,2,2,2,2,2,2,2,2,2,2,4),(-4.85680415953354,-4.8501799720293,-4.82795587041218,
-4.79832010131199,-4.79124321059898,-4.78658794634873,-4.78206143088215,
-4.77542775596836,-4.75470353170186,-4.72943885798795,-4.7176911448229,
-4.71386627329548,-4.71128726556225,-4.70844794529031,-4.703223995751,-4.68410777517529,
-4.65940719494081,-4.64497557392077,-4.63909845834549,-4.63468350385385,
-4.62984784705791,-4.62168669624962,-4.5857391656108,-4.56605598267604,
-4.56177473355638,-4.55914552997483,-4.55652816323524,-4.5522510195785,
-4.53233977338937,-4.50683526203999,-4.49217064740255,-4.48629976032288,
-4.48192574037172,-4.47717271006402,-4.46925412267292,-4.43307835023872,
-4.4147776420783,-4.40968935067262,-4.40690608234038,-4.40442240623259,
-4.40074367439207,-4.39073777460239,-4.35658262888147,-4.33992777921667,
-4.3337911590246,-4.32934665053616,-4.32463014308964,-4.31703043657081,
-4.28065221276563,-4.26238805368253,-4.25728583749115,-4.25448116258635,
-4.25198471393949,-4.2482683555091,-4.23797743673025,-4.20417495177972,
-4.18759984766012,-4.18147950515469,-4.17704430402583,-4.17233613208709,
-4.16474903166549,-4.12527279211248,-4.10808704674472,-4.10391636238359,
-4.10131284399107,-4.09898506640493,-4.09491271650107,-4.08077476576487,
-4.05062559648586,-4.03477044416374,-4.02873478569039,-4.02431666336258,
-4.01958664091511,-4.01187134965379,-3.9803940400591,-3.95594501702431,
-3.95155457371567,-3.94890593978513,-3.94629702828529,-3.94210273808332,
-3.92554506752803,-3.89743871250035,-3.88535150283469),.UNSPECIFIED.);
#375=B_SPLINE_CURVE_WITH_KNOTS('',3,(#34389,#34390,#34391,#34392,#34393,
#34394,#34395,#34396,#34397,#34398,#34399,#34400,#34401,#34402,#34403,#34404,
#34405,#34406,#34407,#34408,#34409,#34410,#34411,#34412,#34413,#34414,#34415,
#34416,#34417,#34418,#34419,#34420,#34421,#34422,#34423,#34424,#34425,#34426,
#34427,#34428,#34429,#34430,#34431,#34432,#34433,#34434,#34435,#34436,#34437,
#34438,#34439,#34440,#34441,#34442,#34443,#34444,#34445,#34446,#34447,#34448,
#34449,#34450,#34451,#34452,#34453,#34454,#34455,#34456,#34457,#34458,#34459,
#34460,#34461,#34462,#34463,#34464,#34465,#34466,#34467,#34468,#34469,#34470,
#34471,#34472,#34473,#34474,#34475,#34476,#34477,#34478,#34479,#34480,#34481,
#34482,#34483,#34484,#34485,#34486,#34487,#34488,#34489,#34490,#34491,#34492,
#34493,#34494,#34495,#34496,#34497,#34498,#34499,#34500,#34501,#34502,#34503,
#34504,#34505,#34506,#34507,#34508,#34509,#34510,#34511,#34512,#34513,#34514,
#34515,#34516,#34517,#34518,#34519,#34520,#34521,#34522,#34523,#34524,#34525,
#34526,#34527,#34528,#34529,#34530,#34531,#34532,#34533,#34534,#34535,#34536,
#34537,#34538,#34539,#34540,#34541,#34542,#34543,#34544,#34545,#34546,#34547,
#34548,#34549,#34550,#34551,#34552,#34553,#34554,#34555,#34556,#34557,#34558,
#34559,#34560,#34561,#34562,#34563,#34564),.UNSPECIFIED.,.F.,.F.,(4,2,2,
2,2,2,2,2,2,2,2,2,2,2,2,2,2,2,2,2,2,2,2,2,2,2,2,2,2,2,2,2,2,2,2,2,2,2,2,
2,2,2,2,2,2,2,2,2,2,2,2,2,2,2,2,2,2,2,2,2,2,2,2,2,2,2,2,2,2,2,2,2,2,2,2,
2,2,2,2,2,2,2,2,2,2,2,2,4),(0.000139559779193673,0.00418312955586237,0.00978488685190961,
0.0413781338730359,0.0574037092840092,0.0666164948624175,0.0700458250993038,
0.0724637085699126,0.0752465177003127,0.08037206612107,0.100124782142703,
0.124948084354604,0.13939323491165,0.145150543418712,0.149416608566436,
0.154022811938123,0.161603791189514,0.199956422345138,0.218677502217384,
0.222845565440813,0.225396316072621,0.227925417719586,0.231996183820311,
0.247481281138077,0.276999600765713,0.29269249409177,0.298599224334203,
0.302884034373717,0.307426724561561,0.31470887053306,0.349892125706388,
0.365065477915852,0.373976686412166,0.377357746153798,0.379762464599789,
0.382557255377237,0.387747460835412,0.408650817284414,0.427703933187463,
0.445734894405103,0.451892404985478,0.456223250300085,0.460169759950361,
0.46662169681185,0.485760179307897,0.503808128813803,0.524013803822886,
0.529158800802302,0.531944757206762,0.534354258517986,0.537758757349042,
0.546831252763403,0.562453735156471,0.596693913331176,0.604091487611082,
0.608659888223021,0.612938810495531,0.618789244053598,0.63398213803354,
0.661455620923727,0.679437337704363,0.683625524980089,0.686180651837019,
0.688707737771483,0.692763739718316,0.709135302875068,0.743836215926229,
0.755132396510595,0.760426365199457,0.764637484032459,0.769486109674433,
0.778300983637962,0.801020550619598,0.830599067149249,0.836196045961441,
0.839039940921639,0.841195115832224,0.844336540072541,0.851610758378909,
0.862698005023155,0.897182523982601,0.908660285201998,0.91398456758211,
0.918198714606633,0.923028089704658,0.931740813946652,0.956469632034719,
0.971411654023308),.UNSPECIFIED.);
#376=B_SPLINE_CURVE_WITH_KNOTS('',3,(#34565,#34566,#34567,#34568),
 .UNSPECIFIED.,.F.,.F.,(4,4),(0.537782073242468,0.537816282017176),
 .UNSPECIFIED.);
#377=B_SPLINE_CURVE_WITH_KNOTS('',3,(#34569,#34570,#34571,#34572,#34573,
#34574,#34575,#34576,#34577,#34578,#34579,#34580,#34581,#34582,#34583,#34584,
#34585,#34586,#34587),.UNSPECIFIED.,.F.,.F.,(4,3,3,3,3,3,4),(0.,0.321652726498616,
0.335818547580298,0.5,0.813168066582452,0.83581854758052,1.),
 .UNSPECIFIED.);
#378=B_SPLINE_CURVE_WITH_KNOTS('',3,(#34600,#34601,#34602,#34603,#34604,
#34605,#34606),.UNSPECIFIED.,.F.,.F.,(4,3,4),(8.942092232521E-7,0.897079636775044,
1.),.UNSPECIFIED.);
#379=B_SPLINE_CURVE_WITH_KNOTS('',3,(#34629,#34630,#34631,#34632,#34633,
#34634,#34635),.UNSPECIFIED.,.F.,.F.,(4,3,4),(0.000178264861484437,0.742416332780832,
0.999844713842845),.UNSPECIFIED.);
#380=B_SPLINE_CURVE_WITH_KNOTS('',3,(#34637,#34638,#34639,#34640,#34641,
#34642,#34643,#34644,#34645,#34646),.UNSPECIFIED.,.F.,.F.,(4,3,3,4),(0.,
0.519872273097902,0.615160302254839,1.),.UNSPECIFIED.);
#381=B_SPLINE_CURVE_WITH_KNOTS('',3,(#34667,#34668,#34669,#34670,#34671,
#34672,#34673,#34674,#34675,#34676),.UNSPECIFIED.,.F.,.F.,(4,2,2,2,4),(3.67941030579461E-9,
0.326260440009545,0.5,0.826260436373397,1.),.UNSPECIFIED.);
#382=B_SPLINE_CURVE_WITH_KNOTS('',3,(#34679,#34680,#34681,#34682,#34683,
#34684,#34685,#34686,#34687,#34688,#34689,#34690,#34691,#34692),
 .UNSPECIFIED.,.F.,.F.,(4,2,2,2,2,2,4),(-0.224981239925635,-0.193512649663793,
-0.161961102829213,-0.112487004321429,-0.062975091378892,-0.0314451815916685,
-1.40071649520604E-6),.UNSPECIFIED.);
#383=B_SPLINE_CURVE_WITH_KNOTS('',3,(#34713,#34714,#34715,#34716,#34717,
#34718,#34719,#34720,#34721,#34722,#34723,#34724,#34725),.UNSPECIFIED.,
 .F.,.F.,(4,3,3,3,4),(1.02472631714155E-12,0.387568508029344,0.49999981776731,
0.887555122346297,0.999873703557718),.UNSPECIFIED.);
#384=B_SPLINE_CURVE_WITH_KNOTS('',3,(#34727,#34728,#34729,#34730,#34731,
#34732,#34733,#34734,#34735,#34736),.UNSPECIFIED.,.F.,.F.,(4,2,2,2,4),(2.94135345515086E-12,
0.448076600669202,0.5,0.948076600665885,0.999999999999085),
 .UNSPECIFIED.);
#385=B_SPLINE_CURVE_WITH_KNOTS('',3,(#34757,#34758,#34759,#34760,#34761,
#34762),.UNSPECIFIED.,.F.,.F.,(4,2,4),(9.99999979321194E-7,0.0329350911858533,
0.0651002228197631),.UNSPECIFIED.);
#630=CONICAL_SURFACE('',#10537,0.0032,0.785398163397449);
#631=CONICAL_SURFACE('',#10542,0.0032,0.785398163397448);
#632=CONICAL_SURFACE('',#10543,0.0016,0.785398163397449);
#633=CONICAL_SURFACE('',#10544,0.0031,0.785398163397449);
#634=CONICAL_SURFACE('',#10547,0.0016,0.785398163397449);
#635=CONICAL_SURFACE('',#10556,0.00175,0.785398163397448);
#636=CONICAL_SURFACE('',#10561,0.00175,0.785398163397449);
#637=CONICAL_SURFACE('',#10585,0.0031,0.785398163397448);
#638=CONICAL_SURFACE('',#10592,0.0016,0.785398163397448);
#677=(
BOUNDED_CURVE()
B_SPLINE_CURVE(2,(#27879,#27880,#27881),.UNSPECIFIED.,.F.,.F.)
B_SPLINE_CURVE_WITH_KNOTS((3,3),(1.09880286001687,1.11425993114071),
 .UNSPECIFIED.)
CURVE()
GEOMETRIC_REPRESENTATION_ITEM()
RATIONAL_B_SPLINE_CURVE((1.37837837838126,1.31211005581294,1.24390243902605))
REPRESENTATION_ITEM('')
);
#678=(
BOUNDED_CURVE()
B_SPLINE_CURVE(2,(#27888,#27889,#27890),.UNSPECIFIED.,.F.,.F.)
B_SPLINE_CURVE_WITH_KNOTS((3,3),(0.0269674782770168,0.0424245494010484),
 .UNSPECIFIED.)
CURVE()
GEOMETRIC_REPRESENTATION_ITEM()
RATIONAL_B_SPLINE_CURVE((1.24390243902529,1.31211005581301,1.37837837838213))
REPRESENTATION_ITEM('')
);
#679=(
BOUNDED_CURVE()
B_SPLINE_CURVE(2,(#27949,#27950,#27951),.UNSPECIFIED.,.F.,.F.)
B_SPLINE_CURVE_WITH_KNOTS((3,3),(0.0269674782769955,0.0424245494010537),
 .UNSPECIFIED.)
CURVE()
GEOMETRIC_REPRESENTATION_ITEM()
RATIONAL_B_SPLINE_CURVE((1.2439024390251,1.31211005581295,1.37837837838218))
REPRESENTATION_ITEM('')
);
#680=(
BOUNDED_CURVE()
B_SPLINE_CURVE(2,(#27969,#27970,#27971),.UNSPECIFIED.,.F.,.F.)
B_SPLINE_CURVE_WITH_KNOTS((3,3),(1.09880286001689,1.11425993114073),
 .UNSPECIFIED.)
CURVE()
GEOMETRIC_REPRESENTATION_ITEM()
RATIONAL_B_SPLINE_CURVE((1.37837837838082,1.3121100558125,1.24390243902561))
REPRESENTATION_ITEM('')
);
#705=ELLIPSE('',#10579,0.00198146070825073,0.00138139923663895);
#706=ELLIPSE('',#10580,0.00189052267529393,0.00133517872970212);
#707=ELLIPSE('',#10581,0.00182395398435439,0.00131739606577714);
#708=ELLIPSE('',#10582,0.0020993200218241,0.00147094440040091);
#709=ELLIPSE('',#10600,0.00132114477356862,0.00112846649906451);
#741=FACE_BOUND('',#1894,.T.);
#742=FACE_BOUND('',#1897,.T.);
#743=FACE_BOUND('',#1898,.T.);
#744=FACE_BOUND('',#1917,.T.);
#745=FACE_BOUND('',#1931,.T.);
#746=FACE_BOUND('',#1932,.T.);
#747=FACE_BOUND('',#1939,.T.);
#789=SHAPE_REPRESENTATION_RELATIONSHIP('SRR','None',#50157,#809);
#809=ADVANCED_BREP_SHAPE_REPRESENTATION('',(#849),#50070);
#829=STYLED_ITEM('',(#50259),#849);
#849=MANIFOLD_SOLID_BREP('Body1',#9874);
#960=PLANE('',#10515);
#961=PLANE('',#10516);
#962=PLANE('',#10517);
#963=PLANE('',#10518);
#964=PLANE('',#10520);
#965=PLANE('',#10521);
#966=PLANE('',#10526);
#967=PLANE('',#10527);
#968=PLANE('',#10528);
#969=PLANE('',#10539);
#970=PLANE('',#10549);
#971=PLANE('',#10550);
#972=PLANE('',#10551);
#973=PLANE('',#10552);
#974=PLANE('',#10553);
#975=PLANE('',#10554);
#976=PLANE('',#10555);
#977=PLANE('',#10558);
#978=PLANE('',#10559);
#979=PLANE('',#10560);
#980=PLANE('',#10565);
#981=PLANE('',#10567);
#982=PLANE('',#10568);
#983=PLANE('',#10569);
#984=PLANE('',#10570);
#985=PLANE('',#10571);
#986=PLANE('',#10572);
#987=PLANE('',#10575);
#988=PLANE('',#10576);
#989=PLANE('',#10583);
#990=PLANE('',#10584);
#991=PLANE('',#10591);
#992=PLANE('',#10595);
#993=PLANE('',#10596);
#994=PLANE('',#10599);
#995=PLANE('',#10605);
#996=PLANE('',#10606);
#1276=FACE_OUTER_BOUND('',#1848,.T.);
#1277=FACE_OUTER_BOUND('',#1849,.T.);
#1278=FACE_OUTER_BOUND('',#1850,.T.);
#1279=FACE_OUTER_BOUND('',#1851,.T.);
#1280=FACE_OUTER_BOUND('',#1852,.T.);
#1281=FACE_OUTER_BOUND('',#1853,.T.);
#1282=FACE_OUTER_BOUND('',#1854,.T.);
#1283=FACE_OUTER_BOUND('',#1855,.T.);
#1284=FACE_OUTER_BOUND('',#1856,.T.);
#1285=FACE_OUTER_BOUND('',#1857,.T.);
#1286=FACE_OUTER_BOUND('',#1858,.T.);
#1287=FACE_OUTER_BOUND('',#1859,.T.);
#1288=FACE_OUTER_BOUND('',#1860,.T.);
#1289=FACE_OUTER_BOUND('',#1861,.T.);
#1290=FACE_OUTER_BOUND('',#1862,.T.);
#1291=FACE_OUTER_BOUND('',#1863,.T.);
#1292=FACE_OUTER_BOUND('',#1864,.T.);
#1293=FACE_OUTER_BOUND('',#1865,.T.);
#1294=FACE_OUTER_BOUND('',#1866,.T.);
#1295=FACE_OUTER_BOUND('',#1867,.T.);
#1296=FACE_OUTER_BOUND('',#1868,.T.);
#1297=FACE_OUTER_BOUND('',#1869,.T.);
#1298=FACE_OUTER_BOUND('',#1870,.T.);
#1299=FACE_OUTER_BOUND('',#1871,.T.);
#1300=FACE_OUTER_BOUND('',#1872,.T.);
#1301=FACE_OUTER_BOUND('',#1873,.T.);
#1302=FACE_OUTER_BOUND('',#1874,.T.);
#1303=FACE_OUTER_BOUND('',#1875,.T.);
#1304=FACE_OUTER_BOUND('',#1876,.T.);
#1305=FACE_OUTER_BOUND('',#1877,.T.);
#1306=FACE_OUTER_BOUND('',#1878,.T.);
#1307=FACE_OUTER_BOUND('',#1879,.T.);
#1308=FACE_OUTER_BOUND('',#1880,.T.);
#1309=FACE_OUTER_BOUND('',#1881,.T.);
#1310=FACE_OUTER_BOUND('',#1882,.T.);
#1311=FACE_OUTER_BOUND('',#1883,.T.);
#1312=FACE_OUTER_BOUND('',#1884,.T.);
#1313=FACE_OUTER_BOUND('',#1885,.T.);
#1314=FACE_OUTER_BOUND('',#1886,.T.);
#1315=FACE_OUTER_BOUND('',#1887,.T.);
#1316=FACE_OUTER_BOUND('',#1888,.T.);
#1317=FACE_OUTER_BOUND('',#1889,.T.);
#1318=FACE_OUTER_BOUND('',#1890,.T.);
#1319=FACE_OUTER_BOUND('',#1891,.T.);
#1320=FACE_OUTER_BOUND('',#1892,.T.);
#1321=FACE_OUTER_BOUND('',#1893,.T.);
#1322=FACE_OUTER_BOUND('',#1895,.T.);
#1323=FACE_OUTER_BOUND('',#1896,.T.);
#1324=FACE_OUTER_BOUND('',#1899,.T.);
#1325=FACE_OUTER_BOUND('',#1900,.T.);
#1326=FACE_OUTER_BOUND('',#1901,.T.);
#1327=FACE_OUTER_BOUND('',#1902,.T.);
#1328=FACE_OUTER_BOUND('',#1903,.T.);
#1329=FACE_OUTER_BOUND('',#1904,.T.);
#1330=FACE_OUTER_BOUND('',#1905,.T.);
#1331=FACE_OUTER_BOUND('',#1906,.T.);
#1332=FACE_OUTER_BOUND('',#1907,.T.);
#1333=FACE_OUTER_BOUND('',#1908,.T.);
#1334=FACE_OUTER_BOUND('',#1909,.T.);
#1335=FACE_OUTER_BOUND('',#1910,.T.);
#1336=FACE_OUTER_BOUND('',#1911,.T.);
#1337=FACE_OUTER_BOUND('',#1912,.T.);
#1338=FACE_OUTER_BOUND('',#1913,.T.);
#1339=FACE_OUTER_BOUND('',#1914,.T.);
#1340=FACE_OUTER_BOUND('',#1915,.T.);
#1341=FACE_OUTER_BOUND('',#1916,.T.);
#1342=FACE_OUTER_BOUND('',#1918,.T.);
#1343=FACE_OUTER_BOUND('',#1919,.T.);
#1344=FACE_OUTER_BOUND('',#1920,.T.);
#1345=FACE_OUTER_BOUND('',#1921,.T.);
#1346=FACE_OUTER_BOUND('',#1922,.T.);
#1347=FACE_OUTER_BOUND('',#1923,.T.);
#1348=FACE_OUTER_BOUND('',#1924,.T.);
#1349=FACE_OUTER_BOUND('',#1925,.T.);
#1350=FACE_OUTER_BOUND('',#1926,.T.);
#1351=FACE_OUTER_BOUND('',#1927,.T.);
#1352=FACE_OUTER_BOUND('',#1928,.T.);
#1353=FACE_OUTER_BOUND('',#1929,.T.);
#1354=FACE_OUTER_BOUND('',#1930,.T.);
#1355=FACE_OUTER_BOUND('',#1933,.T.);
#1356=FACE_OUTER_BOUND('',#1934,.T.);
#1357=FACE_OUTER_BOUND('',#1935,.T.);
#1358=FACE_OUTER_BOUND('',#1936,.T.);
#1359=FACE_OUTER_BOUND('',#1937,.T.);
#1360=FACE_OUTER_BOUND('',#1938,.T.);
#1361=FACE_OUTER_BOUND('',#1940,.T.);
#1362=FACE_OUTER_BOUND('',#1941,.T.);
#1363=FACE_OUTER_BOUND('',#1942,.T.);
#1364=FACE_OUTER_BOUND('',#1943,.T.);
#1365=FACE_OUTER_BOUND('',#1944,.T.);
#1366=FACE_OUTER_BOUND('',#1945,.T.);
#1367=FACE_OUTER_BOUND('',#1946,.T.);
#1368=FACE_OUTER_BOUND('',#1947,.T.);
#1369=FACE_OUTER_BOUND('',#1948,.T.);
#1370=FACE_OUTER_BOUND('',#1949,.T.);
#1371=FACE_OUTER_BOUND('',#1950,.T.);
#1372=FACE_OUTER_BOUND('',#1951,.T.);
#1373=FACE_OUTER_BOUND('',#1952,.T.);
#1374=FACE_OUTER_BOUND('',#1953,.T.);
#1375=FACE_OUTER_BOUND('',#1954,.T.);
#1376=FACE_OUTER_BOUND('',#1955,.T.);
#1377=FACE_OUTER_BOUND('',#1956,.T.);
#1378=FACE_OUTER_BOUND('',#1957,.T.);
#1379=FACE_OUTER_BOUND('',#1958,.T.);
#1380=FACE_OUTER_BOUND('',#1959,.T.);
#1381=FACE_OUTER_BOUND('',#1960,.T.);
#1382=FACE_OUTER_BOUND('',#1961,.T.);
#1383=FACE_OUTER_BOUND('',#1962,.T.);
#1384=FACE_OUTER_BOUND('',#1963,.T.);
#1385=FACE_OUTER_BOUND('',#1964,.T.);
#1848=EDGE_LOOP('',(#7052,#7053,#7054,#7055,#7056,#7057));
#1849=EDGE_LOOP('',(#7058,#7059,#7060,#7061,#7062));
#1850=EDGE_LOOP('',(#7063,#7064,#7065,#7066,#7067));
#1851=EDGE_LOOP('',(#7068,#7069,#7070,#7071));
#1852=EDGE_LOOP('',(#7072,#7073,#7074,#7075));
#1853=EDGE_LOOP('',(#7076,#7077,#7078,#7079));
#1854=EDGE_LOOP('',(#7080,#7081,#7082,#7083,#7084));
#1855=EDGE_LOOP('',(#7085,#7086,#7087,#7088));
#1856=EDGE_LOOP('',(#7089,#7090,#7091,#7092,#7093));
#1857=EDGE_LOOP('',(#7094,#7095,#7096,#7097,#7098,#7099));
#1858=EDGE_LOOP('',(#7100,#7101,#7102,#7103));
#1859=EDGE_LOOP('',(#7104,#7105,#7106,#7107));
#1860=EDGE_LOOP('',(#7108,#7109,#7110,#7111));
#1861=EDGE_LOOP('',(#7112,#7113,#7114,#7115,#7116,#7117));
#1862=EDGE_LOOP('',(#7118,#7119,#7120,#7121));
#1863=EDGE_LOOP('',(#7122,#7123,#7124,#7125));
#1864=EDGE_LOOP('',(#7126,#7127,#7128,#7129));
#1865=EDGE_LOOP('',(#7130,#7131,#7132,#7133));
#1866=EDGE_LOOP('',(#7134,#7135,#7136,#7137,#7138));
#1867=EDGE_LOOP('',(#7139,#7140,#7141,#7142,#7143));
#1868=EDGE_LOOP('',(#7144,#7145,#7146,#7147));
#1869=EDGE_LOOP('',(#7148,#7149,#7150,#7151));
#1870=EDGE_LOOP('',(#7152,#7153,#7154,#7155));
#1871=EDGE_LOOP('',(#7156,#7157,#7158,#7159));
#1872=EDGE_LOOP('',(#7160,#7161,#7162,#7163));
#1873=EDGE_LOOP('',(#7164,#7165,#7166,#7167));
#1874=EDGE_LOOP('',(#7168,#7169,#7170,#7171));
#1875=EDGE_LOOP('',(#7172,#7173,#7174,#7175));
#1876=EDGE_LOOP('',(#7176,#7177,#7178,#7179));
#1877=EDGE_LOOP('',(#7180,#7181,#7182,#7183));
#1878=EDGE_LOOP('',(#7184,#7185,#7186,#7187));
#1879=EDGE_LOOP('',(#7188,#7189,#7190,#7191));
#1880=EDGE_LOOP('',(#7192,#7193,#7194,#7195));
#1881=EDGE_LOOP('',(#7196,#7197,#7198,#7199));
#1882=EDGE_LOOP('',(#7200,#7201,#7202,#7203));
#1883=EDGE_LOOP('',(#7204,#7205,#7206,#7207));
#1884=EDGE_LOOP('',(#7208,#7209,#7210,#7211));
#1885=EDGE_LOOP('',(#7212,#7213,#7214,#7215));
#1886=EDGE_LOOP('',(#7216,#7217,#7218,#7219));
#1887=EDGE_LOOP('',(#7220,#7221,#7222,#7223));
#1888=EDGE_LOOP('',(#7224,#7225,#7226,#7227));
#1889=EDGE_LOOP('',(#7228,#7229,#7230,#7231));
#1890=EDGE_LOOP('',(#7232,#7233,#7234,#7235));
#1891=EDGE_LOOP('',(#7236,#7237,#7238,#7239));
#1892=EDGE_LOOP('',(#7240,#7241,#7242,#7243));
#1893=EDGE_LOOP('',(#7244,#7245,#7246,#7247,#7248,#7249,#7250,#7251));
#1894=EDGE_LOOP('',(#7252));
#1895=EDGE_LOOP('',(#7253,#7254,#7255,#7256));
#1896=EDGE_LOOP('',(#7257,#7258,#7259,#7260,#7261,#7262,#7263));
#1897=EDGE_LOOP('',(#7264));
#1898=EDGE_LOOP('',(#7265));
#1899=EDGE_LOOP('',(#7266,#7267,#7268));
#1900=EDGE_LOOP('',(#7269,#7270,#7271));
#1901=EDGE_LOOP('',(#7272,#7273,#7274,#7275,#7276,#7277,#7278,#7279,#7280,
#7281,#7282));
#1902=EDGE_LOOP('',(#7283,#7284,#7285,#7286));
#1903=EDGE_LOOP('',(#7287,#7288,#7289,#7290));
#1904=EDGE_LOOP('',(#7291,#7292,#7293,#7294));
#1905=EDGE_LOOP('',(#7295,#7296,#7297,#7298,#7299,#7300,#7301,#7302,#7303,
#7304,#7305));
#1906=EDGE_LOOP('',(#7306,#7307,#7308,#7309));
#1907=EDGE_LOOP('',(#7310,#7311,#7312,#7313));
#1908=EDGE_LOOP('',(#7314,#7315,#7316,#7317,#7318));
#1909=EDGE_LOOP('',(#7319,#7320,#7321,#7322,#7323,#7324,#7325));
#1910=EDGE_LOOP('',(#7326,#7327,#7328,#7329,#7330,#7331));
#1911=EDGE_LOOP('',(#7332,#7333,#7334,#7335));
#1912=EDGE_LOOP('',(#7336,#7337,#7338,#7339));
#1913=EDGE_LOOP('',(#7340,#7341,#7342,#7343,#7344,#7345));
#1914=EDGE_LOOP('',(#7346,#7347,#7348,#7349));
#1915=EDGE_LOOP('',(#7350,#7351,#7352,#7353));
#1916=EDGE_LOOP('',(#7354,#7355,#7356,#7357,#7358,#7359,#7360,#7361));
#1917=EDGE_LOOP('',(#7362,#7363,#7364,#7365));
#1918=EDGE_LOOP('',(#7366,#7367,#7368,#7369,#7370,#7371));
#1919=EDGE_LOOP('',(#7372,#7373,#7374,#7375,#7376,#7377));
#1920=EDGE_LOOP('',(#7378,#7379,#7380,#7381));
#1921=EDGE_LOOP('',(#7382,#7383,#7384,#7385));
#1922=EDGE_LOOP('',(#7386,#7387,#7388,#7389,#7390,#7391));
#1923=EDGE_LOOP('',(#7392,#7393,#7394,#7395,#7396,#7397,#7398,#7399,#7400,
#7401,#7402,#7403,#7404,#7405,#7406,#7407,#7408,#7409,#7410,#7411,#7412,
#7413,#7414,#7415));
#1924=EDGE_LOOP('',(#7416,#7417,#7418,#7419));
#1925=EDGE_LOOP('',(#7420,#7421,#7422,#7423));
#1926=EDGE_LOOP('',(#7424,#7425,#7426));
#1927=EDGE_LOOP('',(#7427,#7428,#7429,#7430));
#1928=EDGE_LOOP('',(#7431,#7432,#7433));
#1929=EDGE_LOOP('',(#7434,#7435,#7436));
#1930=EDGE_LOOP('',(#7437,#7438,#7439,#7440));
#1931=EDGE_LOOP('',(#7441));
#1932=EDGE_LOOP('',(#7442));
#1933=EDGE_LOOP('',(#7443,#7444,#7445));
#1934=EDGE_LOOP('',(#7446,#7447,#7448,#7449));
#1935=EDGE_LOOP('',(#7450,#7451,#7452,#7453,#7454));
#1936=EDGE_LOOP('',(#7455,#7456,#7457,#7458,#7459,#7460,#7461,#7462,#7463,
#7464,#7465,#7466,#7467,#7468,#7469,#7470,#7471,#7472,#7473,#7474,#7475,
#7476,#7477,#7478,#7479,#7480,#7481,#7482,#7483,#7484,#7485,#7486,#7487,
#7488));
#1937=EDGE_LOOP('',(#7489,#7490,#7491,#7492,#7493,#7494,#7495,#7496,#7497,
#7498,#7499,#7500,#7501,#7502,#7503,#7504,#7505,#7506,#7507,#7508,#7509,
#7510,#7511,#7512,#7513,#7514,#7515,#7516,#7517,#7518,#7519,#7520));
#1938=EDGE_LOOP('',(#7521,#7522,#7523,#7524));
#1939=EDGE_LOOP('',(#7525,#7526,#7527,#7528,#7529,#7530,#7531,#7532,#7533,
#7534,#7535,#7536,#7537,#7538,#7539,#7540,#7541,#7542,#7543,#7544,#7545,
#7546,#7547,#7548,#7549));
#1940=EDGE_LOOP('',(#7550,#7551,#7552));
#1941=EDGE_LOOP('',(#7553,#7554,#7555));
#1942=EDGE_LOOP('',(#7556,#7557,#7558,#7559,#7560,#7561,#7562,#7563,#7564,
#7565,#7566,#7567,#7568,#7569,#7570,#7571,#7572,#7573,#7574,#7575,#7576,
#7577,#7578,#7579));
#1943=EDGE_LOOP('',(#7580,#7581,#7582,#7583,#7584,#7585,#7586,#7587,#7588,
#7589,#7590,#7591,#7592,#7593,#7594,#7595,#7596,#7597));
#1944=EDGE_LOOP('',(#7598,#7599,#7600,#7601,#7602,#7603));
#1945=EDGE_LOOP('',(#7604,#7605,#7606,#7607,#7608,#7609,#7610,#7611,#7612,
#7613,#7614,#7615,#7616,#7617,#7618,#7619,#7620,#7621));
#1946=EDGE_LOOP('',(#7622,#7623,#7624,#7625,#7626,#7627,#7628,#7629,#7630,
#7631,#7632,#7633,#7634,#7635,#7636,#7637,#7638,#7639,#7640,#7641,#7642,
#7643,#7644));
#1947=EDGE_LOOP('',(#7645,#7646,#7647,#7648,#7649,#7650,#7651,#7652,#7653,
#7654,#7655,#7656,#7657,#7658,#7659,#7660,#7661,#7662,#7663,#7664,#7665,
#7666,#7667,#7668,#7669));
#1948=EDGE_LOOP('',(#7670,#7671,#7672,#7673,#7674));
#1949=EDGE_LOOP('',(#7675,#7676,#7677,#7678));
#1950=EDGE_LOOP('',(#7679,#7680,#7681,#7682,#7683,#7684));
#1951=EDGE_LOOP('',(#7685,#7686,#7687,#7688));
#1952=EDGE_LOOP('',(#7689,#7690,#7691,#7692,#7693));
#1953=EDGE_LOOP('',(#7694,#7695,#7696));
#1954=EDGE_LOOP('',(#7697,#7698,#7699));
#1955=EDGE_LOOP('',(#7700,#7701,#7702,#7703,#7704));
#1956=EDGE_LOOP('',(#7705,#7706,#7707,#7708));
#1957=EDGE_LOOP('',(#7709,#7710,#7711,#7712));
#1958=EDGE_LOOP('',(#7713,#7714,#7715,#7716));
#1959=EDGE_LOOP('',(#7717,#7718,#7719,#7720));
#1960=EDGE_LOOP('',(#7721,#7722,#7723,#7724));
#1961=EDGE_LOOP('',(#7725,#7726,#7727,#7728));
#1962=EDGE_LOOP('',(#7729,#7730,#7731,#7732));
#1963=EDGE_LOOP('',(#7733,#7734));
#1964=EDGE_LOOP('',(#7735,#7736,#7737,#7738,#7739));
#2403=LINE('',#18143,#2981);
#2404=LINE('',#18223,#2982);
#2405=LINE('',#18592,#2983);
#2406=LINE('',#18957,#2984);
#2407=LINE('',#19317,#2985);
#2408=LINE('',#19677,#2986);
#2409=LINE('',#20039,#2987);
#2410=LINE('',#20412,#2988);
#2411=LINE('',#20536,#2989);
#2412=LINE('',#20646,#2990);
#2413=LINE('',#21044,#2991);
#2414=LINE('',#21466,#2992);
#2415=LINE('',#21858,#2993);
#2416=LINE('',#22280,#2994);
#2417=LINE('',#22704,#2995);
#2418=LINE('',#23110,#2996);
#2419=LINE('',#23528,#2997);
#2420=LINE('',#23930,#2998);
#2421=LINE('',#24346,#2999);
#2422=LINE('',#24745,#3000);
#2423=LINE('',#25168,#3001);
#2424=LINE('',#25304,#3002);
#2425=LINE('',#25357,#3003);
#2426=LINE('',#25444,#3004);
#2427=LINE('',#25659,#3005);
#2428=LINE('',#25866,#3006);
#2429=LINE('',#26073,#3007);
#2430=LINE('',#26298,#3008);
#2431=LINE('',#26379,#3009);
#2432=LINE('',#26436,#3010);
#2433=LINE('',#26538,#3011);
#2434=LINE('',#26640,#3012);
#2435=LINE('',#26742,#3013);
#2436=LINE('',#26850,#3014);
#2437=LINE('',#26952,#3015);
#2438=LINE('',#27054,#3016);
#2439=LINE('',#27168,#3017);
#2440=LINE('',#27267,#3018);
#2441=LINE('',#27369,#3019);
#2442=LINE('',#27471,#3020);
#2443=LINE('',#27858,#3021);
#2444=LINE('',#27860,#3022);
#2445=LINE('',#27862,#3023);
#2446=LINE('',#27863,#3024);
#2447=LINE('',#27866,#3025);
#2448=LINE('',#27868,#3026);
#2449=LINE('',#27869,#3027);
#2450=LINE('',#27872,#3028);
#2451=LINE('',#27874,#3029);
#2452=LINE('',#27875,#3030);
#2453=LINE('',#27882,#3031);
#2454=LINE('',#27884,#3032);
#2455=LINE('',#27886,#3033);
#2456=LINE('',#27891,#3034);
#2457=LINE('',#27896,#3035);
#2458=LINE('',#27897,#3036);
#2459=LINE('',#27901,#3037);
#2460=LINE('',#27902,#3038);
#2461=LINE('',#27904,#3039);
#2462=LINE('',#27906,#3040);
#2463=LINE('',#27915,#3041);
#2464=LINE('',#27917,#3042);
#2465=LINE('',#27923,#3043);
#2466=LINE('',#27924,#3044);
#2467=LINE('',#27928,#3045);
#2468=LINE('',#27930,#3046);
#2469=LINE('',#27932,#3047);
#2470=LINE('',#27934,#3048);
#2471=LINE('',#27939,#3049);
#2472=LINE('',#27945,#3050);
#2473=LINE('',#27957,#3051);
#2474=LINE('',#27959,#3052);
#2475=LINE('',#27961,#3053);
#2476=LINE('',#27962,#3054);
#2477=LINE('',#27964,#3055);
#2478=LINE('',#27966,#3056);
#2479=LINE('',#27973,#3057);
#2480=LINE('',#27979,#3058);
#2481=LINE('',#27982,#3059);
#2482=LINE('',#27988,#3060);
#2483=LINE('',#27990,#3061);
#2484=LINE('',#27991,#3062);
#2485=LINE('',#27993,#3063);
#2486=LINE('',#27995,#3064);
#2487=LINE('',#28002,#3065);
#2488=LINE('',#28003,#3066);
#2489=LINE('',#28004,#3067);
#2490=LINE('',#28007,#3068);
#2491=LINE('',#28009,#3069);
#2492=LINE('',#28010,#3070);
#2493=LINE('',#28013,#3071);
#2494=LINE('',#28015,#3072);
#2495=LINE('',#28016,#3073);
#2496=LINE('',#28019,#3074);
#2497=LINE('',#28020,#3075);
#2498=LINE('',#28077,#3076);
#2499=LINE('',#28083,#3077);
#2500=LINE('',#28085,#3078);
#2501=LINE('',#28086,#3079);
#2502=LINE('',#28089,#3080);
#2503=LINE('',#28090,#3081);
#2504=LINE('',#28093,#3082);
#2505=LINE('',#28095,#3083);
#2506=LINE('',#28096,#3084);
#2507=LINE('',#28100,#3085);
#2508=LINE('',#29355,#3086);
#2509=LINE('',#29358,#3087);
#2510=LINE('',#29360,#3088);
#2511=LINE('',#29361,#3089);
#2512=LINE('',#29367,#3090);
#2513=LINE('',#29369,#3091);
#2514=LINE('',#30512,#3092);
#2515=LINE('',#30597,#3093);
#2516=LINE('',#30682,#3094);
#2517=LINE('',#30685,#3095);
#2518=LINE('',#30687,#3096);
#2519=LINE('',#33779,#3097);
#2520=LINE('',#34593,#3098);
#2981=VECTOR('',#11919,0.001543);
#2982=VECTOR('',#11922,0.001543);
#2983=VECTOR('',#11925,0.001543);
#2984=VECTOR('',#11928,0.001543);
#2985=VECTOR('',#11931,0.001543);
#2986=VECTOR('',#11934,0.001543);
#2987=VECTOR('',#11937,0.001543);
#2988=VECTOR('',#11940,0.001543);
#2989=VECTOR('',#11945,0.001543);
#2990=VECTOR('',#11950,0.001543);
#2991=VECTOR('',#11953,0.001543);
#2992=VECTOR('',#11956,0.001543);
#2993=VECTOR('',#11959,0.001543);
#2994=VECTOR('',#11962,0.001543);
#2995=VECTOR('',#11965,0.001543);
#2996=VECTOR('',#11968,0.001543);
#2997=VECTOR('',#11971,0.001543);
#2998=VECTOR('',#11974,0.001543);
#2999=VECTOR('',#11977,0.001543);
#3000=VECTOR('',#11980,0.001543);
#3001=VECTOR('',#11983,0.001543);
#3002=VECTOR('',#11988,0.0012645);
#3003=VECTOR('',#11991,0.0012645);
#3004=VECTOR('',#11994,0.0012645);
#3005=VECTOR('',#11997,0.0012645);
#3006=VECTOR('',#12000,0.0012645);
#3007=VECTOR('',#12003,0.0012645);
#3008=VECTOR('',#12006,0.0012645);
#3009=VECTOR('',#12011,0.0012645);
#3010=VECTOR('',#12016,0.0012645);
#3011=VECTOR('',#12019,0.0012645);
#3012=VECTOR('',#12022,0.0012645);
#3013=VECTOR('',#12025,0.0012645);
#3014=VECTOR('',#12028,0.0012645);
#3015=VECTOR('',#12031,0.0012645);
#3016=VECTOR('',#12034,0.0012645);
#3017=VECTOR('',#12037,0.0012645);
#3018=VECTOR('',#12040,0.0012645);
#3019=VECTOR('',#12043,0.0012645);
#3020=VECTOR('',#12046,0.0012645);
#3021=VECTOR('',#12055,1.);
#3022=VECTOR('',#12056,1.);
#3023=VECTOR('',#12057,1.);
#3024=VECTOR('',#12058,1.);
#3025=VECTOR('',#12061,1.);
#3026=VECTOR('',#12062,1.);
#3027=VECTOR('',#12063,1.);
#3028=VECTOR('',#12066,1.);
#3029=VECTOR('',#12067,1.);
#3030=VECTOR('',#12068,1.);
#3031=VECTOR('',#12071,1.);
#3032=VECTOR('',#12072,1.);
#3033=VECTOR('',#12073,1.);
#3034=VECTOR('',#12074,1.);
#3035=VECTOR('',#12079,1.);
#3036=VECTOR('',#12080,1.);
#3037=VECTOR('',#12083,1.);
#3038=VECTOR('',#12084,1.);
#3039=VECTOR('',#12085,1.);
#3040=VECTOR('',#12086,1.);
#3041=VECTOR('',#12097,1.);
#3042=VECTOR('',#12100,1.);
#3043=VECTOR('',#12105,1.);
#3044=VECTOR('',#12106,1.);
#3045=VECTOR('',#12109,1.);
#3046=VECTOR('',#12110,1.);
#3047=VECTOR('',#12111,1.);
#3048=VECTOR('',#12112,1.);
#3049=VECTOR('',#12119,0.0015);
#3050=VECTOR('',#12126,1.);
#3051=VECTOR('',#12135,1.);
#3052=VECTOR('',#12136,1.);
#3053=VECTOR('',#12137,1.);
#3054=VECTOR('',#12138,1.);
#3055=VECTOR('',#12139,1.);
#3056=VECTOR('',#12140,1.);
#3057=VECTOR('',#12147,0.0016);
#3058=VECTOR('',#12154,0.0031);
#3059=VECTOR('',#12159,0.0016);
#3060=VECTOR('',#12162,1.);
#3061=VECTOR('',#12163,1.);
#3062=VECTOR('',#12164,1.);
#3063=VECTOR('',#12167,1.);
#3064=VECTOR('',#12170,1.);
#3065=VECTOR('',#12173,1.);
#3066=VECTOR('',#12174,1.);
#3067=VECTOR('',#12175,1.);
#3068=VECTOR('',#12178,1.);
#3069=VECTOR('',#12179,1.);
#3070=VECTOR('',#12180,1.);
#3071=VECTOR('',#12183,1.);
#3072=VECTOR('',#12184,1.);
#3073=VECTOR('',#12185,1.);
#3074=VECTOR('',#12188,1.);
#3075=VECTOR('',#12189,1.);
#3076=VECTOR('',#12194,0.00175);
#3077=VECTOR('',#12197,1.);
#3078=VECTOR('',#12198,1.);
#3079=VECTOR('',#12199,1.);
#3080=VECTOR('',#12202,1.);
#3081=VECTOR('',#12203,1.);
#3082=VECTOR('',#12206,1.);
#3083=VECTOR('',#12207,1.);
#3084=VECTOR('',#12208,1.);
#3085=VECTOR('',#12213,0.00175);
#3086=VECTOR('',#12228,1.);
#3087=VECTOR('',#12233,1.);
#3088=VECTOR('',#12236,1.);
#3089=VECTOR('',#12237,1.);
#3090=VECTOR('',#12244,1.);
#3091=VECTOR('',#12247,1.);
#3092=VECTOR('',#12252,0.00155);
#3093=VECTOR('',#12255,1.);
#3094=VECTOR('',#12260,1.);
#3095=VECTOR('',#12265,1.);
#3096=VECTOR('',#12268,1.);
#3097=VECTOR('',#12273,0.0031);
#3098=VECTOR('',#12288,0.0016);
#3559=CIRCLE('',#10475,0.00154300000001001);
#3560=CIRCLE('',#10477,0.00154300000001);
#3561=CIRCLE('',#10490,0.00154300000001);
#3562=CIRCLE('',#10498,0.00126450000001);
#3563=CIRCLE('',#10500,0.00126450000001);
#3564=CIRCLE('',#10512,0.00126450000001);
#3565=CIRCLE('',#10519,0.00150000000001);
#3566=CIRCLE('',#10522,0.00170000000001);
#3567=CIRCLE('',#10523,0.00170000000001);
#3568=CIRCLE('',#10524,0.00320000000001);
#3569=CIRCLE('',#10525,0.00170000000001);
#3570=CIRCLE('',#10529,0.00195000000001);
#3571=CIRCLE('',#10530,0.00340000000001);
#3572=CIRCLE('',#10531,0.00195000000001);
#3573=CIRCLE('',#10533,0.00150000000001);
#3574=CIRCLE('',#10535,0.00300000000001);
#3575=CIRCLE('',#10536,0.00300000000001);
#3576=CIRCLE('',#10538,0.00340000000001);
#3577=CIRCLE('',#10540,0.00195000000001);
#3578=CIRCLE('',#10541,0.00195000000001);
#3579=CIRCLE('',#10545,0.00250000000001);
#3580=CIRCLE('',#10546,0.00250000000001);
#3581=CIRCLE('',#10548,0.00126450000001);
#3582=CIRCLE('',#10557,0.00155000000001);
#3583=CIRCLE('',#10562,0.00155000000001);
#3584=CIRCLE('',#10564,0.00250000000001);
#3585=CIRCLE('',#10566,0.00300000000001);
#3586=CIRCLE('',#10573,0.00320000000001);
#3587=CIRCLE('',#10574,0.00170000000001);
#3588=CIRCLE('',#10586,0.00250000000001);
#3589=CIRCLE('',#10587,0.00250000000001);
#3590=CIRCLE('',#10589,0.00300000000001);
#3591=CIRCLE('',#10593,0.00126450000001);
#3592=CIRCLE('',#10594,0.00126450000001);
#3593=CIRCLE('',#10598,0.00154300000001001);
#4056=VERTEX_POINT('',#18141);
#4057=VERTEX_POINT('',#18142);
#4058=VERTEX_POINT('',#18144);
#4059=VERTEX_POINT('',#18149);
#4060=VERTEX_POINT('',#18160);
#4061=VERTEX_POINT('',#18167);
#4062=VERTEX_POINT('',#18221);
#4063=VERTEX_POINT('',#18222);
#4064=VERTEX_POINT('',#18224);
#4065=VERTEX_POINT('',#18590);
#4066=VERTEX_POINT('',#18591);
#4067=VERTEX_POINT('',#18769);
#4068=VERTEX_POINT('',#18955);
#4069=VERTEX_POINT('',#18956);
#4070=VERTEX_POINT('',#19315);
#4071=VERTEX_POINT('',#19316);
#4072=VERTEX_POINT('',#19675);
#4073=VERTEX_POINT('',#19676);
#4074=VERTEX_POINT('',#20037);
#4075=VERTEX_POINT('',#20038);
#4076=VERTEX_POINT('',#20040);
#4077=VERTEX_POINT('',#20410);
#4078=VERTEX_POINT('',#20411);
#4079=VERTEX_POINT('',#20413);
#4080=VERTEX_POINT('',#20433);
#4081=VERTEX_POINT('',#20534);
#4082=VERTEX_POINT('',#20535);
#4083=VERTEX_POINT('',#20537);
#4084=VERTEX_POINT('',#20542);
#4085=VERTEX_POINT('',#20553);
#4086=VERTEX_POINT('',#20644);
#4087=VERTEX_POINT('',#20645);
#4088=VERTEX_POINT('',#20647);
#4089=VERTEX_POINT('',#20844);
#4090=VERTEX_POINT('',#21042);
#4091=VERTEX_POINT('',#21043);
#4092=VERTEX_POINT('',#21464);
#4093=VERTEX_POINT('',#21465);
#4094=VERTEX_POINT('',#21856);
#4095=VERTEX_POINT('',#21857);
#4096=VERTEX_POINT('',#22278);
#4097=VERTEX_POINT('',#22279);
#4098=VERTEX_POINT('',#22281);
#4099=VERTEX_POINT('',#22492);
#4100=VERTEX_POINT('',#22702);
#4101=VERTEX_POINT('',#22703);
#4102=VERTEX_POINT('',#23108);
#4103=VERTEX_POINT('',#23109);
#4104=VERTEX_POINT('',#23526);
#4105=VERTEX_POINT('',#23527);
#4106=VERTEX_POINT('',#23928);
#4107=VERTEX_POINT('',#23929);
#4108=VERTEX_POINT('',#24344);
#4109=VERTEX_POINT('',#24345);
#4110=VERTEX_POINT('',#24545);
#4111=VERTEX_POINT('',#24743);
#4112=VERTEX_POINT('',#24744);
#4113=VERTEX_POINT('',#24746);
#4114=VERTEX_POINT('',#25166);
#4115=VERTEX_POINT('',#25167);
#4116=VERTEX_POINT('',#25169);
#4117=VERTEX_POINT('',#25189);
#4118=VERTEX_POINT('',#25302);
#4119=VERTEX_POINT('',#25303);
#4120=VERTEX_POINT('',#25305);
#4121=VERTEX_POINT('',#25331);
#4122=VERTEX_POINT('',#25355);
#4123=VERTEX_POINT('',#25356);
#4124=VERTEX_POINT('',#25442);
#4125=VERTEX_POINT('',#25443);
#4126=VERTEX_POINT('',#25657);
#4127=VERTEX_POINT('',#25658);
#4128=VERTEX_POINT('',#25864);
#4129=VERTEX_POINT('',#25865);
#4130=VERTEX_POINT('',#26071);
#4131=VERTEX_POINT('',#26072);
#4132=VERTEX_POINT('',#26296);
#4133=VERTEX_POINT('',#26297);
#4134=VERTEX_POINT('',#26299);
#4135=VERTEX_POINT('',#26325);
#4136=VERTEX_POINT('',#26377);
#4137=VERTEX_POINT('',#26378);
#4138=VERTEX_POINT('',#26380);
#4139=VERTEX_POINT('',#26406);
#4140=VERTEX_POINT('',#26434);
#4141=VERTEX_POINT('',#26435);
#4142=VERTEX_POINT('',#26536);
#4143=VERTEX_POINT('',#26537);
#4144=VERTEX_POINT('',#26638);
#4145=VERTEX_POINT('',#26639);
#4146=VERTEX_POINT('',#26740);
#4147=VERTEX_POINT('',#26741);
#4148=VERTEX_POINT('',#26848);
#4149=VERTEX_POINT('',#26849);
#4150=VERTEX_POINT('',#26950);
#4151=VERTEX_POINT('',#26951);
#4152=VERTEX_POINT('',#27052);
#4153=VERTEX_POINT('',#27053);
#4154=VERTEX_POINT('',#27166);
#4155=VERTEX_POINT('',#27167);
#4156=VERTEX_POINT('',#27265);
#4157=VERTEX_POINT('',#27266);
#4158=VERTEX_POINT('',#27367);
#4159=VERTEX_POINT('',#27368);
#4160=VERTEX_POINT('',#27469);
#4161=VERTEX_POINT('',#27470);
#4162=VERTEX_POINT('',#27472);
#4163=VERTEX_POINT('',#27498);
#4164=VERTEX_POINT('',#27856);
#4165=VERTEX_POINT('',#27857);
#4166=VERTEX_POINT('',#27859);
#4167=VERTEX_POINT('',#27861);
#4168=VERTEX_POINT('',#27865);
#4169=VERTEX_POINT('',#27867);
#4170=VERTEX_POINT('',#27871);
#4171=VERTEX_POINT('',#27873);
#4172=VERTEX_POINT('',#27877);
#4173=VERTEX_POINT('',#27878);
#4174=VERTEX_POINT('',#27883);
#4175=VERTEX_POINT('',#27885);
#4176=VERTEX_POINT('',#27887);
#4177=VERTEX_POINT('',#27892);
#4178=VERTEX_POINT('',#27895);
#4179=VERTEX_POINT('',#27899);
#4180=VERTEX_POINT('',#27900);
#4181=VERTEX_POINT('',#27903);
#4182=VERTEX_POINT('',#27905);
#4183=VERTEX_POINT('',#27907);
#4184=VERTEX_POINT('',#27910);
#4185=VERTEX_POINT('',#27912);
#4186=VERTEX_POINT('',#27919);
#4187=VERTEX_POINT('',#27920);
#4188=VERTEX_POINT('',#27922);
#4189=VERTEX_POINT('',#27925);
#4190=VERTEX_POINT('',#27927);
#4191=VERTEX_POINT('',#27929);
#4192=VERTEX_POINT('',#27931);
#4193=VERTEX_POINT('',#27933);
#4194=VERTEX_POINT('',#27937);
#4195=VERTEX_POINT('',#27941);
#4196=VERTEX_POINT('',#27943);
#4197=VERTEX_POINT('',#27947);
#4198=VERTEX_POINT('',#27953);
#4199=VERTEX_POINT('',#27954);
#4200=VERTEX_POINT('',#27956);
#4201=VERTEX_POINT('',#27958);
#4202=VERTEX_POINT('',#27960);
#4203=VERTEX_POINT('',#27963);
#4204=VERTEX_POINT('',#27965);
#4205=VERTEX_POINT('',#27975);
#4206=VERTEX_POINT('',#27976);
#4207=VERTEX_POINT('',#27987);
#4208=VERTEX_POINT('',#27989);
#4209=VERTEX_POINT('',#28001);
#4210=VERTEX_POINT('',#28006);
#4211=VERTEX_POINT('',#28008);
#4212=VERTEX_POINT('',#28012);
#4213=VERTEX_POINT('',#28014);
#4214=VERTEX_POINT('',#28018);
#4215=VERTEX_POINT('',#28075);
#4216=VERTEX_POINT('',#28084);
#4217=VERTEX_POINT('',#28088);
#4218=VERTEX_POINT('',#28092);
#4219=VERTEX_POINT('',#28094);
#4220=VERTEX_POINT('',#28098);
#4221=VERTEX_POINT('',#28102);
#4222=VERTEX_POINT('',#28103);
#4223=VERTEX_POINT('',#28153);
#4224=VERTEX_POINT('',#28203);
#4225=VERTEX_POINT('',#28253);
#4226=VERTEX_POINT('',#28378);
#4227=VERTEX_POINT('',#28428);
#4228=VERTEX_POINT('',#28478);
#4229=VERTEX_POINT('',#28513);
#4230=VERTEX_POINT('',#28563);
#4231=VERTEX_POINT('',#28613);
#4232=VERTEX_POINT('',#28651);
#4233=VERTEX_POINT('',#28653);
#4234=VERTEX_POINT('',#28667);
#4235=VERTEX_POINT('',#28717);
#4236=VERTEX_POINT('',#28767);
#4237=VERTEX_POINT('',#28817);
#4238=VERTEX_POINT('',#28867);
#4239=VERTEX_POINT('',#28917);
#4240=VERTEX_POINT('',#28967);
#4241=VERTEX_POINT('',#29068);
#4242=VERTEX_POINT('',#29118);
#4243=VERTEX_POINT('',#29267);
#4244=VERTEX_POINT('',#29268);
#4245=VERTEX_POINT('',#29362);
#4246=VERTEX_POINT('',#29364);
#4247=VERTEX_POINT('',#29371);
#4248=VERTEX_POINT('',#30513);
#4249=VERTEX_POINT('',#30514);
#4250=VERTEX_POINT('',#30522);
#4251=VERTEX_POINT('',#30527);
#4252=VERTEX_POINT('',#30534);
#4253=VERTEX_POINT('',#30565);
#4254=VERTEX_POINT('',#30572);
#4255=VERTEX_POINT('',#30579);
#4256=VERTEX_POINT('',#30587);
#4257=VERTEX_POINT('',#30589);
#4258=VERTEX_POINT('',#30596);
#4259=VERTEX_POINT('',#30598);
#4260=VERTEX_POINT('',#30607);
#4261=VERTEX_POINT('',#30609);
#4262=VERTEX_POINT('',#30617);
#4263=VERTEX_POINT('',#30650);
#4264=VERTEX_POINT('',#30658);
#4265=VERTEX_POINT('',#30660);
#4266=VERTEX_POINT('',#30668);
#4267=VERTEX_POINT('',#30673);
#4268=VERTEX_POINT('',#30681);
#4269=VERTEX_POINT('',#30964);
#4270=VERTEX_POINT('',#31014);
#4271=VERTEX_POINT('',#31028);
#4272=VERTEX_POINT('',#31078);
#4273=VERTEX_POINT('',#31128);
#4274=VERTEX_POINT('',#31178);
#4275=VERTEX_POINT('',#31228);
#4276=VERTEX_POINT('',#31278);
#4277=VERTEX_POINT('',#31328);
#4278=VERTEX_POINT('',#31378);
#4279=VERTEX_POINT('',#31458);
#4280=VERTEX_POINT('',#31833);
#4281=VERTEX_POINT('',#31883);
#4282=VERTEX_POINT('',#31909);
#4283=VERTEX_POINT('',#32112);
#4284=VERTEX_POINT('',#33069);
#4285=VERTEX_POINT('',#33777);
#4286=VERTEX_POINT('',#34388);
#4287=VERTEX_POINT('',#34591);
#4288=VERTEX_POINT('',#34598);
#5179=EDGE_CURVE('',#4056,#4057,#2403,.T.);
#5180=EDGE_CURVE('',#4057,#4058,#204,.T.);
#5181=EDGE_CURVE('',#4058,#4059,#205,.T.);
#5182=EDGE_CURVE('',#4060,#4059,#206,.T.);
#5183=EDGE_CURVE('',#4061,#4060,#207,.F.);
#5184=EDGE_CURVE('',#4056,#4061,#208,.T.);
#5185=EDGE_CURVE('',#4062,#4063,#2404,.T.);
#5186=EDGE_CURVE('',#4063,#4064,#209,.F.);
#5187=EDGE_CURVE('',#4064,#4057,#210,.T.);
#5188=EDGE_CURVE('',#4062,#4056,#211,.T.);
#5189=EDGE_CURVE('',#4065,#4066,#2405,.T.);
#5190=EDGE_CURVE('',#4066,#4063,#212,.F.);
#5191=EDGE_CURVE('',#4067,#4062,#213,.T.);
#5192=EDGE_CURVE('',#4065,#4067,#214,.T.);
#5193=EDGE_CURVE('',#4068,#4069,#2406,.T.);
#5194=EDGE_CURVE('',#4069,#4066,#215,.F.);
#5195=EDGE_CURVE('',#4068,#4065,#216,.T.);
#5196=EDGE_CURVE('',#4070,#4071,#2407,.T.);
#5197=EDGE_CURVE('',#4071,#4069,#217,.F.);
#5198=EDGE_CURVE('',#4070,#4068,#218,.T.);
#5199=EDGE_CURVE('',#4072,#4073,#2408,.T.);
#5200=EDGE_CURVE('',#4073,#4071,#219,.F.);
#5201=EDGE_CURVE('',#4072,#4070,#220,.T.);
#5202=EDGE_CURVE('',#4074,#4075,#2409,.T.);
#5203=EDGE_CURVE('',#4075,#4076,#221,.T.);
#5204=EDGE_CURVE('',#4076,#4073,#222,.F.);
#5205=EDGE_CURVE('',#4074,#4072,#223,.T.);
#5206=EDGE_CURVE('',#4077,#4078,#2410,.T.);
#5207=EDGE_CURVE('',#4079,#4077,#224,.F.);
#5208=EDGE_CURVE('',#4080,#4079,#3559,.T.);
#5209=EDGE_CURVE('',#4080,#4078,#225,.T.);
#5210=EDGE_CURVE('',#4081,#4082,#2411,.T.);
#5211=EDGE_CURVE('',#4082,#4083,#226,.T.);
#5212=EDGE_CURVE('',#4083,#4084,#227,.T.);
#5213=EDGE_CURVE('',#4085,#4084,#3560,.T.);
#5214=EDGE_CURVE('',#4081,#4085,#228,.F.);
#5215=EDGE_CURVE('',#4086,#4087,#2412,.T.);
#5216=EDGE_CURVE('',#4087,#4088,#229,.T.);
#5217=EDGE_CURVE('',#4088,#4082,#230,.T.);
#5218=EDGE_CURVE('',#4089,#4081,#231,.F.);
#5219=EDGE_CURVE('',#4086,#4089,#232,.F.);
#5220=EDGE_CURVE('',#4090,#4091,#2413,.T.);
#5221=EDGE_CURVE('',#4091,#4087,#233,.T.);
#5222=EDGE_CURVE('',#4090,#4086,#234,.F.);
#5223=EDGE_CURVE('',#4092,#4093,#2414,.T.);
#5224=EDGE_CURVE('',#4093,#4091,#235,.T.);
#5225=EDGE_CURVE('',#4092,#4090,#236,.F.);
#5226=EDGE_CURVE('',#4094,#4095,#2415,.T.);
#5227=EDGE_CURVE('',#4095,#4093,#237,.T.);
#5228=EDGE_CURVE('',#4094,#4092,#238,.F.);
#5229=EDGE_CURVE('',#4096,#4097,#2416,.T.);
#5230=EDGE_CURVE('',#4097,#4098,#239,.T.);
#5231=EDGE_CURVE('',#4098,#4095,#240,.T.);
#5232=EDGE_CURVE('',#4099,#4094,#241,.F.);
#5233=EDGE_CURVE('',#4096,#4099,#242,.F.);
#5234=EDGE_CURVE('',#4100,#4101,#2417,.T.);
#5235=EDGE_CURVE('',#4101,#4097,#243,.T.);
#5236=EDGE_CURVE('',#4100,#4096,#244,.F.);
#5237=EDGE_CURVE('',#4102,#4103,#2418,.T.);
#5238=EDGE_CURVE('',#4103,#4101,#245,.T.);
#5239=EDGE_CURVE('',#4102,#4100,#246,.F.);
#5240=EDGE_CURVE('',#4104,#4105,#2419,.T.);
#5241=EDGE_CURVE('',#4105,#4103,#247,.T.);
#5242=EDGE_CURVE('',#4104,#4102,#248,.F.);
#5243=EDGE_CURVE('',#4106,#4107,#2420,.T.);
#5244=EDGE_CURVE('',#4107,#4105,#249,.T.);
#5245=EDGE_CURVE('',#4106,#4104,#250,.F.);
#5246=EDGE_CURVE('',#4108,#4109,#2421,.T.);
#5247=EDGE_CURVE('',#4109,#4107,#251,.T.);
#5248=EDGE_CURVE('',#4110,#4106,#252,.F.);
#5249=EDGE_CURVE('',#4108,#4110,#253,.F.);
#5250=EDGE_CURVE('',#4111,#4112,#2422,.T.);
#5251=EDGE_CURVE('',#4112,#4113,#254,.T.);
#5252=EDGE_CURVE('',#4113,#4109,#255,.T.);
#5253=EDGE_CURVE('',#4111,#4108,#256,.F.);
#5254=EDGE_CURVE('',#4114,#4115,#2423,.T.);
#5255=EDGE_CURVE('',#4116,#4114,#257,.F.);
#5256=EDGE_CURVE('',#4117,#4116,#3561,.T.);
#5257=EDGE_CURVE('',#4117,#4115,#258,.T.);
#5258=EDGE_CURVE('',#4118,#4119,#2424,.T.);
#5259=EDGE_CURVE('',#4119,#4120,#259,.T.);
#5260=EDGE_CURVE('',#4121,#4120,#260,.F.);
#5261=EDGE_CURVE('',#4121,#4118,#261,.T.);
#5262=EDGE_CURVE('',#4122,#4123,#2425,.T.);
#5263=EDGE_CURVE('',#4123,#4119,#262,.T.);
#5264=EDGE_CURVE('',#4118,#4122,#263,.T.);
#5265=EDGE_CURVE('',#4124,#4125,#2426,.T.);
#5266=EDGE_CURVE('',#4125,#4123,#264,.T.);
#5267=EDGE_CURVE('',#4122,#4124,#265,.T.);
#5268=EDGE_CURVE('',#4126,#4127,#2427,.T.);
#5269=EDGE_CURVE('',#4127,#4125,#266,.T.);
#5270=EDGE_CURVE('',#4124,#4126,#267,.T.);
#5271=EDGE_CURVE('',#4128,#4129,#2428,.T.);
#5272=EDGE_CURVE('',#4129,#4127,#268,.T.);
#5273=EDGE_CURVE('',#4126,#4128,#269,.T.);
#5274=EDGE_CURVE('',#4130,#4131,#2429,.T.);
#5275=EDGE_CURVE('',#4131,#4129,#270,.T.);
#5276=EDGE_CURVE('',#4128,#4130,#271,.T.);
#5277=EDGE_CURVE('',#4132,#4133,#2430,.T.);
#5278=EDGE_CURVE('',#4132,#4134,#272,.T.);
#5279=EDGE_CURVE('',#4135,#4134,#3562,.T.);
#5280=EDGE_CURVE('',#4135,#4133,#273,.T.);
#5281=EDGE_CURVE('',#4136,#4137,#2431,.T.);
#5282=EDGE_CURVE('',#4137,#4138,#274,.T.);
#5283=EDGE_CURVE('',#4139,#4138,#3563,.T.);
#5284=EDGE_CURVE('',#4139,#4136,#275,.T.);
#5285=EDGE_CURVE('',#4140,#4141,#2432,.T.);
#5286=EDGE_CURVE('',#4141,#4137,#276,.T.);
#5287=EDGE_CURVE('',#4136,#4140,#277,.T.);
#5288=EDGE_CURVE('',#4142,#4143,#2433,.T.);
#5289=EDGE_CURVE('',#4143,#4141,#278,.T.);
#5290=EDGE_CURVE('',#4140,#4142,#279,.T.);
#5291=EDGE_CURVE('',#4144,#4145,#2434,.T.);
#5292=EDGE_CURVE('',#4145,#4143,#280,.T.);
#5293=EDGE_CURVE('',#4142,#4144,#281,.T.);
#5294=EDGE_CURVE('',#4146,#4147,#2435,.T.);
#5295=EDGE_CURVE('',#4147,#4145,#282,.T.);
#5296=EDGE_CURVE('',#4144,#4146,#283,.T.);
#5297=EDGE_CURVE('',#4148,#4149,#2436,.T.);
#5298=EDGE_CURVE('',#4149,#4147,#284,.T.);
#5299=EDGE_CURVE('',#4146,#4148,#285,.T.);
#5300=EDGE_CURVE('',#4150,#4151,#2437,.T.);
#5301=EDGE_CURVE('',#4151,#4149,#286,.T.);
#5302=EDGE_CURVE('',#4148,#4150,#287,.T.);
#5303=EDGE_CURVE('',#4152,#4153,#2438,.T.);
#5304=EDGE_CURVE('',#4153,#4151,#288,.T.);
#5305=EDGE_CURVE('',#4150,#4152,#289,.T.);
#5306=EDGE_CURVE('',#4154,#4155,#2439,.T.);
#5307=EDGE_CURVE('',#4155,#4153,#290,.T.);
#5308=EDGE_CURVE('',#4152,#4154,#291,.T.);
#5309=EDGE_CURVE('',#4156,#4157,#2440,.T.);
#5310=EDGE_CURVE('',#4157,#4155,#292,.T.);
#5311=EDGE_CURVE('',#4154,#4156,#293,.T.);
#5312=EDGE_CURVE('',#4158,#4159,#2441,.T.);
#5313=EDGE_CURVE('',#4159,#4157,#294,.T.);
#5314=EDGE_CURVE('',#4156,#4158,#295,.T.);
#5315=EDGE_CURVE('',#4160,#4161,#2442,.T.);
#5316=EDGE_CURVE('',#4160,#4162,#296,.T.);
#5317=EDGE_CURVE('',#4163,#4162,#3564,.T.);
#5318=EDGE_CURVE('',#4163,#4161,#297,.T.);
#5319=EDGE_CURVE('',#4161,#4159,#298,.T.);
#5320=EDGE_CURVE('',#4158,#4160,#299,.T.);
#5321=EDGE_CURVE('',#4133,#4131,#300,.T.);
#5322=EDGE_CURVE('',#4130,#4132,#301,.T.);
#5323=EDGE_CURVE('',#4164,#4165,#2443,.T.);
#5324=EDGE_CURVE('',#4164,#4166,#2444,.T.);
#5325=EDGE_CURVE('',#4167,#4166,#2445,.T.);
#5326=EDGE_CURVE('',#4165,#4167,#2446,.T.);
#5327=EDGE_CURVE('',#4168,#4165,#2447,.T.);
#5328=EDGE_CURVE('',#4167,#4169,#2448,.T.);
#5329=EDGE_CURVE('',#4169,#4168,#2449,.T.);
#5330=EDGE_CURVE('',#4166,#4170,#2450,.T.);
#5331=EDGE_CURVE('',#4170,#4171,#2451,.T.);
#5332=EDGE_CURVE('',#4171,#4167,#2452,.T.);
#5333=EDGE_CURVE('',#4172,#4173,#677,.F.);
#5334=EDGE_CURVE('',#4170,#4172,#2453,.T.);
#5335=EDGE_CURVE('',#4174,#4164,#2454,.T.);
#5336=EDGE_CURVE('',#4175,#4174,#2455,.T.);
#5337=EDGE_CURVE('',#4176,#4175,#678,.F.);
#5338=EDGE_CURVE('',#4176,#4173,#2456,.T.);
#5339=EDGE_CURVE('',#4177,#4177,#3565,.T.);
#5340=EDGE_CURVE('',#4165,#4178,#2457,.T.);
#5341=EDGE_CURVE('',#4178,#4174,#2458,.T.);
#5342=EDGE_CURVE('',#4179,#4180,#2459,.T.);
#5343=EDGE_CURVE('',#4168,#4179,#2460,.T.);
#5344=EDGE_CURVE('',#4181,#4169,#2461,.T.);
#5345=EDGE_CURVE('',#4182,#4181,#2462,.T.);
#5346=EDGE_CURVE('',#4183,#4182,#3566,.T.);
#5347=EDGE_CURVE('',#4180,#4183,#3567,.T.);
#5348=EDGE_CURVE('',#4184,#4184,#3568,.T.);
#5349=EDGE_CURVE('',#4185,#4185,#3569,.T.);
#5350=EDGE_CURVE('',#4169,#4171,#2463,.T.);
#5351=EDGE_CURVE('',#4178,#4168,#2464,.T.);
#5352=EDGE_CURVE('',#4186,#4187,#3570,.T.);
#5353=EDGE_CURVE('',#4188,#4186,#2465,.T.);
#5354=EDGE_CURVE('',#4171,#4188,#2466,.T.);
#5355=EDGE_CURVE('',#4189,#4172,#3571,.T.);
#5356=EDGE_CURVE('',#4189,#4190,#2467,.T.);
#5357=EDGE_CURVE('',#4191,#4190,#2468,.T.);
#5358=EDGE_CURVE('',#4192,#4191,#2469,.T.);
#5359=EDGE_CURVE('',#4193,#4192,#2470,.T.);
#5360=EDGE_CURVE('',#4187,#4193,#3572,.T.);
#5361=EDGE_CURVE('',#4194,#4194,#3573,.T.);
#5362=EDGE_CURVE('',#4194,#4177,#2471,.T.);
#5363=EDGE_CURVE('',#4173,#4195,#3574,.T.);
#5364=EDGE_CURVE('',#4196,#4176,#3575,.T.);
#5365=EDGE_CURVE('',#4196,#4195,#2472,.T.);
#5366=EDGE_CURVE('',#4175,#4197,#3576,.T.);
#5367=EDGE_CURVE('',#4197,#4196,#679,.T.);
#5368=EDGE_CURVE('',#4198,#4199,#3577,.T.);
#5369=EDGE_CURVE('',#4200,#4198,#2473,.T.);
#5370=EDGE_CURVE('',#4201,#4200,#2474,.T.);
#5371=EDGE_CURVE('',#4202,#4201,#2475,.T.);
#5372=EDGE_CURVE('',#4202,#4197,#2476,.T.);
#5373=EDGE_CURVE('',#4203,#4178,#2477,.T.);
#5374=EDGE_CURVE('',#4204,#4203,#2478,.T.);
#5375=EDGE_CURVE('',#4199,#4204,#3578,.T.);
#5376=EDGE_CURVE('',#4195,#4189,#680,.T.);
#5377=EDGE_CURVE('',#4194,#4185,#2479,.T.);
#5378=EDGE_CURVE('',#4205,#4206,#3579,.T.);
#5379=EDGE_CURVE('',#4206,#4205,#3580,.T.);
#5380=EDGE_CURVE('',#4205,#4184,#2480,.T.);
#5381=EDGE_CURVE('',#4134,#4135,#3581,.T.);
#5382=EDGE_CURVE('',#4135,#4183,#2481,.T.);
#5383=EDGE_CURVE('',#4180,#4182,#302,.T.);
#5384=EDGE_CURVE('',#4181,#4207,#2482,.T.);
#5385=EDGE_CURVE('',#4207,#4208,#2483,.T.);
#5386=EDGE_CURVE('',#4208,#4179,#2484,.T.);
#5387=EDGE_CURVE('',#4188,#4181,#2485,.T.);
#5388=EDGE_CURVE('',#4179,#4203,#2486,.T.);
#5389=EDGE_CURVE('',#4193,#4186,#303,.F.);
#5390=EDGE_CURVE('',#4192,#4209,#2487,.T.);
#5391=EDGE_CURVE('',#4209,#4207,#2488,.T.);
#5392=EDGE_CURVE('',#4207,#4188,#2489,.T.);
#5393=EDGE_CURVE('',#4191,#4210,#2490,.T.);
#5394=EDGE_CURVE('',#4210,#4211,#2491,.T.);
#5395=EDGE_CURVE('',#4211,#4192,#2492,.T.);
#5396=EDGE_CURVE('',#4190,#4212,#2493,.T.);
#5397=EDGE_CURVE('',#4212,#4213,#2494,.T.);
#5398=EDGE_CURVE('',#4213,#4191,#2495,.T.);
#5399=EDGE_CURVE('',#4214,#4202,#2496,.T.);
#5400=EDGE_CURVE('',#4212,#4214,#2497,.T.);
#5401=EDGE_CURVE('',#4116,#4163,#304,.T.);
#5402=EDGE_CURVE('',#4162,#4117,#305,.T.);
#5403=EDGE_CURVE('',#4215,#4215,#3582,.T.);
#5404=EDGE_CURVE('',#4215,#4187,#2498,.T.);
#5405=EDGE_CURVE('',#4204,#4198,#306,.F.);
#5406=EDGE_CURVE('',#4203,#4208,#2499,.T.);
#5407=EDGE_CURVE('',#4208,#4216,#2500,.T.);
#5408=EDGE_CURVE('',#4216,#4200,#2501,.T.);
#5409=EDGE_CURVE('',#4201,#4217,#2502,.T.);
#5410=EDGE_CURVE('',#4217,#4214,#2503,.T.);
#5411=EDGE_CURVE('',#4200,#4218,#2504,.T.);
#5412=EDGE_CURVE('',#4218,#4219,#2505,.T.);
#5413=EDGE_CURVE('',#4219,#4201,#2506,.T.);
#5414=EDGE_CURVE('',#4220,#4220,#3583,.T.);
#5415=EDGE_CURVE('',#4220,#4199,#2507,.T.);
#5416=EDGE_CURVE('',#4221,#4222,#307,.T.);
#5417=EDGE_CURVE('',#4222,#4223,#308,.T.);
#5418=EDGE_CURVE('',#4223,#4224,#309,.T.);
#5419=EDGE_CURVE('',#4224,#4225,#310,.T.);
#5420=EDGE_CURVE('',#4225,#4226,#311,.T.);
#5421=EDGE_CURVE('',#4226,#4227,#312,.T.);
#5422=EDGE_CURVE('',#4227,#4228,#313,.T.);
#5423=EDGE_CURVE('',#4228,#4229,#314,.T.);
#5424=EDGE_CURVE('',#4229,#4230,#315,.T.);
#5425=EDGE_CURVE('',#4230,#4231,#316,.T.);
#5426=EDGE_CURVE('',#4232,#4231,#3584,.T.);
#5427=EDGE_CURVE('',#4232,#4233,#317,.T.);
#5428=EDGE_CURVE('',#4233,#4234,#318,.T.);
#5429=EDGE_CURVE('',#4234,#4235,#319,.T.);
#5430=EDGE_CURVE('',#4235,#4236,#320,.T.);
#5431=EDGE_CURVE('',#4236,#4237,#321,.T.);
#5432=EDGE_CURVE('',#4237,#4238,#322,.T.);
#5433=EDGE_CURVE('',#4238,#4239,#323,.T.);
#5434=EDGE_CURVE('',#4239,#4240,#324,.T.);
#5435=EDGE_CURVE('',#4240,#4241,#325,.T.);
#5436=EDGE_CURVE('',#4241,#4242,#326,.T.);
#5437=EDGE_CURVE('',#4242,#4206,#327,.T.);
#5438=EDGE_CURVE('',#4205,#4221,#328,.T.);
#5439=EDGE_CURVE('',#4243,#4244,#3585,.T.);
#5440=EDGE_CURVE('',#4244,#4205,#329,.T.);
#5441=EDGE_CURVE('',#4206,#4243,#330,.T.);
#5442=EDGE_CURVE('',#4079,#4135,#331,.T.);
#5443=EDGE_CURVE('',#4134,#4080,#332,.T.);
#5444=EDGE_CURVE('',#4216,#4209,#2508,.T.);
#5445=EDGE_CURVE('',#4209,#4211,#2509,.T.);
#5446=EDGE_CURVE('',#4211,#4218,#2510,.T.);
#5447=EDGE_CURVE('',#4219,#4210,#2511,.T.);
#5448=EDGE_CURVE('',#4245,#4245,#3586,.T.);
#5449=EDGE_CURVE('',#4246,#4246,#3587,.T.);
#5450=EDGE_CURVE('',#4210,#4213,#2512,.T.);
#5451=EDGE_CURVE('',#4213,#4217,#2513,.T.);
#5452=EDGE_CURVE('',#4115,#4247,#333,.T.);
#5453=EDGE_CURVE('',#4247,#4112,#334,.T.);
#5454=EDGE_CURVE('',#4114,#4111,#335,.F.);
#5455=EDGE_CURVE('',#4084,#4139,#336,.T.);
#5456=EDGE_CURVE('',#4138,#4085,#337,.T.);
#5457=EDGE_CURVE('',#4220,#4215,#2514,.T.);
#5458=EDGE_CURVE('',#4248,#4249,#338,.T.);
#5459=EDGE_CURVE('',#4249,#4250,#339,.T.);
#5460=EDGE_CURVE('',#4250,#4251,#340,.T.);
#5461=EDGE_CURVE('',#4251,#4252,#341,.T.);
#5462=EDGE_CURVE('',#4252,#4060,#342,.T.);
#5463=EDGE_CURVE('',#4059,#4253,#343,.T.);
#5464=EDGE_CURVE('',#4253,#4254,#344,.T.);
#5465=EDGE_CURVE('',#4254,#4255,#345,.T.);
#5466=EDGE_CURVE('',#4255,#4256,#705,.T.);
#5467=EDGE_CURVE('',#4256,#4257,#346,.T.);
#5468=EDGE_CURVE('',#4257,#4258,#2515,.T.);
#5469=EDGE_CURVE('',#4258,#4259,#347,.T.);
#5470=EDGE_CURVE('',#4259,#4260,#706,.T.);
#5471=EDGE_CURVE('',#4260,#4261,#348,.T.);
#5472=EDGE_CURVE('',#4261,#4262,#349,.T.);
#5473=EDGE_CURVE('',#4262,#4121,#350,.T.);
#5474=EDGE_CURVE('',#4120,#4263,#351,.T.);
#5475=EDGE_CURVE('',#4263,#4264,#707,.T.);
#5476=EDGE_CURVE('',#4264,#4265,#352,.T.);
#5477=EDGE_CURVE('',#4265,#4266,#353,.T.);
#5478=EDGE_CURVE('',#4266,#4267,#354,.T.);
#5479=EDGE_CURVE('',#4267,#4268,#2516,.T.);
#5480=EDGE_CURVE('',#4268,#4248,#708,.T.);
#5481=EDGE_CURVE('',#4218,#4216,#2517,.T.);
#5482=EDGE_CURVE('',#4217,#4219,#2518,.T.);
#5483=EDGE_CURVE('',#4231,#4269,#355,.T.);
#5484=EDGE_CURVE('',#4244,#4270,#356,.F.);
#5485=EDGE_CURVE('',#4270,#4271,#357,.F.);
#5486=EDGE_CURVE('',#4271,#4272,#358,.F.);
#5487=EDGE_CURVE('',#4272,#4273,#359,.F.);
#5488=EDGE_CURVE('',#4273,#4274,#360,.F.);
#5489=EDGE_CURVE('',#4274,#4275,#361,.F.);
#5490=EDGE_CURVE('',#4275,#4276,#362,.F.);
#5491=EDGE_CURVE('',#4276,#4277,#363,.F.);
#5492=EDGE_CURVE('',#4277,#4278,#364,.F.);
#5493=EDGE_CURVE('',#4278,#4279,#365,.F.);
#5494=EDGE_CURVE('',#4279,#4269,#366,.F.);
#5495=EDGE_CURVE('',#4280,#4232,#367,.T.);
#5496=EDGE_CURVE('',#4281,#4280,#368,.T.);
#5497=EDGE_CURVE('',#4282,#4281,#369,.T.);
#5498=EDGE_CURVE('',#4283,#4282,#370,.F.);
#5499=EDGE_CURVE('',#4284,#4283,#371,.F.);
#5500=EDGE_CURVE('',#4243,#4284,#372,.T.);
#5501=EDGE_CURVE('',#4231,#4285,#3588,.T.);
#5502=EDGE_CURVE('',#4285,#4245,#2519,.T.);
#5503=EDGE_CURVE('',#4285,#4232,#3589,.T.);
#5504=EDGE_CURVE('',#4269,#4280,#3590,.T.);
#5505=EDGE_CURVE('',#4252,#4263,#373,.F.);
#5506=EDGE_CURVE('',#4077,#4074,#374,.T.);
#5507=EDGE_CURVE('',#4286,#4075,#375,.T.);
#5508=EDGE_CURVE('',#4078,#4286,#376,.T.);
#5509=EDGE_CURVE('',#4253,#4262,#377,.T.);
#5510=EDGE_CURVE('',#4138,#4287,#3591,.T.);
#5511=EDGE_CURVE('',#4287,#4246,#2520,.T.);
#5512=EDGE_CURVE('',#4287,#4139,#3592,.T.);
#5513=EDGE_CURVE('',#4288,#4268,#3593,.T.);
#5514=EDGE_CURVE('',#4248,#4288,#378,.F.);
#5515=EDGE_CURVE('',#4267,#4288,#709,.T.);
#5516=EDGE_CURVE('',#4249,#4266,#379,.T.);
#5517=EDGE_CURVE('',#4265,#4250,#380,.T.);
#5518=EDGE_CURVE('',#4251,#4264,#381,.T.);
#5519=EDGE_CURVE('',#4261,#4254,#382,.T.);
#5520=EDGE_CURVE('',#4260,#4255,#383,.F.);
#5521=EDGE_CURVE('',#4259,#4256,#384,.T.);
#5522=EDGE_CURVE('',#4257,#4258,#385,.T.);
#7052=ORIENTED_EDGE('',*,*,#5179,.T.);
#7053=ORIENTED_EDGE('',*,*,#5180,.T.);
#7054=ORIENTED_EDGE('',*,*,#5181,.T.);
#7055=ORIENTED_EDGE('',*,*,#5182,.F.);
#7056=ORIENTED_EDGE('',*,*,#5183,.F.);
#7057=ORIENTED_EDGE('',*,*,#5184,.F.);
#7058=ORIENTED_EDGE('',*,*,#5185,.T.);
#7059=ORIENTED_EDGE('',*,*,#5186,.T.);
#7060=ORIENTED_EDGE('',*,*,#5187,.T.);
#7061=ORIENTED_EDGE('',*,*,#5179,.F.);
#7062=ORIENTED_EDGE('',*,*,#5188,.F.);
#7063=ORIENTED_EDGE('',*,*,#5189,.T.);
#7064=ORIENTED_EDGE('',*,*,#5190,.T.);
#7065=ORIENTED_EDGE('',*,*,#5185,.F.);
#7066=ORIENTED_EDGE('',*,*,#5191,.F.);
#7067=ORIENTED_EDGE('',*,*,#5192,.F.);
#7068=ORIENTED_EDGE('',*,*,#5193,.T.);
#7069=ORIENTED_EDGE('',*,*,#5194,.T.);
#7070=ORIENTED_EDGE('',*,*,#5189,.F.);
#7071=ORIENTED_EDGE('',*,*,#5195,.F.);
#7072=ORIENTED_EDGE('',*,*,#5196,.T.);
#7073=ORIENTED_EDGE('',*,*,#5197,.T.);
#7074=ORIENTED_EDGE('',*,*,#5193,.F.);
#7075=ORIENTED_EDGE('',*,*,#5198,.F.);
#7076=ORIENTED_EDGE('',*,*,#5199,.T.);
#7077=ORIENTED_EDGE('',*,*,#5200,.T.);
#7078=ORIENTED_EDGE('',*,*,#5196,.F.);
#7079=ORIENTED_EDGE('',*,*,#5201,.F.);
#7080=ORIENTED_EDGE('',*,*,#5202,.T.);
#7081=ORIENTED_EDGE('',*,*,#5203,.T.);
#7082=ORIENTED_EDGE('',*,*,#5204,.T.);
#7083=ORIENTED_EDGE('',*,*,#5199,.F.);
#7084=ORIENTED_EDGE('',*,*,#5205,.F.);
#7085=ORIENTED_EDGE('',*,*,#5206,.F.);
#7086=ORIENTED_EDGE('',*,*,#5207,.F.);
#7087=ORIENTED_EDGE('',*,*,#5208,.F.);
#7088=ORIENTED_EDGE('',*,*,#5209,.T.);
#7089=ORIENTED_EDGE('',*,*,#5210,.T.);
#7090=ORIENTED_EDGE('',*,*,#5211,.T.);
#7091=ORIENTED_EDGE('',*,*,#5212,.T.);
#7092=ORIENTED_EDGE('',*,*,#5213,.F.);
#7093=ORIENTED_EDGE('',*,*,#5214,.F.);
#7094=ORIENTED_EDGE('',*,*,#5215,.T.);
#7095=ORIENTED_EDGE('',*,*,#5216,.T.);
#7096=ORIENTED_EDGE('',*,*,#5217,.T.);
#7097=ORIENTED_EDGE('',*,*,#5210,.F.);
#7098=ORIENTED_EDGE('',*,*,#5218,.F.);
#7099=ORIENTED_EDGE('',*,*,#5219,.F.);
#7100=ORIENTED_EDGE('',*,*,#5220,.T.);
#7101=ORIENTED_EDGE('',*,*,#5221,.T.);
#7102=ORIENTED_EDGE('',*,*,#5215,.F.);
#7103=ORIENTED_EDGE('',*,*,#5222,.F.);
#7104=ORIENTED_EDGE('',*,*,#5223,.T.);
#7105=ORIENTED_EDGE('',*,*,#5224,.T.);
#7106=ORIENTED_EDGE('',*,*,#5220,.F.);
#7107=ORIENTED_EDGE('',*,*,#5225,.F.);
#7108=ORIENTED_EDGE('',*,*,#5226,.T.);
#7109=ORIENTED_EDGE('',*,*,#5227,.T.);
#7110=ORIENTED_EDGE('',*,*,#5223,.F.);
#7111=ORIENTED_EDGE('',*,*,#5228,.F.);
#7112=ORIENTED_EDGE('',*,*,#5229,.T.);
#7113=ORIENTED_EDGE('',*,*,#5230,.T.);
#7114=ORIENTED_EDGE('',*,*,#5231,.T.);
#7115=ORIENTED_EDGE('',*,*,#5226,.F.);
#7116=ORIENTED_EDGE('',*,*,#5232,.F.);
#7117=ORIENTED_EDGE('',*,*,#5233,.F.);
#7118=ORIENTED_EDGE('',*,*,#5234,.T.);
#7119=ORIENTED_EDGE('',*,*,#5235,.T.);
#7120=ORIENTED_EDGE('',*,*,#5229,.F.);
#7121=ORIENTED_EDGE('',*,*,#5236,.F.);
#7122=ORIENTED_EDGE('',*,*,#5237,.T.);
#7123=ORIENTED_EDGE('',*,*,#5238,.T.);
#7124=ORIENTED_EDGE('',*,*,#5234,.F.);
#7125=ORIENTED_EDGE('',*,*,#5239,.F.);
#7126=ORIENTED_EDGE('',*,*,#5240,.T.);
#7127=ORIENTED_EDGE('',*,*,#5241,.T.);
#7128=ORIENTED_EDGE('',*,*,#5237,.F.);
#7129=ORIENTED_EDGE('',*,*,#5242,.F.);
#7130=ORIENTED_EDGE('',*,*,#5243,.T.);
#7131=ORIENTED_EDGE('',*,*,#5244,.T.);
#7132=ORIENTED_EDGE('',*,*,#5240,.F.);
#7133=ORIENTED_EDGE('',*,*,#5245,.F.);
#7134=ORIENTED_EDGE('',*,*,#5246,.T.);
#7135=ORIENTED_EDGE('',*,*,#5247,.T.);
#7136=ORIENTED_EDGE('',*,*,#5243,.F.);
#7137=ORIENTED_EDGE('',*,*,#5248,.F.);
#7138=ORIENTED_EDGE('',*,*,#5249,.F.);
#7139=ORIENTED_EDGE('',*,*,#5250,.T.);
#7140=ORIENTED_EDGE('',*,*,#5251,.T.);
#7141=ORIENTED_EDGE('',*,*,#5252,.T.);
#7142=ORIENTED_EDGE('',*,*,#5246,.F.);
#7143=ORIENTED_EDGE('',*,*,#5253,.F.);
#7144=ORIENTED_EDGE('',*,*,#5254,.F.);
#7145=ORIENTED_EDGE('',*,*,#5255,.F.);
#7146=ORIENTED_EDGE('',*,*,#5256,.F.);
#7147=ORIENTED_EDGE('',*,*,#5257,.T.);
#7148=ORIENTED_EDGE('',*,*,#5258,.T.);
#7149=ORIENTED_EDGE('',*,*,#5259,.T.);
#7150=ORIENTED_EDGE('',*,*,#5260,.F.);
#7151=ORIENTED_EDGE('',*,*,#5261,.T.);
#7152=ORIENTED_EDGE('',*,*,#5262,.T.);
#7153=ORIENTED_EDGE('',*,*,#5263,.T.);
#7154=ORIENTED_EDGE('',*,*,#5258,.F.);
#7155=ORIENTED_EDGE('',*,*,#5264,.T.);
#7156=ORIENTED_EDGE('',*,*,#5265,.T.);
#7157=ORIENTED_EDGE('',*,*,#5266,.T.);
#7158=ORIENTED_EDGE('',*,*,#5262,.F.);
#7159=ORIENTED_EDGE('',*,*,#5267,.T.);
#7160=ORIENTED_EDGE('',*,*,#5268,.T.);
#7161=ORIENTED_EDGE('',*,*,#5269,.T.);
#7162=ORIENTED_EDGE('',*,*,#5265,.F.);
#7163=ORIENTED_EDGE('',*,*,#5270,.T.);
#7164=ORIENTED_EDGE('',*,*,#5271,.T.);
#7165=ORIENTED_EDGE('',*,*,#5272,.T.);
#7166=ORIENTED_EDGE('',*,*,#5268,.F.);
#7167=ORIENTED_EDGE('',*,*,#5273,.T.);
#7168=ORIENTED_EDGE('',*,*,#5274,.T.);
#7169=ORIENTED_EDGE('',*,*,#5275,.T.);
#7170=ORIENTED_EDGE('',*,*,#5271,.F.);
#7171=ORIENTED_EDGE('',*,*,#5276,.T.);
#7172=ORIENTED_EDGE('',*,*,#5277,.F.);
#7173=ORIENTED_EDGE('',*,*,#5278,.T.);
#7174=ORIENTED_EDGE('',*,*,#5279,.F.);
#7175=ORIENTED_EDGE('',*,*,#5280,.T.);
#7176=ORIENTED_EDGE('',*,*,#5281,.T.);
#7177=ORIENTED_EDGE('',*,*,#5282,.T.);
#7178=ORIENTED_EDGE('',*,*,#5283,.F.);
#7179=ORIENTED_EDGE('',*,*,#5284,.T.);
#7180=ORIENTED_EDGE('',*,*,#5285,.T.);
#7181=ORIENTED_EDGE('',*,*,#5286,.T.);
#7182=ORIENTED_EDGE('',*,*,#5281,.F.);
#7183=ORIENTED_EDGE('',*,*,#5287,.T.);
#7184=ORIENTED_EDGE('',*,*,#5288,.T.);
#7185=ORIENTED_EDGE('',*,*,#5289,.T.);
#7186=ORIENTED_EDGE('',*,*,#5285,.F.);
#7187=ORIENTED_EDGE('',*,*,#5290,.T.);
#7188=ORIENTED_EDGE('',*,*,#5291,.T.);
#7189=ORIENTED_EDGE('',*,*,#5292,.T.);
#7190=ORIENTED_EDGE('',*,*,#5288,.F.);
#7191=ORIENTED_EDGE('',*,*,#5293,.T.);
#7192=ORIENTED_EDGE('',*,*,#5294,.T.);
#7193=ORIENTED_EDGE('',*,*,#5295,.T.);
#7194=ORIENTED_EDGE('',*,*,#5291,.F.);
#7195=ORIENTED_EDGE('',*,*,#5296,.T.);
#7196=ORIENTED_EDGE('',*,*,#5297,.T.);
#7197=ORIENTED_EDGE('',*,*,#5298,.T.);
#7198=ORIENTED_EDGE('',*,*,#5294,.F.);
#7199=ORIENTED_EDGE('',*,*,#5299,.T.);
#7200=ORIENTED_EDGE('',*,*,#5300,.T.);
#7201=ORIENTED_EDGE('',*,*,#5301,.T.);
#7202=ORIENTED_EDGE('',*,*,#5297,.F.);
#7203=ORIENTED_EDGE('',*,*,#5302,.T.);
#7204=ORIENTED_EDGE('',*,*,#5303,.T.);
#7205=ORIENTED_EDGE('',*,*,#5304,.T.);
#7206=ORIENTED_EDGE('',*,*,#5300,.F.);
#7207=ORIENTED_EDGE('',*,*,#5305,.T.);
#7208=ORIENTED_EDGE('',*,*,#5306,.T.);
#7209=ORIENTED_EDGE('',*,*,#5307,.T.);
#7210=ORIENTED_EDGE('',*,*,#5303,.F.);
#7211=ORIENTED_EDGE('',*,*,#5308,.T.);
#7212=ORIENTED_EDGE('',*,*,#5309,.T.);
#7213=ORIENTED_EDGE('',*,*,#5310,.T.);
#7214=ORIENTED_EDGE('',*,*,#5306,.F.);
#7215=ORIENTED_EDGE('',*,*,#5311,.T.);
#7216=ORIENTED_EDGE('',*,*,#5312,.T.);
#7217=ORIENTED_EDGE('',*,*,#5313,.T.);
#7218=ORIENTED_EDGE('',*,*,#5309,.F.);
#7219=ORIENTED_EDGE('',*,*,#5314,.T.);
#7220=ORIENTED_EDGE('',*,*,#5315,.F.);
#7221=ORIENTED_EDGE('',*,*,#5316,.T.);
#7222=ORIENTED_EDGE('',*,*,#5317,.F.);
#7223=ORIENTED_EDGE('',*,*,#5318,.T.);
#7224=ORIENTED_EDGE('',*,*,#5315,.T.);
#7225=ORIENTED_EDGE('',*,*,#5319,.T.);
#7226=ORIENTED_EDGE('',*,*,#5312,.F.);
#7227=ORIENTED_EDGE('',*,*,#5320,.T.);
#7228=ORIENTED_EDGE('',*,*,#5277,.T.);
#7229=ORIENTED_EDGE('',*,*,#5321,.T.);
#7230=ORIENTED_EDGE('',*,*,#5274,.F.);
#7231=ORIENTED_EDGE('',*,*,#5322,.T.);
#7232=ORIENTED_EDGE('',*,*,#5323,.F.);
#7233=ORIENTED_EDGE('',*,*,#5324,.T.);
#7234=ORIENTED_EDGE('',*,*,#5325,.F.);
#7235=ORIENTED_EDGE('',*,*,#5326,.F.);
#7236=ORIENTED_EDGE('',*,*,#5327,.T.);
#7237=ORIENTED_EDGE('',*,*,#5326,.T.);
#7238=ORIENTED_EDGE('',*,*,#5328,.T.);
#7239=ORIENTED_EDGE('',*,*,#5329,.T.);
#7240=ORIENTED_EDGE('',*,*,#5330,.T.);
#7241=ORIENTED_EDGE('',*,*,#5331,.T.);
#7242=ORIENTED_EDGE('',*,*,#5332,.T.);
#7243=ORIENTED_EDGE('',*,*,#5325,.T.);
#7244=ORIENTED_EDGE('',*,*,#5333,.F.);
#7245=ORIENTED_EDGE('',*,*,#5334,.F.);
#7246=ORIENTED_EDGE('',*,*,#5330,.F.);
#7247=ORIENTED_EDGE('',*,*,#5324,.F.);
#7248=ORIENTED_EDGE('',*,*,#5335,.F.);
#7249=ORIENTED_EDGE('',*,*,#5336,.F.);
#7250=ORIENTED_EDGE('',*,*,#5337,.F.);
#7251=ORIENTED_EDGE('',*,*,#5338,.T.);
#7252=ORIENTED_EDGE('',*,*,#5339,.T.);
#7253=ORIENTED_EDGE('',*,*,#5335,.T.);
#7254=ORIENTED_EDGE('',*,*,#5323,.T.);
#7255=ORIENTED_EDGE('',*,*,#5340,.T.);
#7256=ORIENTED_EDGE('',*,*,#5341,.T.);
#7257=ORIENTED_EDGE('',*,*,#5342,.F.);
#7258=ORIENTED_EDGE('',*,*,#5343,.F.);
#7259=ORIENTED_EDGE('',*,*,#5329,.F.);
#7260=ORIENTED_EDGE('',*,*,#5344,.F.);
#7261=ORIENTED_EDGE('',*,*,#5345,.F.);
#7262=ORIENTED_EDGE('',*,*,#5346,.F.);
#7263=ORIENTED_EDGE('',*,*,#5347,.F.);
#7264=ORIENTED_EDGE('',*,*,#5348,.F.);
#7265=ORIENTED_EDGE('',*,*,#5349,.F.);
#7266=ORIENTED_EDGE('',*,*,#5350,.F.);
#7267=ORIENTED_EDGE('',*,*,#5328,.F.);
#7268=ORIENTED_EDGE('',*,*,#5332,.F.);
#7269=ORIENTED_EDGE('',*,*,#5340,.F.);
#7270=ORIENTED_EDGE('',*,*,#5327,.F.);
#7271=ORIENTED_EDGE('',*,*,#5351,.F.);
#7272=ORIENTED_EDGE('',*,*,#5352,.F.);
#7273=ORIENTED_EDGE('',*,*,#5353,.F.);
#7274=ORIENTED_EDGE('',*,*,#5354,.F.);
#7275=ORIENTED_EDGE('',*,*,#5331,.F.);
#7276=ORIENTED_EDGE('',*,*,#5334,.T.);
#7277=ORIENTED_EDGE('',*,*,#5355,.F.);
#7278=ORIENTED_EDGE('',*,*,#5356,.T.);
#7279=ORIENTED_EDGE('',*,*,#5357,.F.);
#7280=ORIENTED_EDGE('',*,*,#5358,.F.);
#7281=ORIENTED_EDGE('',*,*,#5359,.F.);
#7282=ORIENTED_EDGE('',*,*,#5360,.F.);
#7283=ORIENTED_EDGE('',*,*,#5361,.F.);
#7284=ORIENTED_EDGE('',*,*,#5362,.T.);
#7285=ORIENTED_EDGE('',*,*,#5339,.F.);
#7286=ORIENTED_EDGE('',*,*,#5362,.F.);
#7287=ORIENTED_EDGE('',*,*,#5363,.F.);
#7288=ORIENTED_EDGE('',*,*,#5338,.F.);
#7289=ORIENTED_EDGE('',*,*,#5364,.F.);
#7290=ORIENTED_EDGE('',*,*,#5365,.T.);
#7291=ORIENTED_EDGE('',*,*,#5337,.T.);
#7292=ORIENTED_EDGE('',*,*,#5366,.T.);
#7293=ORIENTED_EDGE('',*,*,#5367,.T.);
#7294=ORIENTED_EDGE('',*,*,#5364,.T.);
#7295=ORIENTED_EDGE('',*,*,#5368,.F.);
#7296=ORIENTED_EDGE('',*,*,#5369,.F.);
#7297=ORIENTED_EDGE('',*,*,#5370,.F.);
#7298=ORIENTED_EDGE('',*,*,#5371,.F.);
#7299=ORIENTED_EDGE('',*,*,#5372,.T.);
#7300=ORIENTED_EDGE('',*,*,#5366,.F.);
#7301=ORIENTED_EDGE('',*,*,#5336,.T.);
#7302=ORIENTED_EDGE('',*,*,#5341,.F.);
#7303=ORIENTED_EDGE('',*,*,#5373,.F.);
#7304=ORIENTED_EDGE('',*,*,#5374,.F.);
#7305=ORIENTED_EDGE('',*,*,#5375,.F.);
#7306=ORIENTED_EDGE('',*,*,#5376,.T.);
#7307=ORIENTED_EDGE('',*,*,#5355,.T.);
#7308=ORIENTED_EDGE('',*,*,#5333,.T.);
#7309=ORIENTED_EDGE('',*,*,#5363,.T.);
#7310=ORIENTED_EDGE('',*,*,#5361,.T.);
#7311=ORIENTED_EDGE('',*,*,#5377,.T.);
#7312=ORIENTED_EDGE('',*,*,#5349,.T.);
#7313=ORIENTED_EDGE('',*,*,#5377,.F.);
#7314=ORIENTED_EDGE('',*,*,#5378,.T.);
#7315=ORIENTED_EDGE('',*,*,#5379,.T.);
#7316=ORIENTED_EDGE('',*,*,#5380,.T.);
#7317=ORIENTED_EDGE('',*,*,#5348,.T.);
#7318=ORIENTED_EDGE('',*,*,#5380,.F.);
#7319=ORIENTED_EDGE('',*,*,#5279,.T.);
#7320=ORIENTED_EDGE('',*,*,#5381,.T.);
#7321=ORIENTED_EDGE('',*,*,#5382,.T.);
#7322=ORIENTED_EDGE('',*,*,#5346,.T.);
#7323=ORIENTED_EDGE('',*,*,#5383,.F.);
#7324=ORIENTED_EDGE('',*,*,#5347,.T.);
#7325=ORIENTED_EDGE('',*,*,#5382,.F.);
#7326=ORIENTED_EDGE('',*,*,#5383,.T.);
#7327=ORIENTED_EDGE('',*,*,#5345,.T.);
#7328=ORIENTED_EDGE('',*,*,#5384,.T.);
#7329=ORIENTED_EDGE('',*,*,#5385,.T.);
#7330=ORIENTED_EDGE('',*,*,#5386,.T.);
#7331=ORIENTED_EDGE('',*,*,#5342,.T.);
#7332=ORIENTED_EDGE('',*,*,#5350,.T.);
#7333=ORIENTED_EDGE('',*,*,#5354,.T.);
#7334=ORIENTED_EDGE('',*,*,#5387,.T.);
#7335=ORIENTED_EDGE('',*,*,#5344,.T.);
#7336=ORIENTED_EDGE('',*,*,#5388,.T.);
#7337=ORIENTED_EDGE('',*,*,#5373,.T.);
#7338=ORIENTED_EDGE('',*,*,#5351,.T.);
#7339=ORIENTED_EDGE('',*,*,#5343,.T.);
#7340=ORIENTED_EDGE('',*,*,#5389,.F.);
#7341=ORIENTED_EDGE('',*,*,#5359,.T.);
#7342=ORIENTED_EDGE('',*,*,#5390,.T.);
#7343=ORIENTED_EDGE('',*,*,#5391,.T.);
#7344=ORIENTED_EDGE('',*,*,#5392,.T.);
#7345=ORIENTED_EDGE('',*,*,#5353,.T.);
#7346=ORIENTED_EDGE('',*,*,#5393,.T.);
#7347=ORIENTED_EDGE('',*,*,#5394,.T.);
#7348=ORIENTED_EDGE('',*,*,#5395,.T.);
#7349=ORIENTED_EDGE('',*,*,#5358,.T.);
#7350=ORIENTED_EDGE('',*,*,#5396,.T.);
#7351=ORIENTED_EDGE('',*,*,#5397,.T.);
#7352=ORIENTED_EDGE('',*,*,#5398,.T.);
#7353=ORIENTED_EDGE('',*,*,#5357,.T.);
#7354=ORIENTED_EDGE('',*,*,#5376,.F.);
#7355=ORIENTED_EDGE('',*,*,#5365,.F.);
#7356=ORIENTED_EDGE('',*,*,#5367,.F.);
#7357=ORIENTED_EDGE('',*,*,#5372,.F.);
#7358=ORIENTED_EDGE('',*,*,#5399,.F.);
#7359=ORIENTED_EDGE('',*,*,#5400,.F.);
#7360=ORIENTED_EDGE('',*,*,#5396,.F.);
#7361=ORIENTED_EDGE('',*,*,#5356,.F.);
#7362=ORIENTED_EDGE('',*,*,#5401,.T.);
#7363=ORIENTED_EDGE('',*,*,#5317,.T.);
#7364=ORIENTED_EDGE('',*,*,#5402,.T.);
#7365=ORIENTED_EDGE('',*,*,#5256,.T.);
#7366=ORIENTED_EDGE('',*,*,#5403,.T.);
#7367=ORIENTED_EDGE('',*,*,#5404,.T.);
#7368=ORIENTED_EDGE('',*,*,#5360,.T.);
#7369=ORIENTED_EDGE('',*,*,#5389,.T.);
#7370=ORIENTED_EDGE('',*,*,#5352,.T.);
#7371=ORIENTED_EDGE('',*,*,#5404,.F.);
#7372=ORIENTED_EDGE('',*,*,#5405,.F.);
#7373=ORIENTED_EDGE('',*,*,#5374,.T.);
#7374=ORIENTED_EDGE('',*,*,#5406,.T.);
#7375=ORIENTED_EDGE('',*,*,#5407,.T.);
#7376=ORIENTED_EDGE('',*,*,#5408,.T.);
#7377=ORIENTED_EDGE('',*,*,#5369,.T.);
#7378=ORIENTED_EDGE('',*,*,#5399,.T.);
#7379=ORIENTED_EDGE('',*,*,#5371,.T.);
#7380=ORIENTED_EDGE('',*,*,#5409,.T.);
#7381=ORIENTED_EDGE('',*,*,#5410,.T.);
#7382=ORIENTED_EDGE('',*,*,#5411,.T.);
#7383=ORIENTED_EDGE('',*,*,#5412,.T.);
#7384=ORIENTED_EDGE('',*,*,#5413,.T.);
#7385=ORIENTED_EDGE('',*,*,#5370,.T.);
#7386=ORIENTED_EDGE('',*,*,#5414,.T.);
#7387=ORIENTED_EDGE('',*,*,#5415,.T.);
#7388=ORIENTED_EDGE('',*,*,#5375,.T.);
#7389=ORIENTED_EDGE('',*,*,#5405,.T.);
#7390=ORIENTED_EDGE('',*,*,#5368,.T.);
#7391=ORIENTED_EDGE('',*,*,#5415,.F.);
#7392=ORIENTED_EDGE('',*,*,#5416,.T.);
#7393=ORIENTED_EDGE('',*,*,#5417,.T.);
#7394=ORIENTED_EDGE('',*,*,#5418,.T.);
#7395=ORIENTED_EDGE('',*,*,#5419,.T.);
#7396=ORIENTED_EDGE('',*,*,#5420,.T.);
#7397=ORIENTED_EDGE('',*,*,#5421,.T.);
#7398=ORIENTED_EDGE('',*,*,#5422,.T.);
#7399=ORIENTED_EDGE('',*,*,#5423,.T.);
#7400=ORIENTED_EDGE('',*,*,#5424,.T.);
#7401=ORIENTED_EDGE('',*,*,#5425,.T.);
#7402=ORIENTED_EDGE('',*,*,#5426,.F.);
#7403=ORIENTED_EDGE('',*,*,#5427,.T.);
#7404=ORIENTED_EDGE('',*,*,#5428,.T.);
#7405=ORIENTED_EDGE('',*,*,#5429,.T.);
#7406=ORIENTED_EDGE('',*,*,#5430,.T.);
#7407=ORIENTED_EDGE('',*,*,#5431,.T.);
#7408=ORIENTED_EDGE('',*,*,#5432,.T.);
#7409=ORIENTED_EDGE('',*,*,#5433,.T.);
#7410=ORIENTED_EDGE('',*,*,#5434,.T.);
#7411=ORIENTED_EDGE('',*,*,#5435,.T.);
#7412=ORIENTED_EDGE('',*,*,#5436,.T.);
#7413=ORIENTED_EDGE('',*,*,#5437,.T.);
#7414=ORIENTED_EDGE('',*,*,#5378,.F.);
#7415=ORIENTED_EDGE('',*,*,#5438,.T.);
#7416=ORIENTED_EDGE('',*,*,#5439,.T.);
#7417=ORIENTED_EDGE('',*,*,#5440,.T.);
#7418=ORIENTED_EDGE('',*,*,#5379,.F.);
#7419=ORIENTED_EDGE('',*,*,#5441,.T.);
#7420=ORIENTED_EDGE('',*,*,#5208,.T.);
#7421=ORIENTED_EDGE('',*,*,#5442,.T.);
#7422=ORIENTED_EDGE('',*,*,#5381,.F.);
#7423=ORIENTED_EDGE('',*,*,#5443,.T.);
#7424=ORIENTED_EDGE('',*,*,#5406,.F.);
#7425=ORIENTED_EDGE('',*,*,#5388,.F.);
#7426=ORIENTED_EDGE('',*,*,#5386,.F.);
#7427=ORIENTED_EDGE('',*,*,#5385,.F.);
#7428=ORIENTED_EDGE('',*,*,#5391,.F.);
#7429=ORIENTED_EDGE('',*,*,#5444,.F.);
#7430=ORIENTED_EDGE('',*,*,#5407,.F.);
#7431=ORIENTED_EDGE('',*,*,#5392,.F.);
#7432=ORIENTED_EDGE('',*,*,#5384,.F.);
#7433=ORIENTED_EDGE('',*,*,#5387,.F.);
#7434=ORIENTED_EDGE('',*,*,#5445,.F.);
#7435=ORIENTED_EDGE('',*,*,#5390,.F.);
#7436=ORIENTED_EDGE('',*,*,#5395,.F.);
#7437=ORIENTED_EDGE('',*,*,#5446,.F.);
#7438=ORIENTED_EDGE('',*,*,#5394,.F.);
#7439=ORIENTED_EDGE('',*,*,#5447,.F.);
#7440=ORIENTED_EDGE('',*,*,#5412,.F.);
#7441=ORIENTED_EDGE('',*,*,#5448,.F.);
#7442=ORIENTED_EDGE('',*,*,#5449,.F.);
#7443=ORIENTED_EDGE('',*,*,#5393,.F.);
#7444=ORIENTED_EDGE('',*,*,#5398,.F.);
#7445=ORIENTED_EDGE('',*,*,#5450,.F.);
#7446=ORIENTED_EDGE('',*,*,#5410,.F.);
#7447=ORIENTED_EDGE('',*,*,#5451,.F.);
#7448=ORIENTED_EDGE('',*,*,#5397,.F.);
#7449=ORIENTED_EDGE('',*,*,#5400,.T.);
#7450=ORIENTED_EDGE('',*,*,#5254,.T.);
#7451=ORIENTED_EDGE('',*,*,#5452,.T.);
#7452=ORIENTED_EDGE('',*,*,#5453,.T.);
#7453=ORIENTED_EDGE('',*,*,#5250,.F.);
#7454=ORIENTED_EDGE('',*,*,#5454,.F.);
#7455=ORIENTED_EDGE('',*,*,#5455,.F.);
#7456=ORIENTED_EDGE('',*,*,#5212,.F.);
#7457=ORIENTED_EDGE('',*,*,#5211,.F.);
#7458=ORIENTED_EDGE('',*,*,#5217,.F.);
#7459=ORIENTED_EDGE('',*,*,#5216,.F.);
#7460=ORIENTED_EDGE('',*,*,#5221,.F.);
#7461=ORIENTED_EDGE('',*,*,#5224,.F.);
#7462=ORIENTED_EDGE('',*,*,#5227,.F.);
#7463=ORIENTED_EDGE('',*,*,#5231,.F.);
#7464=ORIENTED_EDGE('',*,*,#5230,.F.);
#7465=ORIENTED_EDGE('',*,*,#5235,.F.);
#7466=ORIENTED_EDGE('',*,*,#5238,.F.);
#7467=ORIENTED_EDGE('',*,*,#5241,.F.);
#7468=ORIENTED_EDGE('',*,*,#5244,.F.);
#7469=ORIENTED_EDGE('',*,*,#5247,.F.);
#7470=ORIENTED_EDGE('',*,*,#5252,.F.);
#7471=ORIENTED_EDGE('',*,*,#5251,.F.);
#7472=ORIENTED_EDGE('',*,*,#5453,.F.);
#7473=ORIENTED_EDGE('',*,*,#5452,.F.);
#7474=ORIENTED_EDGE('',*,*,#5257,.F.);
#7475=ORIENTED_EDGE('',*,*,#5402,.F.);
#7476=ORIENTED_EDGE('',*,*,#5316,.F.);
#7477=ORIENTED_EDGE('',*,*,#5320,.F.);
#7478=ORIENTED_EDGE('',*,*,#5314,.F.);
#7479=ORIENTED_EDGE('',*,*,#5311,.F.);
#7480=ORIENTED_EDGE('',*,*,#5308,.F.);
#7481=ORIENTED_EDGE('',*,*,#5305,.F.);
#7482=ORIENTED_EDGE('',*,*,#5302,.F.);
#7483=ORIENTED_EDGE('',*,*,#5299,.F.);
#7484=ORIENTED_EDGE('',*,*,#5296,.F.);
#7485=ORIENTED_EDGE('',*,*,#5293,.F.);
#7486=ORIENTED_EDGE('',*,*,#5290,.F.);
#7487=ORIENTED_EDGE('',*,*,#5287,.F.);
#7488=ORIENTED_EDGE('',*,*,#5284,.F.);
#7489=ORIENTED_EDGE('',*,*,#5456,.F.);
#7490=ORIENTED_EDGE('',*,*,#5282,.F.);
#7491=ORIENTED_EDGE('',*,*,#5286,.F.);
#7492=ORIENTED_EDGE('',*,*,#5289,.F.);
#7493=ORIENTED_EDGE('',*,*,#5292,.F.);
#7494=ORIENTED_EDGE('',*,*,#5295,.F.);
#7495=ORIENTED_EDGE('',*,*,#5298,.F.);
#7496=ORIENTED_EDGE('',*,*,#5301,.F.);
#7497=ORIENTED_EDGE('',*,*,#5304,.F.);
#7498=ORIENTED_EDGE('',*,*,#5307,.F.);
#7499=ORIENTED_EDGE('',*,*,#5310,.F.);
#7500=ORIENTED_EDGE('',*,*,#5313,.F.);
#7501=ORIENTED_EDGE('',*,*,#5319,.F.);
#7502=ORIENTED_EDGE('',*,*,#5318,.F.);
#7503=ORIENTED_EDGE('',*,*,#5401,.F.);
#7504=ORIENTED_EDGE('',*,*,#5255,.T.);
#7505=ORIENTED_EDGE('',*,*,#5454,.T.);
#7506=ORIENTED_EDGE('',*,*,#5253,.T.);
#7507=ORIENTED_EDGE('',*,*,#5249,.T.);
#7508=ORIENTED_EDGE('',*,*,#5248,.T.);
#7509=ORIENTED_EDGE('',*,*,#5245,.T.);
#7510=ORIENTED_EDGE('',*,*,#5242,.T.);
#7511=ORIENTED_EDGE('',*,*,#5239,.T.);
#7512=ORIENTED_EDGE('',*,*,#5236,.T.);
#7513=ORIENTED_EDGE('',*,*,#5233,.T.);
#7514=ORIENTED_EDGE('',*,*,#5232,.T.);
#7515=ORIENTED_EDGE('',*,*,#5228,.T.);
#7516=ORIENTED_EDGE('',*,*,#5225,.T.);
#7517=ORIENTED_EDGE('',*,*,#5222,.T.);
#7518=ORIENTED_EDGE('',*,*,#5219,.T.);
#7519=ORIENTED_EDGE('',*,*,#5218,.T.);
#7520=ORIENTED_EDGE('',*,*,#5214,.T.);
#7521=ORIENTED_EDGE('',*,*,#5414,.F.);
#7522=ORIENTED_EDGE('',*,*,#5457,.T.);
#7523=ORIENTED_EDGE('',*,*,#5403,.F.);
#7524=ORIENTED_EDGE('',*,*,#5457,.F.);
#7525=ORIENTED_EDGE('',*,*,#5458,.T.);
#7526=ORIENTED_EDGE('',*,*,#5459,.T.);
#7527=ORIENTED_EDGE('',*,*,#5460,.T.);
#7528=ORIENTED_EDGE('',*,*,#5461,.T.);
#7529=ORIENTED_EDGE('',*,*,#5462,.T.);
#7530=ORIENTED_EDGE('',*,*,#5182,.T.);
#7531=ORIENTED_EDGE('',*,*,#5463,.T.);
#7532=ORIENTED_EDGE('',*,*,#5464,.T.);
#7533=ORIENTED_EDGE('',*,*,#5465,.T.);
#7534=ORIENTED_EDGE('',*,*,#5466,.T.);
#7535=ORIENTED_EDGE('',*,*,#5467,.T.);
#7536=ORIENTED_EDGE('',*,*,#5468,.T.);
#7537=ORIENTED_EDGE('',*,*,#5469,.T.);
#7538=ORIENTED_EDGE('',*,*,#5470,.T.);
#7539=ORIENTED_EDGE('',*,*,#5471,.T.);
#7540=ORIENTED_EDGE('',*,*,#5472,.T.);
#7541=ORIENTED_EDGE('',*,*,#5473,.T.);
#7542=ORIENTED_EDGE('',*,*,#5260,.T.);
#7543=ORIENTED_EDGE('',*,*,#5474,.T.);
#7544=ORIENTED_EDGE('',*,*,#5475,.T.);
#7545=ORIENTED_EDGE('',*,*,#5476,.T.);
#7546=ORIENTED_EDGE('',*,*,#5477,.T.);
#7547=ORIENTED_EDGE('',*,*,#5478,.T.);
#7548=ORIENTED_EDGE('',*,*,#5479,.T.);
#7549=ORIENTED_EDGE('',*,*,#5480,.T.);
#7550=ORIENTED_EDGE('',*,*,#5411,.F.);
#7551=ORIENTED_EDGE('',*,*,#5408,.F.);
#7552=ORIENTED_EDGE('',*,*,#5481,.F.);
#7553=ORIENTED_EDGE('',*,*,#5482,.F.);
#7554=ORIENTED_EDGE('',*,*,#5409,.F.);
#7555=ORIENTED_EDGE('',*,*,#5413,.F.);
#7556=ORIENTED_EDGE('',*,*,#5483,.F.);
#7557=ORIENTED_EDGE('',*,*,#5425,.F.);
#7558=ORIENTED_EDGE('',*,*,#5424,.F.);
#7559=ORIENTED_EDGE('',*,*,#5423,.F.);
#7560=ORIENTED_EDGE('',*,*,#5422,.F.);
#7561=ORIENTED_EDGE('',*,*,#5421,.F.);
#7562=ORIENTED_EDGE('',*,*,#5420,.F.);
#7563=ORIENTED_EDGE('',*,*,#5419,.F.);
#7564=ORIENTED_EDGE('',*,*,#5418,.F.);
#7565=ORIENTED_EDGE('',*,*,#5417,.F.);
#7566=ORIENTED_EDGE('',*,*,#5416,.F.);
#7567=ORIENTED_EDGE('',*,*,#5438,.F.);
#7568=ORIENTED_EDGE('',*,*,#5440,.F.);
#7569=ORIENTED_EDGE('',*,*,#5484,.T.);
#7570=ORIENTED_EDGE('',*,*,#5485,.T.);
#7571=ORIENTED_EDGE('',*,*,#5486,.T.);
#7572=ORIENTED_EDGE('',*,*,#5487,.T.);
#7573=ORIENTED_EDGE('',*,*,#5488,.T.);
#7574=ORIENTED_EDGE('',*,*,#5489,.T.);
#7575=ORIENTED_EDGE('',*,*,#5490,.T.);
#7576=ORIENTED_EDGE('',*,*,#5491,.T.);
#7577=ORIENTED_EDGE('',*,*,#5492,.T.);
#7578=ORIENTED_EDGE('',*,*,#5493,.T.);
#7579=ORIENTED_EDGE('',*,*,#5494,.T.);
#7580=ORIENTED_EDGE('',*,*,#5495,.F.);
#7581=ORIENTED_EDGE('',*,*,#5496,.F.);
#7582=ORIENTED_EDGE('',*,*,#5497,.F.);
#7583=ORIENTED_EDGE('',*,*,#5498,.F.);
#7584=ORIENTED_EDGE('',*,*,#5499,.F.);
#7585=ORIENTED_EDGE('',*,*,#5500,.F.);
#7586=ORIENTED_EDGE('',*,*,#5441,.F.);
#7587=ORIENTED_EDGE('',*,*,#5437,.F.);
#7588=ORIENTED_EDGE('',*,*,#5436,.F.);
#7589=ORIENTED_EDGE('',*,*,#5435,.F.);
#7590=ORIENTED_EDGE('',*,*,#5434,.F.);
#7591=ORIENTED_EDGE('',*,*,#5433,.F.);
#7592=ORIENTED_EDGE('',*,*,#5432,.F.);
#7593=ORIENTED_EDGE('',*,*,#5431,.F.);
#7594=ORIENTED_EDGE('',*,*,#5430,.F.);
#7595=ORIENTED_EDGE('',*,*,#5429,.F.);
#7596=ORIENTED_EDGE('',*,*,#5428,.F.);
#7597=ORIENTED_EDGE('',*,*,#5427,.F.);
#7598=ORIENTED_EDGE('',*,*,#5501,.T.);
#7599=ORIENTED_EDGE('',*,*,#5502,.T.);
#7600=ORIENTED_EDGE('',*,*,#5448,.T.);
#7601=ORIENTED_EDGE('',*,*,#5502,.F.);
#7602=ORIENTED_EDGE('',*,*,#5503,.T.);
#7603=ORIENTED_EDGE('',*,*,#5426,.T.);
#7604=ORIENTED_EDGE('',*,*,#5500,.T.);
#7605=ORIENTED_EDGE('',*,*,#5499,.T.);
#7606=ORIENTED_EDGE('',*,*,#5498,.T.);
#7607=ORIENTED_EDGE('',*,*,#5497,.T.);
#7608=ORIENTED_EDGE('',*,*,#5496,.T.);
#7609=ORIENTED_EDGE('',*,*,#5504,.F.);
#7610=ORIENTED_EDGE('',*,*,#5494,.F.);
#7611=ORIENTED_EDGE('',*,*,#5493,.F.);
#7612=ORIENTED_EDGE('',*,*,#5492,.F.);
#7613=ORIENTED_EDGE('',*,*,#5491,.F.);
#7614=ORIENTED_EDGE('',*,*,#5490,.F.);
#7615=ORIENTED_EDGE('',*,*,#5489,.F.);
#7616=ORIENTED_EDGE('',*,*,#5488,.F.);
#7617=ORIENTED_EDGE('',*,*,#5487,.F.);
#7618=ORIENTED_EDGE('',*,*,#5486,.F.);
#7619=ORIENTED_EDGE('',*,*,#5485,.F.);
#7620=ORIENTED_EDGE('',*,*,#5484,.F.);
#7621=ORIENTED_EDGE('',*,*,#5439,.F.);
#7622=ORIENTED_EDGE('',*,*,#5462,.F.);
#7623=ORIENTED_EDGE('',*,*,#5505,.T.);
#7624=ORIENTED_EDGE('',*,*,#5474,.F.);
#7625=ORIENTED_EDGE('',*,*,#5259,.F.);
#7626=ORIENTED_EDGE('',*,*,#5263,.F.);
#7627=ORIENTED_EDGE('',*,*,#5266,.F.);
#7628=ORIENTED_EDGE('',*,*,#5269,.F.);
#7629=ORIENTED_EDGE('',*,*,#5272,.F.);
#7630=ORIENTED_EDGE('',*,*,#5275,.F.);
#7631=ORIENTED_EDGE('',*,*,#5321,.F.);
#7632=ORIENTED_EDGE('',*,*,#5280,.F.);
#7633=ORIENTED_EDGE('',*,*,#5442,.F.);
#7634=ORIENTED_EDGE('',*,*,#5207,.T.);
#7635=ORIENTED_EDGE('',*,*,#5506,.T.);
#7636=ORIENTED_EDGE('',*,*,#5205,.T.);
#7637=ORIENTED_EDGE('',*,*,#5201,.T.);
#7638=ORIENTED_EDGE('',*,*,#5198,.T.);
#7639=ORIENTED_EDGE('',*,*,#5195,.T.);
#7640=ORIENTED_EDGE('',*,*,#5192,.T.);
#7641=ORIENTED_EDGE('',*,*,#5191,.T.);
#7642=ORIENTED_EDGE('',*,*,#5188,.T.);
#7643=ORIENTED_EDGE('',*,*,#5184,.T.);
#7644=ORIENTED_EDGE('',*,*,#5183,.T.);
#7645=ORIENTED_EDGE('',*,*,#5463,.F.);
#7646=ORIENTED_EDGE('',*,*,#5181,.F.);
#7647=ORIENTED_EDGE('',*,*,#5180,.F.);
#7648=ORIENTED_EDGE('',*,*,#5187,.F.);
#7649=ORIENTED_EDGE('',*,*,#5186,.F.);
#7650=ORIENTED_EDGE('',*,*,#5190,.F.);
#7651=ORIENTED_EDGE('',*,*,#5194,.F.);
#7652=ORIENTED_EDGE('',*,*,#5197,.F.);
#7653=ORIENTED_EDGE('',*,*,#5200,.F.);
#7654=ORIENTED_EDGE('',*,*,#5204,.F.);
#7655=ORIENTED_EDGE('',*,*,#5203,.F.);
#7656=ORIENTED_EDGE('',*,*,#5507,.F.);
#7657=ORIENTED_EDGE('',*,*,#5508,.F.);
#7658=ORIENTED_EDGE('',*,*,#5209,.F.);
#7659=ORIENTED_EDGE('',*,*,#5443,.F.);
#7660=ORIENTED_EDGE('',*,*,#5278,.F.);
#7661=ORIENTED_EDGE('',*,*,#5322,.F.);
#7662=ORIENTED_EDGE('',*,*,#5276,.F.);
#7663=ORIENTED_EDGE('',*,*,#5273,.F.);
#7664=ORIENTED_EDGE('',*,*,#5270,.F.);
#7665=ORIENTED_EDGE('',*,*,#5267,.F.);
#7666=ORIENTED_EDGE('',*,*,#5264,.F.);
#7667=ORIENTED_EDGE('',*,*,#5261,.F.);
#7668=ORIENTED_EDGE('',*,*,#5473,.F.);
#7669=ORIENTED_EDGE('',*,*,#5509,.F.);
#7670=ORIENTED_EDGE('',*,*,#5206,.T.);
#7671=ORIENTED_EDGE('',*,*,#5508,.T.);
#7672=ORIENTED_EDGE('',*,*,#5507,.T.);
#7673=ORIENTED_EDGE('',*,*,#5202,.F.);
#7674=ORIENTED_EDGE('',*,*,#5506,.F.);
#7675=ORIENTED_EDGE('',*,*,#5445,.T.);
#7676=ORIENTED_EDGE('',*,*,#5446,.T.);
#7677=ORIENTED_EDGE('',*,*,#5481,.T.);
#7678=ORIENTED_EDGE('',*,*,#5444,.T.);
#7679=ORIENTED_EDGE('',*,*,#5510,.T.);
#7680=ORIENTED_EDGE('',*,*,#5511,.T.);
#7681=ORIENTED_EDGE('',*,*,#5449,.T.);
#7682=ORIENTED_EDGE('',*,*,#5511,.F.);
#7683=ORIENTED_EDGE('',*,*,#5512,.T.);
#7684=ORIENTED_EDGE('',*,*,#5283,.T.);
#7685=ORIENTED_EDGE('',*,*,#5482,.T.);
#7686=ORIENTED_EDGE('',*,*,#5447,.T.);
#7687=ORIENTED_EDGE('',*,*,#5450,.T.);
#7688=ORIENTED_EDGE('',*,*,#5451,.T.);
#7689=ORIENTED_EDGE('',*,*,#5510,.F.);
#7690=ORIENTED_EDGE('',*,*,#5456,.T.);
#7691=ORIENTED_EDGE('',*,*,#5213,.T.);
#7692=ORIENTED_EDGE('',*,*,#5455,.T.);
#7693=ORIENTED_EDGE('',*,*,#5512,.F.);
#7694=ORIENTED_EDGE('',*,*,#5480,.F.);
#7695=ORIENTED_EDGE('',*,*,#5513,.F.);
#7696=ORIENTED_EDGE('',*,*,#5514,.F.);
#7697=ORIENTED_EDGE('',*,*,#5479,.F.);
#7698=ORIENTED_EDGE('',*,*,#5515,.T.);
#7699=ORIENTED_EDGE('',*,*,#5513,.T.);
#7700=ORIENTED_EDGE('',*,*,#5458,.F.);
#7701=ORIENTED_EDGE('',*,*,#5514,.T.);
#7702=ORIENTED_EDGE('',*,*,#5515,.F.);
#7703=ORIENTED_EDGE('',*,*,#5478,.F.);
#7704=ORIENTED_EDGE('',*,*,#5516,.F.);
#7705=ORIENTED_EDGE('',*,*,#5516,.T.);
#7706=ORIENTED_EDGE('',*,*,#5477,.F.);
#7707=ORIENTED_EDGE('',*,*,#5517,.T.);
#7708=ORIENTED_EDGE('',*,*,#5459,.F.);
#7709=ORIENTED_EDGE('',*,*,#5476,.F.);
#7710=ORIENTED_EDGE('',*,*,#5518,.F.);
#7711=ORIENTED_EDGE('',*,*,#5460,.F.);
#7712=ORIENTED_EDGE('',*,*,#5517,.F.);
#7713=ORIENTED_EDGE('',*,*,#5461,.F.);
#7714=ORIENTED_EDGE('',*,*,#5518,.T.);
#7715=ORIENTED_EDGE('',*,*,#5475,.F.);
#7716=ORIENTED_EDGE('',*,*,#5505,.F.);
#7717=ORIENTED_EDGE('',*,*,#5519,.T.);
#7718=ORIENTED_EDGE('',*,*,#5464,.F.);
#7719=ORIENTED_EDGE('',*,*,#5509,.T.);
#7720=ORIENTED_EDGE('',*,*,#5472,.F.);
#7721=ORIENTED_EDGE('',*,*,#5471,.F.);
#7722=ORIENTED_EDGE('',*,*,#5520,.T.);
#7723=ORIENTED_EDGE('',*,*,#5465,.F.);
#7724=ORIENTED_EDGE('',*,*,#5519,.F.);
#7725=ORIENTED_EDGE('',*,*,#5470,.F.);
#7726=ORIENTED_EDGE('',*,*,#5521,.T.);
#7727=ORIENTED_EDGE('',*,*,#5466,.F.);
#7728=ORIENTED_EDGE('',*,*,#5520,.F.);
#7729=ORIENTED_EDGE('',*,*,#5469,.F.);
#7730=ORIENTED_EDGE('',*,*,#5522,.F.);
#7731=ORIENTED_EDGE('',*,*,#5467,.F.);
#7732=ORIENTED_EDGE('',*,*,#5521,.F.);
#7733=ORIENTED_EDGE('',*,*,#5468,.F.);
#7734=ORIENTED_EDGE('',*,*,#5522,.T.);
#7735=ORIENTED_EDGE('',*,*,#5501,.F.);
#7736=ORIENTED_EDGE('',*,*,#5483,.T.);
#7737=ORIENTED_EDGE('',*,*,#5504,.T.);
#7738=ORIENTED_EDGE('',*,*,#5495,.T.);
#7739=ORIENTED_EDGE('',*,*,#5503,.F.);
#9186=CYLINDRICAL_SURFACE('',#10467,0.001543);
#9187=CYLINDRICAL_SURFACE('',#10468,0.001543);
#9188=CYLINDRICAL_SURFACE('',#10469,0.001543);
#9189=CYLINDRICAL_SURFACE('',#10470,0.001543);
#9190=CYLINDRICAL_SURFACE('',#10471,0.001543);
#9191=CYLINDRICAL_SURFACE('',#10472,0.001543);
#9192=CYLINDRICAL_SURFACE('',#10473,0.001543);
#9193=CYLINDRICAL_SURFACE('',#10474,0.001543);
#9194=CYLINDRICAL_SURFACE('',#10476,0.001543);
#9195=CYLINDRICAL_SURFACE('',#10478,0.001543);
#9196=CYLINDRICAL_SURFACE('',#10479,0.001543);
#9197=CYLINDRICAL_SURFACE('',#10480,0.001543);
#9198=CYLINDRICAL_SURFACE('',#10481,0.001543);
#9199=CYLINDRICAL_SURFACE('',#10482,0.001543);
#9200=CYLINDRICAL_SURFACE('',#10483,0.001543);
#9201=CYLINDRICAL_SURFACE('',#10484,0.001543);
#9202=CYLINDRICAL_SURFACE('',#10485,0.001543);
#9203=CYLINDRICAL_SURFACE('',#10486,0.001543);
#9204=CYLINDRICAL_SURFACE('',#10487,0.001543);
#9205=CYLINDRICAL_SURFACE('',#10488,0.001543);
#9206=CYLINDRICAL_SURFACE('',#10489,0.001543);
#9207=CYLINDRICAL_SURFACE('',#10491,0.0012645);
#9208=CYLINDRICAL_SURFACE('',#10492,0.0012645);
#9209=CYLINDRICAL_SURFACE('',#10493,0.0012645);
#9210=CYLINDRICAL_SURFACE('',#10494,0.0012645);
#9211=CYLINDRICAL_SURFACE('',#10495,0.0012645);
#9212=CYLINDRICAL_SURFACE('',#10496,0.0012645);
#9213=CYLINDRICAL_SURFACE('',#10497,0.0012645);
#9214=CYLINDRICAL_SURFACE('',#10499,0.0012645);
#9215=CYLINDRICAL_SURFACE('',#10501,0.0012645);
#9216=CYLINDRICAL_SURFACE('',#10502,0.0012645);
#9217=CYLINDRICAL_SURFACE('',#10503,0.0012645);
#9218=CYLINDRICAL_SURFACE('',#10504,0.0012645);
#9219=CYLINDRICAL_SURFACE('',#10505,0.0012645);
#9220=CYLINDRICAL_SURFACE('',#10506,0.0012645);
#9221=CYLINDRICAL_SURFACE('',#10507,0.0012645);
#9222=CYLINDRICAL_SURFACE('',#10508,0.0012645);
#9223=CYLINDRICAL_SURFACE('',#10509,0.0012645);
#9224=CYLINDRICAL_SURFACE('',#10510,0.0012645);
#9225=CYLINDRICAL_SURFACE('',#10511,0.0012645);
#9226=CYLINDRICAL_SURFACE('',#10513,0.0012645);
#9227=CYLINDRICAL_SURFACE('',#10514,0.0012645);
#9228=CYLINDRICAL_SURFACE('',#10532,0.0015);
#9229=CYLINDRICAL_SURFACE('',#10534,0.003);
#9230=CYLINDRICAL_SURFACE('',#10563,0.0025);
#9231=CYLINDRICAL_SURFACE('',#10577,0.001543);
#9232=CYLINDRICAL_SURFACE('',#10578,0.00155);
#9233=CYLINDRICAL_SURFACE('',#10588,0.003);
#9234=CYLINDRICAL_SURFACE('',#10590,0.001543);
#9235=CYLINDRICAL_SURFACE('',#10597,0.001543);
#9236=CYLINDRICAL_SURFACE('',#10601,0.0012645);
#9237=CYLINDRICAL_SURFACE('',#10602,0.001543);
#9238=CYLINDRICAL_SURFACE('',#10603,0.0012645);
#9239=CYLINDRICAL_SURFACE('',#10604,0.001543);
#9498=ADVANCED_FACE('',(#1276),#9186,.F.);
#9499=ADVANCED_FACE('',(#1277),#9187,.F.);
#9500=ADVANCED_FACE('',(#1278),#9188,.F.);
#9501=ADVANCED_FACE('',(#1279),#9189,.F.);
#9502=ADVANCED_FACE('',(#1280),#9190,.F.);
#9503=ADVANCED_FACE('',(#1281),#9191,.F.);
#9504=ADVANCED_FACE('',(#1282),#9192,.F.);
#9505=ADVANCED_FACE('',(#1283),#9193,.F.);
#9506=ADVANCED_FACE('',(#1284),#9194,.F.);
#9507=ADVANCED_FACE('',(#1285),#9195,.F.);
#9508=ADVANCED_FACE('',(#1286),#9196,.F.);
#9509=ADVANCED_FACE('',(#1287),#9197,.F.);
#9510=ADVANCED_FACE('',(#1288),#9198,.F.);
#9511=ADVANCED_FACE('',(#1289),#9199,.F.);
#9512=ADVANCED_FACE('',(#1290),#9200,.F.);
#9513=ADVANCED_FACE('',(#1291),#9201,.F.);
#9514=ADVANCED_FACE('',(#1292),#9202,.F.);
#9515=ADVANCED_FACE('',(#1293),#9203,.F.);
#9516=ADVANCED_FACE('',(#1294),#9204,.F.);
#9517=ADVANCED_FACE('',(#1295),#9205,.F.);
#9518=ADVANCED_FACE('',(#1296),#9206,.F.);
#9519=ADVANCED_FACE('',(#1297),#9207,.F.);
#9520=ADVANCED_FACE('',(#1298),#9208,.F.);
#9521=ADVANCED_FACE('',(#1299),#9209,.F.);
#9522=ADVANCED_FACE('',(#1300),#9210,.F.);
#9523=ADVANCED_FACE('',(#1301),#9211,.F.);
#9524=ADVANCED_FACE('',(#1302),#9212,.F.);
#9525=ADVANCED_FACE('',(#1303),#9213,.F.);
#9526=ADVANCED_FACE('',(#1304),#9214,.F.);
#9527=ADVANCED_FACE('',(#1305),#9215,.F.);
#9528=ADVANCED_FACE('',(#1306),#9216,.F.);
#9529=ADVANCED_FACE('',(#1307),#9217,.F.);
#9530=ADVANCED_FACE('',(#1308),#9218,.F.);
#9531=ADVANCED_FACE('',(#1309),#9219,.F.);
#9532=ADVANCED_FACE('',(#1310),#9220,.F.);
#9533=ADVANCED_FACE('',(#1311),#9221,.F.);
#9534=ADVANCED_FACE('',(#1312),#9222,.F.);
#9535=ADVANCED_FACE('',(#1313),#9223,.F.);
#9536=ADVANCED_FACE('',(#1314),#9224,.F.);
#9537=ADVANCED_FACE('',(#1315),#9225,.F.);
#9538=ADVANCED_FACE('',(#1316),#9226,.F.);
#9539=ADVANCED_FACE('',(#1317),#9227,.F.);
#9540=ADVANCED_FACE('',(#1318),#960,.T.);
#9541=ADVANCED_FACE('',(#1319),#961,.T.);
#9542=ADVANCED_FACE('',(#1320),#962,.T.);
#9543=ADVANCED_FACE('',(#1321,#741),#963,.F.);
#9544=ADVANCED_FACE('',(#1322),#964,.T.);
#9545=ADVANCED_FACE('',(#1323,#742,#743),#965,.F.);
#9546=ADVANCED_FACE('',(#1324),#966,.T.);
#9547=ADVANCED_FACE('',(#1325),#967,.T.);
#9548=ADVANCED_FACE('',(#1326),#968,.T.);
#9549=ADVANCED_FACE('',(#1327),#9228,.F.);
#9550=ADVANCED_FACE('',(#1328),#9229,.F.);
#9551=ADVANCED_FACE('',(#1329),#630,.F.);
#9552=ADVANCED_FACE('',(#1330),#969,.T.);
#9553=ADVANCED_FACE('',(#1331),#631,.F.);
#9554=ADVANCED_FACE('',(#1332),#632,.F.);
#9555=ADVANCED_FACE('',(#1333),#633,.F.);
#9556=ADVANCED_FACE('',(#1334),#634,.F.);
#9557=ADVANCED_FACE('',(#1335),#970,.T.);
#9558=ADVANCED_FACE('',(#1336),#971,.T.);
#9559=ADVANCED_FACE('',(#1337),#972,.T.);
#9560=ADVANCED_FACE('',(#1338),#973,.T.);
#9561=ADVANCED_FACE('',(#1339),#974,.T.);
#9562=ADVANCED_FACE('',(#1340),#975,.T.);
#9563=ADVANCED_FACE('',(#1341,#744),#976,.F.);
#9564=ADVANCED_FACE('',(#1342),#635,.F.);
#9565=ADVANCED_FACE('',(#1343),#977,.T.);
#9566=ADVANCED_FACE('',(#1344),#978,.T.);
#9567=ADVANCED_FACE('',(#1345),#979,.T.);
#9568=ADVANCED_FACE('',(#1346),#636,.F.);
#9569=ADVANCED_FACE('',(#1347),#9230,.F.);
#9570=ADVANCED_FACE('',(#1348),#980,.T.);
#9571=ADVANCED_FACE('',(#1349),#981,.T.);
#9572=ADVANCED_FACE('',(#1350),#982,.T.);
#9573=ADVANCED_FACE('',(#1351),#983,.T.);
#9574=ADVANCED_FACE('',(#1352),#984,.T.);
#9575=ADVANCED_FACE('',(#1353),#985,.T.);
#9576=ADVANCED_FACE('',(#1354,#745,#746),#986,.T.);
#9577=ADVANCED_FACE('',(#1355),#987,.T.);
#9578=ADVANCED_FACE('',(#1356),#988,.T.);
#9579=ADVANCED_FACE('',(#1357),#9231,.F.);
#9580=ADVANCED_FACE('',(#1358),#96,.F.);
#9581=ADVANCED_FACE('',(#1359),#97,.F.);
#9582=ADVANCED_FACE('',(#1360,#747),#9232,.F.);
#9583=ADVANCED_FACE('',(#1361),#989,.T.);
#9584=ADVANCED_FACE('',(#1362),#990,.T.);
#9585=ADVANCED_FACE('',(#1363),#98,.F.);
#9586=ADVANCED_FACE('',(#1364),#99,.F.);
#9587=ADVANCED_FACE('',(#1365),#637,.F.);
#9588=ADVANCED_FACE('',(#1366),#9233,.F.);
#9589=ADVANCED_FACE('',(#1367),#100,.F.);
#9590=ADVANCED_FACE('',(#1368),#101,.F.);
#9591=ADVANCED_FACE('',(#1369),#9234,.F.);
#9592=ADVANCED_FACE('',(#1370),#991,.T.);
#9593=ADVANCED_FACE('',(#1371),#638,.F.);
#9594=ADVANCED_FACE('',(#1372),#992,.T.);
#9595=ADVANCED_FACE('',(#1373),#993,.F.);
#9596=ADVANCED_FACE('',(#1374),#9235,.F.);
#9597=ADVANCED_FACE('',(#1375),#994,.F.);
#9598=ADVANCED_FACE('',(#1376),#102,.F.);
#9599=ADVANCED_FACE('',(#1377),#9236,.F.);
#9600=ADVANCED_FACE('',(#1378),#103,.F.);
#9601=ADVANCED_FACE('',(#1379),#9237,.F.);
#9602=ADVANCED_FACE('',(#1380),#9238,.F.);
#9603=ADVANCED_FACE('',(#1381),#104,.F.);
#9604=ADVANCED_FACE('',(#1382),#9239,.F.);
#9605=ADVANCED_FACE('',(#1383),#105,.F.);
#9606=ADVANCED_FACE('',(#1384),#995,.F.);
#9607=ADVANCED_FACE('',(#1385),#996,.F.);
#9874=CLOSED_SHELL('',(#9498,#9499,#9500,#9501,#9502,#9503,#9504,#9505,
#9506,#9507,#9508,#9509,#9510,#9511,#9512,#9513,#9514,#9515,#9516,#9517,
#9518,#9519,#9520,#9521,#9522,#9523,#9524,#9525,#9526,#9527,#9528,#9529,
#9530,#9531,#9532,#9533,#9534,#9535,#9536,#9537,#9538,#9539,#9540,#9541,
#9542,#9543,#9544,#9545,#9546,#9547,#9548,#9549,#9550,#9551,#9552,#9553,
#9554,#9555,#9556,#9557,#9558,#9559,#9560,#9561,#9562,#9563,#9564,#9565,
#9566,#9567,#9568,#9569,#9570,#9571,#9572,#9573,#9574,#9575,#9576,#9577,
#9578,#9579,#9580,#9581,#9582,#9583,#9584,#9585,#9586,#9587,#9588,#9589,
#9590,#9591,#9592,#9593,#9594,#9595,#9596,#9597,#9598,#9599,#9600,#9601,
#9602,#9603,#9604,#9605,#9606,#9607));
#10466=AXIS2_PLACEMENT_3D('',#18139,#11915,#11916);
#10467=AXIS2_PLACEMENT_3D('',#18140,#11917,#11918);
#10468=AXIS2_PLACEMENT_3D('',#18220,#11920,#11921);
#10469=AXIS2_PLACEMENT_3D('',#18589,#11923,#11924);
#10470=AXIS2_PLACEMENT_3D('',#18954,#11926,#11927);
#10471=AXIS2_PLACEMENT_3D('',#19314,#11929,#11930);
#10472=AXIS2_PLACEMENT_3D('',#19674,#11932,#11933);
#10473=AXIS2_PLACEMENT_3D('',#20036,#11935,#11936);
#10474=AXIS2_PLACEMENT_3D('',#20409,#11938,#11939);
#10475=AXIS2_PLACEMENT_3D('',#20434,#11941,#11942);
#10476=AXIS2_PLACEMENT_3D('',#20533,#11943,#11944);
#10477=AXIS2_PLACEMENT_3D('',#20554,#11946,#11947);
#10478=AXIS2_PLACEMENT_3D('',#20643,#11948,#11949);
#10479=AXIS2_PLACEMENT_3D('',#21041,#11951,#11952);
#10480=AXIS2_PLACEMENT_3D('',#21463,#11954,#11955);
#10481=AXIS2_PLACEMENT_3D('',#21855,#11957,#11958);
#10482=AXIS2_PLACEMENT_3D('',#22277,#11960,#11961);
#10483=AXIS2_PLACEMENT_3D('',#22701,#11963,#11964);
#10484=AXIS2_PLACEMENT_3D('',#23107,#11966,#11967);
#10485=AXIS2_PLACEMENT_3D('',#23525,#11969,#11970);
#10486=AXIS2_PLACEMENT_3D('',#23927,#11972,#11973);
#10487=AXIS2_PLACEMENT_3D('',#24343,#11975,#11976);
#10488=AXIS2_PLACEMENT_3D('',#24742,#11978,#11979);
#10489=AXIS2_PLACEMENT_3D('',#25165,#11981,#11982);
#10490=AXIS2_PLACEMENT_3D('',#25190,#11984,#11985);
#10491=AXIS2_PLACEMENT_3D('',#25301,#11986,#11987);
#10492=AXIS2_PLACEMENT_3D('',#25354,#11989,#11990);
#10493=AXIS2_PLACEMENT_3D('',#25441,#11992,#11993);
#10494=AXIS2_PLACEMENT_3D('',#25656,#11995,#11996);
#10495=AXIS2_PLACEMENT_3D('',#25863,#11998,#11999);
#10496=AXIS2_PLACEMENT_3D('',#26070,#12001,#12002);
#10497=AXIS2_PLACEMENT_3D('',#26295,#12004,#12005);
#10498=AXIS2_PLACEMENT_3D('',#26326,#12007,#12008);
#10499=AXIS2_PLACEMENT_3D('',#26376,#12009,#12010);
#10500=AXIS2_PLACEMENT_3D('',#26407,#12012,#12013);
#10501=AXIS2_PLACEMENT_3D('',#26433,#12014,#12015);
#10502=AXIS2_PLACEMENT_3D('',#26535,#12017,#12018);
#10503=AXIS2_PLACEMENT_3D('',#26637,#12020,#12021);
#10504=AXIS2_PLACEMENT_3D('',#26739,#12023,#12024);
#10505=AXIS2_PLACEMENT_3D('',#26847,#12026,#12027);
#10506=AXIS2_PLACEMENT_3D('',#26949,#12029,#12030);
#10507=AXIS2_PLACEMENT_3D('',#27051,#12032,#12033);
#10508=AXIS2_PLACEMENT_3D('',#27165,#12035,#12036);
#10509=AXIS2_PLACEMENT_3D('',#27264,#12038,#12039);
#10510=AXIS2_PLACEMENT_3D('',#27366,#12041,#12042);
#10511=AXIS2_PLACEMENT_3D('',#27468,#12044,#12045);
#10512=AXIS2_PLACEMENT_3D('',#27499,#12047,#12048);
#10513=AXIS2_PLACEMENT_3D('',#27549,#12049,#12050);
#10514=AXIS2_PLACEMENT_3D('',#27633,#12051,#12052);
#10515=AXIS2_PLACEMENT_3D('',#27855,#12053,#12054);
#10516=AXIS2_PLACEMENT_3D('',#27864,#12059,#12060);
#10517=AXIS2_PLACEMENT_3D('',#27870,#12064,#12065);
#10518=AXIS2_PLACEMENT_3D('',#27876,#12069,#12070);
#10519=AXIS2_PLACEMENT_3D('',#27893,#12075,#12076);
#10520=AXIS2_PLACEMENT_3D('',#27894,#12077,#12078);
#10521=AXIS2_PLACEMENT_3D('',#27898,#12081,#12082);
#10522=AXIS2_PLACEMENT_3D('',#27908,#12087,#12088);
#10523=AXIS2_PLACEMENT_3D('',#27909,#12089,#12090);
#10524=AXIS2_PLACEMENT_3D('',#27911,#12091,#12092);
#10525=AXIS2_PLACEMENT_3D('',#27913,#12093,#12094);
#10526=AXIS2_PLACEMENT_3D('',#27914,#12095,#12096);
#10527=AXIS2_PLACEMENT_3D('',#27916,#12098,#12099);
#10528=AXIS2_PLACEMENT_3D('',#27918,#12101,#12102);
#10529=AXIS2_PLACEMENT_3D('',#27921,#12103,#12104);
#10530=AXIS2_PLACEMENT_3D('',#27926,#12107,#12108);
#10531=AXIS2_PLACEMENT_3D('',#27935,#12113,#12114);
#10532=AXIS2_PLACEMENT_3D('',#27936,#12115,#12116);
#10533=AXIS2_PLACEMENT_3D('',#27938,#12117,#12118);
#10534=AXIS2_PLACEMENT_3D('',#27940,#12120,#12121);
#10535=AXIS2_PLACEMENT_3D('',#27942,#12122,#12123);
#10536=AXIS2_PLACEMENT_3D('',#27944,#12124,#12125);
#10537=AXIS2_PLACEMENT_3D('',#27946,#12127,#12128);
#10538=AXIS2_PLACEMENT_3D('',#27948,#12129,#12130);
#10539=AXIS2_PLACEMENT_3D('',#27952,#12131,#12132);
#10540=AXIS2_PLACEMENT_3D('',#27955,#12133,#12134);
#10541=AXIS2_PLACEMENT_3D('',#27967,#12141,#12142);
#10542=AXIS2_PLACEMENT_3D('',#27968,#12143,#12144);
#10543=AXIS2_PLACEMENT_3D('',#27972,#12145,#12146);
#10544=AXIS2_PLACEMENT_3D('',#27974,#12148,#12149);
#10545=AXIS2_PLACEMENT_3D('',#27977,#12150,#12151);
#10546=AXIS2_PLACEMENT_3D('',#27978,#12152,#12153);
#10547=AXIS2_PLACEMENT_3D('',#27980,#12155,#12156);
#10548=AXIS2_PLACEMENT_3D('',#27981,#12157,#12158);
#10549=AXIS2_PLACEMENT_3D('',#27986,#12160,#12161);
#10550=AXIS2_PLACEMENT_3D('',#27992,#12165,#12166);
#10551=AXIS2_PLACEMENT_3D('',#27994,#12168,#12169);
#10552=AXIS2_PLACEMENT_3D('',#27996,#12171,#12172);
#10553=AXIS2_PLACEMENT_3D('',#28005,#12176,#12177);
#10554=AXIS2_PLACEMENT_3D('',#28011,#12181,#12182);
#10555=AXIS2_PLACEMENT_3D('',#28017,#12186,#12187);
#10556=AXIS2_PLACEMENT_3D('',#28074,#12190,#12191);
#10557=AXIS2_PLACEMENT_3D('',#28076,#12192,#12193);
#10558=AXIS2_PLACEMENT_3D('',#28078,#12195,#12196);
#10559=AXIS2_PLACEMENT_3D('',#28087,#12200,#12201);
#10560=AXIS2_PLACEMENT_3D('',#28091,#12204,#12205);
#10561=AXIS2_PLACEMENT_3D('',#28097,#12209,#12210);
#10562=AXIS2_PLACEMENT_3D('',#28099,#12211,#12212);
#10563=AXIS2_PLACEMENT_3D('',#28101,#12214,#12215);
#10564=AXIS2_PLACEMENT_3D('',#28652,#12216,#12217);
#10565=AXIS2_PLACEMENT_3D('',#29266,#12218,#12219);
#10566=AXIS2_PLACEMENT_3D('',#29269,#12220,#12221);
#10567=AXIS2_PLACEMENT_3D('',#29305,#12222,#12223);
#10568=AXIS2_PLACEMENT_3D('',#29353,#12224,#12225);
#10569=AXIS2_PLACEMENT_3D('',#29354,#12226,#12227);
#10570=AXIS2_PLACEMENT_3D('',#29356,#12229,#12230);
#10571=AXIS2_PLACEMENT_3D('',#29357,#12231,#12232);
#10572=AXIS2_PLACEMENT_3D('',#29359,#12234,#12235);
#10573=AXIS2_PLACEMENT_3D('',#29363,#12238,#12239);
#10574=AXIS2_PLACEMENT_3D('',#29365,#12240,#12241);
#10575=AXIS2_PLACEMENT_3D('',#29366,#12242,#12243);
#10576=AXIS2_PLACEMENT_3D('',#29368,#12245,#12246);
#10577=AXIS2_PLACEMENT_3D('',#29370,#12248,#12249);
#10578=AXIS2_PLACEMENT_3D('',#30511,#12250,#12251);
#10579=AXIS2_PLACEMENT_3D('',#30588,#12253,#12254);
#10580=AXIS2_PLACEMENT_3D('',#30608,#12256,#12257);
#10581=AXIS2_PLACEMENT_3D('',#30659,#12258,#12259);
#10582=AXIS2_PLACEMENT_3D('',#30683,#12261,#12262);
#10583=AXIS2_PLACEMENT_3D('',#30684,#12263,#12264);
#10584=AXIS2_PLACEMENT_3D('',#30686,#12266,#12267);
#10585=AXIS2_PLACEMENT_3D('',#33776,#12269,#12270);
#10586=AXIS2_PLACEMENT_3D('',#33778,#12271,#12272);
#10587=AXIS2_PLACEMENT_3D('',#33780,#12274,#12275);
#10588=AXIS2_PLACEMENT_3D('',#33781,#12276,#12277);
#10589=AXIS2_PLACEMENT_3D('',#33782,#12278,#12279);
#10590=AXIS2_PLACEMENT_3D('',#34588,#12280,#12281);
#10591=AXIS2_PLACEMENT_3D('',#34589,#12282,#12283);
#10592=AXIS2_PLACEMENT_3D('',#34590,#12284,#12285);
#10593=AXIS2_PLACEMENT_3D('',#34592,#12286,#12287);
#10594=AXIS2_PLACEMENT_3D('',#34594,#12289,#12290);
#10595=AXIS2_PLACEMENT_3D('',#34595,#12291,#12292);
#10596=AXIS2_PLACEMENT_3D('',#34596,#12293,#12294);
#10597=AXIS2_PLACEMENT_3D('',#34597,#12295,#12296);
#10598=AXIS2_PLACEMENT_3D('',#34599,#12297,#12298);
#10599=AXIS2_PLACEMENT_3D('',#34607,#12299,#12300);
#10600=AXIS2_PLACEMENT_3D('',#34608,#12301,#12302);
#10601=AXIS2_PLACEMENT_3D('',#34636,#12303,#12304);
#10602=AXIS2_PLACEMENT_3D('',#34677,#12305,#12306);
#10603=AXIS2_PLACEMENT_3D('',#34678,#12307,#12308);
#10604=AXIS2_PLACEMENT_3D('',#34726,#12309,#12310);
#10605=AXIS2_PLACEMENT_3D('',#34763,#12311,#12312);
#10606=AXIS2_PLACEMENT_3D('',#34764,#12313,#12314);
#11915=DIRECTION('axis',(0.,0.,1.));
#11916=DIRECTION('refdir',(1.,0.,0.));
#11917=DIRECTION('center_axis',(1.66533453693773E-16,1.,1.1518563880486E-15));
#11918=DIRECTION('ref_axis',(1.,-1.66533453693753E-16,-1.72407814243868E-14));
#11919=DIRECTION('',(1.66533453693773E-16,1.,1.1518563880486E-15));
#11920=DIRECTION('center_axis',(1.66533453693773E-16,1.,1.1518563880486E-15));
#11921=DIRECTION('ref_axis',(1.,-1.66533453693753E-16,-1.72407814243868E-14));
#11922=DIRECTION('',(1.66533453693773E-16,1.,1.1518563880486E-15));
#11923=DIRECTION('center_axis',(1.66533453693773E-16,1.,1.1518563880486E-15));
#11924=DIRECTION('ref_axis',(1.,-1.66533453693753E-16,-1.72407814243868E-14));
#11925=DIRECTION('',(1.66533453693773E-16,1.,1.1518563880486E-15));
#11926=DIRECTION('center_axis',(1.66533453693773E-16,1.,1.1518563880486E-15));
#11927=DIRECTION('ref_axis',(1.,-1.66533453693753E-16,-1.72407814243868E-14));
#11928=DIRECTION('',(1.66533453693773E-16,1.,1.1518563880486E-15));
#11929=DIRECTION('center_axis',(1.66533453693773E-16,1.,1.1518563880486E-15));
#11930=DIRECTION('ref_axis',(1.,-1.66533453693753E-16,-1.72407814243868E-14));
#11931=DIRECTION('',(1.66533453693773E-16,1.,1.1518563880486E-15));
#11932=DIRECTION('center_axis',(1.66533453693773E-16,1.,1.1518563880486E-15));
#11933=DIRECTION('ref_axis',(1.,-1.66533453693753E-16,-1.72407814243868E-14));
#11934=DIRECTION('',(1.66533453693773E-16,1.,1.1518563880486E-15));
#11935=DIRECTION('center_axis',(1.66533453693773E-16,1.,1.1518563880486E-15));
#11936=DIRECTION('ref_axis',(1.,-1.66533453693753E-16,-1.72407814243868E-14));
#11937=DIRECTION('',(1.66533453693773E-16,1.,1.1518563880486E-15));
#11938=DIRECTION('center_axis',(1.66533453693773E-16,1.,1.1518563880486E-15));
#11939=DIRECTION('ref_axis',(1.,-1.66533453693753E-16,-1.72407814243868E-14));
#11940=DIRECTION('',(1.66533453693773E-16,1.,1.1518563880486E-15));
#11941=DIRECTION('center_axis',(1.66533453693773E-16,1.,1.1518563880486E-15));
#11942=DIRECTION('ref_axis',(1.,-1.66533453686288E-16,-6.49812218125261E-12));
#11943=DIRECTION('center_axis',(1.66533453693773E-16,1.,1.1518563880486E-15));
#11944=DIRECTION('ref_axis',(1.,-1.66533453693706E-16,-5.82535567993926E-14));
#11945=DIRECTION('',(1.66533453693773E-16,1.,1.1518563880486E-15));
#11946=DIRECTION('center_axis',(-1.66533453693773E-16,-1.,-1.1518563880486E-15));
#11947=DIRECTION('ref_axis',(1.,-1.66533453686241E-16,-6.53913495662739E-12));
#11948=DIRECTION('center_axis',(1.66533453693773E-16,1.,1.1518563880486E-15));
#11949=DIRECTION('ref_axis',(1.,-1.66533453693706E-16,-5.82535567993926E-14));
#11950=DIRECTION('',(1.66533453693773E-16,1.,1.1518563880486E-15));
#11951=DIRECTION('center_axis',(1.66533453693773E-16,1.,1.1518563880486E-15));
#11952=DIRECTION('ref_axis',(1.,-1.66533453693706E-16,-5.82535567993926E-14));
#11953=DIRECTION('',(1.66533453693773E-16,1.,1.1518563880486E-15));
#11954=DIRECTION('center_axis',(1.66533453693773E-16,1.,1.1518563880486E-15));
#11955=DIRECTION('ref_axis',(1.,-1.66533453693706E-16,-5.82535567993926E-14));
#11956=DIRECTION('',(1.66533453693773E-16,1.,1.1518563880486E-15));
#11957=DIRECTION('center_axis',(1.66533453693773E-16,1.,1.1518563880486E-15));
#11958=DIRECTION('ref_axis',(1.,-1.66533453693706E-16,-5.82535567993926E-14));
#11959=DIRECTION('',(1.66533453693773E-16,1.,1.1518563880486E-15));
#11960=DIRECTION('center_axis',(1.66533453693773E-16,1.,1.1518563880486E-15));
#11961=DIRECTION('ref_axis',(1.,-1.66533453693706E-16,-5.82535567993926E-14));
#11962=DIRECTION('',(1.66533453693773E-16,1.,1.1518563880486E-15));
#11963=DIRECTION('center_axis',(1.66533453693773E-16,1.,1.1518563880486E-15));
#11964=DIRECTION('ref_axis',(1.,-1.66533453693706E-16,-5.82535567993926E-14));
#11965=DIRECTION('',(1.66533453693773E-16,1.,1.1518563880486E-15));
#11966=DIRECTION('center_axis',(1.66533453693773E-16,1.,1.1518563880486E-15));
#11967=DIRECTION('ref_axis',(1.,-1.66533453693706E-16,-5.82535567993926E-14));
#11968=DIRECTION('',(1.66533453693773E-16,1.,1.1518563880486E-15));
#11969=DIRECTION('center_axis',(1.66533453693773E-16,1.,1.1518563880486E-15));
#11970=DIRECTION('ref_axis',(1.,-1.66533453693706E-16,-5.82535567993926E-14));
#11971=DIRECTION('',(1.66533453693773E-16,1.,1.1518563880486E-15));
#11972=DIRECTION('center_axis',(1.66533453693773E-16,1.,1.1518563880486E-15));
#11973=DIRECTION('ref_axis',(1.,-1.66533453693706E-16,-5.82535567993926E-14));
#11974=DIRECTION('',(1.66533453693773E-16,1.,1.1518563880486E-15));
#11975=DIRECTION('center_axis',(1.66533453693773E-16,1.,1.1518563880486E-15));
#11976=DIRECTION('ref_axis',(1.,-1.66533453693706E-16,-5.82535567993926E-14));
#11977=DIRECTION('',(1.66533453693773E-16,1.,1.1518563880486E-15));
#11978=DIRECTION('center_axis',(1.66533453693773E-16,1.,1.1518563880486E-15));
#11979=DIRECTION('ref_axis',(1.,-1.66533453693706E-16,-5.82535567993926E-14));
#11980=DIRECTION('',(1.66533453693773E-16,1.,1.1518563880486E-15));
#11981=DIRECTION('center_axis',(1.66533453693773E-16,1.,1.1518563880486E-15));
#11982=DIRECTION('ref_axis',(1.,-1.66533453693706E-16,-5.82535567993926E-14));
#11983=DIRECTION('',(1.66533453693773E-16,1.,1.1518563880486E-15));
#11984=DIRECTION('center_axis',(1.66533453693773E-16,1.,1.1518563880486E-15));
#11985=DIRECTION('ref_axis',(1.,-1.66533453686241E-16,-6.53913495662739E-12));
#11986=DIRECTION('center_axis',(1.66533453693773E-16,1.,1.1518563880486E-15));
#11987=DIRECTION('ref_axis',(1.,-1.66533453693773E-16,2.77555756156287E-17));
#11988=DIRECTION('',(1.66533453693773E-16,1.,1.1518563880486E-15));
#11989=DIRECTION('center_axis',(1.66533453693773E-16,1.,1.1518563880486E-15));
#11990=DIRECTION('ref_axis',(1.,-1.66533453693773E-16,2.77555756156287E-17));
#11991=DIRECTION('',(1.66533453693773E-16,1.,1.1518563880486E-15));
#11992=DIRECTION('center_axis',(1.66533453693773E-16,1.,1.1518563880486E-15));
#11993=DIRECTION('ref_axis',(1.,-1.66533453693773E-16,2.77555756156287E-17));
#11994=DIRECTION('',(1.66533453693773E-16,1.,1.1518563880486E-15));
#11995=DIRECTION('center_axis',(1.66533453693773E-16,1.,1.1518563880486E-15));
#11996=DIRECTION('ref_axis',(1.,-1.66533453693773E-16,2.77555756156287E-17));
#11997=DIRECTION('',(1.66533453693773E-16,1.,1.1518563880486E-15));
#11998=DIRECTION('center_axis',(1.66533453693773E-16,1.,1.1518563880486E-15));
#11999=DIRECTION('ref_axis',(1.,-1.66533453693773E-16,2.77555756156287E-17));
#12000=DIRECTION('',(1.66533453693773E-16,1.,1.1518563880486E-15));
#12001=DIRECTION('center_axis',(1.66533453693773E-16,1.,1.1518563880486E-15));
#12002=DIRECTION('ref_axis',(1.,-1.66533453693773E-16,2.77555756156287E-17));
#12003=DIRECTION('',(1.66533453693773E-16,1.,1.1518563880486E-15));
#12004=DIRECTION('center_axis',(1.66533453693773E-16,1.,1.1518563880486E-15));
#12005=DIRECTION('ref_axis',(1.,-1.66533453693773E-16,2.77555756156287E-17));
#12006=DIRECTION('',(1.66533453693773E-16,1.,1.1518563880486E-15));
#12007=DIRECTION('center_axis',(1.66533453693773E-16,1.,1.1518563880486E-15));
#12008=DIRECTION('ref_axis',(1.,-1.66533453693773E-16,2.77555756156287E-17));
#12009=DIRECTION('center_axis',(1.66533453693773E-16,1.,1.1518563880486E-15));
#12010=DIRECTION('ref_axis',(1.,-1.66533453693773E-16,2.77555756156287E-17));
#12011=DIRECTION('',(1.66533453693773E-16,1.,1.1518563880486E-15));
#12012=DIRECTION('center_axis',(-1.66533453693773E-16,-1.,-1.1518563880486E-15));
#12013=DIRECTION('ref_axis',(1.,-1.66533453693773E-16,2.77555756156287E-17));
#12014=DIRECTION('center_axis',(1.66533453693773E-16,1.,1.1518563880486E-15));
#12015=DIRECTION('ref_axis',(1.,-1.66533453693773E-16,2.77555756156287E-17));
#12016=DIRECTION('',(1.66533453693773E-16,1.,1.1518563880486E-15));
#12017=DIRECTION('center_axis',(1.66533453693773E-16,1.,1.1518563880486E-15));
#12018=DIRECTION('ref_axis',(1.,-1.66533453693773E-16,2.77555756156287E-17));
#12019=DIRECTION('',(1.66533453693773E-16,1.,1.1518563880486E-15));
#12020=DIRECTION('center_axis',(1.66533453693773E-16,1.,1.1518563880486E-15));
#12021=DIRECTION('ref_axis',(1.,-1.66533453693773E-16,2.77555756156287E-17));
#12022=DIRECTION('',(1.66533453693773E-16,1.,1.1518563880486E-15));
#12023=DIRECTION('center_axis',(1.66533453693773E-16,1.,1.1518563880486E-15));
#12024=DIRECTION('ref_axis',(1.,-1.66533453693773E-16,2.77555756156287E-17));
#12025=DIRECTION('',(1.66533453693773E-16,1.,1.1518563880486E-15));
#12026=DIRECTION('center_axis',(1.66533453693773E-16,1.,1.1518563880486E-15));
#12027=DIRECTION('ref_axis',(1.,-1.66533453693773E-16,2.77555756156287E-17));
#12028=DIRECTION('',(1.66533453693773E-16,1.,1.1518563880486E-15));
#12029=DIRECTION('center_axis',(1.66533453693773E-16,1.,1.1518563880486E-15));
#12030=DIRECTION('ref_axis',(1.,-1.66533453693773E-16,2.77555756156287E-17));
#12031=DIRECTION('',(1.66533453693773E-16,1.,1.1518563880486E-15));
#12032=DIRECTION('center_axis',(1.66533453693773E-16,1.,1.1518563880486E-15));
#12033=DIRECTION('ref_axis',(1.,-1.66533453693773E-16,2.77555756156287E-17));
#12034=DIRECTION('',(1.66533453693773E-16,1.,1.1518563880486E-15));
#12035=DIRECTION('center_axis',(1.66533453693773E-16,1.,1.1518563880486E-15));
#12036=DIRECTION('ref_axis',(1.,-1.66533453693773E-16,2.77555756156287E-17));
#12037=DIRECTION('',(1.66533453693773E-16,1.,1.1518563880486E-15));
#12038=DIRECTION('center_axis',(1.66533453693773E-16,1.,1.1518563880486E-15));
#12039=DIRECTION('ref_axis',(1.,-1.66533453693773E-16,2.77555756156287E-17));
#12040=DIRECTION('',(1.66533453693773E-16,1.,1.1518563880486E-15));
#12041=DIRECTION('center_axis',(1.66533453693773E-16,1.,1.1518563880486E-15));
#12042=DIRECTION('ref_axis',(1.,-1.66533453693773E-16,2.77555756156287E-17));
#12043=DIRECTION('',(1.66533453693773E-16,1.,1.1518563880486E-15));
#12044=DIRECTION('center_axis',(1.66533453693773E-16,1.,1.1518563880486E-15));
#12045=DIRECTION('ref_axis',(1.,-1.66533453693773E-16,2.77555756156287E-17));
#12046=DIRECTION('',(1.66533453693773E-16,1.,1.1518563880486E-15));
#12047=DIRECTION('center_axis',(1.66533453693773E-16,1.,1.1518563880486E-15));
#12048=DIRECTION('ref_axis',(1.,-1.66533453693773E-16,2.77555756156287E-17));
#12049=DIRECTION('center_axis',(1.66533453693773E-16,1.,1.1518563880486E-15));
#12050=DIRECTION('ref_axis',(1.,-1.66533453693773E-16,2.77555756156287E-17));
#12051=DIRECTION('center_axis',(1.66533453693773E-16,1.,1.1518563880486E-15));
#12052=DIRECTION('ref_axis',(1.,-1.66533453693773E-16,2.77555756156287E-17));
#12053=DIRECTION('center_axis',(-1.,2.96593211435634E-32,-2.77555756156289E-17));
#12054=DIRECTION('ref_axis',(-2.3111159332647E-33,1.,1.1518563880486E-15));
#12055=DIRECTION('',(-1.66533453693773E-16,-1.,-1.1518563880486E-15));
#12056=DIRECTION('',(2.77555756156289E-17,1.1518563880486E-15,-1.));
#12057=DIRECTION('',(1.66533453693773E-16,1.,1.1518563880486E-15));
#12058=DIRECTION('',(2.77555756156289E-17,1.1518563880486E-15,-1.));
#12059=DIRECTION('center_axis',(-0.707106781186547,-0.707106781186548,-8.34111618675756E-16));
#12060=DIRECTION('ref_axis',(-0.707106781186548,0.707106781186547,7.94859307208661E-16));
#12061=DIRECTION('',(-0.707106781186548,0.707106781186547,7.94859307208661E-16));
#12062=DIRECTION('',(0.707106781186548,-0.707106781186547,-7.94859307208661E-16));
#12063=DIRECTION('',(-2.77555756156289E-17,-1.1518563880486E-15,1.));
#12064=DIRECTION('center_axis',(-0.707106781186548,8.14485462942207E-16,
-0.707106781186548));
#12065=DIRECTION('ref_axis',(8.32667268468875E-17,1.,1.06858966120171E-15));
#12066=DIRECTION('',(0.707106781186548,8.14485462942207E-16,-0.707106781186548));
#12067=DIRECTION('',(-1.66533453693773E-16,-1.,-1.1518563880486E-15));
#12068=DIRECTION('',(-0.707106781186548,-8.14485462942207E-16,0.707106781186548));
#12069=DIRECTION('center_axis',(-1.66533453693773E-16,-1.,-1.1518563880486E-15));
#12070=DIRECTION('ref_axis',(-2.77555756156289E-17,-1.1518563880486E-15,
1.));
#12071=DIRECTION('',(1.,-2.96593211435634E-32,2.77555756156289E-17));
#12072=DIRECTION('',(-0.707106781186547,8.14485462942209E-16,-0.707106781186548));
#12073=DIRECTION('',(-1.,2.96593211435634E-32,-2.77555756156289E-17));
#12074=DIRECTION('',(2.77555756156289E-17,1.1518563880486E-15,-1.));
#12075=DIRECTION('center_axis',(-1.66533453693773E-16,-1.,-1.1518563880486E-15));
#12076=DIRECTION('ref_axis',(1.,-1.66533453693773E-16,2.77555756156287E-17));
#12077=DIRECTION('center_axis',(-0.707106781186548,-8.14485462942208E-16,
0.707106781186547));
#12078=DIRECTION('ref_axis',(-0.707106781186547,8.14485462942209E-16,-0.707106781186548));
#12079=DIRECTION('',(0.707106781186547,-8.14485462942209E-16,0.707106781186548));
#12080=DIRECTION('',(1.66533453693773E-16,1.,1.1518563880486E-15));
#12081=DIRECTION('center_axis',(1.66533453693773E-16,1.,1.1518563880486E-15));
#12082=DIRECTION('ref_axis',(1.,-1.66533453693773E-16,2.77555756156287E-17));
#12083=DIRECTION('',(2.77555756156289E-17,1.1518563880486E-15,-1.));
#12084=DIRECTION('',(1.,-2.96593211435634E-32,2.77555756156289E-17));
#12085=DIRECTION('',(-1.,2.96593211435634E-32,-2.77555756156289E-17));
#12086=DIRECTION('',(2.77555756156289E-17,1.1518563880486E-15,-1.));
#12087=DIRECTION('center_axis',(-1.66533453693773E-16,-1.,-1.1518563880486E-15));
#12088=DIRECTION('ref_axis',(1.,-1.66533453693773E-16,2.77555756156287E-17));
#12089=DIRECTION('center_axis',(-1.66533453693773E-16,-1.,-1.1518563880486E-15));
#12090=DIRECTION('ref_axis',(1.,-1.66533453693773E-16,2.77555756156287E-17));
#12091=DIRECTION('center_axis',(-1.66533453693773E-16,-1.,-1.1518563880486E-15));
#12092=DIRECTION('ref_axis',(1.,-1.66533453693773E-16,2.77555756156287E-17));
#12093=DIRECTION('center_axis',(-1.66533453693773E-16,-1.,-1.1518563880486E-15));
#12094=DIRECTION('ref_axis',(1.,-1.66533453693773E-16,2.77555756156287E-17));
#12095=DIRECTION('center_axis',(-0.577350269189626,-0.577350269189625,-0.577350269189627));
#12096=DIRECTION('ref_axis',(-0.707106781186547,0.707106781186548,6.63491932426099E-16));
#12097=DIRECTION('',(1.3738309013483E-16,0.707106781186548,-0.707106781186547));
#12098=DIRECTION('center_axis',(-0.577350269189626,-0.577350269189627,0.577350269189625));
#12099=DIRECTION('ref_axis',(1.073776216497E-16,0.707106781186546,0.707106781186549));
#12100=DIRECTION('',(-9.81307786677355E-17,-0.707106781186546,-0.707106781186549));
#12101=DIRECTION('center_axis',(2.77555756156289E-17,1.1518563880486E-15,
-1.));
#12102=DIRECTION('ref_axis',(1.,-2.96593211435634E-32,2.77555756156289E-17));
#12103=DIRECTION('center_axis',(2.77555756156289E-17,1.1518563880486E-15,
-1.));
#12104=DIRECTION('ref_axis',(1.,-2.96593211435634E-32,2.77555756156289E-17));
#12105=DIRECTION('',(1.66533453693773E-16,1.,1.1518563880486E-15));
#12106=DIRECTION('',(1.,-2.96593211435634E-32,2.77555756156289E-17));
#12107=DIRECTION('center_axis',(2.77555756156289E-17,1.1518563880486E-15,
-1.));
#12108=DIRECTION('ref_axis',(1.,-2.96593211435634E-32,2.77555756156289E-17));
#12109=DIRECTION('',(-1.,2.96593211435634E-32,-2.77555756156289E-17));
#12110=DIRECTION('',(-1.66533453693773E-16,-1.,-1.1518563880486E-15));
#12111=DIRECTION('',(-1.,2.96593211435634E-32,-2.77555756156289E-17));
#12112=DIRECTION('',(1.66533453693773E-16,1.,1.1518563880486E-15));
#12113=DIRECTION('center_axis',(2.77555756156289E-17,1.1518563880486E-15,
-1.));
#12114=DIRECTION('ref_axis',(1.,-2.96593211435634E-32,2.77555756156289E-17));
#12115=DIRECTION('center_axis',(1.66533453693773E-16,1.,1.1518563880486E-15));
#12116=DIRECTION('ref_axis',(1.,-1.66533453693773E-16,2.77555756156287E-17));
#12117=DIRECTION('center_axis',(1.66533453693773E-16,1.,1.1518563880486E-15));
#12118=DIRECTION('ref_axis',(1.,-1.66533453693773E-16,2.77555756156287E-17));
#12119=DIRECTION('',(1.66533453693773E-16,1.,1.1518563880486E-15));
#12120=DIRECTION('center_axis',(2.77555756156289E-17,1.1518563880486E-15,
-1.));
#12121=DIRECTION('ref_axis',(1.,-2.96593211435634E-32,2.77555756156289E-17));
#12122=DIRECTION('center_axis',(-2.77555756156289E-17,-1.1518563880486E-15,
1.));
#12123=DIRECTION('ref_axis',(1.,-2.96593211435634E-32,2.77555756156289E-17));
#12124=DIRECTION('center_axis',(2.77555756156289E-17,1.1518563880486E-15,
-1.));
#12125=DIRECTION('ref_axis',(1.,-2.96593211435634E-32,2.77555756156289E-17));
#12126=DIRECTION('',(2.77555756156289E-17,1.1518563880486E-15,-1.));
#12127=DIRECTION('center_axis',(-2.77555756156289E-17,-1.1518563880486E-15,
1.));
#12128=DIRECTION('ref_axis',(1.,-2.96593211435634E-32,2.77555756156289E-17));
#12129=DIRECTION('center_axis',(-2.77555756156289E-17,-1.1518563880486E-15,
1.));
#12130=DIRECTION('ref_axis',(1.,-2.96593211435634E-32,2.77555756156289E-17));
#12131=DIRECTION('center_axis',(-2.77555756156289E-17,-1.1518563880486E-15,
1.));
#12132=DIRECTION('ref_axis',(-1.66533453693773E-16,-1.,-1.1518563880486E-15));
#12133=DIRECTION('center_axis',(-2.77555756156289E-17,-1.1518563880486E-15,
1.));
#12134=DIRECTION('ref_axis',(1.,-2.96593211435634E-32,2.77555756156289E-17));
#12135=DIRECTION('',(-1.66533453693773E-16,-1.,-1.1518563880486E-15));
#12136=DIRECTION('',(1.,-2.96593211435634E-32,2.77555756156289E-17));
#12137=DIRECTION('',(1.66533453693773E-16,1.,1.1518563880486E-15));
#12138=DIRECTION('',(1.,-2.96593211435634E-32,2.77555756156289E-17));
#12139=DIRECTION('',(-1.,2.96593211435634E-32,-2.77555756156289E-17));
#12140=DIRECTION('',(-1.66533453693773E-16,-1.,-1.1518563880486E-15));
#12141=DIRECTION('center_axis',(-2.77555756156289E-17,-1.1518563880486E-15,
1.));
#12142=DIRECTION('ref_axis',(1.,-2.96593211435634E-32,2.77555756156289E-17));
#12143=DIRECTION('center_axis',(2.77555756156289E-17,1.1518563880486E-15,
-1.));
#12144=DIRECTION('ref_axis',(1.,-2.96593211435634E-32,2.77555756156289E-17));
#12145=DIRECTION('center_axis',(-1.66533453693773E-16,-1.,-1.1518563880486E-15));
#12146=DIRECTION('ref_axis',(1.,-1.66533453693773E-16,2.77555756156287E-17));
#12147=DIRECTION('',(-0.707106781186548,-0.707106781186547,-9.20707224299304E-16));
#12148=DIRECTION('center_axis',(-1.66533453693773E-16,-1.,-1.1518563880486E-15));
#12149=DIRECTION('ref_axis',(1.,-1.66533453693773E-16,2.77555756156287E-17));
#12150=DIRECTION('center_axis',(1.66533453693773E-16,1.,1.1518563880486E-15));
#12151=DIRECTION('ref_axis',(1.,-1.66533453693773E-16,2.77555756156287E-17));
#12152=DIRECTION('center_axis',(1.66533453693773E-16,1.,1.1518563880486E-15));
#12153=DIRECTION('ref_axis',(1.,-1.66533453693773E-16,2.77555756156287E-17));
#12154=DIRECTION('',(-0.707106781186548,-0.707106781186547,-9.20707224299304E-16));
#12155=DIRECTION('center_axis',(-1.66533453693773E-16,-1.,-1.1518563880486E-15));
#12156=DIRECTION('ref_axis',(1.,-1.66533453693773E-16,2.77555756156287E-17));
#12157=DIRECTION('center_axis',(1.66533453693773E-16,1.,1.1518563880486E-15));
#12158=DIRECTION('ref_axis',(1.,-1.66533453693773E-16,2.77555756156287E-17));
#12159=DIRECTION('',(-0.707106781186548,-0.707106781186547,-9.20707224299304E-16));
#12160=DIRECTION('center_axis',(0.707106781186547,-0.707106781186548,-7.94859307208662E-16));
#12161=DIRECTION('ref_axis',(-2.77555756156286E-17,-1.1518563880486E-15,
1.));
#12162=DIRECTION('',(0.707106781186548,0.707106781186547,8.34111618675755E-16));
#12163=DIRECTION('',(-2.77555756156289E-17,-1.1518563880486E-15,1.));
#12164=DIRECTION('',(-0.707106781186548,-0.707106781186547,-8.34111618675755E-16));
#12165=DIRECTION('center_axis',(-9.81307786677357E-17,-0.707106781186547,
-0.707106781186548));
#12166=DIRECTION('ref_axis',(-1.,8.32667268468865E-17,5.55111512312577E-17));
#12167=DIRECTION('',(-1.3738309013483E-16,-0.707106781186548,0.707106781186547));
#12168=DIRECTION('center_axis',(-1.3738309013483E-16,-0.707106781186549,
0.707106781186546));
#12169=DIRECTION('ref_axis',(9.81307786677355E-17,0.707106781186546,0.707106781186549));
#12170=DIRECTION('',(9.81307786677355E-17,0.707106781186546,0.707106781186549));
#12171=DIRECTION('center_axis',(0.707106781186548,8.14485462942207E-16,
-0.707106781186548));
#12172=DIRECTION('ref_axis',(-8.32667268468889E-17,-1.,-1.23512311489549E-15));
#12173=DIRECTION('',(0.707106781186548,-8.14485462942207E-16,0.707106781186548));
#12174=DIRECTION('',(-1.66533453693773E-16,-1.,-1.1518563880486E-15));
#12175=DIRECTION('',(-0.707106781186548,8.14485462942207E-16,-0.707106781186548));
#12176=DIRECTION('center_axis',(1.3738309013483E-16,0.707106781186549,-0.707106781186547));
#12177=DIRECTION('ref_axis',(1.,-8.32667268468867E-17,1.11022302462515E-16));
#12178=DIRECTION('',(9.81307786677356E-17,0.707106781186547,0.707106781186548));
#12179=DIRECTION('',(1.,-2.96593211435634E-32,2.77555756156289E-17));
#12180=DIRECTION('',(-9.81307786677356E-17,-0.707106781186547,-0.707106781186548));
#12181=DIRECTION('center_axis',(-0.707106781186548,8.14485462942207E-16,
-0.707106781186548));
#12182=DIRECTION('ref_axis',(8.32667268468875E-17,1.,1.06858966120171E-15));
#12183=DIRECTION('',(-0.707106781186548,-8.14485462942207E-16,0.707106781186548));
#12184=DIRECTION('',(1.66533453693773E-16,1.,1.1518563880486E-15));
#12185=DIRECTION('',(0.707106781186548,8.14485462942207E-16,-0.707106781186548));
#12186=DIRECTION('center_axis',(1.66533453693773E-16,1.,1.1518563880486E-15));
#12187=DIRECTION('ref_axis',(1.,-1.66533453693773E-16,2.77555756156287E-17));
#12188=DIRECTION('',(0.707106781186547,-8.14485462942209E-16,0.707106781186548));
#12189=DIRECTION('',(-2.77555756156289E-17,-1.1518563880486E-15,1.));
#12190=DIRECTION('center_axis',(2.77555756156289E-17,1.1518563880486E-15,
-1.));
#12191=DIRECTION('ref_axis',(1.,-2.96593211435634E-32,2.77555756156289E-17));
#12192=DIRECTION('center_axis',(-2.77555756156289E-17,-1.1518563880486E-15,
1.));
#12193=DIRECTION('ref_axis',(1.,-2.96593211435634E-32,2.77555756156289E-17));
#12194=DIRECTION('',(-0.707106781186547,9.01081068565758E-16,-0.707106781186548));
#12195=DIRECTION('center_axis',(0.707106781186547,-8.14485462942209E-16,
0.707106781186548));
#12196=DIRECTION('ref_axis',(-8.32667268468885E-17,-1.,-1.06858966120171E-15));
#12197=DIRECTION('',(0.707106781186548,8.14485462942208E-16,-0.707106781186547));
#12198=DIRECTION('',(1.66533453693773E-16,1.,1.1518563880486E-15));
#12199=DIRECTION('',(-0.707106781186548,-8.14485462942208E-16,0.707106781186547));
#12200=DIRECTION('center_axis',(-0.707106781186548,-8.14485462942208E-16,
0.707106781186547));
#12201=DIRECTION('ref_axis',(-0.707106781186547,8.14485462942209E-16,-0.707106781186548));
#12202=DIRECTION('',(-0.707106781186547,8.14485462942209E-16,-0.707106781186548));
#12203=DIRECTION('',(-1.66533453693773E-16,-1.,-1.1518563880486E-15));
#12204=DIRECTION('center_axis',(9.81307786677355E-17,0.707106781186547,
0.707106781186549));
#12205=DIRECTION('ref_axis',(-1.,8.32667268468864E-17,5.55111512312577E-17));
#12206=DIRECTION('',(1.3738309013483E-16,0.707106781186548,-0.707106781186547));
#12207=DIRECTION('',(-1.,2.96593211435634E-32,-2.77555756156289E-17));
#12208=DIRECTION('',(-1.3738309013483E-16,-0.707106781186548,0.707106781186547));
#12209=DIRECTION('center_axis',(-2.77555756156289E-17,-1.1518563880486E-15,
1.));
#12210=DIRECTION('ref_axis',(1.,-2.96593211435634E-32,2.77555756156289E-17));
#12211=DIRECTION('center_axis',(2.77555756156289E-17,1.1518563880486E-15,
-1.));
#12212=DIRECTION('ref_axis',(1.,-2.96593211435634E-32,2.77555756156289E-17));
#12213=DIRECTION('',(-0.707106781186548,-9.01081068565757E-16,0.707106781186547));
#12214=DIRECTION('center_axis',(1.66533453693773E-16,1.,1.1518563880486E-15));
#12215=DIRECTION('ref_axis',(1.,-1.66533453693773E-16,2.77555756156287E-17));
#12216=DIRECTION('center_axis',(-1.66533453693773E-16,-1.,-1.1518563880486E-15));
#12217=DIRECTION('ref_axis',(1.,-1.66533453693773E-16,2.77555756156287E-17));
#12218=DIRECTION('center_axis',(1.66533453693773E-16,1.,1.1518563880486E-15));
#12219=DIRECTION('ref_axis',(1.,-1.66533453693773E-16,2.77555756156287E-17));
#12220=DIRECTION('center_axis',(-3.33321305916122E-12,1.,1.15185639931397E-15));
#12221=DIRECTION('ref_axis',(1.,3.33321305916122E-12,-3.37956487043916E-12));
#12222=DIRECTION('center_axis',(1.66533453693773E-16,1.,1.1518563880486E-15));
#12223=DIRECTION('ref_axis',(1.,-1.66533453693773E-16,2.77555756156287E-17));
#12224=DIRECTION('center_axis',(0.577350269189626,-0.577350269189627,0.577350269189625));
#12225=DIRECTION('ref_axis',(-1.98170923120496E-17,0.707106781186546,0.707106781186549));
#12226=DIRECTION('center_axis',(1.,-2.96593211435634E-32,2.77555756156289E-17));
#12227=DIRECTION('ref_axis',(2.77555756156289E-17,1.1518563880486E-15,-1.));
#12228=DIRECTION('',(2.77555756156289E-17,1.1518563880486E-15,-1.));
#12229=DIRECTION('center_axis',(0.577350269189626,-0.577350269189625,-0.577350269189627));
#12230=DIRECTION('ref_axis',(-1.44988248207523E-16,-0.707106781186549,0.707106781186546));
#12231=DIRECTION('center_axis',(0.577350269189626,0.577350269189627,-0.577350269189625));
#12232=DIRECTION('ref_axis',(-1.073776216497E-16,-0.707106781186546,-0.707106781186549));
#12233=DIRECTION('',(-0.707106781186548,0.707106781186548,7.94859307208662E-16));
#12234=DIRECTION('center_axis',(1.66533453693773E-16,1.,1.1518563880486E-15));
#12235=DIRECTION('ref_axis',(1.,-1.66533453693773E-16,2.77555756156287E-17));
#12236=DIRECTION('',(-2.77555756156289E-17,-1.1518563880486E-15,1.));
#12237=DIRECTION('',(2.77555756156289E-17,1.1518563880486E-15,-1.));
#12238=DIRECTION('center_axis',(1.66533453693773E-16,1.,1.1518563880486E-15));
#12239=DIRECTION('ref_axis',(1.,-1.66533453693773E-16,2.77555756156287E-17));
#12240=DIRECTION('center_axis',(1.66533453693773E-16,1.,1.1518563880486E-15));
#12241=DIRECTION('ref_axis',(1.,-1.66533453693773E-16,2.77555756156287E-17));
#12242=DIRECTION('center_axis',(-0.577350269189626,0.577350269189627,-0.577350269189625));
#12243=DIRECTION('ref_axis',(0.707106781186548,0.707106781186547,7.17735637696692E-16));
#12244=DIRECTION('',(-0.707106781186548,-0.707106781186548,-8.34111618675754E-16));
#12245=DIRECTION('center_axis',(-1.,2.96593211435634E-32,-2.77555756156289E-17));
#12246=DIRECTION('ref_axis',(-2.3111159332647E-33,1.,1.1518563880486E-15));
#12247=DIRECTION('',(-2.77555756156289E-17,-1.1518563880486E-15,1.));
#12248=DIRECTION('center_axis',(1.66533453693773E-16,1.,1.1518563880486E-15));
#12249=DIRECTION('ref_axis',(1.,-1.66533453693706E-16,-5.82535567993926E-14));
#12250=DIRECTION('center_axis',(2.77555756156289E-17,1.1518563880486E-15,
-1.));
#12251=DIRECTION('ref_axis',(1.,-2.96593211435634E-32,2.77555756156289E-17));
#12252=DIRECTION('',(2.77555756156289E-17,1.1518563880486E-15,-1.));
#12253=DIRECTION('center_axis',(-0.0089256192300513,-0.714647716078422,
-0.699427605421215));
#12254=DIRECTION('ref_axis',(-0.0957941300462763,0.696849620500493,-0.710791172607677));
#12255=DIRECTION('',(2.77555756156289E-17,1.1518563880486E-15,-1.));
#12256=DIRECTION('center_axis',(-0.0044136154535447,-0.712446086579493,
0.701712971033166));
#12257=DIRECTION('ref_axis',(0.138109839253334,-0.69542932579062,-0.705197649692497));
#12258=DIRECTION('center_axis',(0.00217776971565482,-0.711046915342384,
0.703141195992062));
#12259=DIRECTION('ref_axis',(-0.164197556343665,-0.693853653920902,-0.701146396575909));
#12260=DIRECTION('',(-2.77555756156289E-17,-1.1518563880486E-15,1.));
#12261=DIRECTION('center_axis',(0.0157381824501623,-0.717295463101778,-0.696591363876105));
#12262=DIRECTION('ref_axis',(0.0401947273684774,0.69656836830124,-0.716363659166154));
#12263=DIRECTION('center_axis',(0.577350269189626,0.577350269189625,0.577350269189627));
#12264=DIRECTION('ref_axis',(5.74277188698721E-17,-0.707106781186549,0.707106781186546));
#12265=DIRECTION('',(0.707106781186548,-0.707106781186548,-7.94859307208662E-16));
#12266=DIRECTION('center_axis',(-0.577350269189626,0.577350269189625,0.577350269189627));
#12267=DIRECTION('ref_axis',(-0.707106781186548,7.32325096026742E-16,-0.707106781186547));
#12268=DIRECTION('',(0.707106781186548,0.707106781186548,8.34111618675754E-16));
#12269=DIRECTION('center_axis',(1.66533453693773E-16,1.,1.1518563880486E-15));
#12270=DIRECTION('ref_axis',(1.,-1.66533453693773E-16,2.77555756156287E-17));
#12271=DIRECTION('center_axis',(-1.66533453693773E-16,-1.,-1.1518563880486E-15));
#12272=DIRECTION('ref_axis',(1.,-1.66533453693773E-16,2.77555756156287E-17));
#12273=DIRECTION('',(-0.707106781186547,0.707106781186548,8.81454912832211E-16));
#12274=DIRECTION('center_axis',(-1.66533453693773E-16,-1.,-1.1518563880486E-15));
#12275=DIRECTION('ref_axis',(1.,-1.66533453693773E-16,2.77555756156287E-17));
#12276=DIRECTION('center_axis',(1.20274161001058E-16,1.,1.1518563880486E-15));
#12277=DIRECTION('ref_axis',(1.,-1.20274161001005E-16,-4.62315371170993E-14));
#12278=DIRECTION('center_axis',(3.33321305916122E-12,-1.,-1.15185639931397E-15));
#12279=DIRECTION('ref_axis',(1.,3.33321305916122E-12,-3.37956487043916E-12));
#12280=DIRECTION('center_axis',(1.66533453693773E-16,1.,1.1518563880486E-15));
#12281=DIRECTION('ref_axis',(1.,-1.66533453693753E-16,-1.72407814243868E-14));
#12282=DIRECTION('center_axis',(0.707106781186548,0.707106781186548,8.34111618675754E-16));
#12283=DIRECTION('ref_axis',(-2.77555756156281E-17,-1.1518563880486E-15,
1.));
#12284=DIRECTION('center_axis',(1.66533453693773E-16,1.,1.1518563880486E-15));
#12285=DIRECTION('ref_axis',(1.,-1.66533453693773E-16,2.77555756156287E-17));
#12286=DIRECTION('center_axis',(-1.66533453693773E-16,-1.,-1.1518563880486E-15));
#12287=DIRECTION('ref_axis',(1.,-1.66533453693773E-16,2.77555756156287E-17));
#12288=DIRECTION('',(-0.707106781186547,0.707106781186548,8.81454912832211E-16));
#12289=DIRECTION('center_axis',(-1.66533453693773E-16,-1.,-1.1518563880486E-15));
#12290=DIRECTION('ref_axis',(1.,-1.66533453693773E-16,2.77555756156287E-17));
#12291=DIRECTION('center_axis',(-0.707106781186548,0.707106781186548,7.94859307208662E-16));
#12292=DIRECTION('ref_axis',(2.77555756156286E-17,1.1518563880486E-15,-1.));
#12293=DIRECTION('center_axis',(1.66533453693773E-16,1.,1.1518563880486E-15));
#12294=DIRECTION('ref_axis',(1.,-1.66533453693773E-16,2.77555756156287E-17));
#12295=DIRECTION('center_axis',(1.66533453693773E-16,1.,1.1518563880486E-15));
#12296=DIRECTION('ref_axis',(1.,-1.66533453693753E-16,-1.72407814243868E-14));
#12297=DIRECTION('center_axis',(-1.66533453693773E-16,-1.,-1.1518563880486E-15));
#12298=DIRECTION('ref_axis',(1.,-1.66533453686288E-16,-6.49812218125261E-12));
#12299=DIRECTION('center_axis',(1.66533453693773E-16,1.,1.1518563880486E-15));
#12300=DIRECTION('ref_axis',(1.,-1.66533453693773E-16,2.77555756156287E-17));
#12301=DIRECTION('center_axis',(2.90775474051727E-9,-1.,-1.25901276750935E-9));
#12302=DIRECTION('ref_axis',(-0.245664236959599,5.0609894999909E-10,-0.969354982799933));
#12303=DIRECTION('center_axis',(1.66533453693773E-16,1.,1.1518563880486E-15));
#12304=DIRECTION('ref_axis',(1.,-1.66533453693773E-16,2.77555756156287E-17));
#12305=DIRECTION('center_axis',(1.66533453693773E-16,1.,1.1518563880486E-15));
#12306=DIRECTION('ref_axis',(1.,-1.66533453693753E-16,-1.72407814243868E-14));
#12307=DIRECTION('center_axis',(1.66533453693773E-16,1.,1.1518563880486E-15));
#12308=DIRECTION('ref_axis',(-0.987415940103716,3.46597824626892E-16,-0.158144747712638));
#12309=DIRECTION('center_axis',(1.66533453693773E-16,1.,1.1518563880486E-15));
#12310=DIRECTION('ref_axis',(-0.99782706232177,2.42064446342925E-16,-0.0658874320208806));
#12311=DIRECTION('center_axis',(1.66533453693773E-16,1.,1.1518563880486E-15));
#12312=DIRECTION('ref_axis',(1.,-1.66533453693773E-16,2.77555756156287E-17));
#12313=DIRECTION('center_axis',(1.66533453693773E-16,1.,1.1518563880486E-15));
#12314=DIRECTION('ref_axis',(1.,-1.66533453693773E-16,2.77555756156287E-17));
#18139=CARTESIAN_POINT('',(0.,0.,0.));
#18140=CARTESIAN_POINT('Origin',(0.006,-0.0418165664398416,-0.0121758532865581));
#18141=CARTESIAN_POINT('',(0.004457,-0.0371814756795928,-0.0121758532865588));
#18142=CARTESIAN_POINT('',(0.004457,-0.0370665921755392,-0.0121758532865484));
#18143=CARTESIAN_POINT('',(0.004457,-0.0418165664398416,-0.0121758532865581));
#18144=CARTESIAN_POINT('',(0.00445696473503848,-0.0370665033115447,-0.012173946036331));
#18145=CARTESIAN_POINT('Ctrl Pts',(0.004457,-0.0370665921755392,-0.0121758532865387));
#18146=CARTESIAN_POINT('Ctrl Pts',(0.00445700000000001,-0.0370665704100319,
-0.0121754755766259));
#18147=CARTESIAN_POINT('Ctrl Pts',(0.00445700013868904,-0.0370665486443835,
-0.0121750978648529));
#18148=CARTESIAN_POINT('Ctrl Pts',(0.00445700041607119,-0.0370665268786158,
-0.0121747201512957));
#18149=CARTESIAN_POINT('',(0.00543336738605003,-0.0369714897070198,-0.0107406611481222));
#18150=CARTESIAN_POINT('Ctrl Pts',(0.00445696473503848,-0.0370665033115447,
-0.012173946036331));
#18151=CARTESIAN_POINT('Ctrl Pts',(0.00445682508442995,-0.0370607195511547,
-0.0120708997231622));
#18152=CARTESIAN_POINT('Ctrl Pts',(0.00446642871231062,-0.0370552784860267,
-0.0119678729985124));
#18153=CARTESIAN_POINT('Ctrl Pts',(0.00448680026437125,-0.0370500323662534,
-0.0118669686934194));
#18154=CARTESIAN_POINT('Ctrl Pts',(0.0045352522124094,-0.0370375549309602,
-0.0116269766627366));
#18155=CARTESIAN_POINT('Ctrl Pts',(0.00464519561945393,-0.0370261802712467,
-0.0113987962647978));
#18156=CARTESIAN_POINT('Ctrl Pts',(0.00479913627550219,-0.0370139205143147,
-0.0112081339394185));
#18157=CARTESIAN_POINT('Ctrl Pts',(0.00496595972382667,-0.0370006347782426,
-0.0110015157048218));
#18158=CARTESIAN_POINT('Ctrl Pts',(0.00518626704742854,-0.0369851941685886,
-0.0108382129844631));
#18159=CARTESIAN_POINT('Ctrl Pts',(0.00543336738418062,-0.0369714897101142,
-0.010740661146572));
#18160=CARTESIAN_POINT('',(0.00581125245410382,-0.0370677682650875,-0.0106436206577455));
#18161=CARTESIAN_POINT('Ctrl Pts',(0.00581141341884543,-0.0370672590668868,
-0.0106444212438581));
#18162=CARTESIAN_POINT('Ctrl Pts',(0.00576806064819256,-0.0370619449087914,
-0.010649759875004));
#18163=CARTESIAN_POINT('Ctrl Pts',(0.00572496277193653,-0.0370547949103012,
-0.0106569430206965));
#18164=CARTESIAN_POINT('Ctrl Pts',(0.00559660094773692,-0.0370279297986178,
-0.0106839354017503));
#18165=CARTESIAN_POINT('Ctrl Pts',(0.00551294803925241,-0.037002745347212,
-0.0107092416638838));
#18166=CARTESIAN_POINT('Ctrl Pts',(0.00543336738593308,-0.0369714897050595,
-0.010740661145876));
#18167=CARTESIAN_POINT('',(0.00445700028015853,-0.0371814311999794,-0.0121749234644574));
#18168=CARTESIAN_POINT('Ctrl Pts',(0.00581095120124511,-0.0370682602733425,
-0.01064447823397));
#18169=CARTESIAN_POINT('Ctrl Pts',(0.00579234229401333,-0.0370693014592163,
-0.0106467755102331));
#18170=CARTESIAN_POINT('Ctrl Pts',(0.0057737761556256,-0.03707033323956,
-0.0106494118730359));
#18171=CARTESIAN_POINT('Ctrl Pts',(0.00574225603645012,-0.0370720680688304,
-0.0106544754334336));
#18172=CARTESIAN_POINT('Ctrl Pts',(0.00572927689885044,-0.0370727775234059,
-0.0106567313214004));
#18173=CARTESIAN_POINT('Ctrl Pts',(0.00570792885345587,-0.0370739346080628,
-0.0106607240984138));
#18174=CARTESIAN_POINT('Ctrl Pts',(0.00569954283859992,-0.0370743866244655,
-0.0106623647627505));
#18175=CARTESIAN_POINT('Ctrl Pts',(0.00568340492125055,-0.0370752510584431,
-0.0106656614509511));
#18176=CARTESIAN_POINT('Ctrl Pts',(0.00567565122453858,-0.0370756639572011,
-0.0106673077270314));
#18177=CARTESIAN_POINT('Ctrl Pts',(0.00565870685475073,-0.0370765604788409,
-0.010671042067358));
#18178=CARTESIAN_POINT('Ctrl Pts',(0.0056495220206615,-0.0370770427706411,
-0.0106731547103358));
#18179=CARTESIAN_POINT('Ctrl Pts',(0.0056233619690746,-0.0370784073533569,
-0.0106794248005471));
#18180=CARTESIAN_POINT('Ctrl Pts',(0.00560643682090592,-0.0370792792695538,
-0.0106837867698845));
#18181=CARTESIAN_POINT('Ctrl Pts',(0.00552448525263467,-0.0370834631690544,
-0.0107063990048912));
#18182=CARTESIAN_POINT('Ctrl Pts',(0.00546062594759169,-0.0370866084949523,
-0.0107286189551597));
#18183=CARTESIAN_POINT('Ctrl Pts',(0.00532773457379046,-0.0370932706475194,
-0.010784882070171));
#18184=CARTESIAN_POINT('Ctrl Pts',(0.00525937729396276,-0.0370967732312161,
-0.0108200437749403));
#18185=CARTESIAN_POINT('Ctrl Pts',(0.00516528586352355,-0.0371019833621321,
-0.0108776895128799));
#18186=CARTESIAN_POINT('Ctrl Pts',(0.0051372306427446,-0.0371035899557449,
-0.0108961635778762));
#18187=CARTESIAN_POINT('Ctrl Pts',(0.00508780389631469,-0.0371065378973649,
-0.0109310751634043));
#18188=CARTESIAN_POINT('Ctrl Pts',(0.00506621776725708,-0.0371078681862633,
-0.0109471853309022));
#18189=CARTESIAN_POINT('Ctrl Pts',(0.00503252226858799,-0.0371100207712954,
-0.0109737339824954));
#18190=CARTESIAN_POINT('Ctrl Pts',(0.00502013401202563,-0.037110829274222,
-0.0109838102488626));
#18191=CARTESIAN_POINT('Ctrl Pts',(0.00499673714829802,-0.0371123905174636,
-0.0110034517959461));
#18192=CARTESIAN_POINT('Ctrl Pts',(0.00498570335728822,-0.0371131419212072,
-0.0110129844605238));
#18193=CARTESIAN_POINT('Ctrl Pts',(0.00496055713795835,-0.0371148904823943,
-0.0110353397799863));
#18194=CARTESIAN_POINT('Ctrl Pts',(0.00494654418660995,-0.0371158919816601,
-0.0110482703278011));
#18195=CARTESIAN_POINT('Ctrl Pts',(0.00490196780727019,-0.03711916832195,
-0.0110909598345263));
#18196=CARTESIAN_POINT('Ctrl Pts',(0.00487239956716035,-0.0371214845949833,
-0.0111217255363832));
#18197=CARTESIAN_POINT('Ctrl Pts',(0.00479850634010012,-0.0371276564291069,
-0.0112052821974612));
#18198=CARTESIAN_POINT('Ctrl Pts',(0.00475637781415507,-0.0371315784249489,
-0.0112598849892025));
#18199=CARTESIAN_POINT('Ctrl Pts',(0.00467070337278055,-0.0371403937136393,
-0.011387783336617));
#18200=CARTESIAN_POINT('Ctrl Pts',(0.00462928731841433,-0.0371452860467748,
-0.0114622482202439));
#18201=CARTESIAN_POINT('Ctrl Pts',(0.00458722942930083,-0.0371508441390535,
-0.0115551958006175));
#18202=CARTESIAN_POINT('Ctrl Pts',(0.00458049533488884,-0.0371517568163958,
-0.0115707558146567));
#18203=CARTESIAN_POINT('Ctrl Pts',(0.00457043943478568,-0.0371531528710488,
-0.011595083635554));
#18204=CARTESIAN_POINT('Ctrl Pts',(0.00456693893407913,-0.0371536456263738,
-0.0116037756806916));
#18205=CARTESIAN_POINT('Ctrl Pts',(0.00456051083071472,-0.0371545627915118,
-0.0116201665403943));
#18206=CARTESIAN_POINT('Ctrl Pts',(0.00455756539274089,-0.0371549881334905,
-0.0116278576355199));
#18207=CARTESIAN_POINT('Ctrl Pts',(0.00455051208629032,-0.0371560199398415,
-0.0116467260960982));
#18208=CARTESIAN_POINT('Ctrl Pts',(0.00454647170928672,-0.0371566226394305,
-0.0116579282725353));
#18209=CARTESIAN_POINT('Ctrl Pts',(0.00453143623820617,-0.0371589156491401,
-0.0117011772912719));
#18210=CARTESIAN_POINT('Ctrl Pts',(0.00452136746047995,-0.0371605604294028,
-0.0117335378869258));
#18211=CARTESIAN_POINT('Ctrl Pts',(0.00449557653918292,-0.0371651861971653,
-0.0118271971474061));
#18212=CARTESIAN_POINT('Ctrl Pts',(0.00448254734367659,-0.0371680865114223,
-0.0118891666859977));
#18213=CARTESIAN_POINT('Ctrl Pts',(0.00446251211444976,-0.0371744246287094,
-0.0120256592311372));
#18214=CARTESIAN_POINT('Ctrl Pts',(0.00445704528366618,-0.0371778592144949,
-0.0121002420831587));
#18215=CARTESIAN_POINT('Ctrl Pts',(0.00445700028015854,-0.0371814311999789,
-0.0121749234644459));
#18216=CARTESIAN_POINT('Ctrl Pts',(0.004457,-0.0371814756795928,-0.0121758532865595));
#18217=CARTESIAN_POINT('Ctrl Pts',(0.004457,-0.0371814606916064,-0.0121755400169382));
#18218=CARTESIAN_POINT('Ctrl Pts',(0.00445700009137941,-0.0371814461836175,
-0.0121752367352671));
#18219=CARTESIAN_POINT('Ctrl Pts',(0.00445700028015853,-0.0371814311999794,
-0.0121749234644572));
#18220=CARTESIAN_POINT('Origin',(0.006,-0.0418165664398416,-0.0121758532865581));
#18221=CARTESIAN_POINT('',(0.004457,-0.0376822061652104,-0.0121758532865608));
#18222=CARTESIAN_POINT('',(0.004457,-0.037567972222619,-0.0121758532865581));
#18223=CARTESIAN_POINT('',(0.004457,-0.0418165664398416,-0.0121758532865581));
#18224=CARTESIAN_POINT('',(0.00445700000153134,-0.0375679687511446,-0.0121757845426831));
#18225=CARTESIAN_POINT('Ctrl Pts',(0.00445700000200862,-0.0375679682467928,
-0.0121757745554097));
#18226=CARTESIAN_POINT('Ctrl Pts',(0.00445700000083941,-0.0375679695720835,
-0.0121758007991274));
#18227=CARTESIAN_POINT('Ctrl Pts',(0.004457,-0.0375679708973641,-0.0121758270428433));
#18228=CARTESIAN_POINT('Ctrl Pts',(0.004457,-0.037567972222619,-0.0121758532865581));
#18229=CARTESIAN_POINT('Ctrl Pts',(0.00445700000153134,-0.0375679687511446,
-0.0121757845426831));
#18230=CARTESIAN_POINT('Ctrl Pts',(0.00445700036683925,-0.0375675546782457,
-0.0121675849742589));
#18231=CARTESIAN_POINT('Ctrl Pts',(0.004457066091393,-0.0375671386197308,
-0.0121593856361153));
#18232=CARTESIAN_POINT('Ctrl Pts',(0.00445733677550361,-0.037566275221113,
-0.0121424549421407));
#18233=CARTESIAN_POINT('Ctrl Pts',(0.00445755052059262,-0.03756582762505,
-0.0121337240450385));
#18234=CARTESIAN_POINT('Ctrl Pts',(0.00445833751673252,-0.0375645975608631,
-0.0121098599235097));
#18235=CARTESIAN_POINT('Ctrl Pts',(0.00445905944675096,-0.0375638105169478,
-0.0120947328458213));
#18236=CARTESIAN_POINT('Ctrl Pts',(0.00446155134286164,-0.0375617156770453,
-0.0120548560197195));
#18237=CARTESIAN_POINT('Ctrl Pts',(0.0044636957851817,-0.037560396480823,
-0.0120301348115956));
#18238=CARTESIAN_POINT('Ctrl Pts',(0.00447852383692101,-0.0375531609460893,
-0.0118966668724493));
#18239=CARTESIAN_POINT('Ctrl Pts',(0.00450215713675417,-0.0375469090791664,
-0.011789465728744));
#18240=CARTESIAN_POINT('Ctrl Pts',(0.00455415940330839,-0.037537513609922,
-0.011634247692209));
#18241=CARTESIAN_POINT('Ctrl Pts',(0.00457409310536596,-0.0375344053760627,
-0.0115837539491281));
#18242=CARTESIAN_POINT('Ctrl Pts',(0.00460952027265135,-0.0375296448493669,
-0.0115062457089519));
#18243=CARTESIAN_POINT('Ctrl Pts',(0.00462324101949698,-0.0375279415203038,
-0.0114784702343028));
#18244=CARTESIAN_POINT('Ctrl Pts',(0.00464315607613126,-0.037525667984562,
-0.0114410375780365));
#18245=CARTESIAN_POINT('Ctrl Pts',(0.00464863488965225,-0.0375250611632817,
-0.0114310097372368));
#18246=CARTESIAN_POINT('Ctrl Pts',(0.0046581515367496,-0.0375240394412014,
-0.0114140421956841));
#18247=CARTESIAN_POINT('Ctrl Pts',(0.00466213298287001,-0.0375236211993594,
-0.0114070715937107));
#18248=CARTESIAN_POINT('Ctrl Pts',(0.00467079890131458,-0.0375227307038318,
-0.0113921707890997));
#18249=CARTESIAN_POINT('Ctrl Pts',(0.00467550021541715,-0.0375222594936024,
-0.011384251021267));
#18250=CARTESIAN_POINT('Ctrl Pts',(0.00468899872004694,-0.0375209383175919,
-0.0113619685894859));
#18251=CARTESIAN_POINT('Ctrl Pts',(0.00469796076624327,-0.0375200981518808,
-0.0113477068426694));
#18252=CARTESIAN_POINT('Ctrl Pts',(0.0047666831178511,-0.0375139032600975,
-0.0112422198767264));
#18253=CARTESIAN_POINT('Ctrl Pts',(0.00483573667388354,-0.0375090149274492,
-0.0111574046017778));
#18254=CARTESIAN_POINT('Ctrl Pts',(0.00495192617621242,-0.0375014841625381,
-0.011042110701276));
#18255=CARTESIAN_POINT('Ctrl Pts',(0.00499270164061338,-0.0374989480608549,
-0.0110057333950119));
#18256=CARTESIAN_POINT('Ctrl Pts',(0.00506473205692808,-0.037494539477578,
-0.0109480327509385));
#18257=CARTESIAN_POINT('Ctrl Pts',(0.00509499810502276,-0.0374927067697491,
-0.0109255570435091));
#18258=CARTESIAN_POINT('Ctrl Pts',(0.00514059554449525,-0.0374899547927506,
-0.0108942198522462));
#18259=CARTESIAN_POINT('Ctrl Pts',(0.00515530574282756,-0.0374890683793864,
-0.0108844773313338));
#18260=CARTESIAN_POINT('Ctrl Pts',(0.00518189678129539,-0.0374874669049695,
-0.0108675149170964));
#18261=CARTESIAN_POINT('Ctrl Pts',(0.00519371435586635,-0.0374867554790625,
-0.0108601992252512));
#18262=CARTESIAN_POINT('Ctrl Pts',(0.00521942598941529,-0.0374852075702802,
-0.0108447589166292));
#18263=CARTESIAN_POINT('Ctrl Pts',(0.00523335149436794,-0.0374843691820669,
-0.0108366900962038));
#18264=CARTESIAN_POINT('Ctrl Pts',(0.00527208242528318,-0.0374820364000232,
-0.0108150504413171));
#18265=CARTESIAN_POINT('Ctrl Pts',(0.00529713771615109,-0.0374805261187882,
-0.0108019417719247));
#18266=CARTESIAN_POINT('Ctrl Pts',(0.0054368125096652,-0.0374720988443577,
-0.0107336861720272));
#18267=CARTESIAN_POINT('Ctrl Pts',(0.00555754287442518,-0.0374647292666306,
-0.0106921925661276));
#18268=CARTESIAN_POINT('Ctrl Pts',(0.00573757933703765,-0.037454231120333,
-0.0106542704758986));
#18269=CARTESIAN_POINT('Ctrl Pts',(0.00579380023103691,-0.0374510284780135,
-0.0106456371166781));
#18270=CARTESIAN_POINT('Ctrl Pts',(0.00586394308740783,-0.0374472214141527,
-0.010638803056727));
#18271=CARTESIAN_POINT('Ctrl Pts',(0.00587753045972386,-0.0374464927284362,
-0.0106376607989248));
#18272=CARTESIAN_POINT('Ctrl Pts',(0.0058995572969287,-0.0374453275855413,
-0.0106361027838862));
#18273=CARTESIAN_POINT('Ctrl Pts',(0.00590798795073027,-0.0374448854571853,
-0.0106355759940659));
#18274=CARTESIAN_POINT('Ctrl Pts',(0.0059249253774154,-0.0374440054670575,
-0.0106346572222441));
#18275=CARTESIAN_POINT('Ctrl Pts',(0.00593343188448871,-0.0374435676700767,
-0.0106342663768265));
#18276=CARTESIAN_POINT('Ctrl Pts',(0.00595582615989271,-0.0374424250766993,
-0.0106334231480532));
#18277=CARTESIAN_POINT('Ctrl Pts',(0.00596971781879187,-0.0374417263660004,
-0.0106330878880061));
#18278=CARTESIAN_POINT('Ctrl Pts',(0.00604182414024253,-0.0374381433454097,
-0.0106323220389861));
#18279=CARTESIAN_POINT('Ctrl Pts',(0.00610002915600085,-0.0374353979734819,
-0.0106349985707756));
#18280=CARTESIAN_POINT('Ctrl Pts',(0.0062496461293218,-0.037428424753463,
-0.0106503948495736));
#18281=CARTESIAN_POINT('Ctrl Pts',(0.00634031302894067,-0.037424270897813,
-0.010668029077274));
#18282=CARTESIAN_POINT('Ctrl Pts',(0.00647757486073544,-0.0374175503828472,
-0.0107077447724282));
#18283=CARTESIAN_POINT('Ctrl Pts',(0.00652555764722635,-0.0374151173768708,
-0.0107242304229163));
#18284=CARTESIAN_POINT('Ctrl Pts',(0.00659075670370055,-0.0374116442747195,
-0.0107502880731383));
#18285=CARTESIAN_POINT('Ctrl Pts',(0.00660873436705773,-0.0374106685936182,
-0.0107578715912458));
#18286=CARTESIAN_POINT('Ctrl Pts',(0.0066396071801554,-0.0374089593369137,
-0.0107715899906488));
#18287=CARTESIAN_POINT('Ctrl Pts',(0.00665257008243262,-0.0374082311462968,
-0.0107775668284452));
#18288=CARTESIAN_POINT('Ctrl Pts',(0.00667920375237414,-0.0374067123600755,
-0.0107902979029145));
#18289=CARTESIAN_POINT('Ctrl Pts',(0.00669286102072801,-0.0374059209788032,
-0.0107970766395812));
#18290=CARTESIAN_POINT('Ctrl Pts',(0.0067283833117898,-0.0374038286161549,
-0.0108153690640117));
#18291=CARTESIAN_POINT('Ctrl Pts',(0.00675007551911772,-0.0374025164953747,
-0.0108272072281915));
#18292=CARTESIAN_POINT('Ctrl Pts',(0.0068700111172489,-0.0373950642134218,
-0.0108964488881031));
#18293=CARTESIAN_POINT('Ctrl Pts',(0.00696194191788553,-0.0373885570674098,
-0.0109640547249231));
#18294=CARTESIAN_POINT('Ctrl Pts',(0.00708399771578481,-0.0373790338193812,
-0.0110765238618972));
#18295=CARTESIAN_POINT('Ctrl Pts',(0.00712058252476247,-0.0373760456902483,
-0.0111138403540489));
#18296=CARTESIAN_POINT('Ctrl Pts',(0.00717527849721377,-0.0373714413427317,
-0.0111756101955631));
#18297=CARTESIAN_POINT('Ctrl Pts',(0.00719468087906294,-0.0373697775682962,
-0.0111988662842938));
#18298=CARTESIAN_POINT('Ctrl Pts',(0.00722039464420038,-0.0373675464793812,
-0.0112315998325648));
#18299=CARTESIAN_POINT('Ctrl Pts',(0.00722730355542674,-0.0373669442667177,
-0.0112405973479549));
#18300=CARTESIAN_POINT('Ctrl Pts',(0.00723891757216372,-0.0373659283631549,
-0.011256072702156));
#18301=CARTESIAN_POINT('Ctrl Pts',(0.00724367257172003,-0.0373655113977234,
-0.0112625123760226));
#18302=CARTESIAN_POINT('Ctrl Pts',(0.00725377398820771,-0.037364623735917,
-0.0112764178554385));
#18303=CARTESIAN_POINT('Ctrl Pts',(0.00725910419246762,-0.0373641540858661,
-0.0112838947959566));
#18304=CARTESIAN_POINT('Ctrl Pts',(0.0072740536613627,-0.0373628319007741,
-0.011305266223386));
#18305=CARTESIAN_POINT('Ctrl Pts',(0.00728351209778681,-0.0373619893569193,
-0.0113192721142523));
#18306=CARTESIAN_POINT('Ctrl Pts',(0.00734754084555967,-0.0373562226148416,
-0.0114175274206311));
#18307=CARTESIAN_POINT('Ctrl Pts',(0.00739401157649186,-0.0373516961613388,
-0.0115067791373772));
#18308=CARTESIAN_POINT('Ctrl Pts',(0.00746243966882219,-0.0373432940227781,
-0.0116768575188318));
#18309=CARTESIAN_POINT('Ctrl Pts',(0.00748713932881683,-0.0373394561462299,
-0.0117561609103953));
#18310=CARTESIAN_POINT('Ctrl Pts',(0.007511045570467,-0.0373341551442661,
-0.0118623823723639));
#18311=CARTESIAN_POINT('Ctrl Pts',(0.00751610465056322,-0.0373328736306451,
-0.011887844047252));
#18312=CARTESIAN_POINT('Ctrl Pts',(0.00752313988089788,-0.0373307991420372,
-0.0119286057033465));
#18313=CARTESIAN_POINT('Ctrl Pts',(0.00752553309264297,-0.0373300193551603,
-0.0119438290953035));
#18314=CARTESIAN_POINT('Ctrl Pts',(0.00752967067934738,-0.0373285150887994,
-0.0119729892418283));
#18315=CARTESIAN_POINT('Ctrl Pts',(0.00753145356782104,-0.0373277919089775,
-0.0119869190116834));
#18316=CARTESIAN_POINT('Ctrl Pts',(0.00753511882058764,-0.0373261135709884,
-0.0120190308186336));
#18317=CARTESIAN_POINT('Ctrl Pts',(0.00753686870113858,-0.037325154357965,
-0.012037225595434));
#18318=CARTESIAN_POINT('Ctrl Pts',(0.00754143203016847,-0.0373220533324374,
-0.0120955259236818));
#18319=CARTESIAN_POINT('Ctrl Pts',(0.00754300139234045,-0.0373198739337048,
-0.0121357097610633));
#18320=CARTESIAN_POINT('Ctrl Pts',(0.0075429978187607,-0.0373141789562194,
-0.0122388179429579));
#18321=CARTESIAN_POINT('Ctrl Pts',(0.00753914814721549,-0.0373106074087205,
-0.0123016657468015));
#18322=CARTESIAN_POINT('Ctrl Pts',(0.00751960223318753,-0.0373014257575527,
-0.0124606816976951));
#18323=CARTESIAN_POINT('Ctrl Pts',(0.00749862014934309,-0.0372957809931752,
-0.0125559292485683));
#18324=CARTESIAN_POINT('Ctrl Pts',(0.00746391223862542,-0.0372896181361719,
-0.0126637723737436));
#18325=CARTESIAN_POINT('Ctrl Pts',(0.00745878334720777,-0.0372887595169188,
-0.0126788992712031));
#18326=CARTESIAN_POINT('Ctrl Pts',(0.00745043058387969,-0.0372874416061686,
-0.0127023315914479));
#18327=CARTESIAN_POINT('Ctrl Pts',(0.00744736822694468,-0.0372869737693592,
-0.0127106929891292));
#18328=CARTESIAN_POINT('Ctrl Pts',(0.00744137248617305,-0.0372860871171274,
-0.0127266349250464));
#18329=CARTESIAN_POINT('Ctrl Pts',(0.00743845132405704,-0.0372856676704713,
-0.0127342195167429));
#18330=CARTESIAN_POINT('Ctrl Pts',(0.00743105918551647,-0.0372846359532452,
-0.0127529696147484));
#18331=CARTESIAN_POINT('Ctrl Pts',(0.00742651723500039,-0.0372840277243301,
-0.0127641068406663));
#18332=CARTESIAN_POINT('Ctrl Pts',(0.00740791653239397,-0.0372816319761763,
-0.0128082344845304));
#18333=CARTESIAN_POINT('Ctrl Pts',(0.00739283903672585,-0.0372798964208051,
-0.0128407853772031));
#18334=CARTESIAN_POINT('Ctrl Pts',(0.00734493960735212,-0.0372748657479876,
-0.0129354007355388));
#18335=CARTESIAN_POINT('Ctrl Pts',(0.00730900242836076,-0.0372716707543755,
-0.0129957852335895));
#18336=CARTESIAN_POINT('Ctrl Pts',(0.00721956307573803,-0.0372644591299455,
-0.0131251123255407));
#18337=CARTESIAN_POINT('Ctrl Pts',(0.00716408109886085,-0.0372604366230465,
-0.0131923868203658));
#18338=CARTESIAN_POINT('Ctrl Pts',(0.00708503837444482,-0.0372549273831142,
-0.0132732217595692));
#18339=CARTESIAN_POINT('Ctrl Pts',(0.00706638272686283,-0.0372536419645699,
-0.0132913592807271));
#18340=CARTESIAN_POINT('Ctrl Pts',(0.00703586695466366,-0.0372515567934154,
-0.0133195622053423));
#18341=CARTESIAN_POINT('Ctrl Pts',(0.00702429742344623,-0.0372507700642419,
-0.0133299352613626));
#18342=CARTESIAN_POINT('Ctrl Pts',(0.0070018383465379,-0.0372492490353765,
-0.0133494679326557));
#18343=CARTESIAN_POINT('Ctrl Pts',(0.00699097485842589,-0.0372485159869813,
-0.0133586551390801));
#18344=CARTESIAN_POINT('Ctrl Pts',(0.00696534417377876,-0.0372467919535568,
-0.0133797299237081));
#18345=CARTESIAN_POINT('Ctrl Pts',(0.00695048208177023,-0.0372457963723621,
-0.0133914980131092));
#18346=CARTESIAN_POINT('Ctrl Pts',(0.00689872123111179,-0.0372423416385964,
-0.0134309537000006));
#18347=CARTESIAN_POINT('Ctrl Pts',(0.00686080230786232,-0.0372398313314462,
-0.0134572570927065));
#18348=CARTESIAN_POINT('Ctrl Pts',(0.00675704604002398,-0.0372330255087243,
-0.0135225444867078));
#18349=CARTESIAN_POINT('Ctrl Pts',(0.00668939375266912,-0.0372286464948173,
-0.0135583982849544));
#18350=CARTESIAN_POINT('Ctrl Pts',(0.00655178285281245,-0.0372200334028997,
-0.0136187080353799));
#18351=CARTESIAN_POINT('Ctrl Pts',(0.00648215511062513,-0.0372158120649407,
-0.0136434438346568));
#18352=CARTESIAN_POINT('Ctrl Pts',(0.00639425967259434,-0.0372108396799751,
-0.0136677348842645));
#18353=CARTESIAN_POINT('Ctrl Pts',(0.00637742078717573,-0.0372099030030866,
-0.013672083545818));
#18354=CARTESIAN_POINT('Ctrl Pts',(0.0063514911051979,-0.0372084886935629,
-0.0136783142896055));
#18355=CARTESIAN_POINT('Ctrl Pts',(0.00634245128303714,-0.0372080008106931,
-0.0136804004576085));
#18356=CARTESIAN_POINT('Ctrl Pts',(0.00632534517926319,-0.0372070880791505,
-0.0136841859597881));
#18357=CARTESIAN_POINT('Ctrl Pts',(0.00631728325447214,-0.0372066623618087,
-0.01368590238398));
#18358=CARTESIAN_POINT('Ctrl Pts',(0.00629754519214838,-0.0372056301708268,
-0.0136899396669655));
#18359=CARTESIAN_POINT('Ctrl Pts',(0.00628585496735973,-0.0372050274127528,
-0.0136921902090326));
#18360=CARTESIAN_POINT('Ctrl Pts',(0.00624115918010713,-0.0372027515779952,
-0.0137002595339077));
#18361=CARTESIAN_POINT('Ctrl Pts',(0.00620799158463117,-0.0372011221897333,
-0.013705138061047));
#18362=CARTESIAN_POINT('Ctrl Pts',(0.00611278983737598,-0.0371965502406656,
-0.0137159860027831));
#18363=CARTESIAN_POINT('Ctrl Pts',(0.0060505169583431,-0.0371936842479466,
-0.0137192842186365));
#18364=CARTESIAN_POINT('Ctrl Pts',(0.00589621090538066,-0.0371865709334765,
-0.0137181054416812));
#18365=CARTESIAN_POINT('Ctrl Pts',(0.00580445998840567,-0.0371823212708795,
-0.0137091753127247));
#18366=CARTESIAN_POINT('Ctrl Pts',(0.0056888613771523,-0.037176578327035,
-0.0136873754193712));
#18367=CARTESIAN_POINT('Ctrl Pts',(0.00566378896351049,-0.0371753098393779,
-0.0136819968550634));
#18368=CARTESIAN_POINT('Ctrl Pts',(0.00562373997997504,-0.0371732409887976,
-0.0136723556612654));
#18369=CARTESIAN_POINT('Ctrl Pts',(0.00560867323883922,-0.037172452864617,
-0.0136684866320135));
#18370=CARTESIAN_POINT('Ctrl Pts',(0.00557976098804718,-0.03717092042846,
-0.013660594336834));
#18371=CARTESIAN_POINT('Ctrl Pts',(0.00556590828193305,-0.0371701772117645,
-0.0136566034935576));
#18372=CARTESIAN_POINT('Ctrl Pts',(0.00553346071652693,-0.0371684143765495,
-0.0136467611860309));
#18373=CARTESIAN_POINT('Ctrl Pts',(0.00551491710228931,-0.037167389752226,
-0.0136407503779218));
#18374=CARTESIAN_POINT('Ctrl Pts',(0.00544988287782188,-0.0371637337486952,
-0.013618299661399));
#18375=CARTESIAN_POINT('Ctrl Pts',(0.00540407476868716,-0.0371610432282816,
-0.0135999855898826));
#18376=CARTESIAN_POINT('Ctrl Pts',(0.00528113155401764,-0.0371535134887665,
-0.0135438615638305));
#18377=CARTESIAN_POINT('Ctrl Pts',(0.0052061537061278,-0.0371485647664251,
-0.0135017585197347));
#18378=CARTESIAN_POINT('Ctrl Pts',(0.00507860386490017,-0.0371397378488797,
-0.0134154208772557));
#18379=CARTESIAN_POINT('Ctrl Pts',(0.0050247267537187,-0.0371358618188004,
-0.0133734935581902));
#18380=CARTESIAN_POINT('Ctrl Pts',(0.00496327450046798,-0.0371314099478229,
-0.0133187652591531));
#18381=CARTESIAN_POINT('Ctrl Pts',(0.00495288056979588,-0.0371306559439367,
-0.0133092501564194));
#18382=CARTESIAN_POINT('Ctrl Pts',(0.004936401900974,-0.0371294609968974,
-0.0132937445768664));
#18383=CARTESIAN_POINT('Ctrl Pts',(0.00493023420373071,-0.0371290138551249,
-0.0132878438445751));
#18384=CARTESIAN_POINT('Ctrl Pts',(0.00491840823320606,-0.037128157293777,
-0.0132763402911021));
#18385=CARTESIAN_POINT('Ctrl Pts',(0.00491274408740752,-0.0371277474741468,
-0.0132707445970626));
#18386=CARTESIAN_POINT('Ctrl Pts',(0.00489840297896655,-0.0371267107361774,
-0.0132563557584913));
#18387=CARTESIAN_POINT('Ctrl Pts',(0.00488978794184987,-0.0371260886438505,
-0.013247501920157));
#18388=CARTESIAN_POINT('Ctrl Pts',(0.00485110529340055,-0.0371232932042599,
-0.0132067798143143));
#18389=CARTESIAN_POINT('Ctrl Pts',(0.00482229490831655,-0.0371212048971061,
-0.0131737409864193));
#18390=CARTESIAN_POINT('Ctrl Pts',(0.00472690436993282,-0.0371140883404748,
-0.013054454228842));
#18391=CARTESIAN_POINT('Ctrl Pts',(0.0046680773447329,-0.0371093006658215,
-0.0129624256491001));
#18392=CARTESIAN_POINT('Ctrl Pts',(0.0045941558243124,-0.0371016288004911,
-0.0128143310011492));
#18393=CARTESIAN_POINT('Ctrl Pts',(0.00457168820640274,-0.0370989459360733,
-0.0127623481655958));
#18394=CARTESIAN_POINT('Ctrl Pts',(0.00454519485622604,-0.0370951774976147,
-0.0126904338707258));
#18395=CARTESIAN_POINT('Ctrl Pts',(0.00453862997742936,-0.0370941795294457,
-0.012671482979072));
#18396=CARTESIAN_POINT('Ctrl Pts',(0.00452859850786245,-0.0370925425153628,
-0.012640590923695));
#18397=CARTESIAN_POINT('Ctrl Pts',(0.00452490351678714,-0.0370919113836385,
-0.0126287260891729));
#18398=CARTESIAN_POINT('Ctrl Pts',(0.00451742936429641,-0.0370905726751009,
-0.0126036636878704));
#18399=CARTESIAN_POINT('Ctrl Pts',(0.00451368222439348,-0.0370898640717603,
-0.0125904577755391));
#18400=CARTESIAN_POINT('Ctrl Pts',(0.00450500606134507,-0.0370881275338222,
-0.0125582502453487));
#18401=CARTESIAN_POINT('Ctrl Pts',(0.00450026258437286,-0.0370870934650772,
-0.0125392015287696));
#18402=CARTESIAN_POINT('Ctrl Pts',(0.00448311486713233,-0.0370829972426645,
-0.0124642711175056));
#18403=CARTESIAN_POINT('Ctrl Pts',(0.00447346168928386,-0.0370798466612121,
-0.012407812369097));
#18404=CARTESIAN_POINT('Ctrl Pts',(0.0044603274821594,-0.0370733288368832,
-0.012292819406208));
#18405=CARTESIAN_POINT('Ctrl Pts',(0.00445699999999927,-0.0370699635392117,
-0.0122343585838898));
#18406=CARTESIAN_POINT('Ctrl Pts',(0.004457,-0.0370665921755392,-0.0121758532865387));
#18407=CARTESIAN_POINT('Ctrl Pts',(0.004457,-0.0376822061652104,-0.0121758532865636));
#18408=CARTESIAN_POINT('Ctrl Pts',(0.004457,-0.0376821983899012,-0.0121757169191301));
#18409=CARTESIAN_POINT('Ctrl Pts',(0.00445700001808376,-0.0376821906147461,
-0.0121755805512917));
#18410=CARTESIAN_POINT('Ctrl Pts',(0.00445702249714396,-0.037677356706163,
-0.0120907971419327));
#18411=CARTESIAN_POINT('Ctrl Pts',(0.00446401023444583,-0.0376726175689111,
-0.0120062872456995));
#18412=CARTESIAN_POINT('Ctrl Pts',(0.00448164007563339,-0.0376668620486047,
-0.0119002577688501));
#18413=CARTESIAN_POINT('Ctrl Pts',(0.00448588206624491,-0.0376656549327456,
-0.0118778319706476));
#18414=CARTESIAN_POINT('Ctrl Pts',(0.00449377393537067,-0.0376636697411631,
-0.0118406476637458));
#18415=CARTESIAN_POINT('Ctrl Pts',(0.00449714712307352,-0.0376628832558311,
-0.0118258346883064));
#18416=CARTESIAN_POINT('Ctrl Pts',(0.00450429976257569,-0.0376613304500835,
-0.0117964370098263));
#18417=CARTESIAN_POINT('Ctrl Pts',(0.00450807515227078,-0.0376605641009239,
-0.0117818530576273));
#18418=CARTESIAN_POINT('Ctrl Pts',(0.00451792543255403,-0.0376586876087716,
-0.0117459763727549));
#18419=CARTESIAN_POINT('Ctrl Pts',(0.00452424628365089,-0.0376575853155197,
-0.0117247543909254));
#18420=CARTESIAN_POINT('Ctrl Pts',(0.00455468739899603,-0.0376526918995844,
-0.0116300500309386));
#18421=CARTESIAN_POINT('Ctrl Pts',(0.00458385579798844,-0.0376490619789112,
-0.0115583042819736));
#18422=CARTESIAN_POINT('Ctrl Pts',(0.0046677939372941,-0.0376403489136198,
-0.0113894381773857));
#18423=CARTESIAN_POINT('Ctrl Pts',(0.00472792502657949,-0.0376353593281247,
-0.0112954886199944));
#18424=CARTESIAN_POINT('Ctrl Pts',(0.00480845391318702,-0.0376290346887517,
-0.0111953607431604));
#18425=CARTESIAN_POINT('Ctrl Pts',(0.00481951062290811,-0.0376281722933577,
-0.0111820764051238));
#18426=CARTESIAN_POINT('Ctrl Pts',(0.00483690493349415,-0.0376268198088133,
-0.0111618775733889));
#18427=CARTESIAN_POINT('Ctrl Pts',(0.00484308662687585,-0.0376263399447525,
-0.011154830113861));
#18428=CARTESIAN_POINT('Ctrl Pts',(0.0048548997317603,-0.0376254234627615,
-0.0111416075645628));
#18429=CARTESIAN_POINT('Ctrl Pts',(0.00486051769591762,-0.0376249877471595,
-0.0111354212105127));
#18430=CARTESIAN_POINT('Ctrl Pts',(0.00487448403784089,-0.0376239053912461,
-0.0111202906350169));
#18431=CARTESIAN_POINT('Ctrl Pts',(0.00488288899638949,-0.037623254802692,
-0.0111113995863379));
#18432=CARTESIAN_POINT('Ctrl Pts',(0.00491640107119769,-0.03762066720149,
-0.0110767834602418));
#18433=CARTESIAN_POINT('Ctrl Pts',(0.00494229692903798,-0.0376186817512341,
-0.0110518403848605));
#18434=CARTESIAN_POINT('Ctrl Pts',(0.00502136260936218,-0.0376127202419409,
-0.0109808371149455));
#18435=CARTESIAN_POINT('Ctrl Pts',(0.00507683709268155,-0.0376086672246894,
-0.0109374814912981));
#18436=CARTESIAN_POINT('Ctrl Pts',(0.00520453955408694,-0.0375998600917408,
-0.0108510408065051));
#18437=CARTESIAN_POINT('Ctrl Pts',(0.00527773036734072,-0.037595140243852,
-0.0108097585416849));
#18438=CARTESIAN_POINT('Ctrl Pts',(0.00537762056247263,-0.0375892102211124,
-0.0107637010746876));
#18439=CARTESIAN_POINT('Ctrl Pts',(0.00540159361452585,-0.0375878223017475,
-0.0107533765944144));
#18440=CARTESIAN_POINT('Ctrl Pts',(0.0054405152621558,-0.0375856242761721,
-0.0107377724277635));
#18441=CARTESIAN_POINT('Ctrl Pts',(0.00545530267491293,-0.037584801706765,
-0.0107321065716766));
#18442=CARTESIAN_POINT('Ctrl Pts',(0.0054839684975815,-0.0375832304825638,
-0.0107216262827532));
#18443=CARTESIAN_POINT('Ctrl Pts',(0.00549783352443621,-0.0375824808751488,
-0.0107167804508415));
#18444=CARTESIAN_POINT('Ctrl Pts',(0.00553064378375233,-0.0375807303220066,
-0.0107058363596132));
#18445=CARTESIAN_POINT('Ctrl Pts',(0.00554964217272093,-0.0375797347947286,
-0.0106999051521767));
#18446=CARTESIAN_POINT('Ctrl Pts',(0.00561782267326762,-0.0375762213445696,
-0.010680058646221));
#18447=CARTESIAN_POINT('Ctrl Pts',(0.00566757630504001,-0.0375737676418703,
-0.01066822064498));
#18448=CARTESIAN_POINT('Ctrl Pts',(0.00580955004207624,-0.0375669696125143,
-0.0106418123286862));
#18449=CARTESIAN_POINT('Ctrl Pts',(0.00590262687148162,-0.037562759715691,
-0.0106331054044798));
#18450=CARTESIAN_POINT('Ctrl Pts',(0.00605126616104672,-0.0375558433495857,
-0.0106327123118396));
#18451=CARTESIAN_POINT('Ctrl Pts',(0.00610657660049057,-0.0375532233499259,
-0.0106355439827025));
#18452=CARTESIAN_POINT('Ctrl Pts',(0.00617550388538196,-0.0375497776150157,
-0.0106428032046979));
#18453=CARTESIAN_POINT('Ctrl Pts',(0.00618937631668384,-0.0375490748288729,
-0.0106444549867308));
#18454=CARTESIAN_POINT('Ctrl Pts',(0.00621183366259654,-0.0375479193566133,
-0.010647438769779));
#18455=CARTESIAN_POINT('Ctrl Pts',(0.00622043340817816,-0.0375474726396624,
-0.0106486553481972));
#18456=CARTESIAN_POINT('Ctrl Pts',(0.00623775067485377,-0.037546563721024,
-0.0106512544810376));
#18457=CARTESIAN_POINT('Ctrl Pts',(0.00624646747082618,-0.0375461014259477,
-0.0106526393555384));
#18458=CARTESIAN_POINT('Ctrl Pts',(0.00626959841868577,-0.0375448628265635,
-0.0106565180124865));
#18459=CARTESIAN_POINT('Ctrl Pts',(0.00628398951923239,-0.037544079957627,
-0.0106591420728864));
#18460=CARTESIAN_POINT('Ctrl Pts',(0.0063782115717785,-0.037538883224458,
-0.0106777103935569));
#18461=CARTESIAN_POINT('Ctrl Pts',(0.0064567061052238,-0.0375342242950894,
-0.0106997456356024));
#18462=CARTESIAN_POINT('Ctrl Pts',(0.00663120722308047,-0.0375235783645969,
-0.0107639898541918));
#18463=CARTESIAN_POINT('Ctrl Pts',(0.00672541144264658,-0.0375176315463681,
-0.010809996625809));
#18464=CARTESIAN_POINT('Ctrl Pts',(0.00683606850738029,-0.0375106141710772,
-0.0108787416895683));
#18465=CARTESIAN_POINT('Ctrl Pts',(0.00685755023799678,-0.0375092486823873,
-0.0108928424773348));
#18466=CARTESIAN_POINT('Ctrl Pts',(0.00689162378409269,-0.0375070768518482,
-0.0109164469467425));
#18467=CARTESIAN_POINT('Ctrl Pts',(0.0069044389319358,-0.0375062585871621,
-0.0109256182912334));
#18468=CARTESIAN_POINT('Ctrl Pts',(0.00692895281527635,-0.0375046898991506,
-0.0109437362177048));
#18469=CARTESIAN_POINT('Ctrl Pts',(0.0069406683365693,-0.0375039386284311,
-0.0109526571027446));
#18470=CARTESIAN_POINT('Ctrl Pts',(0.00696809069859235,-0.0375021754063024,
-0.0109741651192625));
#18471=CARTESIAN_POINT('Ctrl Pts',(0.00698368265019711,-0.0375011691044739,
-0.0109868946909788));
#18472=CARTESIAN_POINT('Ctrl Pts',(0.00703939594029263,-0.0374975542438987,
-0.0110342265121515));
#18473=CARTESIAN_POINT('Ctrl Pts',(0.00707797878024858,-0.037495015271026,
-0.0110705849951919));
#18474=CARTESIAN_POINT('Ctrl Pts',(0.00718464362119928,-0.0374877673061877,
-0.0111820105473435));
#18475=CARTESIAN_POINT('Ctrl Pts',(0.00724729560961758,-0.0374832203713592,
-0.011261874868321));
#18476=CARTESIAN_POINT('Ctrl Pts',(0.00731674825861279,-0.0374771541419818,
-0.0113709859433026));
#18477=CARTESIAN_POINT('Ctrl Pts',(0.00733117597733396,-0.0374758215376672,
-0.0113950794274066));
#18478=CARTESIAN_POINT('Ctrl Pts',(0.00735686320852034,-0.0374732838909979,
-0.0114407592847954));
#18479=CARTESIAN_POINT('Ctrl Pts',(0.0073682848189581,-0.0374720859029069,
-0.0114622445013686));
#18480=CARTESIAN_POINT('Ctrl Pts',(0.00738392524632726,-0.0374703287901045,
-0.0114934228576332));
#18481=CARTESIAN_POINT('Ctrl Pts',(0.00738856031706123,-0.0374697920364909,
-0.0115029040968448));
#18482=CARTESIAN_POINT('Ctrl Pts',(0.00739661936599757,-0.0374688284443794,
-0.0115198270390851));
#18483=CARTESIAN_POINT('Ctrl Pts',(0.00740008191421842,-0.03746840386379,
-0.0115272496174671));
#18484=CARTESIAN_POINT('Ctrl Pts',(0.00740776482080798,-0.0374674373186778,
-0.0115440674999729));
#18485=CARTESIAN_POINT('Ctrl Pts',(0.00741195032133339,-0.0374668934620033,
-0.0115534777169207));
#18486=CARTESIAN_POINT('Ctrl Pts',(0.0074248586077519,-0.0374651620118918,
-0.0115832997715091));
#18487=CARTESIAN_POINT('Ctrl Pts',(0.00743323501150416,-0.0374639568670845,
-0.0116038576320402));
#18488=CARTESIAN_POINT('Ctrl Pts',(0.00745271016618792,-0.0374609563357964,
-0.0116547712388972));
#18489=CARTESIAN_POINT('Ctrl Pts',(0.00746330411812472,-0.0374591431795591,
-0.0116853084856268));
#18490=CARTESIAN_POINT('Ctrl Pts',(0.00751547155275493,-0.0374492220565311,
-0.0118524592544573));
#18491=CARTESIAN_POINT('Ctrl Pts',(0.00753889408427512,-0.0374409174894126,
-0.0119940415693968));
#18492=CARTESIAN_POINT('Ctrl Pts',(0.00754313739746618,-0.0374318924433555,
-0.0121617693645397));
#18493=CARTESIAN_POINT('Ctrl Pts',(0.00754316342641352,-0.0374305679844783,
-0.0121867215180258));
#18494=CARTESIAN_POINT('Ctrl Pts',(0.00754222236655664,-0.0374284450963234,
-0.0122272582957389));
#18495=CARTESIAN_POINT('Ctrl Pts',(0.00754162390736574,-0.0374276356721985,
-0.0122428462296096));
#18496=CARTESIAN_POINT('Ctrl Pts',(0.00753999875788756,-0.03742607376452,
-0.0122731723482762));
#18497=CARTESIAN_POINT('Ctrl Pts',(0.00753899657698308,-0.0374253206209278,
-0.0122879100999666));
#18498=CARTESIAN_POINT('Ctrl Pts',(0.0075360979178634,-0.0374235369610373,
-0.0123230699858119));
#18499=CARTESIAN_POINT('Ctrl Pts',(0.00753400558251348,-0.0374225125152147,
-0.0123434733669885));
#18500=CARTESIAN_POINT('Ctrl Pts',(0.00752461595810618,-0.0374187055939707,
-0.0124199738385339));
#18501=CARTESIAN_POINT('Ctrl Pts',(0.00751464249878353,-0.037416003759487,
-0.0124756990944652));
#18502=CARTESIAN_POINT('Ctrl Pts',(0.00747376146849427,-0.0374076804308529,
-0.0126486717499723));
#18503=CARTESIAN_POINT('Ctrl Pts',(0.00743210339603019,-0.0374023040266418,
-0.0127628844676466));
#18504=CARTESIAN_POINT('Ctrl Pts',(0.00736568852945161,-0.0373952023856881,
-0.0128944864390118));
#18505=CARTESIAN_POINT('Ctrl Pts',(0.00735325962921836,-0.0373939152317161,
-0.0129176261662842));
#18506=CARTESIAN_POINT('Ctrl Pts',(0.00733517308707057,-0.0373920824533119,
-0.0129493302906303));
#18507=CARTESIAN_POINT('Ctrl Pts',(0.00733001093581626,-0.0373915635584854,
-0.012958173392676));
#18508=CARTESIAN_POINT('Ctrl Pts',(0.00732048177057484,-0.0373906120126245,
-0.0129741305338813));
#18509=CARTESIAN_POINT('Ctrl Pts',(0.00731614425601137,-0.0373901811349147,
-0.0129812618575723));
#18510=CARTESIAN_POINT('Ctrl Pts',(0.00730680647957924,-0.0373892576755227,
-0.0129963372455667));
#18511=CARTESIAN_POINT('Ctrl Pts',(0.00730179132230508,-0.0373887642369093,
-0.0130042713250668));
#18512=CARTESIAN_POINT('Ctrl Pts',(0.00728730396493611,-0.0373873470726835,
-0.0130267341853457));
#18513=CARTESIAN_POINT('Ctrl Pts',(0.00727765900021106,-0.0373864133406789,
-0.0130411493247408));
#18514=CARTESIAN_POINT('Ctrl Pts',(0.00723122073545717,-0.0373819735987214,
-0.0131080853029943));
#18515=CARTESIAN_POINT('Ctrl Pts',(0.00719142141032065,-0.0373783299592346,
-0.0131584391388518));
#18516=CARTESIAN_POINT('Ctrl Pts',(0.00706774521995361,-0.0373677370707179,
-0.0132963150729106));
#18517=CARTESIAN_POINT('Ctrl Pts',(0.00697653680228718,-0.0373608008922294,
-0.0133766441056771));
#18518=CARTESIAN_POINT('Ctrl Pts',(0.00685730558447382,-0.0373530255358731,
-0.0134589904842994));
#18519=CARTESIAN_POINT('Ctrl Pts',(0.00683743810418692,-0.0373517661400594,
-0.0134720444133268));
#18520=CARTESIAN_POINT('Ctrl Pts',(0.00680423192873222,-0.0373497191905715,
-0.013492780205002));
#18521=CARTESIAN_POINT('Ctrl Pts',(0.00679106630928515,-0.0373489221165044,
-0.0135007304960838));
#18522=CARTESIAN_POINT('Ctrl Pts',(0.00676489082328246,-0.0373473650747437,
-0.0135160077100935));
#18523=CARTESIAN_POINT('Ctrl Pts',(0.00675188913838051,-0.0373466047880497,
-0.0135233452508863));
#18524=CARTESIAN_POINT('Ctrl Pts',(0.00672002868750576,-0.0373447722573444,
-0.0135407210505973));
#18525=CARTESIAN_POINT('Ctrl Pts',(0.00670106376593467,-0.0373437069874764,
-0.0135505587004084));
#18526=CARTESIAN_POINT('Ctrl Pts',(0.00662301489153961,-0.0373394185038155,
-0.0135890094989001));
#18527=CARTESIAN_POINT('Ctrl Pts',(0.00656233541584108,-0.0373363073012548,
-0.0136142336127846));
#18528=CARTESIAN_POINT('Ctrl Pts',(0.00644484741048625,-0.0373305308797699,
-0.0136544970020777));
#18529=CARTESIAN_POINT('Ctrl Pts',(0.00638842912809595,-0.0373278576209602,
-0.0136703094792597));
#18530=CARTESIAN_POINT('Ctrl Pts',(0.0062670691292105,-0.0373221238971621,
-0.0136969848319452));
#18531=CARTESIAN_POINT('Ctrl Pts',(0.00620205808420158,-0.0373190617216438,
-0.0137069764978541));
#18532=CARTESIAN_POINT('Ctrl Pts',(0.00611926892202126,-0.0373149718629774,
-0.0137143353811948));
#18533=CARTESIAN_POINT('Ctrl Pts',(0.00610189956618336,-0.037314103176606,
-0.0137155833485041));
#18534=CARTESIAN_POINT('Ctrl Pts',(0.00607511974164655,-0.0373127425987683,
-0.0137170523432732));
#18535=CARTESIAN_POINT('Ctrl Pts',(0.00606572170632952,-0.0373122610971433,
-0.0137174816972722));
#18536=CARTESIAN_POINT('Ctrl Pts',(0.0060479464523563,-0.0373113418328254,
-0.0137181309389245));
#18537=CARTESIAN_POINT('Ctrl Pts',(0.00603957043463689,-0.0373109049846501,
-0.0137183685663306));
#18538=CARTESIAN_POINT('Ctrl Pts',(0.00601894482892701,-0.0373098207476937,
-0.0137187856169297));
#18539=CARTESIAN_POINT('Ctrl Pts',(0.00600669435854373,-0.0373091694244024,
-0.0137188873918589));
#18540=CARTESIAN_POINT('Ctrl Pts',(0.00595857730818526,-0.0373065857307427,
-0.0137187141429715));
#18541=CARTESIAN_POINT('Ctrl Pts',(0.0059227278460709,-0.0373046054110942,
-0.0137173344404372));
#18542=CARTESIAN_POINT('Ctrl Pts',(0.00581708100760184,-0.0372986657796179,
-0.0137095740159387));
#18543=CARTESIAN_POINT('Ctrl Pts',(0.00574763281794559,-0.0372946305970241,
-0.0136996869745772));
#18544=CARTESIAN_POINT('Ctrl Pts',(0.00559739634266737,-0.0372858643966202,
-0.0136677434628822));
#18545=CARTESIAN_POINT('Ctrl Pts',(0.00551723213865605,-0.0372811671372832,
-0.0136437647250388));
#18546=CARTESIAN_POINT('Ctrl Pts',(0.00541510911312887,-0.037275259126433,
-0.0136039398422354));
#18547=CARTESIAN_POINT('Ctrl Pts',(0.00539106518799816,-0.0372738729400698,
-0.0135938543663173));
#18548=CARTESIAN_POINT('Ctrl Pts',(0.00535282918037681,-0.0372716757105772,
-0.0135766638455378));
#18549=CARTESIAN_POINT('Ctrl Pts',(0.00533847170844655,-0.0372708522986791,
-0.0135699410297759));
#18550=CARTESIAN_POINT('Ctrl Pts',(0.00531097887850482,-0.037269278111746,
-0.013556547254839));
#18551=CARTESIAN_POINT('Ctrl Pts',(0.00529783049928252,-0.0372685264072893,
-0.0135499071251397));
#18552=CARTESIAN_POINT('Ctrl Pts',(0.00526705488752359,-0.0372667687060703,
-0.0135338078397885));
#18553=CARTESIAN_POINT('Ctrl Pts',(0.00524951236730342,-0.0372657682020693,
-0.0135241920663343));
#18554=CARTESIAN_POINT('Ctrl Pts',(0.00518729557183864,-0.0372622198401728,
-0.0134884979353156));
#18555=CARTESIAN_POINT('Ctrl Pts',(0.00514375059639078,-0.037259737839284,
-0.0134605174517959));
#18556=CARTESIAN_POINT('Ctrl Pts',(0.00502393807064255,-0.037252804737251,
-0.013374726582427));
#18557=CARTESIAN_POINT('Ctrl Pts',(0.00495153203669132,-0.0372484957539897,
-0.013311946826388));
#18558=CARTESIAN_POINT('Ctrl Pts',(0.00484903587818129,-0.0372415848914354,
-0.0132048802117191));
#18559=CARTESIAN_POINT('Ctrl Pts',(0.00481463671439681,-0.0372390885589735,
-0.0131650589568449));
#18560=CARTESIAN_POINT('Ctrl Pts',(0.00477381281581633,-0.0372357831137204,
-0.0131126065887554));
#18561=CARTESIAN_POINT('Ctrl Pts',(0.00476543393386964,-0.0372350845052494,
-0.0131015359337883));
#18562=CARTESIAN_POINT('Ctrl Pts',(0.00475206850752643,-0.0372339341367546,
-0.0130833725012001));
#18563=CARTESIAN_POINT('Ctrl Pts',(0.00474699020064702,-0.037233488247222,
-0.0130763479121047));
#18564=CARTESIAN_POINT('Ctrl Pts',(0.00473689282366637,-0.0372325829688868,
-0.0130621298761833));
#18565=CARTESIAN_POINT('Ctrl Pts',(0.00473187537859859,-0.0372321234929344,
-0.0130549356882221));
#18566=CARTESIAN_POINT('Ctrl Pts',(0.0047186854282799,-0.0372308905180822,
-0.0130356755597257));
#18567=CARTESIAN_POINT('Ctrl Pts',(0.00471062222018163,-0.0372301104296057,
-0.01302353617799));
#18568=CARTESIAN_POINT('Ctrl Pts',(0.00469288009207113,-0.0372283367042366,
-0.0129959860014368));
#18569=CARTESIAN_POINT('Ctrl Pts',(0.0046832994779795,-0.0372273383517275,
-0.0129805145893346));
#18570=CARTESIAN_POINT('Ctrl Pts',(0.00465298141416091,-0.0372240519919394,
-0.0129295632001459));
#18571=CARTESIAN_POINT('Ctrl Pts',(0.00463338781477493,-0.0372217237235393,
-0.0128934245661015));
#18572=CARTESIAN_POINT('Ctrl Pts',(0.00459310040674032,-0.0372165105822372,
-0.0128114678809438));
#18573=CARTESIAN_POINT('Ctrl Pts',(0.00457315459911803,-0.037213620658179,
-0.0127653315629158));
#18574=CARTESIAN_POINT('Ctrl Pts',(0.00452846728969945,-0.0372063716407419,
-0.0126463326953032));
#18575=CARTESIAN_POINT('Ctrl Pts',(0.00450685428702723,-0.0372020612084549,
-0.0125724356020587));
#18576=CARTESIAN_POINT('Ctrl Pts',(0.00448544923810147,-0.0371965216288206,
-0.0124719185092907));
#18577=CARTESIAN_POINT('Ctrl Pts',(0.00448069691119912,-0.0371951456067359,
-0.0124464763769168));
#18578=CARTESIAN_POINT('Ctrl Pts',(0.00447408887733859,-0.0371929650938438,
-0.0124053996684703));
#18579=CARTESIAN_POINT('Ctrl Pts',(0.00447182863826404,-0.037192148287569,
-0.0123898360169502));
#18580=CARTESIAN_POINT('Ctrl Pts',(0.00446802693702081,-0.0371906263218655,
-0.0123605128143969));
#18581=CARTESIAN_POINT('Ctrl Pts',(0.00446643197969306,-0.0371899195791157,
-0.0123467618879886));
#18582=CARTESIAN_POINT('Ctrl Pts',(0.00446357384110298,-0.0371884980686156,
-0.0123188425726348));
#18583=CARTESIAN_POINT('Ctrl Pts',(0.0044623210995899,-0.0371877836829529,
-0.0123046744556103));
#18584=CARTESIAN_POINT('Ctrl Pts',(0.00446001899905396,-0.0371862397752352,
-0.0122737742227515));
#18585=CARTESIAN_POINT('Ctrl Pts',(0.00445904606366526,-0.037185412584469,
-0.0122570381653969));
#18586=CARTESIAN_POINT('Ctrl Pts',(0.00445744878958926,-0.03718354204134,
-0.0122188227597701));
#18587=CARTESIAN_POINT('Ctrl Pts',(0.004457,-0.0371825036589017,-0.0121973394742422));
#18588=CARTESIAN_POINT('Ctrl Pts',(0.004457,-0.0371814756795928,-0.0121758532865595));
#18589=CARTESIAN_POINT('Origin',(0.006,-0.0418165664398416,-0.0121758532865581));
#18590=CARTESIAN_POINT('',(0.004457,-0.0381835089768636,-0.0121758532865622));
#18591=CARTESIAN_POINT('',(0.004457,-0.0380657947427934,-0.0121758532821831));
#18592=CARTESIAN_POINT('',(0.004457,-0.0418165664398416,-0.0121758532865581));
#18593=CARTESIAN_POINT('Ctrl Pts',(0.004457,-0.037567972222619,-0.0121758532865581));
#18594=CARTESIAN_POINT('Ctrl Pts',(0.004457,-0.037568678241124,-0.0121898344068753));
#18595=CARTESIAN_POINT('Ctrl Pts',(0.00445719002408502,-0.0375693784287243,
-0.0122038151522925));
#18596=CARTESIAN_POINT('Ctrl Pts',(0.00445808151027365,-0.0375710079749599,
-0.0122366026512338));
#18597=CARTESIAN_POINT('Ctrl Pts',(0.0044589370642531,-0.0375719326749006,
-0.0122554031334834));
#18598=CARTESIAN_POINT('Ctrl Pts',(0.00446679404094303,-0.0375779304842151,
-0.0123784440671839));
#18599=CARTESIAN_POINT('Ctrl Pts',(0.00448402264997262,-0.0375826887137011,
-0.0124817582632797));
#18600=CARTESIAN_POINT('Ctrl Pts',(0.00452632927009839,-0.0375900513271768,
-0.0126365952903472));
#18601=CARTESIAN_POINT('Ctrl Pts',(0.00454403035407989,-0.0375926311243432,
-0.0126897992095187));
#18602=CARTESIAN_POINT('Ctrl Pts',(0.00457617451843771,-0.0375968131917808,
-0.0127713094850159));
#18603=CARTESIAN_POINT('Ctrl Pts',(0.00458866380320455,-0.0375983503945804,
-0.0128003346652087));
#18604=CARTESIAN_POINT('Ctrl Pts',(0.00460691311778797,-0.0376005113407886,
-0.012839397407423));
#18605=CARTESIAN_POINT('Ctrl Pts',(0.00461190866022404,-0.0376010951177554,
-0.0128497852408629));
#18606=CARTESIAN_POINT('Ctrl Pts',(0.00462059548986302,-0.0376020989756306,
-0.012867342408065));
#18607=CARTESIAN_POINT('Ctrl Pts',(0.00462422751550074,-0.0376025155503683,
-0.0128745406826348));
#18608=CARTESIAN_POINT('Ctrl Pts',(0.00463213180611988,-0.037603415976494,
-0.0128899054837215));
#18609=CARTESIAN_POINT('Ctrl Pts',(0.00463642100623976,-0.0376039007819443,
-0.0128980625744427));
#18610=CARTESIAN_POINT('Ctrl Pts',(0.00464872682046266,-0.037605280089016,
-0.0129209650098798));
#18611=CARTESIAN_POINT('Ctrl Pts',(0.00465691111621596,-0.037606184003529,
-0.0129356183108848));
#18612=CARTESIAN_POINT('Ctrl Pts',(0.00470799010563829,-0.0376117329409057,
-0.0130236657262171));
#18613=CARTESIAN_POINT('Ctrl Pts',(0.00475664874101791,-0.0376166304450483,
-0.0130935413668386));
#18614=CARTESIAN_POINT('Ctrl Pts',(0.00485525609258224,-0.0376255100341241,
-0.0132128083728953));
#18615=CARTESIAN_POINT('Ctrl Pts',(0.00490329946283619,-0.0376294899279881,
-0.0132634946130268));
#18616=CARTESIAN_POINT('Ctrl Pts',(0.00498686227427952,-0.0376357837459509,
-0.0133404663845039));
#18617=CARTESIAN_POINT('Ctrl Pts',(0.00502036739842618,-0.037638165803492,
-0.0133687875613264));
#18618=CARTESIAN_POINT('Ctrl Pts',(0.00506975900280824,-0.0376414793398714,
-0.0134070508966981));
#18619=CARTESIAN_POINT('Ctrl Pts',(0.00508468789446661,-0.0376424567849377,
-0.013418189657265));
#18620=CARTESIAN_POINT('Ctrl Pts',(0.00511132004003647,-0.0376441593126957,
-0.0134373197278642));
#18621=CARTESIAN_POINT('Ctrl Pts',(0.00512293833039767,-0.0376448887004029,
-0.0134454250644067));
#18622=CARTESIAN_POINT('Ctrl Pts',(0.00514762669966909,-0.0376464114394628,
-0.0134621478777868));
#18623=CARTESIAN_POINT('Ctrl Pts',(0.00516071966444018,-0.0376472033733367,
-0.0134707287863118));
#18624=CARTESIAN_POINT('Ctrl Pts',(0.00519647241119483,-0.0376493256235521,
-0.0134933903903574));
#18625=CARTESIAN_POINT('Ctrl Pts',(0.00521937086139691,-0.0376506419506198,
-0.0135070853690383));
#18626=CARTESIAN_POINT('Ctrl Pts',(0.00535590594848493,-0.0376582659327228,
-0.0135840084654818));
#18627=CARTESIAN_POINT('Ctrl Pts',(0.00547680491045863,-0.0376640665963067,
-0.0136332567900804));
#18628=CARTESIAN_POINT('Ctrl Pts',(0.00565787736508249,-0.0376727574647282,
-0.0136815397652588));
#18629=CARTESIAN_POINT('Ctrl Pts',(0.00571408179197582,-0.0376754648397836,
-0.013693215920058));
#18630=CARTESIAN_POINT('Ctrl Pts',(0.00578433075752823,-0.0376789966041887,
-0.0137037678715674));
#18631=CARTESIAN_POINT('Ctrl Pts',(0.00579788711941135,-0.0376796849322712,
-0.013705620118642));
#18632=CARTESIAN_POINT('Ctrl Pts',(0.00581987325141321,-0.0376808147744672,
-0.0137083268131556));
#18633=CARTESIAN_POINT('Ctrl Pts',(0.00582828882786665,-0.0376812504303419,
-0.0137092925655745));
#18634=CARTESIAN_POINT('Ctrl Pts',(0.00584517407129322,-0.0376821316745481,
-0.0137110895399734));
#18635=CARTESIAN_POINT('Ctrl Pts',(0.00585364350714671,-0.0376825772795396,
-0.0137119200794625));
#18636=CARTESIAN_POINT('Ctrl Pts',(0.00587594096430578,-0.037683759055172,
-0.0137139205591896));
#18637=CARTESIAN_POINT('Ctrl Pts',(0.00588977838890079,-0.0376845011630794,
-0.0137149740582421));
#18638=CARTESIAN_POINT('Ctrl Pts',(0.00596114800471843,-0.0376883670961703,
-0.01371944036544));
#18639=CARTESIAN_POINT('Ctrl Pts',(0.00601882061328578,-0.0376916178401928,
-0.0137198141964576));
#18640=CARTESIAN_POINT('Ctrl Pts',(0.00616936667675947,-0.03770022391967,
-0.0137123534780442));
#18641=CARTESIAN_POINT('Ctrl Pts',(0.00626175900387458,-0.0377056145604786,
-0.0136993368656634));
#18642=CARTESIAN_POINT('Ctrl Pts',(0.00640207921997938,-0.0377136612537982,
-0.0136664181094068));
#18643=CARTESIAN_POINT('Ctrl Pts',(0.00645113740171161,-0.037716450143879,
-0.0136523108727218));
#18644=CARTESIAN_POINT('Ctrl Pts',(0.00651792114498997,-0.0377202034757736,
-0.0136294658315586));
#18645=CARTESIAN_POINT('Ctrl Pts',(0.00653631033396669,-0.0377212325065626,
-0.013622782108565));
#18646=CARTESIAN_POINT('Ctrl Pts',(0.00656790670424053,-0.0377229934939561,
-0.0136106129485017));
#18647=CARTESIAN_POINT('Ctrl Pts',(0.00658117363117577,-0.0377237307151269,
-0.0136052904278226));
#18648=CARTESIAN_POINT('Ctrl Pts',(0.00660843786701875,-0.0377252417939346,
-0.0135939100251527));
#18649=CARTESIAN_POINT('Ctrl Pts',(0.00662242319405501,-0.037726014720564,
-0.0135878274154827));
#18650=CARTESIAN_POINT('Ctrl Pts',(0.00665879454150574,-0.037728020425607,
-0.0135713630699997));
#18651=CARTESIAN_POINT('Ctrl Pts',(0.0066810260937949,-0.0377292418776456,
-0.0135606497865872));
#18652=CARTESIAN_POINT('Ctrl Pts',(0.00680436302976774,-0.0377360095945636,
-0.0134975253247468));
#18653=CARTESIAN_POINT('Ctrl Pts',(0.00689967779314488,-0.0377411731969113,
-0.0134345821810689));
#18654=CARTESIAN_POINT('Ctrl Pts',(0.00702720726955131,-0.0377487958333585,
-0.0133284172286406));
#18655=CARTESIAN_POINT('Ctrl Pts',(0.00706549906044883,-0.0377512020427642,
-0.0132931131728694));
#18656=CARTESIAN_POINT('Ctrl Pts',(0.0071230947291257,-0.0377551384070272,
-0.0132343528247423));
#18657=CARTESIAN_POINT('Ctrl Pts',(0.00714361742761331,-0.0377566124091082,
-0.0132121457233357));
#18658=CARTESIAN_POINT('Ctrl Pts',(0.00717093292913957,-0.0377586983546337,
-0.0131807881359926));
#18659=CARTESIAN_POINT('Ctrl Pts',(0.00717829748583572,-0.0377592739099808,
-0.0131721429013325));
#18660=CARTESIAN_POINT('Ctrl Pts',(0.00719071304813249,-0.0377602685109808,
-0.0131572380816037));
#18661=CARTESIAN_POINT('Ctrl Pts',(0.00719581184136165,-0.0377606842327645,
-0.0131510187687202));
#18662=CARTESIAN_POINT('Ctrl Pts',(0.00720670626839883,-0.0377615887549717,
-0.0131375162254816));
#18663=CARTESIAN_POINT('Ctrl Pts',(0.00721248487748851,-0.0377620786132465,
-0.0131302201130723));
#18664=CARTESIAN_POINT('Ctrl Pts',(0.00722876540335598,-0.0377634866814276,
-0.0131092776757534));
#18665=CARTESIAN_POINT('Ctrl Pts',(0.00723910510481083,-0.0377644148962775,
-0.0130955075687727));
#18666=CARTESIAN_POINT('Ctrl Pts',(0.00728944283900557,-0.0377690947268764,
-0.0130260789757216));
#18667=CARTESIAN_POINT('Ctrl Pts',(0.00732592942432527,-0.0377730072835353,
-0.0129679747726239));
#18668=CARTESIAN_POINT('Ctrl Pts',(0.00738778435969847,-0.0377804887130888,
-0.0128531526162443));
#18669=CARTESIAN_POINT('Ctrl Pts',(0.00741383416331627,-0.0377840476500943,
-0.0127969437031496));
#18670=CARTESIAN_POINT('Ctrl Pts',(0.0074517506613499,-0.0377899019115409,
-0.0127002838079475));
#18671=CARTESIAN_POINT('Ctrl Pts',(0.00746546659798519,-0.0377922329370755,
-0.012660637141102));
#18672=CARTESIAN_POINT('Ctrl Pts',(0.00748662659889514,-0.0377962329342473,
-0.0125903195624184));
#18673=CARTESIAN_POINT('Ctrl Pts',(0.0074947769795301,-0.0377979214700999,
-0.0125598883254413));
#18674=CARTESIAN_POINT('Ctrl Pts',(0.00750578805759868,-0.037800454140006,
-0.012513086548362));
#18675=CARTESIAN_POINT('Ctrl Pts',(0.00750932518532635,-0.0378013193517727,
-0.0124968851553233));
#18676=CARTESIAN_POINT('Ctrl Pts',(0.00751537314918192,-0.0378029017227214,
-0.0124668691815798));
#18677=CARTESIAN_POINT('Ctrl Pts',(0.00751795788826667,-0.0378036211484498,
-0.0124530714297225));
#18678=CARTESIAN_POINT('Ctrl Pts',(0.00752328746026531,-0.037805208272874,
-0.0124223074036548));
#18679=CARTESIAN_POINT('Ctrl Pts',(0.00752593786390774,-0.037806072928249,
-0.0124053265614354));
#18680=CARTESIAN_POINT('Ctrl Pts',(0.00753309967034735,-0.0378086643837219,
-0.0123538068922219));
#18681=CARTESIAN_POINT('Ctrl Pts',(0.00753672599787411,-0.0378103639239807,
-0.0123191554455367));
#18682=CARTESIAN_POINT('Ctrl Pts',(0.00754754436034415,-0.0378177399914758,
-0.012165765757112));
#18683=CARTESIAN_POINT('Ctrl Pts',(0.00754216658919725,-0.0378230494984337,
-0.012046558670885));
#18684=CARTESIAN_POINT('Ctrl Pts',(0.00751432616600706,-0.037831137355823,
-0.0118746698541655));
#18685=CARTESIAN_POINT('Ctrl Pts',(0.00750258559480269,-0.0378337480307295,
-0.01182070438724));
#18686=CARTESIAN_POINT('Ctrl Pts',(0.00748439078673871,-0.0378371672791377,
-0.0117544069527176));
#18687=CARTESIAN_POINT('Ctrl Pts',(0.00748062837626584,-0.0378378499389566,
-0.0117413735887382));
#18688=CARTESIAN_POINT('Ctrl Pts',(0.00747424637304036,-0.0378389726259518,
-0.0117203119464514));
#18689=CARTESIAN_POINT('Ctrl Pts',(0.00747173177866306,-0.0378394069231991,
-0.0117122523297544));
#18690=CARTESIAN_POINT('Ctrl Pts',(0.00746654316091263,-0.0378402880226924,
-0.0116960898452881));
#18691=CARTESIAN_POINT('Ctrl Pts',(0.00746386782332745,-0.0378407348793186,
-0.0116879877400799));
#18692=CARTESIAN_POINT('Ctrl Pts',(0.00745663037210988,-0.0378419237712366,
-0.0116666651588377));
#18693=CARTESIAN_POINT('Ctrl Pts',(0.00745195556074729,-0.0378426718672093,
-0.0116534840557328));
#18694=CARTESIAN_POINT('Ctrl Pts',(0.00742613923800333,-0.0378466948643999,
-0.0115837175882531));
#18695=CARTESIAN_POINT('Ctrl Pts',(0.00740186903369166,-0.0378501091495675,
-0.0115283504884533));
#18696=CARTESIAN_POINT('Ctrl Pts',(0.00733311134558308,-0.0378587566253638,
-0.0113935980992907));
#18697=CARTESIAN_POINT('Ctrl Pts',(0.00728472869940064,-0.0378640122185914,
-0.0113164446414694));
#18698=CARTESIAN_POINT('Ctrl Pts',(0.00719937268103303,-0.0378718984062556,
-0.0112037944775888));
#18699=CARTESIAN_POINT('Ctrl Pts',(0.00716695606857058,-0.0378746546885683,
-0.0111651073072806));
#18700=CARTESIAN_POINT('Ctrl Pts',(0.00711946181833625,-0.0378783732253046,
-0.011113763700785));
#18701=CARTESIAN_POINT('Ctrl Pts',(0.00710595335127584,-0.0378793984694344,
-0.0110997044668799));
#18702=CARTESIAN_POINT('Ctrl Pts',(0.00708209203673046,-0.0378811551263349,
-0.0110757942689379));
#18703=CARTESIAN_POINT('Ctrl Pts',(0.00707186231035027,-0.037881891732357,
-0.0110658243572278));
#18704=CARTESIAN_POINT('Ctrl Pts',(0.00705040906936235,-0.0378834034353072,
-0.0110454891313197));
#18705=CARTESIAN_POINT('Ctrl Pts',(0.00703916707260944,-0.037884177568683,
-0.0110351455443623));
#18706=CARTESIAN_POINT('Ctrl Pts',(0.00700927458838185,-0.0378861906770952,
-0.0110084506570932));
#18707=CARTESIAN_POINT('Ctrl Pts',(0.00699037993875028,-0.037887418163699,
-0.0109923788442991));
#18708=CARTESIAN_POINT('Ctrl Pts',(0.00688347468550523,-0.0378941360026634,
-0.0109057992266374));
#18709=CARTESIAN_POINT('Ctrl Pts',(0.00678833009440698,-0.0378992528980613,
-0.0108446499911663));
#18710=CARTESIAN_POINT('Ctrl Pts',(0.00664026164079196,-0.0379068487433321,
-0.0107709753005912));
#18711=CARTESIAN_POINT('Ctrl Pts',(0.00659199170693112,-0.0379092795551161,
-0.0107499632422185));
#18712=CARTESIAN_POINT('Ctrl Pts',(0.00652311060910942,-0.0379127987398857,
-0.0107240804873457));
#18713=CARTESIAN_POINT('Ctrl Pts',(0.00650332788175168,-0.037913815203053,
-0.0107171038395648));
#18714=CARTESIAN_POINT('Ctrl Pts',(0.00646806335569633,-0.0379156470032412,
-0.01070547005692));
#18715=CARTESIAN_POINT('Ctrl Pts',(0.00645263883063274,-0.0379164548427084,
-0.0107006488269146));
#18716=CARTESIAN_POINT('Ctrl Pts',(0.00642852017037536,-0.0379177322749562,
-0.0106935239416549));
#18717=CARTESIAN_POINT('Ctrl Pts',(0.00641987644180926,-0.037918192906761,
-0.0106910524281609));
#18718=CARTESIAN_POINT('Ctrl Pts',(0.00640344627989107,-0.0379190746638328,
-0.0106865094668853));
#18719=CARTESIAN_POINT('Ctrl Pts',(0.0063956644367984,-0.0379194949737761,
-0.0106844232490246));
#18720=CARTESIAN_POINT('Ctrl Pts',(0.00637814733779928,-0.0379204466583869,
-0.0106798738642972));
#18721=CARTESIAN_POINT('Ctrl Pts',(0.00636840365671405,-0.0379209798323623,
-0.0106774446052178));
#18722=CARTESIAN_POINT('Ctrl Pts',(0.00633315130660186,-0.0379229208119484,
-0.0106690202394396));
#18723=CARTESIAN_POINT('Ctrl Pts',(0.0063075157062571,-0.0379243547835765,
-0.0106635803057966));
#18724=CARTESIAN_POINT('Ctrl Pts',(0.00616290266057789,-0.0379325234067393,
-0.0106367220447446));
#18725=CARTESIAN_POINT('Ctrl Pts',(0.00604186737402234,-0.0379396201874804,
-0.0106286908510281));
#18726=CARTESIAN_POINT('Ctrl Pts',(0.00586260049968923,-0.0379497116860012,
-0.010637865913351));
#18727=CARTESIAN_POINT('Ctrl Pts',(0.00580428414016355,-0.037952935505009,
-0.0106441939824192));
#18728=CARTESIAN_POINT('Ctrl Pts',(0.00572634702991176,-0.0379571461978135,
-0.0106571765669704));
#18729=CARTESIAN_POINT('Ctrl Pts',(0.00570629776553585,-0.0379582208390945,
-0.010660926233141));
#18730=CARTESIAN_POINT('Ctrl Pts',(0.00567219953469682,-0.0379600345408175,
-0.0106680057892819));
#18731=CARTESIAN_POINT('Ctrl Pts',(0.00565811255163312,-0.0379607797348449,
-0.0106711372962689));
#18732=CARTESIAN_POINT('Ctrl Pts',(0.00563122001510145,-0.0379621950272905,
-0.0106775126181763));
#18733=CARTESIAN_POINT('Ctrl Pts',(0.00561840818961115,-0.0379628660787223,
-0.0106807241483264));
#18734=CARTESIAN_POINT('Ctrl Pts',(0.00558462877119288,-0.0379646276962723,
-0.0106896541013495));
#18735=CARTESIAN_POINT('Ctrl Pts',(0.00556373772068329,-0.0379657092751702,
-0.0106956517604971));
#18736=CARTESIAN_POINT('Ctrl Pts',(0.00547676146541318,-0.0379701870165771,
-0.0107226234519438));
#18737=CARTESIAN_POINT('Ctrl Pts',(0.00541199893961501,-0.0379734549048751,
-0.0107475985945882));
#18738=CARTESIAN_POINT('Ctrl Pts',(0.00527735885934287,-0.0379803258465395,
-0.0108102379914169));
#18739=CARTESIAN_POINT('Ctrl Pts',(0.00520826405311605,-0.0379838999420277,
-0.0108491019970386));
#18740=CARTESIAN_POINT('Ctrl Pts',(0.00510125736816331,-0.037989907623262,
-0.0109206374574219));
#18741=CARTESIAN_POINT('Ctrl Pts',(0.00506141083126633,-0.0379922662657697,
-0.0109501474828508));
#18742=CARTESIAN_POINT('Ctrl Pts',(0.00501282020636505,-0.0379953922100594,
-0.0109898937837802));
#18743=CARTESIAN_POINT('Ctrl Pts',(0.00500269240355866,-0.037996058371806,
-0.0109983977998296));
#18744=CARTESIAN_POINT('Ctrl Pts',(0.00498633318825823,-0.0379971608383284,
-0.0110124966360593));
#18745=CARTESIAN_POINT('Ctrl Pts',(0.00498003558507807,-0.0379975918025418,
-0.0110180140534124));
#18746=CARTESIAN_POINT('Ctrl Pts',(0.00496735012263712,-0.0379984740334646,
-0.0110293117730038));
#18747=CARTESIAN_POINT('Ctrl Pts',(0.00496096520631356,-0.0379989254755268,
-0.0110350948099002));
#18748=CARTESIAN_POINT('Ctrl Pts',(0.00494405723907815,-0.0380001399927284,
-0.0110506686455708));
#18749=CARTESIAN_POINT('Ctrl Pts',(0.00493362221799278,-0.0380009095750944,
-0.0110605533323193));
#18750=CARTESIAN_POINT('Ctrl Pts',(0.00486754540254391,-0.0380059039048724,
-0.0111249204354672));
#18751=CARTESIAN_POINT('Ctrl Pts',(0.00481596133795193,-0.0380103590664143,
-0.0111833998149025));
#18752=CARTESIAN_POINT('Ctrl Pts',(0.00472471966667389,-0.0380190431794876,
-0.0113041272069601));
#18753=CARTESIAN_POINT('Ctrl Pts',(0.00468466372013476,-0.038023259303859,
-0.0113658298368658));
#18754=CARTESIAN_POINT('Ctrl Pts',(0.00462507340229277,-0.038030135143714,
-0.0114737786134851));
#18755=CARTESIAN_POINT('Ctrl Pts',(0.00460311759566668,-0.0380328566815838,
-0.0115185464607139));
#18756=CARTESIAN_POINT('Ctrl Pts',(0.00457566874831347,-0.0380365379927172,
-0.011582130636113));
#18757=CARTESIAN_POINT('Ctrl Pts',(0.00456830924681202,-0.038037559075236,
-0.011600103572483));
#18758=CARTESIAN_POINT('Ctrl Pts',(0.0045561331106894,-0.0380393109226003,
-0.0116315178444111));
#18759=CARTESIAN_POINT('Ctrl Pts',(0.00455116022499072,-0.0380400468037795,
-0.0116448956686408));
#18760=CARTESIAN_POINT('Ctrl Pts',(0.00454124135223827,-0.0380415590612276,
-0.0116727565185476));
#18761=CARTESIAN_POINT('Ctrl Pts',(0.00453632378006639,-0.0380423344387303,
-0.0116872480316083));
#18762=CARTESIAN_POINT('Ctrl Pts',(0.00452396119820181,-0.0380443554230636,
-0.0117255419228124));
#18763=CARTESIAN_POINT('Ctrl Pts',(0.0045168761133895,-0.0380455893642825,
-0.0117494561811065));
#18764=CARTESIAN_POINT('Ctrl Pts',(0.00448127997067977,-0.0380522541178259,
-0.0118812538988614));
#18765=CARTESIAN_POINT('Ctrl Pts',(0.00446395646686249,-0.0380573210498084,
-0.0119918116526313));
#18766=CARTESIAN_POINT('Ctrl Pts',(0.00445756920838888,-0.0380635562817696,
-0.0121274568329522));
#18767=CARTESIAN_POINT('Ctrl Pts',(0.00445700000013722,-0.0380646707421583,
-0.0121516556448979));
#18768=CARTESIAN_POINT('Ctrl Pts',(0.004457,-0.0380657947427934,-0.0121758532778082));
#18769=CARTESIAN_POINT('',(0.00445700007887821,-0.0381834855813947,-0.0121753599123031));
#18770=CARTESIAN_POINT('Ctrl Pts',(0.00445700007571663,-0.0381834860550969,
-0.0121753699010766));
#18771=CARTESIAN_POINT('Ctrl Pts',(0.00445700807984317,-0.0381822989275644,
-0.0121503374505815));
#18772=CARTESIAN_POINT('Ctrl Pts',(0.00445762492030033,-0.0381810959311471,
-0.012125309835296));
#18773=CARTESIAN_POINT('Ctrl Pts',(0.00445962253413835,-0.0381790958161663,
-0.0120845571132157));
#18774=CARTESIAN_POINT('Ctrl Pts',(0.00446063611188745,-0.0381783132920324,
-0.0120688181718112));
#18775=CARTESIAN_POINT('Ctrl Pts',(0.00446257170777129,-0.0381770882764331,
-0.0120445653706469));
#18776=CARTESIAN_POINT('Ctrl Pts',(0.00446332367190949,-0.0381766539205719,
-0.0120360386694657));
#18777=CARTESIAN_POINT('Ctrl Pts',(0.00446489085249986,-0.0381758196083426,
-0.0120198120955244));
#18778=CARTESIAN_POINT('Ctrl Pts',(0.00446569316761004,-0.0381754203257101,
-0.0120121111393718));
#18779=CARTESIAN_POINT('Ctrl Pts',(0.00446756295966174,-0.0381745453786827,
-0.0119953864492878));
#18780=CARTESIAN_POINT('Ctrl Pts',(0.00446865223033783,-0.0381740685839721,
-0.0119863656554562));
#18781=CARTESIAN_POINT('Ctrl Pts',(0.00447186392729497,-0.0381727475633907,
-0.0119616073729424));
#18782=CARTESIAN_POINT('Ctrl Pts',(0.00447414968119314,-0.0381718952545135,
-0.0119458925604982));
#18783=CARTESIAN_POINT('Ctrl Pts',(0.00449016356999372,-0.0381664331563208,
-0.0118465820682879));
#18784=CARTESIAN_POINT('Ctrl Pts',(0.00451051349907191,-0.0381615687160591,
-0.0117642056823892));
#18785=CARTESIAN_POINT('Ctrl Pts',(0.0045559364556698,-0.0381534125390411,
-0.0116291661022431));
#18786=CARTESIAN_POINT('Ctrl Pts',(0.00457741581831107,-0.0381501169455277,
-0.0115754857057749));
#18787=CARTESIAN_POINT('Ctrl Pts',(0.00462431818260893,-0.0381439220813868,
-0.0114750194002862));
#18788=CARTESIAN_POINT('Ctrl Pts',(0.00464925060196407,-0.0381410161507218,
-0.0114280929604154));
#18789=CARTESIAN_POINT('Ctrl Pts',(0.0046869077234412,-0.0381371196432484,
-0.0113652713226151));
#18790=CARTESIAN_POINT('Ctrl Pts',(0.00469759758237722,-0.0381360601704495,
-0.011348204544784));
#18791=CARTESIAN_POINT('Ctrl Pts',(0.00471667604155027,-0.038134246788412,
-0.0113190304687672));
#18792=CARTESIAN_POINT('Ctrl Pts',(0.00472490939227096,-0.0381334874138191,
-0.011306825274943));
#18793=CARTESIAN_POINT('Ctrl Pts',(0.00474230745449342,-0.0381319290747664,
-0.0112818139298716));
#18794=CARTESIAN_POINT('Ctrl Pts',(0.00475149607945117,-0.0381311311216071,
-0.0112690264597757));
#18795=CARTESIAN_POINT('Ctrl Pts',(0.00477616232250487,-0.038129052077859,
-0.0112357851344111));
#18796=CARTESIAN_POINT('Ctrl Pts',(0.00479195722761334,-0.0381277831069042,
-0.0112155723157098));
#18797=CARTESIAN_POINT('Ctrl Pts',(0.00487507652800483,-0.0381213955429583,
-0.0111145026714802));
#18798=CARTESIAN_POINT('Ctrl Pts',(0.00495003877684577,-0.0381165867220101,
-0.0110402912785554));
#18799=CARTESIAN_POINT('Ctrl Pts',(0.00507519223321637,-0.0381091917841313,
-0.0109394634943782));
#18800=CARTESIAN_POINT('Ctrl Pts',(0.00512025569620734,-0.0381066292231524,
-0.0109070039961268));
#18801=CARTESIAN_POINT('Ctrl Pts',(0.00519348889081106,-0.0381024700344351,
-0.0108600335463647));
#18802=CARTESIAN_POINT('Ctrl Pts',(0.00522052391392337,-0.0381009353425285,
-0.010843840312821));
#18803=CARTESIAN_POINT('Ctrl Pts',(0.0052582563208355,-0.0380987688325838,
-0.0108227818329828));
#18804=CARTESIAN_POINT('Ctrl Pts',(0.00526854295633942,-0.0380981757596999,
-0.0108171934241297));
#18805=CARTESIAN_POINT('Ctrl Pts',(0.00528621188648847,-0.0380971512637479,
-0.0108078532556764));
#18806=CARTESIAN_POINT('Ctrl Pts',(0.00529356246781917,-0.0380967233298339,
-0.0108040429618428));
#18807=CARTESIAN_POINT('Ctrl Pts',(0.00530953191190565,-0.038095789429608,
-0.0107959273373983));
#18808=CARTESIAN_POINT('Ctrl Pts',(0.00531816057534008,-0.0380952823298245,
-0.0107916434775061));
#18809=CARTESIAN_POINT('Ctrl Pts',(0.00534354809358269,-0.0380937843119392,
-0.0107793343458034));
#18810=CARTESIAN_POINT('Ctrl Pts',(0.00536041201016674,-0.0380927816436721,
-0.0107715308865477));
#18811=CARTESIAN_POINT('Ctrl Pts',(0.00549805625916409,-0.0380845608367445,
-0.0107108321336211));
#18812=CARTESIAN_POINT('Ctrl Pts',(0.00562502124387916,-0.0380768048646116,
-0.0106733128717973));
#18813=CARTESIAN_POINT('Ctrl Pts',(0.00581244822232353,-0.038066152985259,
-0.0106431975338362));
#18814=CARTESIAN_POINT('Ctrl Pts',(0.00587015912738619,-0.0380629684097801,
-0.0106372332057918));
#18815=CARTESIAN_POINT('Ctrl Pts',(0.00594871316956669,-0.0380587791022423,
-0.0106335674585809));
#18816=CARTESIAN_POINT('Ctrl Pts',(0.00596937048082932,-0.0380576907119355,
-0.0106330189464952));
#18817=CARTESIAN_POINT('Ctrl Pts',(0.00600483799414925,-0.038055844035549,
-0.0106327898455211));
#18818=CARTESIAN_POINT('Ctrl Pts',(0.00601964365291815,-0.038055079730333,
-0.0106329072939921));
#18819=CARTESIAN_POINT('Ctrl Pts',(0.00605000969443451,-0.0380535249906304,
-0.0106335853494047));
#18820=CARTESIAN_POINT('Ctrl Pts',(0.00606556790175287,-0.0380527353294816,
-0.0106341684185913));
#18821=CARTESIAN_POINT('Ctrl Pts',(0.00610583294606137,-0.0380507081970563,
-0.0106362880693841));
#18822=CARTESIAN_POINT('Ctrl Pts',(0.00613051676522877,-0.0380494816953564,
-0.0106381839049589));
#18823=CARTESIAN_POINT('Ctrl Pts',(0.00626824397463171,-0.0380427120303106,
-0.0106521026018443));
#18824=CARTESIAN_POINT('Ctrl Pts',(0.00637973157732812,-0.038037543715466,
-0.0106759944487953));
#18825=CARTESIAN_POINT('Ctrl Pts',(0.00653586664681331,-0.0380299597710212,
-0.0107279978777897));
#18826=CARTESIAN_POINT('Ctrl Pts',(0.00658331775017463,-0.0380275997335011,
-0.0107464554153444));
#18827=CARTESIAN_POINT('Ctrl Pts',(0.00664864808128062,-0.0380241697618877,
-0.010775663163989));
#18828=CARTESIAN_POINT('Ctrl Pts',(0.0066673560474783,-0.038023165755405,
-0.0107844825387745));
#18829=CARTESIAN_POINT('Ctrl Pts',(0.00670026979723398,-0.0380213509544965,
-0.0108008153773835));
#18830=CARTESIAN_POINT('Ctrl Pts',(0.00671454628657624,-0.0380205471693319,
-0.0108081798577217));
#18831=CARTESIAN_POINT('Ctrl Pts',(0.00673674766594897,-0.0380192670276144,
-0.0108200748621562));
#18832=CARTESIAN_POINT('Ctrl Pts',(0.00674475208108348,-0.0380187992270411,
-0.0108244552737066));
#18833=CARTESIAN_POINT('Ctrl Pts',(0.00676002458251343,-0.0380178937080423,
-0.0108329900352291));
#18834=CARTESIAN_POINT('Ctrl Pts',(0.00676729850016675,-0.0380174566531655,
-0.0108371329728309));
#18835=CARTESIAN_POINT('Ctrl Pts',(0.00678560906360607,-0.0380163424112395,
-0.0108477601980334));
#18836=CARTESIAN_POINT('Ctrl Pts',(0.00679659929907176,-0.0380156606040953,
-0.0108543229657534));
#18837=CARTESIAN_POINT('Ctrl Pts',(0.00684014445618043,-0.0380129107379959,
-0.0108810663006635));
#18838=CARTESIAN_POINT('Ctrl Pts',(0.00687202293689719,-0.038010788414809,
-0.0109023181837307));
#18839=CARTESIAN_POINT('Ctrl Pts',(0.00698681436741511,-0.0380028234465747,
-0.0109851761497589));
#18840=CARTESIAN_POINT('Ctrl Pts',(0.00706427446941344,-0.0379968177445107,
-0.0110538746208163));
#18841=CARTESIAN_POINT('Ctrl Pts',(0.0071740077331866,-0.0379877305783903,
-0.0111728644334368));
#18842=CARTESIAN_POINT('Ctrl Pts',(0.0072112402895965,-0.0379845108065972,
-0.0112181587267912));
#18843=CARTESIAN_POINT('Ctrl Pts',(0.00725803680560202,-0.0379802848797113,
-0.0112821968320577));
#18844=CARTESIAN_POINT('Ctrl Pts',(0.00726992594912318,-0.0379791931046738,
-0.0112991739829865));
#18845=CARTESIAN_POINT('Ctrl Pts',(0.00728972215826971,-0.0379773425095217,
-0.011328690228237));
#18846=CARTESIAN_POINT('Ctrl Pts',(0.00729779697143078,-0.0379765776049487,
-0.0113411128875556));
#18847=CARTESIAN_POINT('Ctrl Pts',(0.00731397731524256,-0.0379750231675733,
-0.0113668079291437));
#18848=CARTESIAN_POINT('Ctrl Pts',(0.00732206364079725,-0.0379742343817509,
-0.0113800904278613));
#18849=CARTESIAN_POINT('Ctrl Pts',(0.00734244984074504,-0.0379722127824101,
-0.0114147452965651));
#18850=CARTESIAN_POINT('Ctrl Pts',(0.00735444086040068,-0.0379709908180102,
-0.0114362946446358));
#18851=CARTESIAN_POINT('Ctrl Pts',(0.00741913772724974,-0.0379641875599236,
-0.0115594190686797));
#18852=CARTESIAN_POINT('Ctrl Pts',(0.00746093124990526,-0.0379589873458232,
-0.0116663196475656));
#18853=CARTESIAN_POINT('Ctrl Pts',(0.00750812729823622,-0.0379505746811456,
-0.01184263198142));
#18854=CARTESIAN_POINT('Ctrl Pts',(0.00752135881475362,-0.0379474105157327,
-0.0119094883294143));
#18855=CARTESIAN_POINT('Ctrl Pts',(0.00753242208193721,-0.0379431907103036,
-0.0119946149908679));
#18856=CARTESIAN_POINT('Ctrl Pts',(0.00753440754080903,-0.0379423049753607,
-0.0120122739264848));
#18857=CARTESIAN_POINT('Ctrl Pts',(0.00753698319781072,-0.037940923684118,
-0.0120393930815286));
#18858=CARTESIAN_POINT('Ctrl Pts',(0.00753779198449694,-0.0379404390503911,
-0.0120488314712813));
#18859=CARTESIAN_POINT('Ctrl Pts',(0.00753914811192466,-0.0379395196003125,
-0.0120665766436435));
#18860=CARTESIAN_POINT('Ctrl Pts',(0.00753971521668366,-0.0379390858087027,
-0.0120748813337784));
#18861=CARTESIAN_POINT('Ctrl Pts',(0.00754082247524485,-0.037938117140808,
-0.0120932857777353));
#18862=CARTESIAN_POINT('Ctrl Pts',(0.00754133056990211,-0.0379375806535036,
-0.0121033870347872));
#18863=CARTESIAN_POINT('Ctrl Pts',(0.00754276521091481,-0.0379356816540669,
-0.0121388554005697));
#18864=CARTESIAN_POINT('Ctrl Pts',(0.00754316502977748,-0.0379342953127187,
-0.0121642387069013));
#18865=CARTESIAN_POINT('Ctrl Pts',(0.00754184859055401,-0.0379261207809339,
-0.0123117932454939));
#18866=CARTESIAN_POINT('Ctrl Pts',(0.00752625215587118,-0.0379189639945425,
-0.01243340616555));
#18867=CARTESIAN_POINT('Ctrl Pts',(0.00748264940151215,-0.0379089356998104,
-0.0126069178101067));
#18868=CARTESIAN_POINT('Ctrl Pts',(0.0074658030157952,-0.0379058228519004,
-0.0126611247624748));
#18869=CARTESIAN_POINT('Ctrl Pts',(0.00743884320527958,-0.0379017084221201,
-0.0127335277771436));
#18870=CARTESIAN_POINT('Ctrl Pts',(0.00743129457268651,-0.0379006271128298,
-0.0127526257774028));
#18871=CARTESIAN_POINT('Ctrl Pts',(0.00741765903974918,-0.037898788619515,
-0.0127852057392401));
#18872=CARTESIAN_POINT('Ctrl Pts',(0.00741175549746775,-0.0378980255527028,
-0.0127987609841155));
#18873=CARTESIAN_POINT('Ctrl Pts',(0.0073992205315759,-0.0378964700999605,
-0.0128264488057111));
#18874=CARTESIAN_POINT('Ctrl Pts',(0.00739256762208163,-0.0378956785434963,
-0.0128405698170947));
#18875=CARTESIAN_POINT('Ctrl Pts',(0.00737472283245302,-0.0378936394780892,
-0.012877001662737));
#18876=CARTESIAN_POINT('Ctrl Pts',(0.00736320168852828,-0.0378924031998277,
-0.0128991465552474));
#18877=CARTESIAN_POINT('Ctrl Pts',(0.00728918753461557,-0.037884911346354,
-0.0130333532422099));
#18878=CARTESIAN_POINT('Ctrl Pts',(0.00721346018153639,-0.0378791503089205,
-0.0131375318015117));
#18879=CARTESIAN_POINT('Ctrl Pts',(0.00709762948768706,-0.0378712948858956,
-0.0132610925740447));
#18880=CARTESIAN_POINT('Ctrl Pts',(0.00706836561876731,-0.0378693693736668,
-0.013289913160092));
#18881=CARTESIAN_POINT('Ctrl Pts',(0.00702451332050914,-0.0378665094785237,
-0.0133297827250322));
#18882=CARTESIAN_POINT('Ctrl Pts',(0.00701082237679593,-0.0378656199006003,
-0.0133417944391915));
#18883=CARTESIAN_POINT('Ctrl Pts',(0.00698577913624491,-0.037863992055212,
-0.0133629933991921));
#18884=CARTESIAN_POINT('Ctrl Pts',(0.00697450281609892,-0.0378632588495482,
-0.0133722672556405));
#18885=CARTESIAN_POINT('Ctrl Pts',(0.00695620831328639,-0.0378620659213311,
-0.0133868827670183));
#18886=CARTESIAN_POINT('Ctrl Pts',(0.00694927275554217,-0.0378616129127327,
-0.0133923268659148));
#18887=CARTESIAN_POINT('Ctrl Pts',(0.00693541194317428,-0.0378607052369154,
-0.0134030162602077));
#18888=CARTESIAN_POINT('Ctrl Pts',(0.00692848831584314,-0.0378602506931865,
-0.0134082630829192));
#18889=CARTESIAN_POINT('Ctrl Pts',(0.00691030559669374,-0.0378590548142371,
-0.0134218020190708));
#18890=CARTESIAN_POINT('Ctrl Pts',(0.00689897761272639,-0.0378583076407613,
-0.013429999908378));
#18891=CARTESIAN_POINT('Ctrl Pts',(0.0068420288953634,-0.0378545472819169,
-0.0134700448371934));
#18892=CARTESIAN_POINT('Ctrl Pts',(0.00679482326411402,-0.0378514185731017,
-0.0134995600040748));
#18893=CARTESIAN_POINT('Ctrl Pts',(0.00666467282035146,-0.037842953753567,
-0.01357146054196));
#18894=CARTESIAN_POINT('Ctrl Pts',(0.00657930379798323,-0.0378375769561464,
-0.0136090031920098));
#18895=CARTESIAN_POINT('Ctrl Pts',(0.00644267103213172,-0.0378295399490264,
-0.0136548725091541));
#18896=CARTESIAN_POINT('Ctrl Pts',(0.00639349207595639,-0.0378267506887686,
-0.0136687096907971));
#18897=CARTESIAN_POINT('Ctrl Pts',(0.00632431982629685,-0.0378229783734204,
-0.0136845154129562));
#18898=CARTESIAN_POINT('Ctrl Pts',(0.00630484148510345,-0.0378219321949302,
-0.0136885715282358));
#18899=CARTESIAN_POINT('Ctrl Pts',(0.00627085742960144,-0.0378201340227966,
-0.0136949651687964));
#18900=CARTESIAN_POINT('Ctrl Pts',(0.00625638699410977,-0.0378193768152442,
-0.0136974742598952));
#18901=CARTESIAN_POINT('Ctrl Pts',(0.00622624169192059,-0.0378178162303741,
-0.0137022590315536));
#18902=CARTESIAN_POINT('Ctrl Pts',(0.00621056313719906,-0.0378170139817988,
-0.0137045007247273));
#18903=CARTESIAN_POINT('Ctrl Pts',(0.00616895240852485,-0.0378149081547002,
-0.0137097977991449));
#18904=CARTESIAN_POINT('Ctrl Pts',(0.00614297201513083,-0.0378136173055151,
-0.0137124370893317));
#18905=CARTESIAN_POINT('Ctrl Pts',(0.00603102321530504,-0.0378081421068277,
-0.0137209455930713));
#18906=CARTESIAN_POINT('Ctrl Pts',(0.0059447099690384,-0.0378041511837471,
-0.0137202681247507));
#18907=CARTESIAN_POINT('Ctrl Pts',(0.00579060372199138,-0.037797032614861,
-0.0137061167025053));
#18908=CARTESIAN_POINT('Ctrl Pts',(0.0057228030738379,-0.0377938993302986,
-0.0136952985722337));
#18909=CARTESIAN_POINT('Ctrl Pts',(0.00562136959709282,-0.0377889543294175,
-0.0136720973882863));
#18910=CARTESIAN_POINT('Ctrl Pts',(0.00558707394227576,-0.0377872356323674,
-0.0136629979180245));
#18911=CARTESIAN_POINT('Ctrl Pts',(0.00554146382910192,-0.0377848510823236,
-0.0136491971031509));
#18912=CARTESIAN_POINT('Ctrl Pts',(0.00552984562799984,-0.0377842348900536,
-0.0136455308944181));
#18913=CARTESIAN_POINT('Ctrl Pts',(0.00551034065796981,-0.0377831837102982,
-0.0136391210117759));
#18914=CARTESIAN_POINT('Ctrl Pts',(0.00550243034242742,-0.0377827527039749,
-0.0136364501308802));
#18915=CARTESIAN_POINT('Ctrl Pts',(0.00548566071650898,-0.0377818283889091,
-0.0136306359028756));
#18916=CARTESIAN_POINT('Ctrl Pts',(0.00547680795746787,-0.0377813342124315,
-0.0136274756331677));
#18917=CARTESIAN_POINT('Ctrl Pts',(0.00545164789698164,-0.0377799130550043,
-0.013618233914956));
#18918=CARTESIAN_POINT('Ctrl Pts',(0.00543541427619001,-0.0377789759911882,
-0.0136119573282488));
#18919=CARTESIAN_POINT('Ctrl Pts',(0.00535849093638101,-0.0377744508016309,
-0.0135807097756336));
#18920=CARTESIAN_POINT('Ctrl Pts',(0.00529933233094438,-0.0377707186420423,
-0.0135521596877642));
#18921=CARTESIAN_POINT('Ctrl Pts',(0.00518747121469487,-0.0377633730753424,
-0.013489089675816));
#18922=CARTESIAN_POINT('Ctrl Pts',(0.00513469924815449,-0.0377597683981727,
-0.0134549341945922));
#18923=CARTESIAN_POINT('Ctrl Pts',(0.00503405821432215,-0.0377527278115195,
-0.0133807101955868));
#18924=CARTESIAN_POINT('Ctrl Pts',(0.00498623977971189,-0.037749297188404,
-0.0133407632566839));
#18925=CARTESIAN_POINT('Ctrl Pts',(0.00492563777726345,-0.0377448535662062,
-0.0132835711065105));
#18926=CARTESIAN_POINT('Ctrl Pts',(0.00491061137684016,-0.037743742731776,
-0.0132687967615019));
#18927=CARTESIAN_POINT('Ctrl Pts',(0.0048855013686708,-0.0377418700184975,
-0.0132430754017576));
#18928=CARTESIAN_POINT('Ctrl Pts',(0.00487526517504037,-0.0377411016846315,
-0.0132322820991348));
#18929=CARTESIAN_POINT('Ctrl Pts',(0.00485471834755247,-0.0377395486010616,
-0.0132099797883413));
#18930=CARTESIAN_POINT('Ctrl Pts',(0.00484442130313724,-0.0377387644546698,
-0.0131984605339193));
#18931=CARTESIAN_POINT('Ctrl Pts',(0.00481847798327455,-0.0377367723073857,
-0.0131685454950425));
#18932=CARTESIAN_POINT('Ctrl Pts',(0.00480308715622287,-0.0377355745219901,
-0.0131499332721656));
#18933=CARTESIAN_POINT('Ctrl Pts',(0.00471495254004244,-0.0377286024367416,
-0.0130381068754308));
#18934=CARTESIAN_POINT('Ctrl Pts',(0.00465268274694993,-0.0377232417255833,
-0.0129371455930511));
#18935=CARTESIAN_POINT('Ctrl Pts',(0.00457468299869719,-0.0377147545366238,
-0.0127705302791683));
#18936=CARTESIAN_POINT('Ctrl Pts',(0.00455064934321615,-0.0377116925299048,
-0.0127092861449259));
#18937=CARTESIAN_POINT('Ctrl Pts',(0.00452524934850776,-0.0377075980442318,
-0.0126300189172918));
#18938=CARTESIAN_POINT('Ctrl Pts',(0.00452018820768795,-0.037706724340247,
-0.0126132466069257));
#18939=CARTESIAN_POINT('Ctrl Pts',(0.00451284577453923,-0.0377053578740374,
-0.0125873263699636));
#18940=CARTESIAN_POINT('Ctrl Pts',(0.00451036079410119,-0.0377048756710023,
-0.0125782372030808));
#18941=CARTESIAN_POINT('Ctrl Pts',(0.00450583351982344,-0.0377039577637918,
-0.0125610611414061));
#18942=CARTESIAN_POINT('Ctrl Pts',(0.00450377330456181,-0.0377035230221076,
-0.012552979560188));
#18943=CARTESIAN_POINT('Ctrl Pts',(0.00449934107489913,-0.0377025491341382,
-0.0125349851270053));
#18944=CARTESIAN_POINT('Ctrl Pts',(0.00449700157425229,-0.0377020083096759,
-0.0125250646980416));
#18945=CARTESIAN_POINT('Ctrl Pts',(0.0044901785992861,-0.0377003476516746,
-0.0124947930931023));
#18946=CARTESIAN_POINT('Ctrl Pts',(0.00448600910315711,-0.0376992133191691,
-0.0124743742259443));
#18947=CARTESIAN_POINT('Ctrl Pts',(0.00446545223544528,-0.0376929243330159,
-0.0123621537026758));
#18948=CARTESIAN_POINT('Ctrl Pts',(0.004457,-0.0376875227620494,-0.0122690985381315));
#18949=CARTESIAN_POINT('Ctrl Pts',(0.004457,-0.0376822061652104,-0.0121758532865636));
#18950=CARTESIAN_POINT('Ctrl Pts',(0.004457,-0.0381835089768636,-0.0121758532865662));
#18951=CARTESIAN_POINT('Ctrl Pts',(0.004457,-0.0381835010212319,-0.0121756854996429));
#18952=CARTESIAN_POINT('Ctrl Pts',(0.00445700002522786,-0.0381834935385169,
-0.012175527700736));
#18953=CARTESIAN_POINT('Ctrl Pts',(0.00445700007887821,-0.0381834855813947,
-0.0121753599123022));
#18954=CARTESIAN_POINT('Origin',(0.006,-0.0418165664398416,-0.0121758532865581));
#18955=CARTESIAN_POINT('',(0.004457,-0.0386811151660051,-0.0121758532865589));
#18956=CARTESIAN_POINT('',(0.004457,-0.0385661060144854,-0.0121758532811924));
#18957=CARTESIAN_POINT('',(0.004457,-0.0418165664398416,-0.0121758532865581));
#18958=CARTESIAN_POINT('Ctrl Pts',(0.004457,-0.0380657947427934,-0.0121758532778082));
#18959=CARTESIAN_POINT('Ctrl Pts',(0.00445699999983535,-0.0380671435044447,
-0.0122048895953197));
#18960=CARTESIAN_POINT('Ctrl Pts',(0.00445781961298393,-0.038068505989213,
-0.0122339242157708));
#18961=CARTESIAN_POINT('Ctrl Pts',(0.00446118822220695,-0.0380713599617527,
-0.0122935261098348));
#18962=CARTESIAN_POINT('Ctrl Pts',(0.0044638293621826,-0.0380728535150145,
-0.0123240698070411));
#18963=CARTESIAN_POINT('Ctrl Pts',(0.00446869948897067,-0.0380749627659856,
-0.0123658479666247));
#18964=CARTESIAN_POINT('Ctrl Pts',(0.00447014652476572,-0.0380755410043585,
-0.0123771678740451));
#18965=CARTESIAN_POINT('Ctrl Pts',(0.00447282823197034,-0.0380765386945114,
-0.0123964438528787));
#18966=CARTESIAN_POINT('Ctrl Pts',(0.00447399987108635,-0.0380769547654142,
-0.0124044083395628));
#18967=CARTESIAN_POINT('Ctrl Pts',(0.00447665618908617,-0.0380778581390544,
-0.0124215334582408));
#18968=CARTESIAN_POINT('Ctrl Pts',(0.00447816123761015,-0.0380783464666718,
-0.0124306902653564));
#18969=CARTESIAN_POINT('Ctrl Pts',(0.00448267182002354,-0.0380797457356139,
-0.0124566666027664));
#18970=CARTESIAN_POINT('Ctrl Pts',(0.00448587418102869,-0.0380806664982276,
-0.012473450131933));
#18971=CARTESIAN_POINT('Ctrl Pts',(0.00450278334738427,-0.0380851947666801,
-0.012554716069166));
#18972=CARTESIAN_POINT('Ctrl Pts',(0.00452033361440335,-0.0380889513892934,
-0.012618324651428));
#18973=CARTESIAN_POINT('Ctrl Pts',(0.00456054257561717,-0.0380959989429903,
-0.0127344771135427));
#18974=CARTESIAN_POINT('Ctrl Pts',(0.00458216071951842,-0.0380992791774221,
-0.0127872699712157));
#18975=CARTESIAN_POINT('Ctrl Pts',(0.00463618295554917,-0.0381064019535798,
-0.0129008204621711));
#18976=CARTESIAN_POINT('Ctrl Pts',(0.00466983246931066,-0.0381102115358557,
-0.0129608567631454));
#18977=CARTESIAN_POINT('Ctrl Pts',(0.00471898888154054,-0.0381150191045294,
-0.0130362669221104));
#18978=CARTESIAN_POINT('Ctrl Pts',(0.00473096741426037,-0.0381161414827133,
-0.0130538381760918));
#18979=CARTESIAN_POINT('Ctrl Pts',(0.00475176843359826,-0.0381180109082736,
-0.0130830355604993));
#18980=CARTESIAN_POINT('Ctrl Pts',(0.00476039933485078,-0.03811876502757,
-0.0130947939439439));
#18981=CARTESIAN_POINT('Ctrl Pts',(0.00477810579649577,-0.0381202701655854,
-0.0131182129936916));
#18982=CARTESIAN_POINT('Ctrl Pts',(0.00478718471451662,-0.0381210209387773,
-0.0131298692010061));
#18983=CARTESIAN_POINT('Ctrl Pts',(0.00481036138111931,-0.0381228870031466,
-0.0131587594989513));
#18984=CARTESIAN_POINT('Ctrl Pts',(0.00482466753772719,-0.038123993898954,
-0.0131758224517869));
#18985=CARTESIAN_POINT('Ctrl Pts',(0.00489444620257537,-0.0381291945185664,
-0.013255480219889));
#18986=CARTESIAN_POINT('Ctrl Pts',(0.00495458055196259,-0.0381330928762353,
-0.0133138090911115));
#18987=CARTESIAN_POINT('Ctrl Pts',(0.00506820173835038,-0.0381398592891376,
-0.013407372142183));
#18988=CARTESIAN_POINT('Ctrl Pts',(0.00511970096203076,-0.0381427464205802,
-0.0134446952507317));
#18989=CARTESIAN_POINT('Ctrl Pts',(0.00521532228253025,-0.0381480312710724,
-0.0135053646154909));
#18990=CARTESIAN_POINT('Ctrl Pts',(0.00525855063894455,-0.0381503964402284,
-0.0135299476637632));
#18991=CARTESIAN_POINT('Ctrl Pts',(0.00531469273167647,-0.0381535299917057,
-0.0135583792707786));
#18992=CARTESIAN_POINT('Ctrl Pts',(0.00532657551026155,-0.0381541966332639,
-0.0135642061176475));
#18993=CARTESIAN_POINT('Ctrl Pts',(0.00534609763065624,-0.0381552996934874,
-0.0135734694101563));
#18994=CARTESIAN_POINT('Ctrl Pts',(0.00535369286322768,-0.0381557307606498,
-0.0135769978966976));
#18995=CARTESIAN_POINT('Ctrl Pts',(0.00536915626440788,-0.0381566129714147,
-0.013584029182476));
#18996=CARTESIAN_POINT('Ctrl Pts',(0.0053770257148027,-0.0381570642868594,
-0.013587528251132));
#18997=CARTESIAN_POINT('Ctrl Pts',(0.00539809565114217,-0.0381582780774296,
-0.0135966862915016));
#18998=CARTESIAN_POINT('Ctrl Pts',(0.00541134628720841,-0.0381590470467546,
-0.0136022270281897));
#18999=CARTESIAN_POINT('Ctrl Pts',(0.00549674573701938,-0.0381640298882131,
-0.013636544083683));
#19000=CARTESIAN_POINT('Ctrl Pts',(0.00557089842790941,-0.0381684730869033,
-0.01366002055429));
#19001=CARTESIAN_POINT('Ctrl Pts',(0.00571773034744465,-0.0381771292662065,
-0.0136945791371872));
#19002=CARTESIAN_POINT('Ctrl Pts',(0.00579007104340357,-0.038181329476216,
-0.0137062569606283));
#19003=CARTESIAN_POINT('Ctrl Pts',(0.00591298706225166,-0.0381882135544161,
-0.0137172160909405));
#19004=CARTESIAN_POINT('Ctrl Pts',(0.00596319466645026,-0.0381909570406077,
-0.0137192316097876));
#19005=CARTESIAN_POINT('Ctrl Pts',(0.0060328811100179,-0.0381946618576342,
-0.0137186257219291));
#19006=CARTESIAN_POINT('Ctrl Pts',(0.00605234274003579,-0.0381956855584709,
-0.0137180881060579));
#19007=CARTESIAN_POINT('Ctrl Pts',(0.00608605273259973,-0.0381974404138359,
-0.0137165180149759));
#19008=CARTESIAN_POINT('Ctrl Pts',(0.00610030625282324,-0.0381981767334831,
-0.0137156557258019));
#19009=CARTESIAN_POINT('Ctrl Pts',(0.00612978837194869,-0.0381996885863862,
-0.0137134610367704));
#19010=CARTESIAN_POINT('Ctrl Pts',(0.00614501329676942,-0.0382004631434111,
-0.0137120999400151));
#19011=CARTESIAN_POINT('Ctrl Pts',(0.00618493078721593,-0.0382024790188276,
-0.0137079326218436));
#19012=CARTESIAN_POINT('Ctrl Pts',(0.00620958055973648,-0.0382037087855468,
-0.0137047556901279));
#19013=CARTESIAN_POINT('Ctrl Pts',(0.00634520183711845,-0.0382104084754807,
-0.0136839346158737));
#19014=CARTESIAN_POINT('Ctrl Pts',(0.0064540638989913,-0.0382155082278199,
-0.0136548060586707));
#19015=CARTESIAN_POINT('Ctrl Pts',(0.0066080527406302,-0.0382230949450686,
-0.0135949771448086));
#19016=CARTESIAN_POINT('Ctrl Pts',(0.00665628472931976,-0.0382255354925383,
-0.0135733261791716));
#19017=CARTESIAN_POINT('Ctrl Pts',(0.00673046276573406,-0.0382295206826934,
-0.013535339902022));
#19018=CARTESIAN_POINT('Ctrl Pts',(0.00675719700238102,-0.0382310074785839,
-0.0135206328955101));
#19019=CARTESIAN_POINT('Ctrl Pts',(0.00679329132080773,-0.03823310868262,
-0.0134993591171764));
#19020=CARTESIAN_POINT('Ctrl Pts',(0.00680304182349797,-0.038233686004875,
-0.0134934657555407));
#19021=CARTESIAN_POINT('Ctrl Pts',(0.0068195667804657,-0.0382346826484039,
-0.0134832262472041));
#19022=CARTESIAN_POINT('Ctrl Pts',(0.00682637422978806,-0.0382350986085255,
-0.0134789340196165));
#19023=CARTESIAN_POINT('Ctrl Pts',(0.0068409668984029,-0.038236002406832,
-0.0134695727199938));
#19024=CARTESIAN_POINT('Ctrl Pts',(0.00684874025884699,-0.0382364912814053,
-0.0134644863845009));
#19025=CARTESIAN_POINT('Ctrl Pts',(0.00687071813542158,-0.0382378936499025,
-0.0134498204993014));
#19026=CARTESIAN_POINT('Ctrl Pts',(0.00688480931842805,-0.0382388170290535,
-0.0134400743724093));
#19027=CARTESIAN_POINT('Ctrl Pts',(0.00695318541922314,-0.0382434064491255,
-0.0133910790917609));
#19028=CARTESIAN_POINT('Ctrl Pts',(0.00700503398884929,-0.0382472264109391,
-0.0133485602651859));
#19029=CARTESIAN_POINT('Ctrl Pts',(0.00711364808810536,-0.0382557546904811,
-0.0132469823122669));
#19030=CARTESIAN_POINT('Ctrl Pts',(0.00716881789551368,-0.0382604558362534,
-0.0131864946073077));
#19031=CARTESIAN_POINT('Ctrl Pts',(0.00724827278224507,-0.0382676670690895,
-0.0130841225701488));
#19032=CARTESIAN_POINT('Ctrl Pts',(0.00727583545307731,-0.0382702756367614,
-0.0130449807613799));
#19033=CARTESIAN_POINT('Ctrl Pts',(0.00731183127054694,-0.0382738354530292,
-0.0129884510230028));
#19034=CARTESIAN_POINT('Ctrl Pts',(0.00732182412396684,-0.0382748426814859,
-0.0129720928190118));
#19035=CARTESIAN_POINT('Ctrl Pts',(0.00733870259558942,-0.038276578704659,
-0.0129432690603765));
#19036=CARTESIAN_POINT('Ctrl Pts',(0.00734572511522204,-0.0382773123576638,
-0.0129308867570101));
#19037=CARTESIAN_POINT('Ctrl Pts',(0.0073599870690814,-0.0382788271658381,
-0.0129049084037625));
#19038=CARTESIAN_POINT('Ctrl Pts',(0.00736719630766292,-0.0382796071984416,
-0.012891297533345));
#19039=CARTESIAN_POINT('Ctrl Pts',(0.00738576650746705,-0.0382816569149313,
-0.0128549313001057));
#19040=CARTESIAN_POINT('Ctrl Pts',(0.00739677092433287,-0.0382829142872373,
-0.0128319987257191));
#19041=CARTESIAN_POINT('Ctrl Pts',(0.00745910568851641,-0.0382903251724763,
-0.0126934132851662));
#19042=CARTESIAN_POINT('Ctrl Pts',(0.00749661634607974,-0.038295995319929,
-0.0125720829410429));
#19043=CARTESIAN_POINT('Ctrl Pts',(0.00752641323578653,-0.0383038150650187,
-0.0124054948146707));
#19044=CARTESIAN_POINT('Ctrl Pts',(0.00753218344960865,-0.0383058100427304,
-0.0123631662121021));
#19045=CARTESIAN_POINT('Ctrl Pts',(0.00753869538771927,-0.0383091507532485,
-0.0122940815738798));
#19046=CARTESIAN_POINT('Ctrl Pts',(0.00754051014702595,-0.0383104590097946,
-0.0122674489309357));
#19047=CARTESIAN_POINT('Ctrl Pts',(0.00754209023758461,-0.0383123466062829,
-0.0122299332980799));
#19048=CARTESIAN_POINT('Ctrl Pts',(0.00754243266808351,-0.0383128980394328,
-0.0122190782802948));
#19049=CARTESIAN_POINT('Ctrl Pts',(0.00754282799913165,-0.0383138656868881,
-0.0122002365298423));
#19050=CARTESIAN_POINT('Ctrl Pts',(0.00754293352804778,-0.0383142790835482,
-0.0121922515437699));
#19051=CARTESIAN_POINT('Ctrl Pts',(0.00754302945416275,-0.0383151975917776,
-0.012174657195347));
#19052=CARTESIAN_POINT('Ctrl Pts',(0.00754299208568446,-0.0383157040914283,
-0.0121650486037614));
#19053=CARTESIAN_POINT('Ctrl Pts',(0.0075426099839195,-0.0383172399311027,
-0.0121361670637015));
#19054=CARTESIAN_POINT('Ctrl Pts',(0.00754199384730864,-0.0383182824232954,
-0.0121169001787294));
#19055=CARTESIAN_POINT('Ctrl Pts',(0.00753429929071721,-0.0383266015347025,
-0.0119652753631933));
#19056=CARTESIAN_POINT('Ctrl Pts',(0.00751055399220591,-0.0383344211604439,
-0.0118343176925457));
#19057=CARTESIAN_POINT('Ctrl Pts',(0.0074527409386233,-0.0383451361653055,
-0.0116526227619363));
#19058=CARTESIAN_POINT('Ctrl Pts',(0.00743200395649937,-0.0383483317346125,
-0.0115982788779986));
#19059=CARTESIAN_POINT('Ctrl Pts',(0.00739993305659684,-0.0383525131053811,
-0.011526661191722));
#19060=CARTESIAN_POINT('Ctrl Pts',(0.00739125117212372,-0.0383535850660717,
-0.0115082582238994));
#19061=CARTESIAN_POINT('Ctrl Pts',(0.00737579762136287,-0.0383553956542925,
-0.0114771130742473));
#19062=CARTESIAN_POINT('Ctrl Pts',(0.00736920672792558,-0.0383561403636114,
-0.0114642846432739));
#19063=CARTESIAN_POINT('Ctrl Pts',(0.00735623250052009,-0.0383575556329396,
-0.0114398797149205));
#19064=CARTESIAN_POINT('Ctrl Pts',(0.00734987838464185,-0.0383582271308845,
-0.0114282892061757));
#19065=CARTESIAN_POINT('Ctrl Pts',(0.0073326569759924,-0.0383599919828613,
-0.0113978114194754));
#19066=CARTESIAN_POINT('Ctrl Pts',(0.00732153703285888,-0.0383610762836326,
-0.0113790699458166));
#19067=CARTESIAN_POINT('Ctrl Pts',(0.00727277703884525,-0.0383656134123758,
-0.0113007208444145));
#19068=CARTESIAN_POINT('Ctrl Pts',(0.0072314710588288,-0.0383689330870022,
-0.0112434915260968));
#19069=CARTESIAN_POINT('Ctrl Pts',(0.00713666224147379,-0.038375789466167,
-0.0111294796788135));
#19070=CARTESIAN_POINT('Ctrl Pts',(0.0070824815473084,-0.0383793031862586,
-0.0110735230549431));
#19071=CARTESIAN_POINT('Ctrl Pts',(0.00698719408205497,-0.0383852496005133,
-0.010988941121996));
#19072=CARTESIAN_POINT('Ctrl Pts',(0.00694850794566672,-0.0383876116666768,
-0.0109578037945299));
#19073=CARTESIAN_POINT('Ctrl Pts',(0.0068976980667432,-0.03839074160144,
-0.0109207986240512));
#19074=CARTESIAN_POINT('Ctrl Pts',(0.00688690460279309,-0.0383914080155726,
-0.0109131481632644));
#19075=CARTESIAN_POINT('Ctrl Pts',(0.0068691210274355,-0.0383925107951502,
-0.0109008835769566));
#19076=CARTESIAN_POINT('Ctrl Pts',(0.006862189125193,-0.0383929418143081,
-0.0108961857402235));
#19077=CARTESIAN_POINT('Ctrl Pts',(0.00684805002197483,-0.0383938240390514,
-0.0108867705303029));
#19078=CARTESIAN_POINT('Ctrl Pts',(0.00684084093976675,-0.0383942754181773,
-0.0108820566644812));
#19079=CARTESIAN_POINT('Ctrl Pts',(0.00682150244178063,-0.0383954895661715,
-0.0108696415247008));
#19080=CARTESIAN_POINT('Ctrl Pts',(0.0068093045319716,-0.0383962588355577,
-0.010862049049065));
#19081=CARTESIAN_POINT('Ctrl Pts',(0.00673041054715641,-0.0384012471820097,
-0.0108144578151061));
#19082=CARTESIAN_POINT('Ctrl Pts',(0.00666088142703747,-0.0384056961038836,
-0.0107793823368367));
#19083=CARTESIAN_POINT('Ctrl Pts',(0.00652124517955258,-0.0384143657152724,
-0.0107217116003165));
#19084=CARTESIAN_POINT('Ctrl Pts',(0.00645156624148771,-0.0384185736073102,
-0.010698587660835));
#19085=CARTESIAN_POINT('Ctrl Pts',(0.00633201987255703,-0.0384254537258592,
-0.010668168063386));
#19086=CARTESIAN_POINT('Ctrl Pts',(0.00628296127953114,-0.0384281866313684,
-0.0106581953640873));
#19087=CARTESIAN_POINT('Ctrl Pts',(0.00621428101686512,-0.0384318801254271,
-0.010647680943186));
#19088=CARTESIAN_POINT('Ctrl Pts',(0.00619500659929544,-0.0384329025710778,
-0.0106451019881817));
#19089=CARTESIAN_POINT('Ctrl Pts',(0.00616150568970234,-0.0384346559878718,
-0.0106412625622064));
#19090=CARTESIAN_POINT('Ctrl Pts',(0.00614730123415734,-0.0384353921006449,
-0.0106398340342204));
#19091=CARTESIAN_POINT('Ctrl Pts',(0.00611784268506092,-0.038436904156625,
-0.0106372838287038));
#19092=CARTESIAN_POINT('Ctrl Pts',(0.00610258759797816,-0.0384376791127551,
-0.0106361914141553));
#19093=CARTESIAN_POINT('Ctrl Pts',(0.00606246660066957,-0.0384396974558967,
-0.010633917321175));
#19094=CARTESIAN_POINT('Ctrl Pts',(0.00603758355311282,-0.0384409292364718,
-0.0106331102232206));
#19095=CARTESIAN_POINT('Ctrl Pts',(0.00590070773605617,-0.0384476122290726,
-0.0106319844003105));
#19096=CARTESIAN_POINT('Ctrl Pts',(0.00578895855843419,-0.0384526962910275,
-0.0106432563634802));
#19097=CARTESIAN_POINT('Ctrl Pts',(0.00562753024324628,-0.0384602744794229,
-0.0106775449104602));
#19098=CARTESIAN_POINT('Ctrl Pts',(0.00557625759070285,-0.0384627237239554,
-0.0106912309280556));
#19099=CARTESIAN_POINT('Ctrl Pts',(0.0054966971565738,-0.0384667212688756,
-0.0107169255354325));
#19100=CARTESIAN_POINT('Ctrl Pts',(0.0054678876145529,-0.0384682112883679,
-0.0107271848874768));
#19101=CARTESIAN_POINT('Ctrl Pts',(0.00542878057143002,-0.0384703163332968,
-0.0107424352128361));
#19102=CARTESIAN_POINT('Ctrl Pts',(0.00541820409357194,-0.0384708940952837,
-0.0107466953113026));
#19103=CARTESIAN_POINT('Ctrl Pts',(0.00540024381031434,-0.0384718912423945,
-0.0107541619350641));
#19104=CARTESIAN_POINT('Ctrl Pts',(0.00539283599439193,-0.0384723072569423,
-0.0107573097888319));
#19105=CARTESIAN_POINT('Ctrl Pts',(0.00537693635652429,-0.0384732108542385,
-0.0107642134935593));
#19106=CARTESIAN_POINT('Ctrl Pts',(0.00536845343464775,-0.0384736994678609,
-0.0107679881878198));
#19107=CARTESIAN_POINT('Ctrl Pts',(0.00534443616982334,-0.0384751003586363,
-0.01077893602743));
#19108=CARTESIAN_POINT('Ctrl Pts',(0.00532898675762177,-0.0384760224905309,
-0.0107862911445877));
#19109=CARTESIAN_POINT('Ctrl Pts',(0.00525410389899635,-0.0384805839235611,
-0.0108234811789877));
#19110=CARTESIAN_POINT('Ctrl Pts',(0.00519652276539376,-0.0384843749496947,
-0.0108568785200506));
#19111=CARTESIAN_POINT('Ctrl Pts',(0.00509244026825954,-0.0384915585975431,
-0.010926597552579));
#19112=CARTESIAN_POINT('Ctrl Pts',(0.00504550866506663,-0.0384949409309736,
-0.0109620776735448));
#19113=CARTESIAN_POINT('Ctrl Pts',(0.0049665555155074,-0.0385008022567649,
-0.0110291836133958));
#19114=CARTESIAN_POINT('Ctrl Pts',(0.00493367576372713,-0.0385033029436651,
-0.0110596938369025));
#19115=CARTESIAN_POINT('Ctrl Pts',(0.00487897702943803,-0.0385075531204408,
-0.0111150772351447));
#19116=CARTESIAN_POINT('Ctrl Pts',(0.00485654292742318,-0.0385093258457484,
-0.0111392991518396));
#19117=CARTESIAN_POINT('Ctrl Pts',(0.00482384759768811,-0.0385119554977753,
-0.0111769544901834));
#19118=CARTESIAN_POINT('Ctrl Pts',(0.00481300252016924,-0.0385128360635772,
-0.011189866323279));
#19119=CARTESIAN_POINT('Ctrl Pts',(0.00479352285001517,-0.0385144338525416,
-0.011213845589403));
#19120=CARTESIAN_POINT('Ctrl Pts',(0.00478482356381312,-0.0385151536248163,
-0.0112248579296845));
#19121=CARTESIAN_POINT('Ctrl Pts',(0.00476598893787307,-0.0385167266465979,
-0.0112493810020078));
#19122=CARTESIAN_POINT('Ctrl Pts',(0.00475592268616921,-0.0385175771543972,
-0.0112629426330942));
#19123=CARTESIAN_POINT('Ctrl Pts',(0.0047273722585249,-0.0385200206908794,
-0.0113027563338989));
#19124=CARTESIAN_POINT('Ctrl Pts',(0.00470948177230987,-0.0385215915557718,
-0.0113294240021196));
#19125=CARTESIAN_POINT('Ctrl Pts',(0.00462769671452698,-0.0385290080137881,
-0.0114599616109227));
#19126=CARTESIAN_POINT('Ctrl Pts',(0.00457543705715437,-0.0385344496172467,
-0.0115705952591806));
#19127=CARTESIAN_POINT('Ctrl Pts',(0.00451903842397314,-0.038542701158159,
-0.0117391434862632));
#19128=CARTESIAN_POINT('Ctrl Pts',(0.00450421677859805,-0.0385453389011639,
-0.0117929770926619));
#19129=CARTESIAN_POINT('Ctrl Pts',(0.00448945009426728,-0.038548789645804,
-0.0118607772532303));
#19130=CARTESIAN_POINT('Ctrl Pts',(0.00448673205127474,-0.0385494739204851,
-0.0118741017065303));
#19131=CARTESIAN_POINT('Ctrl Pts',(0.00448261115053832,-0.0385505986238379,
-0.0118957613584947));
#19132=CARTESIAN_POINT('Ctrl Pts',(0.0044810999946702,-0.0385510332852672,
-0.0119040754788661));
#19133=CARTESIAN_POINT('Ctrl Pts',(0.00447820165603089,-0.0385519143533416,
-0.0119208013739311));
#19134=CARTESIAN_POINT('Ctrl Pts',(0.00447681574874125,-0.0385523608031171,
-0.0119292130469584));
#19135=CARTESIAN_POINT('Ctrl Pts',(0.00447334572397001,-0.038553547455177,
-0.0119514198506197));
#19136=CARTESIAN_POINT('Ctrl Pts',(0.00447137892316355,-0.0385542936799903,
-0.0119652322461774));
#19137=CARTESIAN_POINT('Ctrl Pts',(0.00446201690499842,-0.0385582632002159,
-0.0120380410557255));
#19138=CARTESIAN_POINT('Ctrl Pts',(0.00445784960596041,-0.0385616215559427,
-0.012097397814629));
#19139=CARTESIAN_POINT('Ctrl Pts',(0.00445703903398348,-0.0385653806389522,
-0.0121631792977559));
#19140=CARTESIAN_POINT('Ctrl Pts',(0.00445700000004407,-0.0385657431904327,
-0.012169516646089));
#19141=CARTESIAN_POINT('Ctrl Pts',(0.004457,-0.0385661060144854,-0.0121758532758267));
#19142=CARTESIAN_POINT('Ctrl Pts',(0.004457,-0.0386811151660051,-0.0121758532865598));
#19143=CARTESIAN_POINT('Ctrl Pts',(0.004457,-0.0386810906944945,-0.0121753703966079));
#19144=CARTESIAN_POINT('Ctrl Pts',(0.00445700022668442,-0.038681066229755,
-0.0121748875055352));
#19145=CARTESIAN_POINT('Ctrl Pts',(0.00445701898307565,-0.0386800543821255,
-0.0121549098447703));
#19146=CARTESIAN_POINT('Ctrl Pts',(0.00445740673902861,-0.0386790782088258,
-0.0121354166724654));
#19147=CARTESIAN_POINT('Ctrl Pts',(0.00446002368905376,-0.0386757399764894,
-0.0120680759099084));
#19148=CARTESIAN_POINT('Ctrl Pts',(0.0044641110029321,-0.0386734334027347,
-0.0120203268189988));
#19149=CARTESIAN_POINT('Ctrl Pts',(0.0044811533560549,-0.0386673151593163,
-0.0118919211402397));
#19150=CARTESIAN_POINT('Ctrl Pts',(0.00449829838744569,-0.038663602515764,
-0.0118119780953627));
#19151=CARTESIAN_POINT('Ctrl Pts',(0.00454032753398168,-0.0386568328281487,
-0.0116714346343537));
#19152=CARTESIAN_POINT('Ctrl Pts',(0.0045628904833326,-0.0386537995783954,
-0.0116103474851028));
#19153=CARTESIAN_POINT('Ctrl Pts',(0.00459627983317719,-0.038649743129664,
-0.0115349781969822));
#19154=CARTESIAN_POINT('Ctrl Pts',(0.00460358873369526,-0.0386488759106765,
-0.0115192051946177));
#19155=CARTESIAN_POINT('Ctrl Pts',(0.00461525587475696,-0.0386475174485943,
-0.0114951029794756));
#19156=CARTESIAN_POINT('Ctrl Pts',(0.00461942654438151,-0.0386470365716885,
-0.0114866840779813));
#19157=CARTESIAN_POINT('Ctrl Pts',(0.00462744876830709,-0.0386461194342514,
-0.0114708555227298));
#19158=CARTESIAN_POINT('Ctrl Pts',(0.00463128399556532,-0.0386456841013622,
-0.0114634382261798));
#19159=CARTESIAN_POINT('Ctrl Pts',(0.0046408662321122,-0.0386446044985353,
-0.0114452692562471));
#19160=CARTESIAN_POINT('Ctrl Pts',(0.00464668076766474,-0.0386439563275059,
-0.0114345539800513));
#19161=CARTESIAN_POINT('Ctrl Pts',(0.00466994530470803,-0.0386413928391975,
-0.011392867194935));
#19162=CARTESIAN_POINT('Ctrl Pts',(0.00468833565358654,-0.0386394301784478,
-0.0113624351703959));
#19163=CARTESIAN_POINT('Ctrl Pts',(0.00474538677056307,-0.0386335759106839,
-0.0112750003716201));
#19164=CARTESIAN_POINT('Ctrl Pts',(0.00478683149534427,-0.0386296099623235,
-0.0112199180655523));
#19165=CARTESIAN_POINT('Ctrl Pts',(0.00488786551499036,-0.0386207736175767,
-0.0111028358377403));
#19166=CARTESIAN_POINT('Ctrl Pts',(0.0049492407491786,-0.0386159412703069,
-0.0110426641657795));
#19167=CARTESIAN_POINT('Ctrl Pts',(0.00503540683196787,-0.0386099075370377,
-0.0109712410551507));
#19168=CARTESIAN_POINT('Ctrl Pts',(0.00505592735877954,-0.0386085190153877,
-0.0109550922271287));
#19169=CARTESIAN_POINT('Ctrl Pts',(0.0050895381809652,-0.0386063202886948,
-0.0109299965250387));
#19170=CARTESIAN_POINT('Ctrl Pts',(0.00510237311183476,-0.03860549760612,
-0.0109207175217214));
#19171=CARTESIAN_POINT('Ctrl Pts',(0.00512738109421129,-0.0386039263137975,
-0.0109032178680065));
#19172=CARTESIAN_POINT('Ctrl Pts',(0.0051395330868172,-0.0386031767486838,
-0.0108949702420811));
#19173=CARTESIAN_POINT('Ctrl Pts',(0.00516842038676475,-0.0386014265189701,
-0.0108759609279524));
#19174=CARTESIAN_POINT('Ctrl Pts',(0.00518524991377004,-0.0386004312670951,
-0.0108653468429247));
#19175=CARTESIAN_POINT('Ctrl Pts',(0.00524598884131841,-0.0385969203903979,
-0.0108286623292766));
#19176=CARTESIAN_POINT('Ctrl Pts',(0.00529098249205345,-0.0385944688565585,
-0.0108044485123423));
#19177=CARTESIAN_POINT('Ctrl Pts',(0.00542116620066221,-0.0385876819934572,
-0.0107425117863365));
#19178=CARTESIAN_POINT('Ctrl Pts',(0.00550868046125469,-0.0385834804678757,
-0.0107102062432397));
#19179=CARTESIAN_POINT('Ctrl Pts',(0.0056522537860829,-0.0385765629595163,
-0.0106715220432754));
#19180=CARTESIAN_POINT('Ctrl Pts',(0.00570667387554513,-0.0385739318653432,
-0.0106599711247281));
#19181=CARTESIAN_POINT('Ctrl Pts',(0.00577540714706734,-0.0385704733419115,
-0.0106492221815898));
#19182=CARTESIAN_POINT('Ctrl Pts',(0.00578924895542135,-0.0385697700165762,
-0.0106472498546131));
#19183=CARTESIAN_POINT('Ctrl Pts',(0.00581173107477527,-0.0385686139221144,
-0.0106443575230082));
#19184=CARTESIAN_POINT('Ctrl Pts',(0.00582035599972359,-0.0385681671369668,
-0.0106433218873311));
#19185=CARTESIAN_POINT('Ctrl Pts',(0.00583775238339277,-0.0385672585985931,
-0.0106413818916083));
#19186=CARTESIAN_POINT('Ctrl Pts',(0.00584652372553353,-0.038566796758713,
-0.0106404797890516));
#19187=CARTESIAN_POINT('Ctrl Pts',(0.00586983984868978,-0.038565560010558,
-0.0106382835951181));
#19188=CARTESIAN_POINT('Ctrl Pts',(0.00588439580153568,-0.0385647785615512,
-0.0106371207364495));
#19189=CARTESIAN_POINT('Ctrl Pts',(0.00598057757042034,-0.0385595628500035,
-0.0106308092832336));
#19190=CARTESIAN_POINT('Ctrl Pts',(0.00606248057391231,-0.0385548808666727,
-0.0106319515709773));
#19191=CARTESIAN_POINT('Ctrl Pts',(0.00624770547829795,-0.0385442291220978,
-0.0106493012700618));
#19192=CARTESIAN_POINT('Ctrl Pts',(0.00635027096222377,-0.0385382996144999,
-0.0106695218005934));
#19193=CARTESIAN_POINT('Ctrl Pts',(0.00647462339648171,-0.0385312961124019,
-0.0107074381061901));
#19194=CARTESIAN_POINT('Ctrl Pts',(0.00649903452250175,-0.0385299290253567,
-0.0107155536052064));
#19195=CARTESIAN_POINT('Ctrl Pts',(0.00653805816088472,-0.0385277555103609,
-0.0107296199793372));
#19196=CARTESIAN_POINT('Ctrl Pts',(0.00655280155367318,-0.0385269371140008,
-0.0107351909979931));
#19197=CARTESIAN_POINT('Ctrl Pts',(0.00658114169539628,-0.0385253687222763,
-0.0107463988877147));
#19198=CARTESIAN_POINT('Ctrl Pts',(0.0065947481774895,-0.0385246178696821,
-0.0107520063239256));
#19199=CARTESIAN_POINT('Ctrl Pts',(0.00662674181885426,-0.0385228565068216,
-0.0107657300416678));
#19200=CARTESIAN_POINT('Ctrl Pts',(0.00664505491347601,-0.0385218516205357,
-0.0107740126829648));
#19201=CARTESIAN_POINT('Ctrl Pts',(0.00671084148448894,-0.0385182486334197,
-0.0108053288480932));
#19202=CARTESIAN_POINT('Ctrl Pts',(0.00675728896990039,-0.0385157195077449,
-0.010830436289441));
#19203=CARTESIAN_POINT('Ctrl Pts',(0.00688804394130476,-0.0385085251748819,
-0.0109100376374027));
#19204=CARTESIAN_POINT('Ctrl Pts',(0.00696843179801197,-0.0385040185832347,
-0.0109704279504564));
#19205=CARTESIAN_POINT('Ctrl Pts',(0.00707706949285719,-0.038497115150683,
-0.0110699677334163));
#19206=CARTESIAN_POINT('Ctrl Pts',(0.00711027709992211,-0.0384948693345765,
-0.0111033115976393));
#19207=CARTESIAN_POINT('Ctrl Pts',(0.00715102546269945,-0.0384918528828708,
-0.0111481504177021));
#19208=CARTESIAN_POINT('Ctrl Pts',(0.00716001048437217,-0.0384911700730022,
-0.0111583030640487));
#19209=CARTESIAN_POINT('Ctrl Pts',(0.00717392051151227,-0.0384900824173775,
-0.0111744444197034));
#19210=CARTESIAN_POINT('Ctrl Pts',(0.00717893632777092,-0.038489683762633,
-0.0111803543081208));
#19211=CARTESIAN_POINT('Ctrl Pts',(0.00718946695720243,-0.0384888323939499,
-0.0111929532348859));
#19212=CARTESIAN_POINT('Ctrl Pts',(0.00719497029626112,-0.0384883788651668,
-0.0111996513934755));
#19213=CARTESIAN_POINT('Ctrl Pts',(0.00720914705712648,-0.0384871887567263,
-0.0112172055552576));
#19214=CARTESIAN_POINT('Ctrl Pts',(0.00721773066450816,-0.0384864464365653,
-0.0112281328206827));
#19215=CARTESIAN_POINT('Ctrl Pts',(0.0072610648383999,-0.0384825917041162,
-0.0112848596707859));
#19216=CARTESIAN_POINT('Ctrl Pts',(0.00729338135720757,-0.0384793551753168,
-0.0113324566991023));
#19217=CARTESIAN_POINT('Ctrl Pts',(0.00739175791517952,-0.0384684656206931,
-0.0114963488249175));
#19218=CARTESIAN_POINT('Ctrl Pts',(0.00744538020307464,-0.0384607488976567,
-0.0116194331818831));
#19219=CARTESIAN_POINT('Ctrl Pts',(0.00748907988097694,-0.03845229313773,
-0.0117708114008163));
#19220=CARTESIAN_POINT('Ctrl Pts',(0.0074951628086487,-0.0384510292650615,
-0.0117938767432119));
#19221=CARTESIAN_POINT('Ctrl Pts',(0.00750428745822559,-0.0384489772655672,
-0.0118320435767394));
#19222=CARTESIAN_POINT('Ctrl Pts',(0.00750764202389111,-0.0384481795149103,
-0.0118470654770381));
#19223=CARTESIAN_POINT('Ctrl Pts',(0.00751380297430129,-0.0384466226588566,
-0.0118767347703391));
#19224=CARTESIAN_POINT('Ctrl Pts',(0.00751662287294446,-0.0384458632078929,
-0.0118913776059936));
#19225=CARTESIAN_POINT('Ctrl Pts',(0.00752295184845898,-0.0384440352975894,
-0.0119270165481736));
#19226=CARTESIAN_POINT('Ctrl Pts',(0.00752623961227817,-0.0384429737349884,
-0.0119480490830947));
#19227=CARTESIAN_POINT('Ctrl Pts',(0.00753776449116768,-0.0384387328826291,
-0.0120333019281696));
#19228=CARTESIAN_POINT('Ctrl Pts',(0.00754239164164807,-0.0384356623039623,
-0.0120979459014267));
#19229=CARTESIAN_POINT('Ctrl Pts',(0.00754363468893113,-0.0384288801778244,
-0.0122436876370925));
#19230=CARTESIAN_POINT('Ctrl Pts',(0.00753794702050676,-0.0384252136974585,
-0.0123246083203443));
#19231=CARTESIAN_POINT('Ctrl Pts',(0.00751836782412125,-0.0384190508880638,
-0.0124551570964609));
#19232=CARTESIAN_POINT('Ctrl Pts',(0.00750830472959757,-0.0384166255455801,
-0.0125051973739129));
#19233=CARTESIAN_POINT('Ctrl Pts',(0.00749239341269471,-0.0384134014665868,
-0.0125680287095958));
#19234=CARTESIAN_POINT('Ctrl Pts',(0.00748882428324351,-0.038412706529619,
-0.0125813676387868));
#19235=CARTESIAN_POINT('Ctrl Pts',(0.00748296028901683,-0.0384116042684971,
-0.0126021613730741));
#19236=CARTESIAN_POINT('Ctrl Pts',(0.0074807870229216,-0.0384112034259478,
-0.0126096500029412));
#19237=CARTESIAN_POINT('Ctrl Pts',(0.00747609314404917,-0.0384103527857387,
-0.0126253777735206));
#19238=CARTESIAN_POINT('Ctrl Pts',(0.0074735601277721,-0.0384099022510064,
-0.0126336128024261));
#19239=CARTESIAN_POINT('Ctrl Pts',(0.00746684072127418,-0.0384087292471139,
-0.0126548242779768));
#19240=CARTESIAN_POINT('Ctrl Pts',(0.00746255110138742,-0.0384080013250164,
-0.0126677670631409));
#19241=CARTESIAN_POINT('Ctrl Pts',(0.0074408399556796,-0.0384044205694814,
-0.0127304789707125));
#19242=CARTESIAN_POINT('Ctrl Pts',(0.00742104758291845,-0.0384014631435197,
-0.0127793865148959));
#19243=CARTESIAN_POINT('Ctrl Pts',(0.00736529235336711,-0.0383939560477157,
-0.0128991265612218));
#19244=CARTESIAN_POINT('Ctrl Pts',(0.00732628962771408,-0.0383893728985182,
-0.0129683833886149));
#19245=CARTESIAN_POINT('Ctrl Pts',(0.00724634686018956,-0.0383812672313015,
-0.0130877773319307));
#19246=CARTESIAN_POINT('Ctrl Pts',(0.00720725222068425,-0.0383777145492173,
-0.0131389366030628));
#19247=CARTESIAN_POINT('Ctrl Pts',(0.00715092324530721,-0.038373127256583,
-0.0132038078279602));
#19248=CARTESIAN_POINT('Ctrl Pts',(0.00713643122051977,-0.0383719881826513,
-0.0132198068288556));
#19249=CARTESIAN_POINT('Ctrl Pts',(0.00711143400935017,-0.0383700903919216,
-0.0132462657837207));
#19250=CARTESIAN_POINT('Ctrl Pts',(0.00710110544148126,-0.0383693245276794,
-0.0132568876513459));
#19251=CARTESIAN_POINT('Ctrl Pts',(0.00707981369716824,-0.038367781699566,
-0.0132781622136346));
#19252=CARTESIAN_POINT('Ctrl Pts',(0.00706884199125089,-0.0383670052388432,
-0.0132888040537846));
#19253=CARTESIAN_POINT('Ctrl Pts',(0.00704075054521407,-0.0383650621557736,
-0.0133152523047962));
#19254=CARTESIAN_POINT('Ctrl Pts',(0.00702342731511748,-0.0383639047241738,
-0.0133308374512071));
#19255=CARTESIAN_POINT('Ctrl Pts',(0.0069334747876976,-0.0383580856871029,
-0.0134081512445624));
#19256=CARTESIAN_POINT('Ctrl Pts',(0.00685558748736433,-0.0383536792434703,
-0.0134634500480332));
#19257=CARTESIAN_POINT('Ctrl Pts',(0.00669340759837118,-0.038345062373516,
-0.0135573426541664));
#19258=CARTESIAN_POINT('Ctrl Pts',(0.00660976051664869,-0.0383408620440565,
-0.013596246142168));
#19259=CARTESIAN_POINT('Ctrl Pts',(0.00650761428110306,-0.0383355062967678,
-0.0136330593876282));
#19260=CARTESIAN_POINT('Ctrl Pts',(0.00649198529757305,-0.0383346806024656,
-0.0136384100568866));
#19261=CARTESIAN_POINT('Ctrl Pts',(0.00646750524636395,-0.0383333733942934,
-0.0136463541649019));
#19262=CARTESIAN_POINT('Ctrl Pts',(0.00645871136508243,-0.0383329010449012,
-0.0136491210368244));
#19263=CARTESIAN_POINT('Ctrl Pts',(0.00644183622826642,-0.0383319884338862,
-0.0136542648319799));
#19264=CARTESIAN_POINT('Ctrl Pts',(0.00643375944569259,-0.0383315488717997,
-0.0136566546513163));
#19265=CARTESIAN_POINT('Ctrl Pts',(0.00641352915153954,-0.0383304415807624,
-0.0136624608403344));
#19266=CARTESIAN_POINT('Ctrl Pts',(0.00640135261775309,-0.038329769491082,
-0.0136657943708276));
#19267=CARTESIAN_POINT('Ctrl Pts',(0.00635071716163203,-0.038326955377435,
-0.013678990941803));
#19268=CARTESIAN_POINT('Ctrl Pts',(0.00631192769250872,-0.0383247540837484,
-0.013687516617592));
#19269=CARTESIAN_POINT('Ctrl Pts',(0.00618803528889515,-0.0383176665934017,
-0.0137097758541176));
#19270=CARTESIAN_POINT('Ctrl Pts',(0.00610208777855087,-0.0383126754488808,
-0.0137178825066896));
#19271=CARTESIAN_POINT('Ctrl Pts',(0.00594452091180687,-0.0383037460751729,
-0.0137195074967112));
#19272=CARTESIAN_POINT('Ctrl Pts',(0.00587315880430296,-0.0382997829439983,
-0.0137152880800327));
#19273=CARTESIAN_POINT('Ctrl Pts',(0.00578037711294673,-0.0382947811978246,
-0.0137033038236897));
#19274=CARTESIAN_POINT('Ctrl Pts',(0.00575847849812121,-0.0382936112973411,
-0.0136999946141831));
#19275=CARTESIAN_POINT('Ctrl Pts',(0.00572329557706447,-0.0382917481804231,
-0.0136939005755142));
#19276=CARTESIAN_POINT('Ctrl Pts',(0.00570996406048768,-0.038291046040352,
-0.0136914099757818));
#19277=CARTESIAN_POINT('Ctrl Pts',(0.00568203656896372,-0.0382895827504961,
-0.0136858105394262));
#19278=CARTESIAN_POINT('Ctrl Pts',(0.00566744932395982,-0.0382888228225961,
-0.0136826650587088));
#19279=CARTESIAN_POINT('Ctrl Pts',(0.00563211085905527,-0.0382869914718425,
-0.0136745067575425));
#19280=CARTESIAN_POINT('Ctrl Pts',(0.00561141336080147,-0.0382859270123157,
-0.0136692738986096));
#19281=CARTESIAN_POINT('Ctrl Pts',(0.00552769350396161,-0.038281647378967,
-0.0136462489348721));
#19282=CARTESIAN_POINT('Ctrl Pts',(0.00546572260379649,-0.0382785436854398,
-0.0136248824427185));
#19283=CARTESIAN_POINT('Ctrl Pts',(0.00535108239995343,-0.0382727653424974,
-0.013576997988481));
#19284=CARTESIAN_POINT('Ctrl Pts',(0.00529820874002883,-0.0382700832500512,
-0.0135512767123211));
#19285=CARTESIAN_POINT('Ctrl Pts',(0.00518950682885686,-0.0382643374613907,
-0.0134904933150084));
#19286=CARTESIAN_POINT('Ctrl Pts',(0.00513419949053004,-0.0382612721988115,
-0.0134547456652044));
#19287=CARTESIAN_POINT('Ctrl Pts',(0.00506735007849969,-0.0382571783445711,
-0.0134052094641428));
#19288=CARTESIAN_POINT('Ctrl Pts',(0.00505353039273019,-0.0382563093329121,
-0.0133946017117112));
#19289=CARTESIAN_POINT('Ctrl Pts',(0.0050325329023907,-0.0382549486598804,
-0.0133779118666027));
#19290=CARTESIAN_POINT('Ctrl Pts',(0.0050252258157321,-0.0382544674180131,
-0.0133719940374326));
#19291=CARTESIAN_POINT('Ctrl Pts',(0.00501153456004873,-0.0382535500630858,
-0.0133606970568774));
#19292=CARTESIAN_POINT('Ctrl Pts',(0.00500513924416309,-0.0382531148871735,
-0.0133553323033181));
#19293=CARTESIAN_POINT('Ctrl Pts',(0.00498952463037424,-0.0382520363580196,
-0.0133420165423097));
#19294=CARTESIAN_POINT('Ctrl Pts',(0.0049803554012407,-0.03825138912159,
-0.0133340078902502));
#19295=CARTESIAN_POINT('Ctrl Pts',(0.00494489936074645,-0.0382488348100471,
-0.0133022922047216));
#19296=CARTESIAN_POINT('Ctrl Pts',(0.00491933805006229,-0.0382468808018378,
-0.0132777931333543));
#19297=CARTESIAN_POINT('Ctrl Pts',(0.00484698483815757,-0.038241066856399,
-0.0132035063153651));
#19298=CARTESIAN_POINT('Ctrl Pts',(0.00480262915094476,-0.0382371335511976,
-0.0131514645767921));
#19299=CARTESIAN_POINT('Ctrl Pts',(0.00471023087156845,-0.0382282851740607,
-0.0130272239135652));
#19300=CARTESIAN_POINT('Ctrl Pts',(0.00466452036365229,-0.0382234094264812,
-0.0129535637667349));
#19301=CARTESIAN_POINT('Ctrl Pts',(0.00461336822153091,-0.0382173358446065,
-0.0128531885450019));
#19302=CARTESIAN_POINT('Ctrl Pts',(0.00460210486739035,-0.0382159471816289,
-0.01282962698433));
#19303=CARTESIAN_POINT('Ctrl Pts',(0.00458497889799723,-0.0382137482881738,
-0.0127913328487209));
#19304=CARTESIAN_POINT('Ctrl Pts',(0.00457873618313873,-0.038212925576805,
-0.0127767767407702));
#19305=CARTESIAN_POINT('Ctrl Pts',(0.00456713872999419,-0.0382113542634237,
-0.0127485427654217));
#19306=CARTESIAN_POINT('Ctrl Pts',(0.00456175303948874,-0.0382106047054126,
-0.012734879545228));
#19307=CARTESIAN_POINT('Ctrl Pts',(0.00454953288070422,-0.0382088545437266,
-0.0127025314455793));
#19308=CARTESIAN_POINT('Ctrl Pts',(0.00454286302742768,-0.038207859351457,
-0.0126837869783028));
#19309=CARTESIAN_POINT('Ctrl Pts',(0.00452037622361846,-0.0382043490389647,
-0.0126164990860643));
#19310=CARTESIAN_POINT('Ctrl Pts',(0.00450660734237072,-0.0382018979803378,
-0.0125673046738582));
#19311=CARTESIAN_POINT('Ctrl Pts',(0.00446984551504731,-0.0381940821302627,
-0.0124054034729965));
#19312=CARTESIAN_POINT('Ctrl Pts',(0.00445700000000001,-0.0381889595111803,
-0.0122908068720926));
#19313=CARTESIAN_POINT('Ctrl Pts',(0.00445700000000001,-0.0381835089768636,
-0.0121758532865662));
#19314=CARTESIAN_POINT('Origin',(0.006,-0.0418165664398416,-0.0121758532865581));
#19315=CARTESIAN_POINT('',(0.004457,-0.0391830969990905,-0.0121758532988723));
#19316=CARTESIAN_POINT('',(0.004457,-0.0390679979850714,-0.0121758532865563));
#19317=CARTESIAN_POINT('',(0.004457,-0.0418165664398416,-0.0121758532865581));
#19318=CARTESIAN_POINT('Ctrl Pts',(0.004457,-0.0385661060144854,-0.0121758532758267));
#19319=CARTESIAN_POINT('Ctrl Pts',(0.00445699999940689,-0.0385709890096937,
-0.0122611335443476));
#19320=CARTESIAN_POINT('Ctrl Pts',(0.00446407020437146,-0.0385759100486242,
-0.0123462843053963));
#19321=CARTESIAN_POINT('Ctrl Pts',(0.00448649972637195,-0.0385834971460825,
-0.0124803692373493));
#19322=CARTESIAN_POINT('Ctrl Pts',(0.0044973078821122,-0.0385862646457588,
-0.0125298733343161));
#19323=CARTESIAN_POINT('Ctrl Pts',(0.00451562854401043,-0.0385899951329252,
-0.0125976012485272));
#19324=CARTESIAN_POINT('Ctrl Pts',(0.00452108232020828,-0.0385910216618756,
-0.0126163444961434));
#19325=CARTESIAN_POINT('Ctrl Pts',(0.00453114143214295,-0.0385927797623273,
-0.0126486192027317));
#19326=CARTESIAN_POINT('Ctrl Pts',(0.00453558175434474,-0.0385935165519015,
-0.0126621991755757));
#19327=CARTESIAN_POINT('Ctrl Pts',(0.00454515550583596,-0.0385950279652326,
-0.0126901581924258));
#19328=CARTESIAN_POINT('Ctrl Pts',(0.00455031503315732,-0.0385958016369882,
-0.0127045266798043));
#19329=CARTESIAN_POINT('Ctrl Pts',(0.00456439801452056,-0.0385978120297865,
-0.0127419882036284));
#19330=CARTESIAN_POINT('Ctrl Pts',(0.00457366560029978,-0.0385990373205938,
-0.0127649475653962));
#19331=CARTESIAN_POINT('Ctrl Pts',(0.00462835386203875,-0.038605773129083,
-0.0128915644051006));
#19332=CARTESIAN_POINT('Ctrl Pts',(0.00468451717056739,-0.0386109068707634,
-0.0129902009822645));
#19333=CARTESIAN_POINT('Ctrl Pts',(0.00478173699898775,-0.0386185122447016,
-0.0131242365729653));
#19334=CARTESIAN_POINT('Ctrl Pts',(0.00481464792204486,-0.038620934059732,
-0.0131650628337481));
#19335=CARTESIAN_POINT('Ctrl Pts',(0.00486980110266417,-0.038624892609201,
-0.0132267676745674));
#19336=CARTESIAN_POINT('Ctrl Pts',(0.00489069450856048,-0.038626372428177,
-0.0132487986324183));
#19337=CARTESIAN_POINT('Ctrl Pts',(0.00492028925441706,-0.0386284653192406,
-0.0132782157780816));
#19338=CARTESIAN_POINT('Ctrl Pts',(0.00492844389039881,-0.0386290416886927,
-0.0132861441701766));
#19339=CARTESIAN_POINT('Ctrl Pts',(0.00494251502703814,-0.0386300372444446,
-0.0132995255053569));
#19340=CARTESIAN_POINT('Ctrl Pts',(0.00494838797927676,-0.0386304530900695,
-0.013305023725347));
#19341=CARTESIAN_POINT('Ctrl Pts',(0.00496114237755294,-0.0386313573372578,
-0.0133167784946628));
#19342=CARTESIAN_POINT('Ctrl Pts',(0.00496803767863141,-0.0386318467872882,
-0.0133230190326023));
#19343=CARTESIAN_POINT('Ctrl Pts',(0.00498783179428647,-0.0386332524102091,
-0.0133406106623483));
#19344=CARTESIAN_POINT('Ctrl Pts',(0.00500086404683463,-0.0386341785355146,
-0.0133518088644727));
#19345=CARTESIAN_POINT('Ctrl Pts',(0.00506632977434108,-0.0386388223371126,
-0.013406187627188));
#19346=CARTESIAN_POINT('Ctrl Pts',(0.00512138492249497,-0.0386426981688242,
-0.0134460882935113));
#19347=CARTESIAN_POINT('Ctrl Pts',(0.00523284927792429,-0.0386502494071937,
-0.0135161485649029));
#19348=CARTESIAN_POINT('Ctrl Pts',(0.0052888657804517,-0.0386539152291565,
-0.0135466925845617));
#19349=CARTESIAN_POINT('Ctrl Pts',(0.00538403385103367,-0.0386598338242587,
-0.0135911769380323));
#19350=CARTESIAN_POINT('Ctrl Pts',(0.00542214445899041,-0.0386621283351545,
-0.0136071599186868));
#19351=CARTESIAN_POINT('Ctrl Pts',(0.00549005124991666,-0.0386660740632042,
-0.0136324837790437));
#19352=CARTESIAN_POINT('Ctrl Pts',(0.0055195742016699,-0.0386677440908403,
-0.0136424859457626));
#19353=CARTESIAN_POINT('Ctrl Pts',(0.00556518152021704,-0.0386702554322559,
-0.013656412239432));
#19354=CARTESIAN_POINT('Ctrl Pts',(0.00558105856779777,-0.0386711172737177,
-0.0136609829199271));
#19355=CARTESIAN_POINT('Ctrl Pts',(0.00561056007057306,-0.0386726964271143,
-0.013668965034545));
#19356=CARTESIAN_POINT('Ctrl Pts',(0.0056241634606518,-0.0386734159411043,
-0.0136724471069856));
#19357=CARTESIAN_POINT('Ctrl Pts',(0.00565459118928566,-0.0386750068497171,
-0.0136797946695633));
#19358=CARTESIAN_POINT('Ctrl Pts',(0.00567143679205483,-0.0386758751263171,
-0.0136835645250743));
#19359=CARTESIAN_POINT('Ctrl Pts',(0.00571508025521172,-0.0386780946783948,
-0.0136925652071506));
#19360=CARTESIAN_POINT('Ctrl Pts',(0.00574196045330526,-0.0386794326957031,
-0.0136973689817397));
#19361=CARTESIAN_POINT('Ctrl Pts',(0.00588340840946179,-0.0386863462829957,
-0.0137187905608759));
#19362=CARTESIAN_POINT('Ctrl Pts',(0.00599944489334954,-0.0386915492269238,
-0.0137231895023478));
#19363=CARTESIAN_POINT('Ctrl Pts',(0.00615886669417164,-0.0386989277351179,
-0.0137112866322648));
#19364=CARTESIAN_POINT('Ctrl Pts',(0.00620268554574487,-0.0387009846113517,
-0.0137061187499411));
#19365=CARTESIAN_POINT('Ctrl Pts',(0.00627312582169957,-0.0387044162589633,
-0.0136947325092945));
#19366=CARTESIAN_POINT('Ctrl Pts',(0.00629990974056779,-0.0387057509541106,
-0.013689671570812));
#19367=CARTESIAN_POINT('Ctrl Pts',(0.00633723965334561,-0.0387076703018036,
-0.0136815883810114));
#19368=CARTESIAN_POINT('Ctrl Pts',(0.00634790997282678,-0.0387082257699806,
-0.0136791587765198));
#19369=CARTESIAN_POINT('Ctrl Pts',(0.00636632852791285,-0.0387091978497788,
-0.0136747583253562));
#19370=CARTESIAN_POINT('Ctrl Pts',(0.00637408875552441,-0.038709611556863,
-0.0136728404295587));
#19371=CARTESIAN_POINT('Ctrl Pts',(0.0063910902895269,-0.0387105273822365,
-0.0136684981377507));
#19372=CARTESIAN_POINT('Ctrl Pts',(0.00640032411273534,-0.038711030826235,
-0.0136660481939017));
#19373=CARTESIAN_POINT('Ctrl Pts',(0.00642783914953927,-0.0387125478352314,
-0.0136584736425784));
#19374=CARTESIAN_POINT('Ctrl Pts',(0.00644604861426834,-0.0387135741067202,
-0.0136530973522419));
#19375=CARTESIAN_POINT('Ctrl Pts',(0.0065909449017571,-0.0387218942948715,
-0.0136073939328253));
#19376=CARTESIAN_POINT('Ctrl Pts',(0.00671203570948084,-0.0387297391216645,
-0.0135511831346742));
#19377=CARTESIAN_POINT('Ctrl Pts',(0.00687358936273519,-0.0387404798493248,
-0.0134490671235244));
#19378=CARTESIAN_POINT('Ctrl Pts',(0.00692096071345067,-0.0387436781036921,
-0.0134152339094243));
#19379=CARTESIAN_POINT('Ctrl Pts',(0.00698217785597301,-0.0387478622631298,
-0.0133660590619536));
#19380=CARTESIAN_POINT('Ctrl Pts',(0.00699778998668464,-0.0387489344797945,
-0.0133530016730107));
#19381=CARTESIAN_POINT('Ctrl Pts',(0.00702401756165004,-0.0387507453647904,
-0.0133301691165515));
#19382=CARTESIAN_POINT('Ctrl Pts',(0.00703476228085287,-0.038751490119866,
-0.0133205471507517));
#19383=CARTESIAN_POINT('Ctrl Pts',(0.00705509168999932,-0.0387529053898367,
-0.0133018218447952));
#19384=CARTESIAN_POINT('Ctrl Pts',(0.00706469735771112,-0.0387535768441155,
-0.0132927432627463));
#19385=CARTESIAN_POINT('Ctrl Pts',(0.00708982335245743,-0.0387553413827213,
-0.01326837723697));
#19386=CARTESIAN_POINT('Ctrl Pts',(0.00710513885758565,-0.0387564254201723,
-0.0132528823882556));
#19387=CARTESIAN_POINT('Ctrl Pts',(0.00716852236978042,-0.0387609565345682,
-0.0131859805195332));
#19388=CARTESIAN_POINT('Ctrl Pts',(0.00721337401237781,-0.0387642709580579,
-0.0131316389823852));
#19389=CARTESIAN_POINT('Ctrl Pts',(0.00730015746286802,-0.0387711620494802,
-0.0130104931506991));
#19390=CARTESIAN_POINT('Ctrl Pts',(0.00734099756007175,-0.0387747134378307,
-0.0129431590276437));
#19391=CARTESIAN_POINT('Ctrl Pts',(0.0073915657781781,-0.0387799400909755,
-0.0128433123926883));
#19392=CARTESIAN_POINT('Ctrl Pts',(0.00740563960438962,-0.0387815157303427,
-0.0128131397834844));
#19393=CARTESIAN_POINT('Ctrl Pts',(0.00742760053641603,-0.0387842272089786,
-0.0127617842941983));
#19394=CARTESIAN_POINT('Ctrl Pts',(0.00743601816660517,-0.0387853410720547,
-0.0127408401603902));
#19395=CARTESIAN_POINT('Ctrl Pts',(0.00744756924535867,-0.0387869937780881,
-0.0127101718977647));
#19396=CARTESIAN_POINT('Ctrl Pts',(0.00745107059966241,-0.038787513246508,
-0.0127005886506733));
#19397=CARTESIAN_POINT('Ctrl Pts',(0.00745713106761091,-0.0387884473550531,
-0.0126834764499495));
#19398=CARTESIAN_POINT('Ctrl Pts',(0.00745972741642108,-0.0387888598714829,
-0.0126759613633439));
#19399=CARTESIAN_POINT('Ctrl Pts',(0.00746550480500243,-0.0387898065931268,
-0.0126588104529277));
#19400=CARTESIAN_POINT('Ctrl Pts',(0.00746864896773013,-0.0387903427754529,
-0.0126491630759093));
#19401=CARTESIAN_POINT('Ctrl Pts',(0.00747838156524733,-0.038792069818363,
-0.0126182691130563));
#19402=CARTESIAN_POINT('Ctrl Pts',(0.00748460556736955,-0.0387932787701087,
-0.012596911512547));
#19403=CARTESIAN_POINT('Ctrl Pts',(0.00749827381271102,-0.0387961878758144,
-0.0125459305990151));
#19404=CARTESIAN_POINT('Ctrl Pts',(0.00750530440886435,-0.0387979023701727,
-0.0125162062061284));
#19405=CARTESIAN_POINT('Ctrl Pts',(0.0075322339012315,-0.0388054921279668,
-0.0123850942017186));
#19406=CARTESIAN_POINT('Ctrl Pts',(0.00754280473558756,-0.0388115056641097,
-0.0122820531008686));
#19407=CARTESIAN_POINT('Ctrl Pts',(0.00754309520517498,-0.0388202263478965,
-0.0121262124846427));
#19408=CARTESIAN_POINT('Ctrl Pts',(0.00754051191508808,-0.0388231043212167,
-0.0120737215490195));
#19409=CARTESIAN_POINT('Ctrl Pts',(0.00753323443262685,-0.0388269784654415,
-0.0120013555296904));
#19410=CARTESIAN_POINT('Ctrl Pts',(0.00753081780543674,-0.0388280427772368,
-0.0119812917520572));
#19411=CARTESIAN_POINT('Ctrl Pts',(0.00752602536084484,-0.0388298370575668,
-0.0119471639639889));
#19412=CARTESIAN_POINT('Ctrl Pts',(0.00752384744410326,-0.0388305730851583,
-0.0119330752123572));
#19413=CARTESIAN_POINT('Ctrl Pts',(0.00751897683311214,-0.038832071375265,
-0.0119042220097796));
#19414=CARTESIAN_POINT('Ctrl Pts',(0.00751626335299476,-0.0388328328978096,
-0.0118894625834476));
#19415=CARTESIAN_POINT('Ctrl Pts',(0.00750875871866872,-0.0388347675688254,
-0.0118517452036579));
#19416=CARTESIAN_POINT('Ctrl Pts',(0.0075036586387808,-0.0388359309165052,
-0.0118288522911677));
#19417=CARTESIAN_POINT('Ctrl Pts',(0.00749131984209509,-0.0388384525972845,
-0.0117788644196382));
#19418=CARTESIAN_POINT('Ctrl Pts',(0.00748386033510217,-0.0388398040659622,
-0.0117518324829939));
#19419=CARTESIAN_POINT('Ctrl Pts',(0.00745785475387192,-0.0388440394432382,
-0.0116667113819958));
#19420=CARTESIAN_POINT('Ctrl Pts',(0.00743660076830057,-0.0388468529650445,
-0.01160951001503));
#19421=CARTESIAN_POINT('Ctrl Pts',(0.00737129899910049,-0.0388542840793461,
-0.0114612999156701));
#19422=CARTESIAN_POINT('Ctrl Pts',(0.00732161082864321,-0.0388588484769401,
-0.0113731154636837));
#19423=CARTESIAN_POINT('Ctrl Pts',(0.00725472005643039,-0.0388646081950955,
-0.0112776495257963));
#19424=CARTESIAN_POINT('Ctrl Pts',(0.0072455742501692,-0.0388653891644274,
-0.0112650090800789));
#19425=CARTESIAN_POINT('Ctrl Pts',(0.00723092857219079,-0.0388666333593654,
-0.0112454003897197));
#19426=CARTESIAN_POINT('Ctrl Pts',(0.00722555735664718,-0.0388670883651384,
-0.0112383369393916));
#19427=CARTESIAN_POINT('Ctrl Pts',(0.00721510315753404,-0.0388679723195448,
-0.011224832448114));
#19428=CARTESIAN_POINT('Ctrl Pts',(0.00721002923548567,-0.038868400688288,
-0.0112183849804889));
#19429=CARTESIAN_POINT('Ctrl Pts',(0.00719718326573156,-0.0388694830023113,
-0.0112023267076361));
#19430=CARTESIAN_POINT('Ctrl Pts',(0.00718934676330783,-0.0388701412416195,
-0.0111927683312699));
#19431=CARTESIAN_POINT('Ctrl Pts',(0.00715630001500794,-0.0388729050837193,
-0.0111534338916031));
#19432=CARTESIAN_POINT('Ctrl Pts',(0.00713008121286506,-0.0388750693167788,
-0.0111245268969704));
#19433=CARTESIAN_POINT('Ctrl Pts',(0.00704457501190154,-0.0388819596506758,
-0.0110371516006546));
#19434=CARTESIAN_POINT('Ctrl Pts',(0.00698163427724544,-0.0388867894521148,
-0.0109824662078976));
#19435=CARTESIAN_POINT('Ctrl Pts',(0.00685258671293617,-0.0388959108445775,
-0.0108874932903238));
#19436=CARTESIAN_POINT('Ctrl Pts',(0.00678725015290552,-0.0389002032558147,
-0.0108465620415681));
#19437=CARTESIAN_POINT('Ctrl Pts',(0.00669965041806136,-0.0389055004582567,
-0.0108004178163234));
#19438=CARTESIAN_POINT('Ctrl Pts',(0.0066799590767812,-0.0389066639305614,
-0.0107905774437305));
#19439=CARTESIAN_POINT('Ctrl Pts',(0.00664675351842411,-0.0389085815847088,
-0.0107748623111406));
#19440=CARTESIAN_POINT('Ctrl Pts',(0.00663335402512636,-0.0389093436730812,
-0.0107687539561798));
#19441=CARTESIAN_POINT('Ctrl Pts',(0.00660647325525143,-0.0389108498348272,
-0.010756961759837));
#19442=CARTESIAN_POINT('Ctrl Pts',(0.00659299451386712,-0.0389115939160566,
-0.0107512759810167));
#19443=CARTESIAN_POINT('Ctrl Pts',(0.00655951499615744,-0.0389134158038965,
-0.0107377107357966));
#19444=CARTESIAN_POINT('Ctrl Pts',(0.00653942629226251,-0.0389144860878995,
-0.0107300558045623));
#19445=CARTESIAN_POINT('Ctrl Pts',(0.0064513003136744,-0.0389190904362821,
-0.0106985674348875));
#19446=CARTESIAN_POINT('Ctrl Pts',(0.00638179704600105,-0.038922483575283,
-0.0106790975315336));
#19447=CARTESIAN_POINT('Ctrl Pts',(0.0062520640856359,-0.0389286052075918,
-0.0106523849084008));
#19448=CARTESIAN_POINT('Ctrl Pts',(0.00619228260851654,-0.0389313482334985,
-0.0106436915670871));
#19449=CARTESIAN_POINT('Ctrl Pts',(0.00606794946760325,-0.038937108598694,
-0.0106330041327398));
#19450=CARTESIAN_POINT('Ctrl Pts',(0.0060034756409791,-0.0389401268100573,
-0.0106315129379326));
#19451=CARTESIAN_POINT('Ctrl Pts',(0.00592503700849566,-0.038944024268265,
-0.0106346110166826));
#19452=CARTESIAN_POINT('Ctrl Pts',(0.00591097889688837,-0.0389447317114968,
-0.010635359079631));
#19453=CARTESIAN_POINT('Ctrl Pts',(0.00588840061015893,-0.0389458850020985,
-0.0106368705991773));
#19454=CARTESIAN_POINT('Ctrl Pts',(0.00587987285156877,-0.0389463245241815,
-0.0106375127529518));
#19455=CARTESIAN_POINT('Ctrl Pts',(0.00586295445886242,-0.0389472050622727,
-0.0106389282668313));
#19456=CARTESIAN_POINT('Ctrl Pts',(0.0058545639783542,-0.0389476459604111,
-0.010639699533745));
#19457=CARTESIAN_POINT('Ctrl Pts',(0.00583276589652524,-0.0389488015840366,
-0.0106418834329746));
#19458=CARTESIAN_POINT('Ctrl Pts',(0.00581936994960617,-0.0389495218091572,
-0.0106434031184022));
#19459=CARTESIAN_POINT('Ctrl Pts',(0.00575274247265542,-0.038953148285221,
-0.0106518473104672));
#19460=CARTESIAN_POINT('Ctrl Pts',(0.00569988123357391,-0.0389561655704196,
-0.0106613704280882));
#19461=CARTESIAN_POINT('Ctrl Pts',(0.00557050287408348,-0.0389637370750815,
-0.010691718242654));
#19462=CARTESIAN_POINT('Ctrl Pts',(0.00549488185313838,-0.0389683233525499,
-0.010715722821767));
#19463=CARTESIAN_POINT('Ctrl Pts',(0.00536096561215517,-0.0389764913960077,
-0.0107698876742696));
#19464=CARTESIAN_POINT('Ctrl Pts',(0.00530209980568882,-0.0389801009721952,
-0.0107981591621908));
#19465=CARTESIAN_POINT('Ctrl Pts',(0.00522648360428544,-0.0389847333876129,
-0.0108405699293108));
#19466=CARTESIAN_POINT('Ctrl Pts',(0.00520799244010336,-0.0389858662553892,
-0.010851454047159));
#19467=CARTESIAN_POINT('Ctrl Pts',(0.00517853376536709,-0.0389876718274265,
-0.0108696314746269));
#19468=CARTESIAN_POINT('Ctrl Pts',(0.00516742256588606,-0.038988353046932,
-0.0108766854655964));
#19469=CARTESIAN_POINT('Ctrl Pts',(0.00514428430888205,-0.0389897724943307,
-0.0108917936601608));
#19470=CARTESIAN_POINT('Ctrl Pts',(0.00513227755707597,-0.0389905095610062,
-0.0108998767003045));
#19471=CARTESIAN_POINT('Ctrl Pts',(0.00510342650426437,-0.0389922828515013,
-0.0109198950610698));
#19472=CARTESIAN_POINT('Ctrl Pts',(0.00508670435504932,-0.0389933124888055,
-0.0109320019237646));
#19473=CARTESIAN_POINT('Ctrl Pts',(0.00502138082295572,-0.0389973484134285,
-0.0109813240610443));
#19474=CARTESIAN_POINT('Ctrl Pts',(0.00497476735735055,-0.0390002565183952,
-0.0110210829587258));
#19475=CARTESIAN_POINT('Ctrl Pts',(0.00488459170877782,-0.0390060806618378,
-0.0111077742178553));
#19476=CARTESIAN_POINT('Ctrl Pts',(0.00484133941089523,-0.0390089860105933,
-0.0111548565688351));
#19477=CARTESIAN_POINT('Ctrl Pts',(0.00475842328701149,-0.0390150419102517,
-0.0112571921418074));
#19478=CARTESIAN_POINT('Ctrl Pts',(0.00471924262128473,-0.0390181905573429,
-0.0113126556948978));
#19479=CARTESIAN_POINT('Ctrl Pts',(0.00467487551045286,-0.0390223694568305,
-0.0113851642352669));
#19480=CARTESIAN_POINT('Ctrl Pts',(0.0046661553351829,-0.0390232256846494,
-0.0113999651156102));
#19481=CARTESIAN_POINT('Ctrl Pts',(0.00465309842247589,-0.039024567756405,
-0.0114229976459652));
#19482=CARTESIAN_POINT('Ctrl Pts',(0.00464858576922245,-0.0390250433452285,
-0.0114311284759502));
#19483=CARTESIAN_POINT('Ctrl Pts',(0.00464030643252561,-0.0390259390929451,
-0.0114463691307259));
#19484=CARTESIAN_POINT('Ctrl Pts',(0.0046365214503827,-0.0390263581373064,
-0.0114534683714704));
#19485=CARTESIAN_POINT('Ctrl Pts',(0.00462751933855483,-0.0390273778066005,
-0.0114706758439578));
#19486=CARTESIAN_POINT('Ctrl Pts',(0.00462235821297537,-0.039027981696368,
-0.0114808126523283));
#19487=CARTESIAN_POINT('Ctrl Pts',(0.00460383053979049,-0.0390302193007762,
-0.0115182195407626));
#19488=CARTESIAN_POINT('Ctrl Pts',(0.00459115845480351,-0.0390318881039376,
-0.0115458242508556));
#19489=CARTESIAN_POINT('Ctrl Pts',(0.00455884783413799,-0.0390365098941275,
-0.0116220668213418));
#19490=CARTESIAN_POINT('Ctrl Pts',(0.00454086135863688,-0.0390395107402695,
-0.011671360465195));
#19491=CARTESIAN_POINT('Ctrl Pts',(0.00449211747054077,-0.0390490085595601,
-0.0118295464053845));
#19492=CARTESIAN_POINT('Ctrl Pts',(0.00447079264704203,-0.039055476574419,
-0.011940970585443));
#19493=CARTESIAN_POINT('Ctrl Pts',(0.00445988021919386,-0.0390628973623372,
-0.0120784200213759));
#19494=CARTESIAN_POINT('Ctrl Pts',(0.00445851487053123,-0.0390642125355577,
-0.0121031492952596));
#19495=CARTESIAN_POINT('Ctrl Pts',(0.0044572708178302,-0.039066308995255,
-0.0121431614622513));
#19496=CARTESIAN_POINT('Ctrl Pts',(0.00445702285893838,-0.0390671015028244,
-0.0121584277511109));
#19497=CARTESIAN_POINT('Ctrl Pts',(0.00445700050288177,-0.0390679240239845,
-0.0121744148175062));
#19498=CARTESIAN_POINT('Ctrl Pts',(0.004457,-0.0390679610123587,-0.01217513405244));
#19499=CARTESIAN_POINT('Ctrl Pts',(0.004457,-0.0390679979850714,-0.0121758532865546));
#19500=CARTESIAN_POINT('Ctrl Pts',(0.004457,-0.0391830969983919,-0.012175853298912));
#19501=CARTESIAN_POINT('Ctrl Pts',(0.00445699999984581,-0.0391820009249089,
-0.0121565951193162));
#19502=CARTESIAN_POINT('Ctrl Pts',(0.00445736054188219,-0.0391809001479444,
-0.0121373347547961));
#19503=CARTESIAN_POINT('Ctrl Pts',(0.00446239454806474,-0.0391732063147042,
-0.0120029760760998));
#19504=CARTESIAN_POINT('Ctrl Pts',(0.0044795837213134,-0.0391666246906011,
-0.0118886974964195));
#19505=CARTESIAN_POINT('Ctrl Pts',(0.0045156791125824,-0.0391591123637734,
-0.0117536643135762));
#19506=CARTESIAN_POINT('Ctrl Pts',(0.00452258626844821,-0.0391578095147989,
-0.0117300946277315));
#19507=CARTESIAN_POINT('Ctrl Pts',(0.00453477508548926,-0.0391557116223949,
-0.0116919048285094));
#19508=CARTESIAN_POINT('Ctrl Pts',(0.00453972000796917,-0.0391549060903489,
-0.0116771825254363));
#19509=CARTESIAN_POINT('Ctrl Pts',(0.00454981867969974,-0.0391533454327335,
-0.0116485555076253));
#19510=CARTESIAN_POINT('Ctrl Pts',(0.00455495225722688,-0.0391525897598165,
-0.0116346455168089));
#19511=CARTESIAN_POINT('Ctrl Pts',(0.00456776353850457,-0.0391507898485505,
-0.0116014145397136));
#19512=CARTESIAN_POINT('Ctrl Pts',(0.00457563287013562,-0.039149751968433,
-0.011582170302556));
#19513=CARTESIAN_POINT('Ctrl Pts',(0.00460741506568473,-0.0391458017171191,
-0.0115087208196458));
#19514=CARTESIAN_POINT('Ctrl Pts',(0.00463405400797084,-0.0391429786223235,
-0.0114557484994959));
#19515=CARTESIAN_POINT('Ctrl Pts',(0.00469533770478568,-0.0391372507995682,
-0.0113495868195775));
#19516=CARTESIAN_POINT('Ctrl Pts',(0.00473034776672741,-0.0391343594094087,
-0.0112967382120021));
#19517=CARTESIAN_POINT('Ctrl Pts',(0.00480979671359546,-0.0391282816728232,
-0.0111914947650657));
#19518=CARTESIAN_POINT('Ctrl Pts',(0.00485468212687263,-0.0391250968055734,
-0.0111396143930974));
#19519=CARTESIAN_POINT('Ctrl Pts',(0.0049152018054228,-0.0391208633551922,
-0.0110784154353194));
#19520=CARTESIAN_POINT('Ctrl Pts',(0.00492775274226097,-0.0391199882071065,
-0.0110661493929499));
#19521=CARTESIAN_POINT('Ctrl Pts',(0.00494736425702434,-0.0391186199671835,
-0.011047626406524));
#19522=CARTESIAN_POINT('Ctrl Pts',(0.00495427789611805,-0.0391181374782679,
-0.0110412153826375));
#19523=CARTESIAN_POINT('Ctrl Pts',(0.00496741595444978,-0.0391172193693551,
-0.0110292545223772));
#19524=CARTESIAN_POINT('Ctrl Pts',(0.00497362728416082,-0.0391167847188831,
-0.0110236911565518));
#19525=CARTESIAN_POINT('Ctrl Pts',(0.00498897441833383,-0.0391157098047501,
-0.0110101676093));
#19526=CARTESIAN_POINT('Ctrl Pts',(0.00499815938510211,-0.0391150657181805,
-0.0110022642657901));
#19527=CARTESIAN_POINT('Ctrl Pts',(0.00503415283220102,-0.0391125420106734,
-0.0109720236165643));
#19528=CARTESIAN_POINT('Ctrl Pts',(0.00506162160770138,-0.039110616811391,
-0.0109504911723559));
#19529=CARTESIAN_POINT('Ctrl Pts',(0.00514349392865255,-0.039104935298988,
-0.0108906805803855));
#19530=CARTESIAN_POINT('Ctrl Pts',(0.00519967173071391,-0.0391011087929687,
-0.0108549650247));
#19531=CARTESIAN_POINT('Ctrl Pts',(0.00533598222954914,-0.0390922196205954,
-0.0107802011851357));
#19532=CARTESIAN_POINT('Ctrl Pts',(0.00541754982499925,-0.0390871998052542,
-0.010744238977239));
#19533=CARTESIAN_POINT('Ctrl Pts',(0.00552648109427711,-0.0390809947467151,
-0.0107070746997244));
#19534=CARTESIAN_POINT('Ctrl Pts',(0.00555140264478281,-0.0390796061368119,
-0.0106992723668724));
#19535=CARTESIAN_POINT('Ctrl Pts',(0.0055917398879053,-0.0390774073063466,
-0.0106877593765357));
#19536=CARTESIAN_POINT('Ctrl Pts',(0.00560703490154429,-0.0390765846061403,
-0.0106836474495651));
#19537=CARTESIAN_POINT('Ctrl Pts',(0.00563662971341949,-0.0390750133015953,
-0.0106761777567649));
#19538=CARTESIAN_POINT('Ctrl Pts',(0.00565091941109882,-0.0390742637414912,
-0.0106727872795905));
#19539=CARTESIAN_POINT('Ctrl Pts',(0.00568467571391375,-0.0390725135560467,
-0.0106652853934554));
#19540=CARTESIAN_POINT('Ctrl Pts',(0.00570417792533073,-0.0390715183425913,
-0.0106613454094218));
#19541=CARTESIAN_POINT('Ctrl Pts',(0.00577398167263248,-0.0390680078261219,
-0.0106486429732906));
#19542=CARTESIAN_POINT('Ctrl Pts',(0.00582463675819904,-0.0390655565953935,
-0.0106420006414148));
#19543=CARTESIAN_POINT('Ctrl Pts',(0.00596830037744303,-0.0390587712443476,
-0.0106303738679852));
#19544=CARTESIAN_POINT('Ctrl Pts',(0.00606155604019374,-0.0390545708411053,
-0.0106312750022569));
#19545=CARTESIAN_POINT('Ctrl Pts',(0.00620951113169414,-0.0390476532338127,
-0.010646131558299));
#19546=CARTESIAN_POINT('Ctrl Pts',(0.00626451565654233,-0.0390450207102955,
-0.0106546780924168));
#19547=CARTESIAN_POINT('Ctrl Pts',(0.00633261484030529,-0.0390415605365138,
-0.0106690646844277));
#19548=CARTESIAN_POINT('Ctrl Pts',(0.00634625548939901,-0.0390408571363762,
-0.0106721406696479));
#19549=CARTESIAN_POINT('Ctrl Pts',(0.00636829965813915,-0.0390397009499894,
-0.0106774275028167));
#19550=CARTESIAN_POINT('Ctrl Pts',(0.0063767298984555,-0.0390392541495181,
-0.0106795247645937));
#19551=CARTESIAN_POINT('Ctrl Pts',(0.00639368003088043,-0.0390383456153133,
-0.010683893911116));
#19552=CARTESIAN_POINT('Ctrl Pts',(0.00640219901486224,-0.0390378837954673,
-0.0106861678533931));
#19553=CARTESIAN_POINT('Ctrl Pts',(0.00642477154092618,-0.0390366471595487,
-0.0106924007900493));
#19554=CARTESIAN_POINT('Ctrl Pts',(0.00643878889834325,-0.0390358658047163,
-0.0106964863798978));
#19555=CARTESIAN_POINT('Ctrl Pts',(0.00647015743340303,-0.0390340902693345,
-0.0107061142901487));
#19556=CARTESIAN_POINT('Ctrl Pts',(0.0064874726165753,-0.0390330914216456,
-0.0107117661541405));
#19557=CARTESIAN_POINT('Ctrl Pts',(0.00654348641183271,-0.0390298075669738,
-0.0107311534569095));
#19558=CARTESIAN_POINT('Ctrl Pts',(0.00658173657543491,-0.0390274828010913,
-0.0107461269699083));
#19559=CARTESIAN_POINT('Ctrl Pts',(0.00673682752679571,-0.0390178249452355,
-0.010814094167959));
#19560=CARTESIAN_POINT('Ctrl Pts',(0.00684745537657086,-0.0390104331868801,
-0.010880040212544));
#19561=CARTESIAN_POINT('Ctrl Pts',(0.00696833479990033,-0.039002188831304,
-0.0109742711152271));
#19562=CARTESIAN_POINT('Ctrl Pts',(0.00698764556277352,-0.0390008637178099,
-0.0109900926292969));
#19563=CARTESIAN_POINT('Ctrl Pts',(0.00701839517662821,-0.0389987396081037,
-0.0110165587146165));
#19564=CARTESIAN_POINT('Ctrl Pts',(0.00703007067967821,-0.0389979296181438,
-0.0110269202778433));
#19565=CARTESIAN_POINT('Ctrl Pts',(0.00705249455834346,-0.0389963664630501,
-0.0110474372418153));
#19566=CARTESIAN_POINT('Ctrl Pts',(0.00706325811453892,-0.0389956126402495,
-0.0110575734617343));
#19567=CARTESIAN_POINT('Ctrl Pts',(0.00708861841509724,-0.0389938270572344,
-0.0110821529038121));
#19568=CARTESIAN_POINT('Ctrl Pts',(0.00710307594744084,-0.0389928013815913,
-0.0110967360158397));
#19569=CARTESIAN_POINT('Ctrl Pts',(0.00715635362440578,-0.0389889860809594,
-0.0111526663914811));
#19570=CARTESIAN_POINT('Ctrl Pts',(0.00719317687776992,-0.0389862774906632,
-0.011195855932776));
#19571=CARTESIAN_POINT('Ctrl Pts',(0.00730154224009851,-0.0389779022255479,
-0.0113381453884242));
#19572=CARTESIAN_POINT('Ctrl Pts',(0.00736373765625368,-0.0389724850345071,
-0.0114437455928714));
#19573=CARTESIAN_POINT('Ctrl Pts',(0.00742305242963822,-0.0389653653146683,
-0.0115788462389623));
#19574=CARTESIAN_POINT('Ctrl Pts',(0.00743269731929412,-0.0389641173885052,
-0.0116023780062819));
#19575=CARTESIAN_POINT('Ctrl Pts',(0.00744536166511449,-0.0389623313679788,
-0.011635593078288));
#19576=CARTESIAN_POINT('Ctrl Pts',(0.00744887421934554,-0.0389618182098895,
-0.01164508504897));
#19577=CARTESIAN_POINT('Ctrl Pts',(0.00745510551182062,-0.0389608734327401,
-0.0116624467576147));
#19578=CARTESIAN_POINT('Ctrl Pts',(0.00745785444588624,-0.0389604434820309,
-0.0116703053383802));
#19579=CARTESIAN_POINT('Ctrl Pts',(0.00746359357554317,-0.0389595165110634,
-0.0116871483671832));
#19580=CARTESIAN_POINT('Ctrl Pts',(0.00746656483844161,-0.0389590185391279,
-0.011696138560573));
#19581=CARTESIAN_POINT('Ctrl Pts',(0.00747486694332621,-0.0389575749548826,
-0.0117220565677848));
#19582=CARTESIAN_POINT('Ctrl Pts',(0.00747998858189135,-0.0389566187838916,
-0.0117390493152656));
#19583=CARTESIAN_POINT('Ctrl Pts',(0.00750327774456135,-0.0389519488289575,
-0.0118214364027258));
#19584=CARTESIAN_POINT('Ctrl Pts',(0.00751740934664829,-0.038948082386374,
-0.0118878897704586));
#19585=CARTESIAN_POINT('Ctrl Pts',(0.00754354090173187,-0.0389376322812079,
-0.0120686228102988));
#19586=CARTESIAN_POINT('Ctrl Pts',(0.00754724351227303,-0.0389310766950217,
-0.0121836874928687));
#19587=CARTESIAN_POINT('Ctrl Pts',(0.00753619894531687,-0.0389235838767184,
-0.012322644342529));
#19588=CARTESIAN_POINT('Ctrl Pts',(0.00753366191799773,-0.0389222778987208,
-0.0123471309149035));
#19589=CARTESIAN_POINT('Ctrl Pts',(0.00752856910022536,-0.0389201763215992,
-0.0123869622947014));
#19590=CARTESIAN_POINT('Ctrl Pts',(0.00752636533178967,-0.0389193701633615,
-0.0124023470048303));
#19591=CARTESIAN_POINT('Ctrl Pts',(0.00752160667643864,-0.0389178091678657,
-0.0124323328155212));
#19592=CARTESIAN_POINT('Ctrl Pts',(0.00751907309202278,-0.0389170537675525,
-0.0124469355381817));
#19593=CARTESIAN_POINT('Ctrl Pts',(0.00751248791027667,-0.0389152559380051,
-0.012481892394416));
#19594=CARTESIAN_POINT('Ctrl Pts',(0.00750823526394893,-0.0389142198271718,
-0.0125022059381731));
#19595=CARTESIAN_POINT('Ctrl Pts',(0.00749035269647383,-0.0389102896839533,
-0.0125797873426293));
#19596=CARTESIAN_POINT('Ctrl Pts',(0.00747385930766225,-0.0389074836670514,
-0.0126363458925351));
#19597=CARTESIAN_POINT('Ctrl Pts',(0.00743276285457901,-0.038901739260366,
-0.0127521683776472));
#19598=CARTESIAN_POINT('Ctrl Pts',(0.00740761702544376,-0.0388988166066109,
-0.012811119312464));
#19599=CARTESIAN_POINT('Ctrl Pts',(0.007348218068312,-0.0388927159273206,
-0.012929395166544));
#19600=CARTESIAN_POINT('Ctrl Pts',(0.007313534998016,-0.0388895400290671,
-0.0129883443063694));
#19601=CARTESIAN_POINT('Ctrl Pts',(0.00726518862711358,-0.0388853172345711,
-0.0130592864904039));
#19602=CARTESIAN_POINT('Ctrl Pts',(0.00725506765641552,-0.038884442732458,
-0.0130736069380024));
#19603=CARTESIAN_POINT('Ctrl Pts',(0.00723913457509837,-0.0388830752889832,
-0.0130953549743917));
#19604=CARTESIAN_POINT('Ctrl Pts',(0.00723349448880731,-0.0388825929311686,
-0.0131029073230419));
#19605=CARTESIAN_POINT('Ctrl Pts',(0.00722273449711926,-0.0388816749024833,
-0.0131170434384656));
#19606=CARTESIAN_POINT('Ctrl Pts',(0.00721762985832142,-0.0388812401977442,
-0.0131236381087119));
#19607=CARTESIAN_POINT('Ctrl Pts',(0.00720497409479823,-0.0388801649079939,
-0.0131397170734844));
#19608=CARTESIAN_POINT('Ctrl Pts',(0.00719736425044089,-0.0388795204938058,
-0.0131491542692982));
#19609=CARTESIAN_POINT('Ctrl Pts',(0.00716738886979466,-0.0388769936245578,
-0.0131854440355372));
#19610=CARTESIAN_POINT('Ctrl Pts',(0.00714422592846327,-0.0388750654521368,
-0.0132116220683606));
#19611=CARTESIAN_POINT('Ctrl Pts',(0.007074335281738,-0.0388693703992489,
-0.0132854026263385));
#19612=CARTESIAN_POINT('Ctrl Pts',(0.00702538550427146,-0.0388655330027893,
-0.0133307906047031));
#19613=CARTESIAN_POINT('Ctrl Pts',(0.00690482984174703,-0.0388566480701473,
-0.0134288508195308));
#19614=CARTESIAN_POINT('Ctrl Pts',(0.00683129821697608,-0.0388516430724164,
-0.0134787985877224));
#19615=CARTESIAN_POINT('Ctrl Pts',(0.00673109230686452,-0.0388454514894299,
-0.0135349098569407));
#19616=CARTESIAN_POINT('Ctrl Pts',(0.00670798999677249,-0.0388440628462404,
-0.01354708667129));
#19617=CARTESIAN_POINT('Ctrl Pts',(0.00667039596381569,-0.0388418639766302,
-0.0135656982634023));
#19618=CARTESIAN_POINT('Ctrl Pts',(0.00665609544373935,-0.038841041269769,
-0.0135725059280733));
#19619=CARTESIAN_POINT('Ctrl Pts',(0.00662833713298731,-0.0388394699606003,
-0.0135851996264756));
#19620=CARTESIAN_POINT('Ctrl Pts',(0.0066148951886901,-0.038838720402377,
-0.0135911160128652));
#19621=CARTESIAN_POINT('Ctrl Pts',(0.00658305007562943,-0.0388369702336013,
-0.0136045930677316));
#19622=CARTESIAN_POINT('Ctrl Pts',(0.00656458091916511,-0.0388359750346175,
-0.0136119915749597));
#19623=CARTESIAN_POINT('Ctrl Pts',(0.00649822346896417,-0.0388324646538866,
-0.0136370954789874));
#19624=CARTESIAN_POINT('Ctrl Pts',(0.00644960447931477,-0.03883001353738,
-0.0136527797439021));
#19625=CARTESIAN_POINT('Ctrl Pts',(0.00631041788138256,-0.0388232287561061,
-0.0136901684397178));
#19626=CARTESIAN_POINT('Ctrl Pts',(0.0062185441687861,-0.0388190287757899,
-0.0137061303249693));
#19627=CARTESIAN_POINT('Ctrl Pts',(0.00607033792702761,-0.0388121111309378,
-0.0137182531696658));
#19628=CARTESIAN_POINT('Ctrl Pts',(0.00601468239509338,-0.0388094780685831,
-0.0137197860162273));
#19629=CARTESIAN_POINT('Ctrl Pts',(0.00594509199167016,-0.0388060172726381,
-0.0137179394224214));
#19630=CARTESIAN_POINT('Ctrl Pts',(0.00593111949503579,-0.0388053138443167,
-0.0137173785022215));
#19631=CARTESIAN_POINT('Ctrl Pts',(0.00590848221466177,-0.0388041576232975,
-0.0137161613611453));
#19632=CARTESIAN_POINT('Ctrl Pts',(0.0058998116710167,-0.038803710817056,
-0.0137156216986488));
#19633=CARTESIAN_POINT('Ctrl Pts',(0.00588235111475376,-0.0388028022844552,
-0.0137143868357823));
#19634=CARTESIAN_POINT('Ctrl Pts',(0.00587356162318101,-0.0388023404721878,
-0.0137136894520232));
#19635=CARTESIAN_POINT('Ctrl Pts',(0.00585023522484449,-0.0388011038786524,
-0.013711637341939));
#19636=CARTESIAN_POINT('Ctrl Pts',(0.0058357110336972,-0.0388003225593684,
-0.0137101515817557));
#19637=CARTESIAN_POINT('Ctrl Pts',(0.00573970412338155,-0.0387950923078076,
-0.0136989516994517));
#19638=CARTESIAN_POINT('Ctrl Pts',(0.00565909161361419,-0.0387903940043232,
-0.0136829572343369));
#19639=CARTESIAN_POINT('Ctrl Pts',(0.0054801130964723,-0.038779744484197,
-0.0136323463305039));
#19640=CARTESIAN_POINT('Ctrl Pts',(0.00538318823585556,-0.0387738334990884,
-0.0135940221098944));
#19641=CARTESIAN_POINT('Ctrl Pts',(0.00526798340782734,-0.038766845214362,
-0.0135344052300495));
#19642=CARTESIAN_POINT('Ctrl Pts',(0.00524541961612259,-0.0387654768773862,
-0.0135220034351331));
#19643=CARTESIAN_POINT('Ctrl Pts',(0.00520955526020677,-0.038763301891781,
-0.01350110594858));
#19644=CARTESIAN_POINT('Ctrl Pts',(0.00519605686572185,-0.0387624832452657,
-0.0134929610899507));
#19645=CARTESIAN_POINT('Ctrl Pts',(0.00517020526310192,-0.0387609146882033,
-0.0134768168483107));
#19646=CARTESIAN_POINT('Ctrl Pts',(0.00515783706482843,-0.0387601639146379,
-0.0134688448194509));
#19647=CARTESIAN_POINT('Ctrl Pts',(0.00512886033229832,-0.0387584032223533,
-0.0134495754168176));
#19648=CARTESIAN_POINT('Ctrl Pts',(0.0051123544587214,-0.0387573989148847,
-0.013438128147564));
#19649=CARTESIAN_POINT('Ctrl Pts',(0.00505340021225542,-0.0387538015648954,
-0.0133955133621236));
#19650=CARTESIAN_POINT('Ctrl Pts',(0.00501232938196228,-0.0387512771926606,
-0.0133624994987274));
#19651=CARTESIAN_POINT('Ctrl Pts',(0.00489850939520006,-0.0387441091084849,
-0.0132609964800816));
#19652=CARTESIAN_POINT('Ctrl Pts',(0.00483062288114043,-0.0387396223224157,
-0.0131874725798259));
#19653=CARTESIAN_POINT('Ctrl Pts',(0.00474158622180993,-0.0387327198280213,
-0.0130700042031375));
#19654=CARTESIAN_POINT('Ctrl Pts',(0.00471462638576875,-0.0387304503182971,
-0.013030794873091));
#19655=CARTESIAN_POINT('Ctrl Pts',(0.00468234447346436,-0.038727406255314,
-0.0129788587550929));
#19656=CARTESIAN_POINT('Ctrl Pts',(0.00467531994155035,-0.0387267215442087,
-0.0129672170388318));
#19657=CARTESIAN_POINT('Ctrl Pts',(0.00466453016997498,-0.0387256316026228,
-0.0129487889438324));
#19658=CARTESIAN_POINT('Ctrl Pts',(0.00466066057851887,-0.0387252326084171,
-0.0129420641624215));
#19659=CARTESIAN_POINT('Ctrl Pts',(0.00465257933629285,-0.0387243813782083,
-0.0129277718710238));
#19660=CARTESIAN_POINT('Ctrl Pts',(0.00464838039864991,-0.0387239283397429,
-0.0129201975932387));
#19661=CARTESIAN_POINT('Ctrl Pts',(0.00463763121422183,-0.038722741016591,
-0.0129004167381425));
#19662=CARTESIAN_POINT('Ctrl Pts',(0.00463118129430683,-0.0387220010383642,
-0.0128881567536514));
#19663=CARTESIAN_POINT('Ctrl Pts',(0.00459919978925148,-0.0387181945419569,
-0.0128253275540626));
#19664=CARTESIAN_POINT('Ctrl Pts',(0.00457630357197659,-0.0387150074745462,
-0.0127734698490567));
#19665=CARTESIAN_POINT('Ctrl Pts',(0.00451092713517522,-0.0387044596490242,
-0.0126001695449571));
#19666=CARTESIAN_POINT('Ctrl Pts',(0.0044807509164299,-0.0386970296432644,
-0.0124746401513882));
#19667=CARTESIAN_POINT('Ctrl Pts',(0.00446351390023315,-0.0386886291404036,
-0.0123200267575324));
#19668=CARTESIAN_POINT('Ctrl Pts',(0.00446122975971187,-0.0386871937913481,
-0.0122931639468433));
#19669=CARTESIAN_POINT('Ctrl Pts',(0.0044587128045693,-0.03868494004789,
-0.0122502771849483));
#19670=CARTESIAN_POINT('Ctrl Pts',(0.00445802375967009,-0.0386841080366129,
-0.0122342864525433));
#19671=CARTESIAN_POINT('Ctrl Pts',(0.0044571945605513,-0.0386825548500941,
-0.0122041463698509));
#19672=CARTESIAN_POINT('Ctrl Pts',(0.004457,-0.0386818320975096,-0.0121900003094259));
#19673=CARTESIAN_POINT('Ctrl Pts',(0.004457,-0.0386811151660051,-0.0121758532865598));
#19674=CARTESIAN_POINT('Origin',(0.006,-0.0418165664398416,-0.0121758532865581));
#19675=CARTESIAN_POINT('',(0.004457,-0.0396826982119552,-0.0121758532865581));
#19676=CARTESIAN_POINT('',(0.004457,-0.0395660360928446,-0.01217585328639));
#19677=CARTESIAN_POINT('',(0.004457,-0.0418165664398416,-0.0121758532865581));
#19678=CARTESIAN_POINT('Ctrl Pts',(0.004457,-0.0390679979850714,-0.0121758532865546));
#19679=CARTESIAN_POINT('Ctrl Pts',(0.00445699999999997,-0.0390686953839983,
-0.0121894198620967));
#19680=CARTESIAN_POINT('Ctrl Pts',(0.00445717892260015,-0.0390693872025768,
-0.0122029861465897));
#19681=CARTESIAN_POINT('Ctrl Pts',(0.00445805141405487,-0.0390710608261081,
-0.0122360559263837));
#19682=CARTESIAN_POINT('Ctrl Pts',(0.00445893610664614,-0.0390720366435178,
-0.0122555522144478));
#19683=CARTESIAN_POINT('Ctrl Pts',(0.00446344280615422,-0.039075504519834,
-0.0123255249457911));
#19684=CARTESIAN_POINT('Ctrl Pts',(0.00446917744010499,-0.0390779322546964,
-0.0123758344947069));
#19685=CARTESIAN_POINT('Ctrl Pts',(0.0044921969495062,-0.0390846143045803,
-0.0125160790739161));
#19686=CARTESIAN_POINT('Ctrl Pts',(0.00451502314309146,-0.0390887366631945,
-0.01260488387904));
#19687=CARTESIAN_POINT('Ctrl Pts',(0.00456549555276677,-0.0390957327627902,
-0.0127473434511737));
#19688=CARTESIAN_POINT('Ctrl Pts',(0.00458864638692,-0.0390985389073823,
-0.012802338565902));
#19689=CARTESIAN_POINT('Ctrl Pts',(0.00462106947919116,-0.0391021931685658,
-0.0128683808641343));
#19690=CARTESIAN_POINT('Ctrl Pts',(0.00462739029966787,-0.039102894822758,
-0.012880825918588));
#19691=CARTESIAN_POINT('Ctrl Pts',(0.00463784278334832,-0.0391040409642443,
-0.0129007321857558));
#19692=CARTESIAN_POINT('Ctrl Pts',(0.0046418691121806,-0.0391044792670903,
-0.01290824811603));
#19693=CARTESIAN_POINT('Ctrl Pts',(0.00465000883326701,-0.0391053598462119,
-0.0129231445533832));
#19694=CARTESIAN_POINT('Ctrl Pts',(0.00465412096044917,-0.0391058020444971,
-0.012930525394924));
#19695=CARTESIAN_POINT('Ctrl Pts',(0.00466500614659929,-0.0391069649779339,
-0.0129496912342172));
#19696=CARTESIAN_POINT('Ctrl Pts',(0.00467187457148897,-0.039107691334684,
-0.0129614209662401));
#19697=CARTESIAN_POINT('Ctrl Pts',(0.00470766636437324,-0.0391114333005876,
-0.0130207340245329));
#19698=CARTESIAN_POINT('Ctrl Pts',(0.00473899350325883,-0.0391145683035145,
-0.0130668141885997));
#19699=CARTESIAN_POINT('Ctrl Pts',(0.00484628643827727,-0.0391246644465148,
-0.0132076079219752));
#19700=CARTESIAN_POINT('Ctrl Pts',(0.00493097347345358,-0.0391317042723518,
-0.0132951217200965));
#19701=CARTESIAN_POINT('Ctrl Pts',(0.0050502642277241,-0.0391401067469135,
-0.0133923686507829));
#19702=CARTESIAN_POINT('Ctrl Pts',(0.00507612840976471,-0.0391418545591673,
-0.0134121255718104));
#19703=CARTESIAN_POINT('Ctrl Pts',(0.00511640525508696,-0.0391444664314168,
-0.0134409214099597));
#19704=CARTESIAN_POINT('Ctrl Pts',(0.00513037342017816,-0.039145353095776,
-0.0134505637134271));
#19705=CARTESIAN_POINT('Ctrl Pts',(0.00515617717978486,-0.0391469571070247,
-0.0134677545931989));
#19706=CARTESIAN_POINT('Ctrl Pts',(0.00516796199648746,-0.0391476771148746,
-0.0134753757818517));
#19707=CARTESIAN_POINT('Ctrl Pts',(0.00519406191203945,-0.0391492450861839,
-0.013491753865759));
#19708=CARTESIAN_POINT('Ctrl Pts',(0.00520841927653804,-0.0391500904185747,
-0.0135004402116778));
#19709=CARTESIAN_POINT('Ctrl Pts',(0.00525104340789119,-0.0391525521840638,
-0.0135252876261503));
#19710=CARTESIAN_POINT('Ctrl Pts',(0.00527968393099445,-0.0391541454467515,
-0.013540790631052));
#19711=CARTESIAN_POINT('Ctrl Pts',(0.00540259418865835,-0.0391607636270299,
-0.0136023743733456));
#19712=CARTESIAN_POINT('Ctrl Pts',(0.00550094045792831,-0.039165506874211,
-0.0136396827169335));
#19713=CARTESIAN_POINT('Ctrl Pts',(0.00566610370748841,-0.0391733719121199,
-0.0136837394866635));
#19714=CARTESIAN_POINT('Ctrl Pts',(0.0057309138947385,-0.0391764413992063,
-0.0136966421615009));
#19715=CARTESIAN_POINT('Ctrl Pts',(0.00581328573465872,-0.0391805275612473,
-0.0137076100751104));
#19716=CARTESIAN_POINT('Ctrl Pts',(0.00583026212705443,-0.0391813795744156,
-0.0137095840602991));
#19717=CARTESIAN_POINT('Ctrl Pts',(0.00585650219428668,-0.0391827164068374,
-0.0137121942349939));
#19718=CARTESIAN_POINT('Ctrl Pts',(0.00586574512224587,-0.0391831910956868,
-0.0137130295124682));
#19719=CARTESIAN_POINT('Ctrl Pts',(0.00588301870259816,-0.0391840862117972,
-0.0137144335361712));
#19720=CARTESIAN_POINT('Ctrl Pts',(0.00589104711586184,-0.0391845055466841,
-0.0137150228896817));
#19721=CARTESIAN_POINT('Ctrl Pts',(0.00591046549139351,-0.039185527414881,
-0.013716295679848));
#19722=CARTESIAN_POINT('Ctrl Pts',(0.00592185897528475,-0.0391861332496683,
-0.0137169156345494));
#19723=CARTESIAN_POINT('Ctrl Pts',(0.00596386839259034,-0.0391883875097967,
-0.0137187344429197));
#19724=CARTESIAN_POINT('Ctrl Pts',(0.00599450976258318,-0.0391900716738004,
-0.0137191476162022));
#19725=CARTESIAN_POINT('Ctrl Pts',(0.00607834829761232,-0.0391947533433757,
-0.0137177813968699));
#19726=CARTESIAN_POINT('Ctrl Pts',(0.00613147297031129,-0.0391978000109013,
-0.0137141624793291));
#19727=CARTESIAN_POINT('Ctrl Pts',(0.00629514240293824,-0.0392072599555462,
-0.0136944721791082));
#19728=CARTESIAN_POINT('Ctrl Pts',(0.00640422403476766,-0.0392136410940809,
-0.0136691455820318));
#19729=CARTESIAN_POINT('Ctrl Pts',(0.00653315678161299,-0.0392209952714821,
-0.0136240294924092));
#19730=CARTESIAN_POINT('Ctrl Pts',(0.00655648506677964,-0.0392223196634337,
-0.0136152263944231));
#19731=CARTESIAN_POINT('Ctrl Pts',(0.00659377084486842,-0.03922442698959,
-0.013600114249361));
#19732=CARTESIAN_POINT('Ctrl Pts',(0.00660786499297001,-0.0392252213587277,
-0.0135941562439969));
#19733=CARTESIAN_POINT('Ctrl Pts',(0.00663493016591397,-0.039226743095013,
-0.0135822374360965));
#19734=CARTESIAN_POINT('Ctrl Pts',(0.00664791162856453,-0.0392274713011273,
-0.0135763043678148));
#19735=CARTESIAN_POINT('Ctrl Pts',(0.00667836150793591,-0.0392291763118657,
-0.0135618734684553));
#19736=CARTESIAN_POINT('Ctrl Pts',(0.00669575563740352,-0.0392301478151441,
-0.0135532241209742));
#19737=CARTESIAN_POINT('Ctrl Pts',(0.0067572058870162,-0.0392335756898309,
-0.0135212063640623));
#19738=CARTESIAN_POINT('Ctrl Pts',(0.00680028839480739,-0.039235969814639,
-0.0134960330851471));
#19739=CARTESIAN_POINT('Ctrl Pts',(0.00690362017739876,-0.0392417721421321,
-0.0134287353106675));
#19740=CARTESIAN_POINT('Ctrl Pts',(0.00696222276467297,-0.0392451144893761,
-0.0133843111824927));
#19741=CARTESIAN_POINT('Ctrl Pts',(0.0070759684016399,-0.0392520614055408,
-0.0132845471335246));
#19742=CARTESIAN_POINT('Ctrl Pts',(0.00713052367811452,-0.0392556611642383,
-0.0132288603807474));
#19743=CARTESIAN_POINT('Ctrl Pts',(0.00718989359644846,-0.0392602349526987,
-0.0131583037140563));
#19744=CARTESIAN_POINT('Ctrl Pts',(0.00719899377424118,-0.0392609567091442,
-0.013147176875781));
#19745=CARTESIAN_POINT('Ctrl Pts',(0.0072132971267044,-0.0392621276847253,
-0.0131291807738793));
#19746=CARTESIAN_POINT('Ctrl Pts',(0.00721860068672292,-0.039262570225207,
-0.0131223920206809));
#19747=CARTESIAN_POINT('Ctrl Pts',(0.00722894616682311,-0.0392634508920071,
-0.0131089183559192));
#19748=CARTESIAN_POINT('Ctrl Pts',(0.00723399103190644,-0.0392638888043464,
-0.0131022361603833));
#19749=CARTESIAN_POINT('Ctrl Pts',(0.00724686308213792,-0.039265027487708,
-0.0130848947251949));
#19750=CARTESIAN_POINT('Ctrl Pts',(0.00725460796428767,-0.0392657334772657,
-0.0130741754536445));
#19751=CARTESIAN_POINT('Ctrl Pts',(0.00729071708465322,-0.0392691206022097,
-0.0130228208919799));
#19752=CARTESIAN_POINT('Ctrl Pts',(0.00731724885600675,-0.0392718964700562,
-0.0129809367734704));
#19753=CARTESIAN_POINT('Ctrl Pts',(0.00738083568070027,-0.0392792146620341,
-0.0128689739860248));
#19754=CARTESIAN_POINT('Ctrl Pts',(0.00741459209835948,-0.0392838036149811,
-0.012797185069273));
#19755=CARTESIAN_POINT('Ctrl Pts',(0.00746725863704162,-0.0392922220190079,
-0.0126583471720437));
#19756=CARTESIAN_POINT('Ctrl Pts',(0.00748744147699956,-0.039296066079905,
-0.0125919877843493));
#19757=CARTESIAN_POINT('Ctrl Pts',(0.00750800701896821,-0.0393009325778648,
-0.0125033223703571));
#19758=CARTESIAN_POINT('Ctrl Pts',(0.00751246920050807,-0.0393020806166226,
-0.0124820528157463));
#19759=CARTESIAN_POINT('Ctrl Pts',(0.00751891884626964,-0.0393039036996923,
-0.0124477153174316));
#19760=CARTESIAN_POINT('Ctrl Pts',(0.00752119019596254,-0.0393045875751073,
-0.0124347042619441));
#19761=CARTESIAN_POINT('Ctrl Pts',(0.00752559311442695,-0.0393060076883288,
-0.0124074194340762));
#19762=CARTESIAN_POINT('Ctrl Pts',(0.00752769205533074,-0.0393067428392544,
-0.012393141652205));
#19763=CARTESIAN_POINT('Ctrl Pts',(0.00753227361886957,-0.0393085022334846,
-0.0123586169939624));
#19764=CARTESIAN_POINT('Ctrl Pts',(0.00753455569284665,-0.0393095201540773,
-0.0123383460251102));
#19765=CARTESIAN_POINT('Ctrl Pts',(0.00754183775557845,-0.039313419275789,
-0.0122596551296015));
#19766=CARTESIAN_POINT('Ctrl Pts',(0.00754390877309404,-0.0393162112225813,
-0.0122010116419741));
#19767=CARTESIAN_POINT('Ctrl Pts',(0.00754005020850498,-0.0393245126117885,
-0.0120231399901397));
#19768=CARTESIAN_POINT('Ctrl Pts',(0.00752364561879022,-0.0393297938282777,
-0.0119046046787139));
#19769=CARTESIAN_POINT('Ctrl Pts',(0.00748685726419432,-0.0393368438622562,
-0.0117624981352158));
#19770=CARTESIAN_POINT('Ctrl Pts',(0.00747924553250601,-0.0393381902075373,
-0.0117360357114069));
#19771=CARTESIAN_POINT('Ctrl Pts',(0.00746753392973297,-0.0393401360248672,
-0.011699072819514));
#19772=CARTESIAN_POINT('Ctrl Pts',(0.0074640204258473,-0.0393407061469304,
-0.0116883908498046));
#19773=CARTESIAN_POINT('Ctrl Pts',(0.00745779889211259,-0.0393416946057261,
-0.0116701499691105));
#19774=CARTESIAN_POINT('Ctrl Pts',(0.00745514809726178,-0.0393421097224252,
-0.0116625722051338));
#19775=CARTESIAN_POINT('Ctrl Pts',(0.0074492751930599,-0.039343017061454,
-0.0116461946996333));
#19776=CARTESIAN_POINT('Ctrl Pts',(0.00744603202849368,-0.0393435104001268,
-0.0116374035045648));
#19777=CARTESIAN_POINT('Ctrl Pts',(0.00743630988549436,-0.0393449661224141,
-0.0116117712851429));
#19778=CARTESIAN_POINT('Ctrl Pts',(0.00742961549899903,-0.0393459398116313,
-0.0115950141844532));
#19779=CARTESIAN_POINT('Ctrl Pts',(0.00741320349817015,-0.0393482560793902,
-0.011555936030971));
#19780=CARTESIAN_POINT('Ctrl Pts',(0.00740324851413722,-0.0393496084347588,
-0.011533720091317));
#19781=CARTESIAN_POINT('Ctrl Pts',(0.00736298331225454,-0.0393548626703705,
-0.0114492749982722));
#19782=CARTESIAN_POINT('Ctrl Pts',(0.00732902487033237,-0.0393588589112449,
-0.0113888767813469));
#19783=CARTESIAN_POINT('Ctrl Pts',(0.0072432381655167,-0.0393678336274405,
-0.0112577808526611));
#19784=CARTESIAN_POINT('Ctrl Pts',(0.00718920850443293,-0.0393727712201326,
-0.0111887947561811));
#19785=CARTESIAN_POINT('Ctrl Pts',(0.00711195822786157,-0.0393788885134016,
-0.0111057738669521));
#19786=CARTESIAN_POINT('Ctrl Pts',(0.00709382236338263,-0.0393802678734445,
-0.0110872423321149));
#19787=CARTESIAN_POINT('Ctrl Pts',(0.00706411065729706,-0.0393824399331051,
-0.011058374987786));
#19788=CARTESIAN_POINT('Ctrl Pts',(0.0070528315603696,-0.0393832453731153,
-0.0110477420473776));
#19789=CARTESIAN_POINT('Ctrl Pts',(0.00703091463089175,-0.0393847749519049,
-0.0110276957592165));
#19790=CARTESIAN_POINT('Ctrl Pts',(0.00702030333587553,-0.039385500174762,
-0.0110182558590788));
#19791=CARTESIAN_POINT('Ctrl Pts',(0.00699524389711843,-0.039387178344524,
-0.0109965750764129));
#19792=CARTESIAN_POINT('Ctrl Pts',(0.00698069761950371,-0.0393881264915898,
-0.0109844508649484));
#19793=CARTESIAN_POINT('Ctrl Pts',(0.0069299835487691,-0.0393913482912109,
-0.0109437394045853));
#19794=CARTESIAN_POINT('Ctrl Pts',(0.00689275896597333,-0.0393935697898956,
-0.0109165058748375));
#19795=CARTESIAN_POINT('Ctrl Pts',(0.0067908828791787,-0.0393993506137635,
-0.0108487640836643));
#19796=CARTESIAN_POINT('Ctrl Pts',(0.00672435413730686,-0.0394028230549071,
-0.0108113119608518));
#19797=CARTESIAN_POINT('Ctrl Pts',(0.00658758886596875,-0.0394097558447258,
-0.0107471521294095));
#19798=CARTESIAN_POINT('Ctrl Pts',(0.00651763195780711,-0.039413208057472,
-0.0107203454985814));
#19799=CARTESIAN_POINT('Ctrl Pts',(0.00642960987282296,-0.0394177287425997,
-0.0106937675988903));
#19800=CARTESIAN_POINT('Ctrl Pts',(0.00641312501222299,-0.0394185829302909,
-0.0106890882385291));
#19801=CARTESIAN_POINT('Ctrl Pts',(0.0063875881418275,-0.0394199224660671,
-0.0106822968797147));
#19802=CARTESIAN_POINT('Ctrl Pts',(0.00637858883336489,-0.0394203976194904,
-0.0106799903934575));
#19803=CARTESIAN_POINT('Ctrl Pts',(0.00636175584962722,-0.0394212930605527,
-0.0106758377954993));
#19804=CARTESIAN_POINT('Ctrl Pts',(0.00635392773562898,-0.0394217122443688,
-0.0106739714949896));
#19805=CARTESIAN_POINT('Ctrl Pts',(0.00633498375343425,-0.0394227329725285,
-0.0106696113858608));
#19806=CARTESIAN_POINT('Ctrl Pts',(0.00632385433012678,-0.0394233377993604,
-0.0106671793203644));
#19807=CARTESIAN_POINT('Ctrl Pts',(0.00628283310367387,-0.0394255834116466,
-0.0106586899368512));
#19808=CARTESIAN_POINT('Ctrl Pts',(0.00625279189752091,-0.0394272595974423,
-0.0106533963156152));
#19809=CARTESIAN_POINT('Ctrl Pts',(0.00617035672210289,-0.0394319101036196,
-0.0106413772775292));
#19810=CARTESIAN_POINT('Ctrl Pts',(0.00611774320291216,-0.0394349329062986,
-0.0106364462131634));
#19811=CARTESIAN_POINT('Ctrl Pts',(0.00595269210824942,-0.0394444123670926,
-0.0106294889760128));
#19812=CARTESIAN_POINT('Ctrl Pts',(0.00584020401004156,-0.0394508385022363,
-0.0106370379744194));
#19813=CARTESIAN_POINT('Ctrl Pts',(0.00570506492205468,-0.0394582272720285,
-0.0106610993360945));
#19814=CARTESIAN_POINT('Ctrl Pts',(0.00568071335427352,-0.0394595469531732,
-0.0106660445689519));
#19815=CARTESIAN_POINT('Ctrl Pts',(0.00564159093022336,-0.0394616487267255,
-0.0106749783674692));
#19816=CARTESIAN_POINT('Ctrl Pts',(0.00562674206081955,-0.0394624421446139,
-0.0106786020994859));
#19817=CARTESIAN_POINT('Ctrl Pts',(0.0055981290235456,-0.0394639632510294,
-0.0106860369861944));
#19818=CARTESIAN_POINT('Ctrl Pts',(0.00558435916065565,-0.0394646917567988,
-0.0106898197738135));
#19819=CARTESIAN_POINT('Ctrl Pts',(0.00555194286451575,-0.0394663993032991,
-0.0106992108562706));
#19820=CARTESIAN_POINT('Ctrl Pts',(0.00553334597538514,-0.0394673729953005,
-0.0107049820727591));
#19821=CARTESIAN_POINT('Ctrl Pts',(0.00546717229893642,-0.03947082108304,
-0.0107268993478225));
#19822=CARTESIAN_POINT('Ctrl Pts',(0.00542027963022814,-0.0394732321872962,
-0.0107450151629393));
#19823=CARTESIAN_POINT('Ctrl Pts',(0.00529196275906799,-0.0394798346253841,
-0.0108019334403542));
#19824=CARTESIAN_POINT('Ctrl Pts',(0.00521293622902167,-0.0394838984970044,
-0.0108456265870401));
#19825=CARTESIAN_POINT('Ctrl Pts',(0.00508727004304241,-0.039490903777605,
-0.0109302452805476));
#19826=CARTESIAN_POINT('Ctrl Pts',(0.00503845935594229,-0.0394937870607772,
-0.010967526514593));
#19827=CARTESIAN_POINT('Ctrl Pts',(0.00498139135085344,-0.0394975301438743,
-0.0110167666444608));
#19828=CARTESIAN_POINT('Ctrl Pts',(0.00497090573769416,-0.0394982345580348,
-0.0110260661769412));
#19829=CARTESIAN_POINT('Ctrl Pts',(0.00495423816799124,-0.0394993841075498,
-0.011041259042327));
#19830=CARTESIAN_POINT('Ctrl Pts',(0.00494797573156072,-0.0394998229914564,
-0.0110470632971329));
#19831=CARTESIAN_POINT('Ctrl Pts',(0.00493562113641095,-0.0395007035436268,
-0.0110587061012606));
#19832=CARTESIAN_POINT('Ctrl Pts',(0.00492952807540038,-0.0395011451148093,
-0.0110645432263977));
#19833=CARTESIAN_POINT('Ctrl Pts',(0.00491378371668259,-0.0395023045275902,
-0.0110798758708019));
#19834=CARTESIAN_POINT('Ctrl Pts',(0.00490420913692148,-0.0395030279319976,
-0.0110894488176715));
#19835=CARTESIAN_POINT('Ctrl Pts',(0.00485659331262227,-0.0395067131943612,
-0.0111383263759616));
#19836=CARTESIAN_POINT('Ctrl Pts',(0.00482053772912876,-0.0395097903013872,
-0.0111795055768089));
#19837=CARTESIAN_POINT('Ctrl Pts',(0.00472857369128798,-0.0395182754451432,
-0.0112965414781219));
#19838=CARTESIAN_POINT('Ctrl Pts',(0.00467729406004648,-0.0395237340592735,
-0.0113757501141798));
#19839=CARTESIAN_POINT('Ctrl Pts',(0.00460934819643015,-0.0395319167039995,
-0.0115052919742768));
#19840=CARTESIAN_POINT('Ctrl Pts',(0.00458749349020553,-0.039534771741006,
-0.0115526429810435));
#19841=CARTESIAN_POINT('Ctrl Pts',(0.00456056200635623,-0.0395386220185198,
-0.0116197291926716));
#19842=CARTESIAN_POINT('Ctrl Pts',(0.00455341594966046,-0.0395396842253357,
-0.0116385913560591));
#19843=CARTESIAN_POINT('Ctrl Pts',(0.00454185561065168,-0.039541476070495,
-0.0116710097793207));
#19844=CARTESIAN_POINT('Ctrl Pts',(0.00453725575577049,-0.0395422117273783,
-0.0116844966737503));
#19845=CARTESIAN_POINT('Ctrl Pts',(0.00452819314722318,-0.0395437101806055,
-0.0117123243313634));
#19846=CARTESIAN_POINT('Ctrl Pts',(0.00452375161652047,-0.0395444722214163,
-0.0117266704341375));
#19847=CARTESIAN_POINT('Ctrl Pts',(0.00451289661452796,-0.0395464101513956,
-0.011763633585646));
#19848=CARTESIAN_POINT('Ctrl Pts',(0.00450678917596303,-0.0395475761713947,
-0.0117863368317175));
#19849=CARTESIAN_POINT('Ctrl Pts',(0.00448586224387566,-0.0395518884847612,
-0.0118718748533699));
#19850=CARTESIAN_POINT('Ctrl Pts',(0.00447447100211849,-0.0395549300823339,
-0.0119354821694805));
#19851=CARTESIAN_POINT('Ctrl Pts',(0.00446063355208643,-0.0395605389620168,
-0.0120558421289123));
#19852=CARTESIAN_POINT('Ctrl Pts',(0.00445726780193232,-0.0395631150864761,
-0.0121123779022069));
#19853=CARTESIAN_POINT('Ctrl Pts',(0.00445700511695951,-0.0395658248041787,
-0.0121712646770232));
#19854=CARTESIAN_POINT('Ctrl Pts',(0.0044570000000005,-0.0395659304248953,
-0.012173559022778));
#19855=CARTESIAN_POINT('Ctrl Pts',(0.004457,-0.0395660360928446,-0.012175853286222));
#19856=CARTESIAN_POINT('Ctrl Pts',(0.004457,-0.0396826982119552,-0.0121758532865581));
#19857=CARTESIAN_POINT('Ctrl Pts',(0.004457,-0.0396813477299627,-0.0121464846796299));
#19858=CARTESIAN_POINT('Ctrl Pts',(0.00445783847339417,-0.0396799949258229,
-0.0121171007278321));
#19859=CARTESIAN_POINT('Ctrl Pts',(0.0044628146601358,-0.0396759462670294,
-0.0120301049610795));
#19860=CARTESIAN_POINT('Ctrl Pts',(0.0044693426023891,-0.0396732191572142,
-0.0119727075344027));
#19861=CARTESIAN_POINT('Ctrl Pts',(0.00448141319135842,-0.0396696575578575,
-0.0119021079550972));
#19862=CARTESIAN_POINT('Ctrl Pts',(0.00448394202212993,-0.03966895783635,
-0.0118884327154763));
#19863=CARTESIAN_POINT('Ctrl Pts',(0.0044883471833378,-0.0396678061649656,
-0.0118662891469104));
#19864=CARTESIAN_POINT('Ctrl Pts',(0.00449011073731352,-0.039667360112438,
-0.0118577988825109));
#19865=CARTESIAN_POINT('Ctrl Pts',(0.00449358570177043,-0.0396665077070338,
-0.0118417499813716));
#19866=CARTESIAN_POINT('Ctrl Pts',(0.00449528267524121,-0.0396661022051225,
-0.0118341885034603));
#19867=CARTESIAN_POINT('Ctrl Pts',(0.00450010243933532,-0.0396649796913041,
-0.0118134449184029));
#19868=CARTESIAN_POINT('Ctrl Pts',(0.00450334192183023,-0.0396642566401885,
-0.0118002909204535));
#19869=CARTESIAN_POINT('Ctrl Pts',(0.00451856796563602,-0.0396609960613739,
-0.0117417936437361));
#19870=CARTESIAN_POINT('Ctrl Pts',(0.00453244432857552,-0.0396583767538485,
-0.0116969708733201));
#19871=CARTESIAN_POINT('Ctrl Pts',(0.00458237804669033,-0.0396500308634471,
-0.0115583727629975));
#19872=CARTESIAN_POINT('Ctrl Pts',(0.00462556288009749,-0.0396442067768584,
-0.0114674332420484));
#19873=CARTESIAN_POINT('Ctrl Pts',(0.00470446074305107,-0.039635648261241,
-0.0113360832850121));
#19874=CARTESIAN_POINT('Ctrl Pts',(0.00473394847505017,-0.0396327601067996,
-0.0112922527054986));
#19875=CARTESIAN_POINT('Ctrl Pts',(0.00477768781464053,-0.0396288824594807,
-0.01123393719722));
#19876=CARTESIAN_POINT('Ctrl Pts',(0.00479006148908284,-0.0396278249657828,
-0.0112180945238591));
#19877=CARTESIAN_POINT('Ctrl Pts',(0.00481202474720552,-0.0396260138521039,
-0.0111910790176491));
#19878=CARTESIAN_POINT('Ctrl Pts',(0.00482147100184777,-0.0396252548043261,
-0.011179793558469));
#19879=CARTESIAN_POINT('Ctrl Pts',(0.00484136391135476,-0.0396236961559212,
-0.0111567067120257));
#19880=CARTESIAN_POINT('Ctrl Pts',(0.00485183284751335,-0.0396228975837342,
-0.0111449267424395));
#19881=CARTESIAN_POINT('Ctrl Pts',(0.00487985460071512,-0.0396208146781954,
-0.0111143522291492));
#19882=CARTESIAN_POINT('Ctrl Pts',(0.00489770024196365,-0.0396195425516972,
-0.0110958322007141));
#19883=CARTESIAN_POINT('Ctrl Pts',(0.00499026602745119,-0.0396131942898049,
-0.011004454012922));
#19884=CARTESIAN_POINT('Ctrl Pts',(0.00507177605414737,-0.0396084218615467,
-0.0109388646206537));
#19885=CARTESIAN_POINT('Ctrl Pts',(0.00522781437372861,-0.03959986063786,
-0.0108374748169949));
#19886=CARTESIAN_POINT('Ctrl Pts',(0.00529976403573722,-0.0395960881101994,
-0.0107984664089359));
#19887=CARTESIAN_POINT('Ctrl Pts',(0.00538780060713031,-0.0395913100917849,
-0.0107594232560758));
#19888=CARTESIAN_POINT('Ctrl Pts',(0.00540122886535887,-0.0395905769266395,
-0.0107536946358699));
#19889=CARTESIAN_POINT('Ctrl Pts',(0.00542289402125798,-0.0395893840455478,
-0.0107448133052319));
#19890=CARTESIAN_POINT('Ctrl Pts',(0.00543108044167049,-0.0395889310424141,
-0.010741539071419));
#19891=CARTESIAN_POINT('Ctrl Pts',(0.00544738792697787,-0.0395880233536636,
-0.0107351783162355));
#19892=CARTESIAN_POINT('Ctrl Pts',(0.0054555078627059,-0.039587568791161,
-0.0107320898789015));
#19893=CARTESIAN_POINT('Ctrl Pts',(0.00547676543253324,-0.0395863728255643,
-0.0107242093404772));
#19894=CARTESIAN_POINT('Ctrl Pts',(0.00548994269434414,-0.0395856255829875,
-0.0107195270602234));
#19895=CARTESIAN_POINT('Ctrl Pts',(0.00555587875445098,-0.0395818637929086,
-0.0106971026181067));
#19896=CARTESIAN_POINT('Ctrl Pts',(0.00560950361920212,-0.0395787336211777,
-0.0106820464514176));
#19897=CARTESIAN_POINT('Ctrl Pts',(0.00575462281729089,-0.0395702686795682,
-0.010649650447936));
#19898=CARTESIAN_POINT('Ctrl Pts',(0.00584708012371164,-0.0395648933650903,
-0.0106376327076299));
#19899=CARTESIAN_POINT('Ctrl Pts',(0.00599106730777496,-0.0395568581375937,
-0.0106320349547745));
#19900=CARTESIAN_POINT('Ctrl Pts',(0.00604214631384966,-0.039554069253411,
-0.0106325842638334));
#19901=CARTESIAN_POINT('Ctrl Pts',(0.00611296474157648,-0.0395502973398212,
-0.0106368654059014));
#19902=CARTESIAN_POINT('Ctrl Pts',(0.00613279694005223,-0.0395492512057836,
-0.0106384497121049));
#19903=CARTESIAN_POINT('Ctrl Pts',(0.00616720681918736,-0.0395474530826791,
-0.0106418694094461));
#19904=CARTESIAN_POINT('Ctrl Pts',(0.00618179888186008,-0.0395466958805926,
-0.0106435302652938));
#19905=CARTESIAN_POINT('Ctrl Pts',(0.00621207369310954,-0.0395451352821237,
-0.010647414683645));
#19906=CARTESIAN_POINT('Ctrl Pts',(0.00622775042261874,-0.0395443330149265,
-0.0106496719137741));
#19907=CARTESIAN_POINT('Ctrl Pts',(0.00626917403819766,-0.0395422270801734,
-0.0106562888367076));
#19908=CARTESIAN_POINT('Ctrl Pts',(0.00629485018986162,-0.0395409361443949,
-0.0106610614719308));
#19909=CARTESIAN_POINT('Ctrl Pts',(0.00640527168510984,-0.0395354312145129,
-0.0106845006360704));
#19910=CARTESIAN_POINT('Ctrl Pts',(0.00648848281896762,-0.0395314138452922,
-0.0107096459613776));
#19911=CARTESIAN_POINT('Ctrl Pts',(0.0066324695229468,-0.039524288718721,
-0.0107667850576158));
#19912=CARTESIAN_POINT('Ctrl Pts',(0.00669406056589768,-0.0395211751249589,
-0.0107960815303267));
#19913=CARTESIAN_POINT('Ctrl Pts',(0.00678435861486421,-0.0395162567234915,
-0.0108466128520862));
#19914=CARTESIAN_POINT('Ctrl Pts',(0.00681460207201887,-0.0395145437879072,
-0.0108649292893225));
#19915=CARTESIAN_POINT('Ctrl Pts',(0.00685437394505175,-0.0395121660453758,
-0.0108909244011376));
#19916=CARTESIAN_POINT('Ctrl Pts',(0.00686448053538532,-0.0395115505375329,
-0.0108977020962806));
#19917=CARTESIAN_POINT('Ctrl Pts',(0.00688138227626394,-0.0395105001679217,
-0.0109093289285492));
#19918=CARTESIAN_POINT('Ctrl Pts',(0.00688822032611236,-0.0395100692725072,
-0.0109141150738139));
#19919=CARTESIAN_POINT('Ctrl Pts',(0.00690268068269267,-0.0395091447748852,
-0.0109244120990847));
#19920=CARTESIAN_POINT('Ctrl Pts',(0.00691029186237285,-0.0395086502977725,
-0.0109299374879752));
#19921=CARTESIAN_POINT('Ctrl Pts',(0.00693186511827695,-0.0395072272758132,
-0.0109459019424193));
#19922=CARTESIAN_POINT('Ctrl Pts',(0.00694570108428603,-0.039506288607471,
-0.0109565082498288));
#19923=CARTESIAN_POINT('Ctrl Pts',(0.00701132081403296,-0.0395017219760775,
-0.0110085994139154));
#19924=CARTESIAN_POINT('Ctrl Pts',(0.00706056951866714,-0.0394979467687672,
-0.0110531589714796));
#19925=CARTESIAN_POINT('Ctrl Pts',(0.00715025608634116,-0.0394905828958167,
-0.0111454888787071));
#19926=CARTESIAN_POINT('Ctrl Pts',(0.00719096653660539,-0.0394870033330039,
-0.0111928278015998));
#19927=CARTESIAN_POINT('Ctrl Pts',(0.00726618388378849,-0.0394800037621922,
-0.0112918469070288));
#19928=CARTESIAN_POINT('Ctrl Pts',(0.00730066353650197,-0.0394765892690963,
-0.0113434083495262));
#19929=CARTESIAN_POINT('Ctrl Pts',(0.00734257510813545,-0.0394721622303368,
-0.0114150747698283));
#19930=CARTESIAN_POINT('Ctrl Pts',(0.00735282647491831,-0.0394710528057832,
-0.0114334568571033));
#19931=CARTESIAN_POINT('Ctrl Pts',(0.00736967399406156,-0.0394691817601985,
-0.0114651752693526));
#19932=CARTESIAN_POINT('Ctrl Pts',(0.00737645900917835,-0.0394684137109337,
-0.0114784074389878));
#19933=CARTESIAN_POINT('Ctrl Pts',(0.00738990428348948,-0.039466860629517,
-0.011505589195671));
#19934=CARTESIAN_POINT('Ctrl Pts',(0.00739654833087479,-0.0394660762105413,
-0.0115195449365994));
#19935=CARTESIAN_POINT('Ctrl Pts',(0.00741304658386693,-0.0394640821783535,
-0.011555584756424));
#19936=CARTESIAN_POINT('Ctrl Pts',(0.00742259351896264,-0.0394628828222944,
-0.0115778052492526));
#19937=CARTESIAN_POINT('Ctrl Pts',(0.00747562986144973,-0.0394559216441528,
-0.0117097129568753));
#19938=CARTESIAN_POINT('Ctrl Pts',(0.00750694344444106,-0.0394505712751792,
-0.0118238685044784));
#19939=CARTESIAN_POINT('Ctrl Pts',(0.00753237966638465,-0.0394428789488251,
-0.0119886672284317));
#19940=CARTESIAN_POINT('Ctrl Pts',(0.00753752853051408,-0.039440612730165,
-0.0120371750878508));
#19941=CARTESIAN_POINT('Ctrl Pts',(0.00754207195897334,-0.0394368747944667,
-0.012114927858575));
#19942=CARTESIAN_POINT('Ctrl Pts',(0.00754294731747926,-0.0394354508996611,
-0.0121440536802233));
#19943=CARTESIAN_POINT('Ctrl Pts',(0.00754301545459039,-0.0394334725882418,
-0.0121834575229681));
#19944=CARTESIAN_POINT('Ctrl Pts',(0.00754293063581711,-0.0394329520788969,
-0.012193729779417));
#19945=CARTESIAN_POINT('Ctrl Pts',(0.00754259079738741,-0.0394319983784609,
-0.0122123564785995));
#19946=CARTESIAN_POINT('Ctrl Pts',(0.0075423704519968,-0.0394315669838307,
-0.0122207112725747));
#19947=CARTESIAN_POINT('Ctrl Pts',(0.00754175894997875,-0.0394306436476368,
-0.0122384330323876));
#19948=CARTESIAN_POINT('Ctrl Pts',(0.0075413502928078,-0.0394301508688712,
-0.012247798756299));
#19949=CARTESIAN_POINT('Ctrl Pts',(0.00753994571567989,-0.0394287377858593,
-0.0122744171383556));
#19950=CARTESIAN_POINT('Ctrl Pts',(0.00753874528646912,-0.0394278075655499,
-0.0122916571571346));
#19951=CARTESIAN_POINT('Ctrl Pts',(0.00753177511392533,-0.0394234021706708,
-0.0123722088515272));
#19952=CARTESIAN_POINT('Ctrl Pts',(0.00752238592811473,-0.0394197916372626,
-0.012435141760605));
#19953=CARTESIAN_POINT('Ctrl Pts',(0.00748376115408445,-0.0394091909128788,
-0.0126164727734878));
#19954=CARTESIAN_POINT('Ctrl Pts',(0.00744435035573978,-0.0394022112486446,
-0.0127322282952963));
#19955=CARTESIAN_POINT('Ctrl Pts',(0.0073815215085189,-0.039394406462627,
-0.012863461934239));
#19956=CARTESIAN_POINT('Ctrl Pts',(0.00737082950555611,-0.0393931547705145,
-0.0128845378977993));
#19957=CARTESIAN_POINT('Ctrl Pts',(0.00735240109533733,-0.0393911171079385,
-0.0129188847988983));
#19958=CARTESIAN_POINT('Ctrl Pts',(0.00734494340957853,-0.0393903217788686,
-0.012932300110989));
#19959=CARTESIAN_POINT('Ctrl Pts',(0.00732983328516685,-0.0393887659401232,
-0.0129585509646158));
#19960=CARTESIAN_POINT('Ctrl Pts',(0.00732219210545131,-0.0393880051504652,
-0.0129713910152601));
#19961=CARTESIAN_POINT('Ctrl Pts',(0.00730312691546296,-0.0393861676315112,
-0.0130023939971382));
#19962=CARTESIAN_POINT('Ctrl Pts',(0.00729150810773439,-0.0393850979851545,
-0.0130204337546251));
#19963=CARTESIAN_POINT('Ctrl Pts',(0.00724215521505821,-0.0393807467790544,
-0.0130936594565076));
#19964=CARTESIAN_POINT('Ctrl Pts',(0.00720122910888186,-0.0393775819218252,
-0.0131466094160062));
#19965=CARTESIAN_POINT('Ctrl Pts',(0.0071189177617141,-0.0393718009711476,
-0.0132398947139605));
#19966=CARTESIAN_POINT('Ctrl Pts',(0.00707845579281076,-0.0393691732790731,
-0.0132808846220152));
#19967=CARTESIAN_POINT('Ctrl Pts',(0.00698731281257816,-0.0393634992861697,
-0.013363431365392));
#19968=CARTESIAN_POINT('Ctrl Pts',(0.00693608663055851,-0.0393604504404471,
-0.0134042134842198));
#19969=CARTESIAN_POINT('Ctrl Pts',(0.00686816131919823,-0.0393563759987104,
-0.0134515678176983));
#19970=CARTESIAN_POINT('Ctrl Pts',(0.00685372372266027,-0.0393555081534511,
-0.013461274385076));
#19971=CARTESIAN_POINT('Ctrl Pts',(0.00683123889132765,-0.039354148919096,
-0.013475845297313));
#19972=CARTESIAN_POINT('Ctrl Pts',(0.00682330577582393,-0.0393536679148107,
-0.0134808839043566));
#19973=CARTESIAN_POINT('Ctrl Pts',(0.00680823861899004,-0.0393527507020857,
-0.0134902615373085));
#19974=CARTESIAN_POINT('Ctrl Pts',(0.00680111461139358,-0.0393523154246154,
-0.0134946156164375));
#19975=CARTESIAN_POINT('Ctrl Pts',(0.00678350750990883,-0.0393512361991847,
-0.0135051814857837));
#19976=CARTESIAN_POINT('Ctrl Pts',(0.00677298560503136,-0.0393505883564157,
-0.013511327253304));
#19977=CARTESIAN_POINT('Ctrl Pts',(0.00673153221613039,-0.0393480280940242,
-0.0135348858674737));
#19978=CARTESIAN_POINT('Ctrl Pts',(0.00670007796683072,-0.0393460684753522,
-0.0135513529986706));
#19979=CARTESIAN_POINT('Ctrl Pts',(0.00660619306212918,-0.0393402284134957,
-0.0135964494906086));
#19980=CARTESIAN_POINT('Ctrl Pts',(0.00654238602229767,-0.0393362739721421,
-0.0136220139417997));
#19981=CARTESIAN_POINT('Ctrl Pts',(0.0063952543354997,-0.0393274334059212,
-0.0136698506289411));
#19982=CARTESIAN_POINT('Ctrl Pts',(0.00631132821339653,-0.0393225857900594,
-0.0136895678719792));
#19983=CARTESIAN_POINT('Ctrl Pts',(0.00620036099988987,-0.0393165380231932,
-0.013706012145665));
#19984=CARTESIAN_POINT('Ctrl Pts',(0.00617444042482592,-0.0393151494417041,
-0.0137091834241441));
#19985=CARTESIAN_POINT('Ctrl Pts',(0.00613268754209303,-0.0393129506447138,
-0.0137132191561805));
#19986=CARTESIAN_POINT('Ctrl Pts',(0.00611690142752418,-0.0393121279502458,
-0.0137145000561371));
#19987=CARTESIAN_POINT('Ctrl Pts',(0.00608644415222851,-0.0393105566497989,
-0.0137164999265871));
#19988=CARTESIAN_POINT('Ctrl Pts',(0.00607177701558757,-0.0393098070881823,
-0.0137172528907943));
#19989=CARTESIAN_POINT('Ctrl Pts',(0.0060372205574106,-0.0393080568887944,
-0.0137185325809435));
#19990=CARTESIAN_POINT('Ctrl Pts',(0.00601732718663373,-0.0393070616631757,
-0.0137188842611421));
#19991=CARTESIAN_POINT('Ctrl Pts',(0.00594637482767709,-0.039303551032031,
-0.0137187661752197));
#19992=CARTESIAN_POINT('Ctrl Pts',(0.00589535115549701,-0.0393010997047533,
-0.0137161471023089));
#19993=CARTESIAN_POINT('Ctrl Pts',(0.00575194066052965,-0.0392943138716219,
-0.013701625102289));
#19994=CARTESIAN_POINT('Ctrl Pts',(0.00566037434013233,-0.0392901131104682,
-0.0136838875047544));
#19995=CARTESIAN_POINT('Ctrl Pts',(0.00551754075649261,-0.039283195535279,
-0.013642541876957));
#19996=CARTESIAN_POINT('Ctrl Pts',(0.00546499537765861,-0.0392805634681504,
-0.0136242011111475));
#19997=CARTESIAN_POINT('Ctrl Pts',(0.00540062601821025,-0.0392771038213513,
-0.0135977517849151));
#19998=CARTESIAN_POINT('Ctrl Pts',(0.00538776603958515,-0.0392764004451236,
-0.0135922621477581));
#19999=CARTESIAN_POINT('Ctrl Pts',(0.00536704035512664,-0.0392752442881333,
-0.0135830798332581));
#20000=CARTESIAN_POINT('Ctrl Pts',(0.0053591278513458,-0.0392747974925742,
-0.0135794940345151));
#20001=CARTESIAN_POINT('Ctrl Pts',(0.00534324601646462,-0.0392738889570015,
-0.0135721344014611));
#20002=CARTESIAN_POINT('Ctrl Pts',(0.00533527795192002,-0.039273427130702,
-0.0135683587042053));
#20003=CARTESIAN_POINT('Ctrl Pts',(0.00531420239727291,-0.0392721904587869,
-0.0135581498666673));
#20004=CARTESIAN_POINT('Ctrl Pts',(0.00530115337438712,-0.0392714090737808,
-0.0135515987396149));
#20005=CARTESIAN_POINT('Ctrl Pts',(0.00527203926043385,-0.0392696334575321,
-0.0135364612110366));
#20006=CARTESIAN_POINT('Ctrl Pts',(0.00525602937070322,-0.0392686345585567,
-0.0135277735573995));
#20007=CARTESIAN_POINT('Ctrl Pts',(0.00520443646351128,-0.0392653504626187,
-0.0134985830437455));
#20008=CARTESIAN_POINT('Ctrl Pts',(0.0051695183200595,-0.0392630255012293,
-0.0134769433051452));
#20009=CARTESIAN_POINT('Ctrl Pts',(0.00502926456191316,-0.0392533679337981,
-0.0133820759774999));
#20010=CARTESIAN_POINT('Ctrl Pts',(0.00493237841609905,-0.0392459766985508,
-0.0132972337122274));
#20011=CARTESIAN_POINT('Ctrl Pts',(0.0048305166975368,-0.0392377326885316,
-0.0131827201552549));
#20012=CARTESIAN_POINT('Ctrl Pts',(0.0048143809576707,-0.0392364074789784,
-0.0131636688904647));
#20013=CARTESIAN_POINT('Ctrl Pts',(0.00478891756095033,-0.0392342832560996,
-0.0131320812807735));
#20014=CARTESIAN_POINT('Ctrl Pts',(0.00477930595930315,-0.0392334732468315,
-0.0131197805790117));
#20015=CARTESIAN_POINT('Ctrl Pts',(0.00476095770797615,-0.0392319100803299,
-0.0130955498446295));
#20016=CARTESIAN_POINT('Ctrl Pts',(0.00475220264996732,-0.0392311562649615,
-0.0130836359438985));
#20017=CARTESIAN_POINT('Ctrl Pts',(0.00473170106261873,-0.0392293707410409,
-0.0130548802160828));
#20018=CARTESIAN_POINT('Ctrl Pts',(0.00472011669724982,-0.0392283451159299,
-0.013037925973519));
#20019=CARTESIAN_POINT('Ctrl Pts',(0.00467782647526548,-0.039224530357409,
-0.0129732999293021));
#20020=CARTESIAN_POINT('Ctrl Pts',(0.00464941657252458,-0.0392218222264274,
-0.0129241775015689));
#20021=CARTESIAN_POINT('Ctrl Pts',(0.00456857432880205,-0.0392134506605656,
-0.0127647251481053));
#20022=CARTESIAN_POINT('Ctrl Pts',(0.0045264948743849,-0.0392080363748214,
-0.0126496966453715));
#20023=CARTESIAN_POINT('Ctrl Pts',(0.00449254436710671,-0.0392009180337278,
-0.012506120026494));
#20024=CARTESIAN_POINT('Ctrl Pts',(0.00448729504029299,-0.0391996673600789,
-0.0124811763649061));
#20025=CARTESIAN_POINT('Ctrl Pts',(0.00448082614761093,-0.0391978780351706,
-0.0124461539039167));
#20026=CARTESIAN_POINT('Ctrl Pts',(0.00447908437208494,-0.0391973644414086,
-0.0124361747419941));
#20027=CARTESIAN_POINT('Ctrl Pts',(0.00447609004540929,-0.0391964191387795,
-0.0124179623436085));
#20028=CARTESIAN_POINT('Ctrl Pts',(0.00447480563451979,-0.0391959891059064,
-0.0124097346486363));
#20029=CARTESIAN_POINT('Ctrl Pts',(0.00447220407531662,-0.0391950623656671,
-0.0123921358694383));
#20030=CARTESIAN_POINT('Ctrl Pts',(0.00447090645100197,-0.0391945647136088,
-0.0123827625726031));
#20031=CARTESIAN_POINT('Ctrl Pts',(0.00446742697084075,-0.0391931230174556,
-0.0123558056381653));
#20032=CARTESIAN_POINT('Ctrl Pts',(0.0044654617234968,-0.0391921684549766,
-0.012338196029259));
#20033=CARTESIAN_POINT('Ctrl Pts',(0.00445926803716274,-0.039188566267966,
-0.0122724428785937));
#20034=CARTESIAN_POINT('Ctrl Pts',(0.00445700000038672,-0.0391858460740657,
-0.0122241549811162));
#20035=CARTESIAN_POINT('Ctrl Pts',(0.004457,-0.0391830969983919,-0.012175853298912));
#20036=CARTESIAN_POINT('Origin',(0.006,-0.0418165664398416,-0.0121758532865581));
#20037=CARTESIAN_POINT('',(0.004457,-0.0401812248373849,-0.0121758532903003));
#20038=CARTESIAN_POINT('',(0.004457,-0.0400658559061629,-0.0121758532865568));
#20039=CARTESIAN_POINT('',(0.004457,-0.0418165664398416,-0.0121758532865581));
#20040=CARTESIAN_POINT('',(0.00445700008689307,-0.0400658264344116,-0.0121753354525968));
#20041=CARTESIAN_POINT('Ctrl Pts',(0.004457,-0.0400658559061629,-0.0121758532865556));
#20042=CARTESIAN_POINT('Ctrl Pts',(0.004457,-0.0400658460818209,-0.0121756806755878));
#20043=CARTESIAN_POINT('Ctrl Pts',(0.00445700002896424,-0.040065836257903,
-0.0121755080642658));
#20044=CARTESIAN_POINT('Ctrl Pts',(0.00445700008689307,-0.0400658264344116,
-0.0121753354525968));
#20045=CARTESIAN_POINT('Ctrl Pts',(0.004457,-0.0395660360928446,-0.012175853286222));
#20046=CARTESIAN_POINT('Ctrl Pts',(0.00445699999998617,-0.0395689601809892,
-0.0122393411137212));
#20047=CARTESIAN_POINT('Ctrl Pts',(0.00446091839675691,-0.0395719185953119,
-0.0123027659954965));
#20048=CARTESIAN_POINT('Ctrl Pts',(0.00447083410518774,-0.0395758801751546,
-0.012382716565834));
#20049=CARTESIAN_POINT('Ctrl Pts',(0.00447321763691439,-0.039576731730892,
-0.012399630679702));
#20050=CARTESIAN_POINT('Ctrl Pts',(0.00447732845847337,-0.039578067994637,
-0.0124256661550697));
#20051=CARTESIAN_POINT('Ctrl Pts',(0.00447885816470674,-0.039578542585737,
-0.0124348177651906));
#20052=CARTESIAN_POINT('Ctrl Pts',(0.00448186914994206,-0.0395794376342485,
-0.0124518832473571));
#20053=CARTESIAN_POINT('Ctrl Pts',(0.00448332996972611,-0.0395798570017059,
-0.0124598001585569));
#20054=CARTESIAN_POINT('Ctrl Pts',(0.00448701159110442,-0.0395808791127856,
-0.0124789132782396));
#20055=CARTESIAN_POINT('Ctrl Pts',(0.00448929477719453,-0.0395814851619161,
-0.012490096820538));
#20056=CARTESIAN_POINT('Ctrl Pts',(0.00449816946914826,-0.0395837412623587,
-0.0125312328576436));
#20057=CARTESIAN_POINT('Ctrl Pts',(0.00450552918193665,-0.0395854271244627,
-0.0125610108273582));
#20058=CARTESIAN_POINT('Ctrl Pts',(0.00452809564029531,-0.0395901154443399,
-0.012641887057726));
#20059=CARTESIAN_POINT('Ctrl Pts',(0.00454507052962667,-0.039593167209448,
-0.0126924476312603));
#20060=CARTESIAN_POINT('Ctrl Pts',(0.00460553185885785,-0.0396026230303215,
-0.012845730439032));
#20061=CARTESIAN_POINT('Ctrl Pts',(0.00465756145700691,-0.0396089946135861,
-0.012944710943898));
#20062=CARTESIAN_POINT('Ctrl Pts',(0.00473373784842731,-0.0396163414180909,
-0.0130579255775263));
#20063=CARTESIAN_POINT('Ctrl Pts',(0.00474816494768303,-0.0396176667909736,
-0.0130782835947885));
#20064=CARTESIAN_POINT('Ctrl Pts',(0.00477222898515148,-0.0396197752738234,
-0.0131105519281751));
#20065=CARTESIAN_POINT('Ctrl Pts',(0.00478156024751075,-0.0396205698415416,
-0.013122683687153));
#20066=CARTESIAN_POINT('Ctrl Pts',(0.00479993847770898,-0.0396220917113368,
-0.0131458558608025));
#20067=CARTESIAN_POINT('Ctrl Pts',(0.00480896113887782,-0.0396228198568822,
-0.013156913478584));
#20068=CARTESIAN_POINT('Ctrl Pts',(0.00483061749799173,-0.0396245243474121,
-0.0131827149840867));
#20069=CARTESIAN_POINT('Ctrl Pts',(0.00484337875531893,-0.0396254954007976,
-0.0131973488825598));
#20070=CARTESIAN_POINT('Ctrl Pts',(0.00488983962916297,-0.0396289191362715,
-0.0132486403230585));
#20071=CARTESIAN_POINT('Ctrl Pts',(0.00492503409007518,-0.0396313097846007,
-0.0132839042429659));
#20072=CARTESIAN_POINT('Ctrl Pts',(0.00501625070944102,-0.039637111644823,
-0.0133668563839947));
#20073=CARTESIAN_POINT('Ctrl Pts',(0.0050740919059058,-0.0396404565945327,
-0.0134123586816373));
#20074=CARTESIAN_POINT('Ctrl Pts',(0.00519945609416132,-0.0396474078313954,
-0.0134972334979307));
#20075=CARTESIAN_POINT('Ctrl Pts',(0.00526716454226148,-0.0396510092741038,
-0.0135359511054023));
#20076=CARTESIAN_POINT('Ctrl Pts',(0.00535048183107094,-0.0396555850980917,
-0.0135755610499423));
#20077=CARTESIAN_POINT('Ctrl Pts',(0.00536355064413303,-0.0396563069575054,
-0.0135815516412352));
#20078=CARTESIAN_POINT('Ctrl Pts',(0.00538458191855621,-0.0396574780605296,
-0.0135908387312328));
#20079=CARTESIAN_POINT('Ctrl Pts',(0.00539249185925064,-0.0396579206229256,
-0.0135942527633123));
#20080=CARTESIAN_POINT('Ctrl Pts',(0.00540814433960766,-0.0396588012915822,
-0.0136008536289086));
#20081=CARTESIAN_POINT('Ctrl Pts',(0.00541588499099693,-0.039659239183179,
-0.0136040440111532));
#20082=CARTESIAN_POINT('Ctrl Pts',(0.00543591648040582,-0.0396603777493729,
-0.0136121100945936));
#20083=CARTESIAN_POINT('Ctrl Pts',(0.00544824456491845,-0.0396610836405821,
-0.0136168910212299));
#20084=CARTESIAN_POINT('Ctrl Pts',(0.00550703656575312,-0.0396644692349134,
-0.0136388260033595));
#20085=CARTESIAN_POINT('Ctrl Pts',(0.00555424435601024,-0.0396672435708072,
-0.0136538936367112));
#20086=CARTESIAN_POINT('Ctrl Pts',(0.0056790908890079,-0.0396745876573639,
-0.0136872161606285));
#20087=CARTESIAN_POINT('Ctrl Pts',(0.00575756796721962,-0.0396792050576329,
-0.0137017719065238));
#20088=CARTESIAN_POINT('Ctrl Pts',(0.00590530365845703,-0.0396876257641781,
-0.0137174838069692));
#20089=CARTESIAN_POINT('Ctrl Pts',(0.00597420365527438,-0.0396914462293089,
-0.0137201746222118));
#20090=CARTESIAN_POINT('Ctrl Pts',(0.00606475895485893,-0.0396962895632833,
-0.0137176465625296));
#20091=CARTESIAN_POINT('Ctrl Pts',(0.00608644376786908,-0.039697436409106,
-0.0137165829081762));
#20092=CARTESIAN_POINT('Ctrl Pts',(0.0061212705641571,-0.0396992581136982,
-0.0137141369983417));
#20093=CARTESIAN_POINT('Ctrl Pts',(0.00613442928562905,-0.0396999417786248,
-0.0137130429655469));
#20094=CARTESIAN_POINT('Ctrl Pts',(0.00616193989285474,-0.0397013618300341,
-0.0137103997326108));
#20095=CARTESIAN_POINT('Ctrl Pts',(0.00617628738550642,-0.0397020971238992,
-0.0137088177675608));
#20096=CARTESIAN_POINT('Ctrl Pts',(0.00621086968106721,-0.0397038575724294,
-0.0137045127503296));
#20097=CARTESIAN_POINT('Ctrl Pts',(0.00623107696766215,-0.0397048763843797,
-0.0137015889328666));
#20098=CARTESIAN_POINT('Ctrl Pts',(0.00630925560918444,-0.0397087856133673,
-0.0136886882765062));
#20099=CARTESIAN_POINT('Ctrl Pts',(0.00636669824511389,-0.0397115861334585,
-0.0136758006093356));
#20100=CARTESIAN_POINT('Ctrl Pts',(0.00652498748898999,-0.0397192652334389,
-0.01363064738563));
#20101=CARTESIAN_POINT('Ctrl Pts',(0.0066234469541039,-0.0397239839481114,
-0.0135912506289183));
#20102=CARTESIAN_POINT('Ctrl Pts',(0.00675058766311486,-0.0397307704770935,
-0.013524518431139));
#20103=CARTESIAN_POINT('Ctrl Pts',(0.00678341738103955,-0.0397325938957296,
-0.0135057165685662));
#20104=CARTESIAN_POINT('Ctrl Pts',(0.00682618318486149,-0.0397351085568061,
-0.013479090829643));
#20105=CARTESIAN_POINT('Ctrl Pts',(0.00683676361891034,-0.0397357425099431,
-0.013472322867994));
#20106=CARTESIAN_POINT('Ctrl Pts',(0.00685407972656392,-0.0397368016850029,
-0.0134609460484393));
#20107=CARTESIAN_POINT('Ctrl Pts',(0.00686086379646569,-0.039737222234509,
-0.0134564114101728));
#20108=CARTESIAN_POINT('Ctrl Pts',(0.00687487027219414,-0.0397381028137609,
-0.0134468875333432));
#20109=CARTESIAN_POINT('Ctrl Pts',(0.00688208656972172,-0.0397385633348284,
-0.0134418901445758));
#20110=CARTESIAN_POINT('Ctrl Pts',(0.00690163617719632,-0.0397398287761829,
-0.0134281034858799));
#20111=CARTESIAN_POINT('Ctrl Pts',(0.00691388308186435,-0.0397406411248792,
-0.0134191939627801));
#20112=CARTESIAN_POINT('Ctrl Pts',(0.00694138527024765,-0.0397425066346812,
-0.0133985604829386));
#20113=CARTESIAN_POINT('Ctrl Pts',(0.00695655631047808,-0.039743565354146,
-0.0133867286250402));
#20114=CARTESIAN_POINT('Ctrl Pts',(0.00700676473713766,-0.0397471594444508,
-0.0133460387221165));
#20115=CARTESIAN_POINT('Ctrl Pts',(0.00704074826069482,-0.0397497433488598,
-0.0133159199019664));
#20116=CARTESIAN_POINT('Ctrl Pts',(0.0071603379273686,-0.039759277615963,
-0.0132001215302169));
#20117=CARTESIAN_POINT('Ctrl Pts',(0.0072371203506172,-0.0397662490460964,
-0.0131059343680073));
#20118=CARTESIAN_POINT('Ctrl Pts',(0.0073161122185734,-0.0397741937360752,
-0.0129816941172273));
#20119=CARTESIAN_POINT('Ctrl Pts',(0.00732956097787736,-0.0397755834594344,
-0.0129593062415404));
#20120=CARTESIAN_POINT('Ctrl Pts',(0.00735009576582189,-0.0397777677088479,
-0.0129230693359607));
#20121=CARTESIAN_POINT('Ctrl Pts',(0.00735755147133362,-0.0397785752273182,
-0.0129094365657447));
#20122=CARTESIAN_POINT('Ctrl Pts',(0.00737142021085156,-0.0397801063723915,
-0.012883141748329));
#20123=CARTESIAN_POINT('Ctrl Pts',(0.00737786691407778,-0.0397808311277069,
-0.0128704993456897));
#20124=CARTESIAN_POINT('Ctrl Pts',(0.00739246934299865,-0.0397825047471759,
-0.0128408596596795));
#20125=CARTESIAN_POINT('Ctrl Pts',(0.00740048987347598,-0.0397834488966269,
-0.0128237981150153));
#20126=CARTESIAN_POINT('Ctrl Pts',(0.00742678961478523,-0.0397866370344907,
-0.0127650810785836));
#20127=CARTESIAN_POINT('Ctrl Pts',(0.00744353936174462,-0.0397888304224039,
-0.0127227651139747));
#20128=CARTESIAN_POINT('Ctrl Pts',(0.00748269907194559,-0.0397945002806422,
-0.0126094318132611));
#20129=CARTESIAN_POINT('Ctrl Pts',(0.00750188267725668,-0.0397978945657103,
-0.0125374273333806));
#20130=CARTESIAN_POINT('Ctrl Pts',(0.00753033840288857,-0.0398048763289034,
-0.0123879016505579));
#20131=CARTESIAN_POINT('Ctrl Pts',(0.00753908032451722,-0.0398084571103968,
-0.0123105001430206));
#20132=CARTESIAN_POINT('Ctrl Pts',(0.00754257501519921,-0.0398131168772153,
-0.0122158370118193));
#20133=CARTESIAN_POINT('Ctrl Pts',(0.00754292117120714,-0.0398139622688355,
-0.0121988878666902));
#20134=CARTESIAN_POINT('Ctrl Pts',(0.00754302448302113,-0.0398152908681977,
-0.0121726857992518));
#20135=CARTESIAN_POINT('Ctrl Pts',(0.00754297775591906,-0.03981576414013,
-0.0121634345665358));
#20136=CARTESIAN_POINT('Ctrl Pts',(0.00754273467718935,-0.0398166582835102,
-0.0121461269897887));
#20137=CARTESIAN_POINT('Ctrl Pts',(0.0075425584006346,-0.0398170780977159,
-0.0121380709209956));
#20138=CARTESIAN_POINT('Ctrl Pts',(0.00754197839178268,-0.039818103523416,
-0.012118554628847));
#20139=CARTESIAN_POINT('Ctrl Pts',(0.00754150999009453,-0.0398187124954392,
-0.0121070969632715));
#20140=CARTESIAN_POINT('Ctrl Pts',(0.00753929842190308,-0.0398209938810427,
-0.0120646091393436));
#20141=CARTESIAN_POINT('Ctrl Pts',(0.00753674565490548,-0.0398227031046073,
-0.0120336300449794));
#20142=CARTESIAN_POINT('Ctrl Pts',(0.00752714590257337,-0.0398274835599751,
-0.01194859982358));
#20143=CARTESIAN_POINT('Ctrl Pts',(0.00751816807466509,-0.0398306061301149,
-0.0118948123749389));
#20144=CARTESIAN_POINT('Ctrl Pts',(0.00748268635084925,-0.0398400069593393,
-0.0117349013369808));
#20145=CARTESIAN_POINT('Ctrl Pts',(0.00744773233527904,-0.0398462485053601,
-0.01163099120274));
#20146=CARTESIAN_POINT('Ctrl Pts',(0.00739157201136306,-0.0398534939955782,
-0.0115087624520685));
#20147=CARTESIAN_POINT('Ctrl Pts',(0.0073805020312642,-0.0398548320192375,
-0.0114861453157445));
#20148=CARTESIAN_POINT('Ctrl Pts',(0.00736179953917276,-0.0398569554130959,
-0.0114501903906567));
#20149=CARTESIAN_POINT('Ctrl Pts',(0.00735451301810145,-0.0398577525369486,
-0.0114366786591717));
#20150=CARTESIAN_POINT('Ctrl Pts',(0.00734007426627104,-0.0398592761463249,
-0.0114108349169459));
#20151=CARTESIAN_POINT('Ctrl Pts',(0.00733295041468553,-0.0398600035329605,
-0.0113984889224063));
#20152=CARTESIAN_POINT('Ctrl Pts',(0.00731578241728123,-0.0398617014471663,
-0.0113696660092753));
#20153=CARTESIAN_POINT('Ctrl Pts',(0.00730559814277987,-0.039862666806145,
-0.0113532751280467));
#20154=CARTESIAN_POINT('Ctrl Pts',(0.00726855940314006,-0.0398660387756522,
-0.0112960854826945));
#20155=CARTESIAN_POINT('Ctrl Pts',(0.00724007749705524,-0.0398683859785276,
-0.0112563737176329));
#20156=CARTESIAN_POINT('Ctrl Pts',(0.00715693817872098,-0.0398746952289001,
-0.0111513611968108));
#20157=CARTESIAN_POINT('Ctrl Pts',(0.00709869069952535,-0.0398785454628627,
-0.0110891293298039));
#20158=CARTESIAN_POINT('Ctrl Pts',(0.00698514534496306,-0.0398856033503526,
-0.0109863274609203));
#20159=CARTESIAN_POINT('Ctrl Pts',(0.00693171780386809,-0.0398887812087911,
-0.0109440321518834));
#20160=CARTESIAN_POINT('Ctrl Pts',(0.00686406838453483,-0.0398928602024527,
-0.0108974035760309));
#20161=CARTESIAN_POINT('Ctrl Pts',(0.00685234946808485,-0.0398935687622146,
-0.0108895608651134));
#20162=CARTESIAN_POINT('Ctrl Pts',(0.00683334923586824,-0.039894723432986,
-0.0108772188994914));
#20163=CARTESIAN_POINT('Ctrl Pts',(0.00682613487775849,-0.0398951631914547,
-0.0108726175530123));
#20164=CARTESIAN_POINT('Ctrl Pts',(0.00681174510379856,-0.0398960437245047,
-0.0108636071937029));
#20165=CARTESIAN_POINT('Ctrl Pts',(0.00680457115034996,-0.0398964843735361,
-0.0108591964680366));
#20166=CARTESIAN_POINT('Ctrl Pts',(0.00678583756339993,-0.0398976386069337,
-0.0108478888616278));
#20167=CARTESIAN_POINT('Ctrl Pts',(0.00677422331734705,-0.0398983576679461,
-0.0108410842350629));
#20168=CARTESIAN_POINT('Ctrl Pts',(0.00671616944245609,-0.0399019632481599,
-0.0108080838832279));
#20169=CARTESIAN_POINT('Ctrl Pts',(0.00666848577528093,-0.039904959325451,
-0.0107841573085156));
#20170=CARTESIAN_POINT('Ctrl Pts',(0.00654009953284305,-0.0399129450479861,
-0.0107278583691635));
#20171=CARTESIAN_POINT('Ctrl Pts',(0.00645772584742924,-0.0399179801517972,
-0.0106997486032343));
#20172=CARTESIAN_POINT('Ctrl Pts',(0.00636495540209971,-0.0399233618993406,
-0.0106766092341851));
#20173=CARTESIAN_POINT('Ctrl Pts',(0.00635646922346127,-0.0399238517299959,
-0.0106745688798677));
#20174=CARTESIAN_POINT('Ctrl Pts',(0.00629713691159126,-0.0399272586245619,
-0.0106608349055305));
#20175=CARTESIAN_POINT('Ctrl Pts',(0.00624574040996592,-0.0399301170106963,
-0.0106516539867863));
#20176=CARTESIAN_POINT('Ctrl Pts',(0.00617395992439847,-0.0399339707724918,
-0.0106425581697567));
#20177=CARTESIAN_POINT('Ctrl Pts',(0.00615389805821313,-0.0399350332861197,
-0.0106404147793104));
#20178=CARTESIAN_POINT('Ctrl Pts',(0.00611960340003261,-0.0399368254789721,
-0.0106374297180434));
#20179=CARTESIAN_POINT('Ctrl Pts',(0.0061053907983198,-0.0399375611828223,
-0.0106363907676631));
#20180=CARTESIAN_POINT('Ctrl Pts',(0.00607617685179372,-0.0399390595911033,
-0.0106346616909453));
#20181=CARTESIAN_POINT('Ctrl Pts',(0.00606117571367919,-0.0399398215423974,
-0.0106339933708603));
#20182=CARTESIAN_POINT('Ctrl Pts',(0.00602267971937258,-0.0399417589455805,
-0.0106328410473603));
#20183=CARTESIAN_POINT('Ctrl Pts',(0.00599917888313545,-0.039942924538978,
-0.0106326745741643));
#20184=CARTESIAN_POINT('Ctrl Pts',(0.0058730508151825,-0.0399491018858477,
-0.0106346625767733));
#20185=CARTESIAN_POINT('Ctrl Pts',(0.00577083080892855,-0.0399538075807174,
-0.0106465173430247));
#20186=CARTESIAN_POINT('Ctrl Pts',(0.00558761675042572,-0.0399624038705263,
-0.010686560030393));
#20187=CARTESIAN_POINT('Ctrl Pts',(0.00550633429027897,-0.0399662881862747,
-0.0107114947681038));
#20188=CARTESIAN_POINT('Ctrl Pts',(0.00541193466877153,-0.039971291047019,
-0.0107492103923557));
#20189=CARTESIAN_POINT('Ctrl Pts',(0.00539644967006315,-0.0399721284833082,
-0.0107556921202117));
#20190=CARTESIAN_POINT('Ctrl Pts',(0.00537263195242766,-0.0399734471835964,
-0.0107661216566464));
#20191=CARTESIAN_POINT('Ctrl Pts',(0.00536422330733505,-0.0399739187431029,
-0.0107698938545947));
#20192=CARTESIAN_POINT('Ctrl Pts',(0.00534851763882525,-0.0399748117239256,
-0.0107771092681014));
#20193=CARTESIAN_POINT('Ctrl Pts',(0.00534121306705222,-0.0399752321304616,
-0.0107805347342034));
#20194=CARTESIAN_POINT('Ctrl Pts',(0.00532352906560271,-0.0399762619286851,
-0.0107889974257831));
#20195=CARTESIAN_POINT('Ctrl Pts',(0.00531317875105843,-0.0399768747537031,
-0.0107940940238631));
#20196=CARTESIAN_POINT('Ctrl Pts',(0.00527466949984423,-0.0399791900389964,
-0.0108135959370207));
#20197=CARTESIAN_POINT('Ctrl Pts',(0.00524689983696445,-0.0399809306734793,
-0.0108287492368905));
#20198=CARTESIAN_POINT('Ctrl Pts',(0.00517119065911777,-0.0399858369391649,
-0.0108731348803742));
#20199=CARTESIAN_POINT('Ctrl Pts',(0.00512435122326446,-0.0399890567326861,
-0.0109041461924806));
#20200=CARTESIAN_POINT('Ctrl Pts',(0.0049938707845171,-0.0399983893664667,
-0.0110011668572233));
#20201=CARTESIAN_POINT('Ctrl Pts',(0.00491522730228807,-0.0400044608068186,
-0.0110733751208373));
#20202=CARTESIAN_POINT('Ctrl Pts',(0.00482778135832493,-0.040011570750854,
-0.011172160394389));
#20203=CARTESIAN_POINT('Ctrl Pts',(0.0048113949695302,-0.0400129230991725,
-0.0111916205146361));
#20204=CARTESIAN_POINT('Ctrl Pts',(0.00478587034249132,-0.0400150633620491,
-0.0112235007301256));
#20205=CARTESIAN_POINT('Ctrl Pts',(0.00477642451753024,-0.0400158633690262,
-0.0112356675184692));
#20206=CARTESIAN_POINT('Ctrl Pts',(0.00475860274850668,-0.0400173889852931,
-0.0112593466226858));
#20207=CARTESIAN_POINT('Ctrl Pts',(0.00475020088785849,-0.0400181155600753,
-0.0112708373762771));
#20208=CARTESIAN_POINT('Ctrl Pts',(0.00473086249891991,-0.0400198063119157,
-0.0112980684097304));
#20209=CARTESIAN_POINT('Ctrl Pts',(0.00472005774684049,-0.0400207654539418,
-0.011313899601009));
#20210=CARTESIAN_POINT('Ctrl Pts',(0.00468332896438323,-0.0400240821854562,
-0.0113699289774251));
#20211=CARTESIAN_POINT('Ctrl Pts',(0.00465898039820578,-0.0400263830975167,
-0.0114111288024565));
#20212=CARTESIAN_POINT('Ctrl Pts',(0.00461716318795908,-0.0400305948554303,
-0.011490045922268));
#20213=CARTESIAN_POINT('Ctrl Pts',(0.004599227949821,-0.0400325153987042,
-0.0115274651103423));
#20214=CARTESIAN_POINT('Ctrl Pts',(0.00454276940954693,-0.0400390806108443,
-0.0116585694926437));
#20215=CARTESIAN_POINT('Ctrl Pts',(0.00451197370351692,-0.0400436332411471,
-0.0117552849964633));
#20216=CARTESIAN_POINT('Ctrl Pts',(0.0044864692753042,-0.0400495937006845,
-0.0118749866806608));
#20217=CARTESIAN_POINT('Ctrl Pts',(0.00448248922326357,-0.04005063973444,
-0.011895751640434));
#20218=CARTESIAN_POINT('Ctrl Pts',(0.00447726486689411,-0.0400522098437399,
-0.0119264023368553));
#20219=CARTESIAN_POINT('Ctrl Pts',(0.00447568753151272,-0.0400527171684212,
-0.0119362295185568));
#20220=CARTESIAN_POINT('Ctrl Pts',(0.00447302054450397,-0.0400536395276828,
-0.0119539387802783));
#20221=CARTESIAN_POINT('Ctrl Pts',(0.00447189662110966,-0.0400540527083957,
-0.0119618150605848));
#20222=CARTESIAN_POINT('Ctrl Pts',(0.00446979058969465,-0.0400548780374543,
-0.0119774367808808));
#20223=CARTESIAN_POINT('Ctrl Pts',(0.0044688062873025,-0.0400552899753772,
-0.0119851814262938));
#20224=CARTESIAN_POINT('Ctrl Pts',(0.00446664725485208,-0.0400562577788002,
-0.012003265237146));
#20225=CARTESIAN_POINT('Ctrl Pts',(0.00446551826907159,-0.0400568158812481,
-0.0120136093883288));
#20226=CARTESIAN_POINT('Ctrl Pts',(0.00445951735299476,-0.0400601122539036,
-0.0120742748694939));
#20227=CARTESIAN_POINT('Ctrl Pts',(0.00445701705122449,-0.0400629496465278,
-0.0121247865047283));
#20228=CARTESIAN_POINT('Ctrl Pts',(0.00445700008689307,-0.0400658264344116,
-0.0121753354525968));
#20229=CARTESIAN_POINT('Ctrl Pts',(0.004457,-0.0401812248373849,-0.0121758532940426));
#20230=CARTESIAN_POINT('Ctrl Pts',(0.00445699999994688,-0.040180635876834,
-0.0121649030018824));
#20231=CARTESIAN_POINT('Ctrl Pts',(0.00445711656713364,-0.0401800501844204,
-0.0121539516973495));
#20232=CARTESIAN_POINT('Ctrl Pts',(0.00445777372115888,-0.0401784091749531,
-0.0121230933874333));
#20233=CARTESIAN_POINT('Ctrl Pts',(0.00445858301204432,-0.0401773619855601,
-0.012103195046473));
#20234=CARTESIAN_POINT('Ctrl Pts',(0.00446065838074593,-0.0401755624340552,
-0.0120686513996819));
#20235=CARTESIAN_POINT('Ctrl Pts',(0.00446174894820756,-0.0401748048444127,
-0.0120539985110329));
#20236=CARTESIAN_POINT('Ctrl Pts',(0.00446444969679944,-0.0401732437697908,
-0.012023586661551));
#20237=CARTESIAN_POINT('Ctrl Pts',(0.00446609359473845,-0.0401724414087836,
-0.0120078323887594));
#20238=CARTESIAN_POINT('Ctrl Pts',(0.00447108784806639,-0.0401703359124529,
-0.0119661920993181));
#20239=CARTESIAN_POINT('Ctrl Pts',(0.00447485297155762,-0.0401690454846411,
-0.0119403605706036));
#20240=CARTESIAN_POINT('Ctrl Pts',(0.00449363255762831,-0.040163635408136,
-0.0118310314728741));
#20241=CARTESIAN_POINT('Ctrl Pts',(0.00451486408403274,-0.0401597022010732,
-0.0117487493909857));
#20242=CARTESIAN_POINT('Ctrl Pts',(0.00456560682539897,-0.0401525996094248,
-0.0116029669746973));
#20243=CARTESIAN_POINT('Ctrl Pts',(0.00459287161515518,-0.0401494252726806,
-0.0115389299110801));
#20244=CARTESIAN_POINT('Ctrl Pts',(0.00463545219743835,-0.0401449590151719,
-0.0114551189031115));
#20245=CARTESIAN_POINT('Ctrl Pts',(0.00464706271274058,-0.0401437798563536,
-0.0114335532385743));
#20246=CARTESIAN_POINT('Ctrl Pts',(0.00466819035336545,-0.0401416834719464,
-0.0113964538337312));
#20247=CARTESIAN_POINT('Ctrl Pts',(0.00467747860489835,-0.0401407768206006,
-0.0113807950814925));
#20248=CARTESIAN_POINT('Ctrl Pts',(0.00469206472575814,-0.0401393696196115,
-0.0113571678985893));
#20249=CARTESIAN_POINT('Ctrl Pts',(0.00469716351239956,-0.040138880626556,
-0.011349077909768));
#20250=CARTESIAN_POINT('Ctrl Pts',(0.00470682864741006,-0.0401379580718214,
-0.0113340541572903));
#20251=CARTESIAN_POINT('Ctrl Pts',(0.004711376262438,-0.0401375256410104,
-0.0113271090535379));
#20252=CARTESIAN_POINT('Ctrl Pts',(0.00472151994265341,-0.0401365650275842,
-0.0113118871058551));
#20253=CARTESIAN_POINT('Ctrl Pts',(0.00472714076799248,-0.040136035341946,
-0.0113036272929654));
#20254=CARTESIAN_POINT('Ctrl Pts',(0.00474687769987846,-0.0401341859482964,
-0.0112752209307432));
#20255=CARTESIAN_POINT('Ctrl Pts',(0.00476139455948665,-0.0401328439239363,
-0.0112553585387399));
#20256=CARTESIAN_POINT('Ctrl Pts',(0.00485138826466713,-0.0401246706679953,
-0.0111382116256438));
#20257=CARTESIAN_POINT('Ctrl Pts',(0.00493781437787786,-0.0401174555169388,
-0.0110498989300811));
#20258=CARTESIAN_POINT('Ctrl Pts',(0.00507814701859921,-0.0401073656540049,
-0.0109371975835703));
#20259=CARTESIAN_POINT('Ctrl Pts',(0.00512440831636699,-0.0401042452452582,
-0.0109040745734365));
#20260=CARTESIAN_POINT('Ctrl Pts',(0.00518973768218066,-0.0401001228971598,
-0.0108625573745158));
#20261=CARTESIAN_POINT('Ctrl Pts',(0.00520729797308878,-0.0400990408257882,
-0.0108518839794864));
#20262=CARTESIAN_POINT('Ctrl Pts',(0.00523785311293039,-0.0400972014413967,
-0.0108341380561172));
#20263=CARTESIAN_POINT('Ctrl Pts',(0.00525074580059029,-0.0400964382313293,
-0.010826895984981));
#20264=CARTESIAN_POINT('Ctrl Pts',(0.00527745433556961,-0.040094882828721,
-0.0108123943536786));
#20265=CARTESIAN_POINT('Ctrl Pts',(0.00529128023460196,-0.0400940914597302,
-0.0108051568156108));
#20266=CARTESIAN_POINT('Ctrl Pts',(0.00532747939285731,-0.0400920536339528,
-0.0107869015718927));
#20267=CARTESIAN_POINT('Ctrl Pts',(0.00535001451932294,-0.0400908183803772,
-0.0107762141216076));
#20268=CARTESIAN_POINT('Ctrl Pts',(0.00549015401438133,-0.0400833203332449,
-0.0107138669531677));
#20269=CARTESIAN_POINT('Ctrl Pts',(0.00561356201952419,-0.0400775535039627,
-0.0106765157152171));
#20270=CARTESIAN_POINT('Ctrl Pts',(0.00578060631355024,-0.0400696932359926,
-0.0106479796427833));
#20271=CARTESIAN_POINT('Ctrl Pts',(0.00582129599906705,-0.0400677695528663,
-0.0106426879218692));
#20272=CARTESIAN_POINT('Ctrl Pts',(0.00588027475748021,-0.0400649120757031,
-0.0106373975153975));
#20273=CARTESIAN_POINT('Ctrl Pts',(0.00589843020376616,-0.0400640230111768,
-0.010636092322633));
#20274=CARTESIAN_POINT('Ctrl Pts',(0.00593117556479208,-0.0400623960117224,
-0.010634319909139));
#20275=CARTESIAN_POINT('Ctrl Pts',(0.0059457572392941,-0.0400616631311297,
-0.01063373796952));
#20276=CARTESIAN_POINT('Ctrl Pts',(0.00596915687348503,-0.0400604706216501,
-0.0106331363937962));
#20277=CARTESIAN_POINT('Ctrl Pts',(0.00597797084470707,-0.0400600176993975,
-0.0106329853665039));
#20278=CARTESIAN_POINT('Ctrl Pts',(0.0059954724680324,-0.0400591100979294,
-0.0106328354733705));
#20279=CARTESIAN_POINT('Ctrl Pts',(0.006004159746182,-0.0400586555405356,
-0.0106328344407947));
#20280=CARTESIAN_POINT('Ctrl Pts',(0.00602683198172644,-0.0400574594727238,
-0.0106330232061765));
#20281=CARTESIAN_POINT('Ctrl Pts',(0.00604081494898436,-0.0400567121197253,
-0.0106333297937456));
#20282=CARTESIAN_POINT('Ctrl Pts',(0.00611047336862383,-0.0400529471792749,
-0.0106358048982512));
#20283=CARTESIAN_POINT('Ctrl Pts',(0.00616600341077887,-0.0400498137250025,
-0.0106407978045264));
#20284=CARTESIAN_POINT('Ctrl Pts',(0.00631317247337864,-0.0400413477464493,
-0.0106621095352319));
#20285=CARTESIAN_POINT('Ctrl Pts',(0.00640382166846383,-0.0400359749604104,
-0.0106837315845034));
#20286=CARTESIAN_POINT('Ctrl Pts',(0.00654034606368712,-0.0400279427671415,
-0.0107296583363048));
#20287=CARTESIAN_POINT('Ctrl Pts',(0.00658788455097591,-0.0400251545052496,
-0.0107483217770079));
#20288=CARTESIAN_POINT('Ctrl Pts',(0.00665254565948249,-0.0400213833228971,
-0.0107774868128229));
#20289=CARTESIAN_POINT('Ctrl Pts',(0.0066705178407242,-0.0400203373203879,
-0.0107860149843751));
#20290=CARTESIAN_POINT('Ctrl Pts',(0.00670146240920835,-0.0400185394075941,
-0.0108014388294517));
#20291=CARTESIAN_POINT('Ctrl Pts',(0.0067145102467585,-0.0400177822852743,
-0.0108081765199103));
#20292=CARTESIAN_POINT('Ctrl Pts',(0.00674142551479173,-0.0400162218421084,
-0.0108225654478264));
#20293=CARTESIAN_POINT('Ctrl Pts',(0.00675527535502652,-0.04001541965048,
-0.010830246014736));
#20294=CARTESIAN_POINT('Ctrl Pts',(0.00679163995331315,-0.0400133139068312,
-0.0108511507358057));
#20295=CARTESIAN_POINT('Ctrl Pts',(0.00681394187386847,-0.0400120230857595,
-0.0108647356771748));
#20296=CARTESIAN_POINT('Ctrl Pts',(0.00691081761335415,-0.0400064025696993,
-0.0109271713596999));
#20297=CARTESIAN_POINT('Ctrl Pts',(0.00698142414794439,-0.0400022822898413,
-0.0109818669012067));
#20298=CARTESIAN_POINT('Ctrl Pts',(0.00709568112485136,-0.0399951303186407,
-0.011087396244405));
#20299=CARTESIAN_POINT('Ctrl Pts',(0.00714148773392469,-0.0399920927442163,
-0.0111355356218492));
#20300=CARTESIAN_POINT('Ctrl Pts',(0.00720640262278176,-0.0399872773634287,
-0.0112132230588179));
#20301=CARTESIAN_POINT('Ctrl Pts',(0.00722784099519396,-0.0399855870549997,
-0.0112407220454935));
#20302=CARTESIAN_POINT('Ctrl Pts',(0.0072554478415355,-0.0399832360743122,
-0.0112787209489036));
#20303=CARTESIAN_POINT('Ctrl Pts',(0.00726245141971938,-0.0399826232967991,
-0.0112886035416483));
#20304=CARTESIAN_POINT('Ctrl Pts',(0.00727407806896822,-0.0399815761320524,
-0.0113054260421249));
#20305=CARTESIAN_POINT('Ctrl Pts',(0.0072787626604972,-0.0399811456516794,
-0.0113123229914047));
#20306=CARTESIAN_POINT('Ctrl Pts',(0.00728862644620145,-0.0399802202154735,
-0.0113271013709235));
#20307=CARTESIAN_POINT('Ctrl Pts',(0.00729378957255423,-0.0399797243538421,
-0.0113349927361226));
#20308=CARTESIAN_POINT('Ctrl Pts',(0.00730835703616764,-0.0399782932379673,
-0.011357709597066));
#20309=CARTESIAN_POINT('Ctrl Pts',(0.0073175808687332,-0.0399773476903546,
-0.0113726485580136));
#20310=CARTESIAN_POINT('Ctrl Pts',(0.00736161887512091,-0.0399726468634982,
-0.0114467731550022));
#20311=CARTESIAN_POINT('Ctrl Pts',(0.00739270856398766,-0.0399687341462472,
-0.0115080768070202));
#20312=CARTESIAN_POINT('Ctrl Pts',(0.00744439709768179,-0.0399611849860902,
-0.0116294400717559));
#20313=CARTESIAN_POINT('Ctrl Pts',(0.0074655823188274,-0.0399575580285109,
-0.0116891095720938));
#20314=CARTESIAN_POINT('Ctrl Pts',(0.00749938259972236,-0.0399506805880792,
-0.0118067958176241));
#20315=CARTESIAN_POINT('Ctrl Pts',(0.00751243480359684,-0.0399474262906029,
-0.0118645757499254));
#20316=CARTESIAN_POINT('Ctrl Pts',(0.00752554220004797,-0.0399431644909464,
-0.0119434701026485));
#20317=CARTESIAN_POINT('Ctrl Pts',(0.00752853395107985,-0.039942069425714,
-0.0119640397747039));
#20318=CARTESIAN_POINT('Ctrl Pts',(0.00753294634577703,-0.0399402149959359,
-0.0119993757981228));
#20319=CARTESIAN_POINT('Ctrl Pts',(0.00753457127847003,-0.0399394494838702,
-0.012014113328108));
#20320=CARTESIAN_POINT('Ctrl Pts',(0.0075374631236616,-0.0399378952565843,
-0.0120443337523687));
#20321=CARTESIAN_POINT('Ctrl Pts',(0.00753870914690623,-0.0399371072633642,
-0.0120598169649866));
#20322=CARTESIAN_POINT('Ctrl Pts',(0.00754132194703761,-0.0399350907907916,
-0.0120998320952297));
#20323=CARTESIAN_POINT('Ctrl Pts',(0.007542337009579,-0.0399338730479364,
-0.0121243829473209));
#20324=CARTESIAN_POINT('Ctrl Pts',(0.00754490271431925,-0.0399266743253487,
-0.0122715044133184));
#20325=CARTESIAN_POINT('Ctrl Pts',(0.00753242995617212,-0.0399211404017791,
-0.012393874190513));
#20326=CARTESIAN_POINT('Ctrl Pts',(0.00749217880680639,-0.0399126362877349,
-0.0125733680256522));
#20327=CARTESIAN_POINT('Ctrl Pts',(0.00747518974740928,-0.0399097642755847,
-0.012632394223254));
#20328=CARTESIAN_POINT('Ctrl Pts',(0.00744905518544103,-0.0399059028752394,
-0.0127063041713141));
#20329=CARTESIAN_POINT('Ctrl Pts',(0.00744311209893908,-0.0399050525535822,
-0.0127222656748768));
#20330=CARTESIAN_POINT('Ctrl Pts',(0.0074335084510247,-0.0399037149184896,
-0.0127468081573597));
#20331=CARTESIAN_POINT('Ctrl Pts',(0.00743003208281494,-0.0399032374733162,
-0.0127554602028076));
#20332=CARTESIAN_POINT('Ctrl Pts',(0.0074233200266341,-0.0399023271763452,
-0.0127717372565016));
#20333=CARTESIAN_POINT('Ctrl Pts',(0.00742010101824096,-0.0399018952470575,
-0.0127793685643752));
#20334=CARTESIAN_POINT('Ctrl Pts',(0.00741274011529055,-0.0399009182254969,
-0.0127964340823686));
#20335=CARTESIAN_POINT('Ctrl Pts',(0.00740856484944494,-0.0399003712909099,
-0.0128058534543916));
#20336=CARTESIAN_POINT('Ctrl Pts',(0.00739312779361206,-0.0398983766293991,
-0.0128397586440691));
#20337=CARTESIAN_POINT('Ctrl Pts',(0.00738131974608067,-0.0398969018330847,
-0.0128639891576903));
#20338=CARTESIAN_POINT('Ctrl Pts',(0.00732765508390651,-0.0398904450897122,
-0.0129671580048346));
#20339=CARTESIAN_POINT('Ctrl Pts',(0.00727962126404893,-0.039885271311129,
-0.0130426866370688));
#20340=CARTESIAN_POINT('Ctrl Pts',(0.00717863886218274,-0.0398758059130695,
-0.0131746324503401));
#20341=CARTESIAN_POINT('Ctrl Pts',(0.00712746031583675,-0.0398715040160061,
-0.0132320657976271));
#20342=CARTESIAN_POINT('Ctrl Pts',(0.00705385904613277,-0.0398659924820446,
-0.0133031870515126));
#20343=CARTESIAN_POINT('Ctrl Pts',(0.00703506883535958,-0.039864636398005,
-0.0133204636630728));
#20344=CARTESIAN_POINT('Ctrl Pts',(0.00700402551975165,-0.0398624758327834,
-0.0133476164342518));
#20345=CARTESIAN_POINT('Ctrl Pts',(0.00699203535755855,-0.0398616596414898,
-0.0133577847531852));
#20346=CARTESIAN_POINT('Ctrl Pts',(0.00696851150286872,-0.039860092689147,
-0.0133771240743346));
#20347=CARTESIAN_POINT('Ctrl Pts',(0.00695699776118241,-0.0398593411221649,
-0.0133863165619317));
#20348=CARTESIAN_POINT('Ctrl Pts',(0.00692938492235703,-0.0398575737479358,
-0.0134077221586867));
#20349=CARTESIAN_POINT('Ctrl Pts',(0.00691317393719463,-0.0398565636789652,
-0.0134197868294619));
#20350=CARTESIAN_POINT('Ctrl Pts',(0.006856337959408,-0.0398531110049468,
-0.0134603757301412));
#20351=CARTESIAN_POINT('Ctrl Pts',(0.00681457572317758,-0.0398507277201316,
-0.0134872569363371));
#20352=CARTESIAN_POINT('Ctrl Pts',(0.00675858267759054,-0.0398476823092097,
-0.0135195894390562));
#20353=CARTESIAN_POINT('Ctrl Pts',(0.00674546852423048,-0.039846979168207,
-0.0135269088797831));
#20354=CARTESIAN_POINT('Ctrl Pts',(0.00666072847975548,-0.0398424922417613,
-0.0135725955613202));
#20355=CARTESIAN_POINT('Ctrl Pts',(0.00658627531055629,-0.0398388137929522,
-0.0136054448366188));
#20356=CARTESIAN_POINT('Ctrl Pts',(0.00645894969104511,-0.0398325273369262,
-0.0136499943157336));
#20357=CARTESIAN_POINT('Ctrl Pts',(0.00640743064427633,-0.0398299823707053,
-0.0136650564178983));
#20358=CARTESIAN_POINT('Ctrl Pts',(0.00634191545618927,-0.039826632122965,
-0.0136805559830389));
#20359=CARTESIAN_POINT('Ctrl Pts',(0.0063285534186693,-0.039825942951924,
-0.0136835299797456));
#20360=CARTESIAN_POINT('Ctrl Pts',(0.0063067092707106,-0.0398248042146958,
-0.0136880876736485));
#20361=CARTESIAN_POINT('Ctrl Pts',(0.00629825002464187,-0.0398243602948811,
-0.0136897787592414));
#20362=CARTESIAN_POINT('Ctrl Pts',(0.00628212820246123,-0.0398235079476141,
-0.0136928613032737));
#20363=CARTESIAN_POINT('Ctrl Pts',(0.00627446844570021,-0.039823100309428,
-0.0136942658499429));
#20364=CARTESIAN_POINT('Ctrl Pts',(0.00625325197977236,-0.0398219644512678,
-0.0136979904682242));
#20365=CARTESIAN_POINT('Ctrl Pts',(0.00623967466098199,-0.0398212299600893,
-0.0137001873040588));
#20366=CARTESIAN_POINT('Ctrl Pts',(0.00617655564368029,-0.0398177858692261,
-0.0137095359735397));
#20367=CARTESIAN_POINT('Ctrl Pts',(0.0061267169227291,-0.0398149830453155,
-0.0137144554332848));
#20368=CARTESIAN_POINT('Ctrl Pts',(0.00597919315170565,-0.0398065984356224,
-0.0137218006900586));
#20369=CARTESIAN_POINT('Ctrl Pts',(0.00588140606231653,-0.0398009426043927,
-0.0137173862474833));
#20370=CARTESIAN_POINT('Ctrl Pts',(0.005733039400861,-0.0397925784840061,
-0.0136964788117756));
#20371=CARTESIAN_POINT('Ctrl Pts',(0.00568178605135361,-0.039789726027195,
-0.0136865851071324));
#20372=CARTESIAN_POINT('Ctrl Pts',(0.00561168269060878,-0.0397858863281619,
-0.0136693256571105));
#20373=CARTESIAN_POINT('Ctrl Pts',(0.00559233151436458,-0.0397848328648956,
-0.0136641598778057));
#20374=CARTESIAN_POINT('Ctrl Pts',(0.00555895494323796,-0.0397830263723816,
-0.0136545501759719));
#20375=CARTESIAN_POINT('Ctrl Pts',(0.00554488270501247,-0.0397822679915335,
-0.0136502797852558));
#20376=CARTESIAN_POINT('Ctrl Pts',(0.00551583512666037,-0.0397807087042385,
-0.0136410094409908));
#20377=CARTESIAN_POINT('Ctrl Pts',(0.00550087112188317,-0.0397799088613901,
-0.0136359795029228));
#20378=CARTESIAN_POINT('Ctrl Pts',(0.00546161193663416,-0.0397778180029361,
-0.0136221089962299));
#20379=CARTESIAN_POINT('Ctrl Pts',(0.00543745679896261,-0.0397765393748755,
-0.0136128858279032));
#20380=CARTESIAN_POINT('Ctrl Pts',(0.00531892205585882,-0.0397702865112573,
-0.0135641784941042));
#20381=CARTESIAN_POINT('Ctrl Pts',(0.00522840109744926,-0.0397656017609241,
-0.0135159842058499));
#20382=CARTESIAN_POINT('Ctrl Pts',(0.00507633818917478,-0.0397571924103273,
-0.0134144743131082));
#20383=CARTESIAN_POINT('Ctrl Pts',(0.00501297346377977,-0.0397534808957977,
-0.0133645961004026));
#20384=CARTESIAN_POINT('Ctrl Pts',(0.00494186653268372,-0.0397487051032339,
-0.0132990033099942));
#20385=CARTESIAN_POINT('Ctrl Pts',(0.00493011182557243,-0.0397478933174103,
-0.0132878117686894));
#20386=CARTESIAN_POINT('Ctrl Pts',(0.00491200330152067,-0.0397466032932837,
-0.0132700178415358));
#20387=CARTESIAN_POINT('Ctrl Pts',(0.00490552777759662,-0.0397461338312949,
-0.0132635404822358));
#20388=CARTESIAN_POINT('Ctrl Pts',(0.00489325716545176,-0.0397452276129151,
-0.0132510458658604));
#20389=CARTESIAN_POINT('Ctrl Pts',(0.00488745264133763,-0.0397447915660869,
-0.0132450385595528));
#20390=CARTESIAN_POINT('Ctrl Pts',(0.00487294553290927,-0.0397436836556677,
-0.0132297786035136));
#20391=CARTESIAN_POINT('Ctrl Pts',(0.00486430797121918,-0.0397430072770849,
-0.0132204651480586));
#20392=CARTESIAN_POINT('Ctrl Pts',(0.00483076022009553,-0.0397403173538923,
-0.0131833843526046));
#20393=CARTESIAN_POINT('Ctrl Pts',(0.00480674668489662,-0.0397382524129708,
-0.013154825542188));
#20394=CARTESIAN_POINT('Ctrl Pts',(0.00472347268414423,-0.0397306466650612,
-0.0130481688067163));
#20395=CARTESIAN_POINT('Ctrl Pts',(0.00467065057179523,-0.0397249525323384,
-0.0129653388406234));
#20396=CARTESIAN_POINT('Ctrl Pts',(0.00459696386158113,-0.0397158252805594,
-0.012821160322121));
#20397=CARTESIAN_POINT('Ctrl Pts',(0.00457144578840077,-0.0397122995917525,
-0.0127625097948082));
#20398=CARTESIAN_POINT('Ctrl Pts',(0.00454239645416376,-0.0397077587772761,
-0.0126825000409533));
#20399=CARTESIAN_POINT('Ctrl Pts',(0.00453556845015233,-0.0397066400393274,
-0.0126624119417765));
#20400=CARTESIAN_POINT('Ctrl Pts',(0.00452465390485401,-0.0397047581673804,
-0.0126279869665255));
#20401=CARTESIAN_POINT('Ctrl Pts',(0.00452035701400596,-0.0397039884222852,
-0.0126137204116534));
#20402=CARTESIAN_POINT('Ctrl Pts',(0.00451203753660726,-0.0397024358429424,
-0.0125845758833694));
#20403=CARTESIAN_POINT('Ctrl Pts',(0.00450802986865213,-0.0397016535540137,
-0.012569695390064));
#20404=CARTESIAN_POINT('Ctrl Pts',(0.00449836542478563,-0.0396996730797273,
-0.0125315441848174));
#20405=CARTESIAN_POINT('Ctrl Pts',(0.0044930261482904,-0.0396984848640402,
-0.0125081969313366));
#20406=CARTESIAN_POINT('Ctrl Pts',(0.00446744827644895,-0.0396922254360072,
-0.0123830101099512));
#20407=CARTESIAN_POINT('Ctrl Pts',(0.004457,-0.039687465566661,-0.012279527802194));
#20408=CARTESIAN_POINT('Ctrl Pts',(0.004457,-0.0396826982119552,-0.0121758532865581));
#20409=CARTESIAN_POINT('Origin',(0.006,-0.0418165664398416,-0.0121758532865581));
#20410=CARTESIAN_POINT('',(0.00445636205606274,-0.040683589227672,-0.0121761473112929));
#20411=CARTESIAN_POINT('',(0.004457,-0.0405679692773165,-0.0121758532865581));
#20412=CARTESIAN_POINT('',(0.004457,-0.0418165664398416,-0.0121758532865581));
#20413=CARTESIAN_POINT('',(0.0066708408081921,-0.0408432743898683,-0.0135653933579799));
#20414=CARTESIAN_POINT('Ctrl Pts',(0.00445636205606274,-0.040683589227672,
-0.0121761473112929));
#20415=CARTESIAN_POINT('Ctrl Pts',(0.00445634241712689,-0.0406848802299932,
-0.0122003684416047));
#20416=CARTESIAN_POINT('Ctrl Pts',(0.00445690191082416,-0.0406861511658211,
-0.0122245773757201));
#20417=CARTESIAN_POINT('Ctrl Pts',(0.00445805707381056,-0.0406874049684561,
-0.0122487525271755));
#20418=CARTESIAN_POINT('Ctrl Pts',(0.00447278947892899,-0.0407033953772335,
-0.0125570710322108));
#20419=CARTESIAN_POINT('Ctrl Pts',(0.00458498283471403,-0.0407165990291478,
-0.0128616719032148));
#20420=CARTESIAN_POINT('Ctrl Pts',(0.00477117346292667,-0.040733100744054,
-0.0131079829187817));
#20421=CARTESIAN_POINT('Ctrl Pts',(0.00488365821068625,-0.0407430700494731,
-0.0132567886493516));
#20422=CARTESIAN_POINT('Ctrl Pts',(0.00502283501146244,-0.0407539848137185,
-0.0133847978149439));
#20423=CARTESIAN_POINT('Ctrl Pts',(0.00517953498196645,-0.0407638089246862,
-0.0134832713791425));
#20424=CARTESIAN_POINT('Ctrl Pts',(0.0051898898536264,-0.0407644581105662,
-0.0134897785987412));
#20425=CARTESIAN_POINT('Ctrl Pts',(0.0052003241170997,-0.0407651027688879,
-0.0134961588328292));
#20426=CARTESIAN_POINT('Ctrl Pts',(0.00521083657242243,-0.0407657432364286,
-0.0135024085181948));
#20427=CARTESIAN_POINT('Ctrl Pts',(0.00548429690826446,-0.0407824037085456,
-0.0136649814858335));
#20428=CARTESIAN_POINT('Ctrl Pts',(0.00581290359061553,-0.0407962283824575,
-0.0137394857874055));
#20429=CARTESIAN_POINT('Ctrl Pts',(0.00613310254693832,-0.0408131453283747,
-0.0137122202173662));
#20430=CARTESIAN_POINT('Ctrl Pts',(0.00631937727002341,-0.0408229867077857,
-0.0136963585588301));
#20431=CARTESIAN_POINT('Ctrl Pts',(0.00650283936617522,-0.0408336528440328,
-0.0136465014534069));
#20432=CARTESIAN_POINT('Ctrl Pts',(0.00667084080819075,-0.0408432743898699,
-0.0135653933579773));
#20433=CARTESIAN_POINT('',(0.00745756139467092,-0.0408425303804537,-0.0116656133925582));
#20434=CARTESIAN_POINT('Origin',(0.00600000000001,-0.0408432743898623,-0.0121758532865681));
#20435=CARTESIAN_POINT('Ctrl Pts',(0.00745636084418434,-0.0408417813214044,
-0.0116660865835196));
#20436=CARTESIAN_POINT('Ctrl Pts',(0.00746165020059864,-0.0408409726501889,
-0.0116811978325024));
#20437=CARTESIAN_POINT('Ctrl Pts',(0.00746670423706467,-0.0408401763062786,
-0.0116963910408018));
#20438=CARTESIAN_POINT('Ctrl Pts',(0.00748091109636588,-0.0408378574212748,
-0.0117414277196461));
#20439=CARTESIAN_POINT('Ctrl Pts',(0.00748939621149823,-0.0408363637400495,
-0.0117714743038455));
#20440=CARTESIAN_POINT('Ctrl Pts',(0.00752140454363981,-0.0408301444250377,
-0.0118995578575828));
#20441=CARTESIAN_POINT('Ctrl Pts',(0.0075362026694581,-0.0408256370371514,
-0.0119995186528621));
#20442=CARTESIAN_POINT('Ctrl Pts',(0.00754416486380153,-0.0408180759448483,
-0.0121617431562191));
#20443=CARTESIAN_POINT('Ctrl Pts',(0.00754349702246392,-0.0408151493490006,
-0.0122233951850473));
#20444=CARTESIAN_POINT('Ctrl Pts',(0.00753767474856551,-0.0408110849046505,
-0.0123056198926866));
#20445=CARTESIAN_POINT('Ctrl Pts',(0.0075357826221537,-0.0408100457985166,
-0.0123263680387618));
#20446=CARTESIAN_POINT('Ctrl Pts',(0.00753184734665668,-0.0408082549074869,
-0.0123616134192528));
#20447=CARTESIAN_POINT('Ctrl Pts',(0.00753001687733962,-0.0408075097373047,
-0.012376131734187));
#20448=CARTESIAN_POINT('Ctrl Pts',(0.0075258757163216,-0.0408059815367131,
-0.0124055942499645));
#20449=CARTESIAN_POINT('Ctrl Pts',(0.0075235512818924,-0.0408051981562626,
-0.0124205348799674));
#20450=CARTESIAN_POINT('Ctrl Pts',(0.00751706407621937,-0.0408031828835839,
-0.0124585458506635));
#20451=CARTESIAN_POINT('Ctrl Pts',(0.00751259453575199,-0.0408019416868216,
-0.0124815593366645));
#20452=CARTESIAN_POINT('Ctrl Pts',(0.00747958573376826,-0.0407936319400856,
-0.0126329986075741));
#20453=CARTESIAN_POINT('Ctrl Pts',(0.00743524769199549,-0.0407860585052013,
-0.0127574112264761));
#20454=CARTESIAN_POINT('Ctrl Pts',(0.00734999191524783,-0.0407753584871154,
-0.0129252458452654));
#20455=CARTESIAN_POINT('Ctrl Pts',(0.00732152704022689,-0.0407721704481418,
-0.0129743735538654));
#20456=CARTESIAN_POINT('Ctrl Pts',(0.00728286616919027,-0.040768366246518,
-0.0130333456575354));
#20457=CARTESIAN_POINT('Ctrl Pts',(0.00727515915993375,-0.0407676307868667,
-0.0130447652015192));
#20458=CARTESIAN_POINT('Ctrl Pts',(0.00726238827445254,-0.0407664505745708,
-0.0130631519834363));
#20459=CARTESIAN_POINT('Ctrl Pts',(0.00725741732687933,-0.0407660002590344,
-0.0130701825356703));
#20460=CARTESIAN_POINT('Ctrl Pts',(0.00724733488458996,-0.0407651054820061,
-0.0130841921601766));
#20461=CARTESIAN_POINT('Ctrl Pts',(0.00724222307824382,-0.0407646611126685,
-0.0130911705275256));
#20462=CARTESIAN_POINT('Ctrl Pts',(0.00722847101029089,-0.0407634890257665,
-0.0131096167086333));
#20463=CARTESIAN_POINT('Ctrl Pts',(0.00721972869714755,-0.0407627678562672,
-0.0131210078158341));
#20464=CARTESIAN_POINT('Ctrl Pts',(0.00716322392993987,-0.040758244510328,
-0.0131925427162463));
#20465=CARTESIAN_POINT('Ctrl Pts',(0.00711118158793278,-0.0407546851745562,
-0.0132491775622032));
#20466=CARTESIAN_POINT('Ctrl Pts',(0.00699813863725094,-0.040747559827924,
-0.0133551199350694));
#20467=CARTESIAN_POINT('Ctrl Pts',(0.00693717047657244,-0.0407440025590901,
-0.0134041291692879));
#20468=CARTESIAN_POINT('Ctrl Pts',(0.00683427346338951,-0.0407381054263292,
-0.0134747044620498));
#20469=CARTESIAN_POINT('Ctrl Pts',(0.00679461576248002,-0.0407358566580044,
-0.0134993380470959));
#20470=CARTESIAN_POINT('Ctrl Pts',(0.00673730244404835,-0.0407326016624396,
-0.0135314329339307));
#20471=CARTESIAN_POINT('Ctrl Pts',(0.00672053004103239,-0.0407316486708917,
-0.0135404218977194));
#20472=CARTESIAN_POINT('Ctrl Pts',(0.00669092545955046,-0.040729963705574,
-0.0135555901095967));
#20473=CARTESIAN_POINT('Ctrl Pts',(0.00667816582828285,-0.0407292365820017,
-0.0135619062376694));
#20474=CARTESIAN_POINT('Ctrl Pts',(0.00665132981715593,-0.0407277046601286,
-0.0135747310244224));
#20475=CARTESIAN_POINT('Ctrl Pts',(0.00663723910326167,-0.0407268988074884,
-0.0135812058253447));
#20476=CARTESIAN_POINT('Ctrl Pts',(0.00659939737363555,-0.0407247298313373,
-0.0135979082863153));
#20477=CARTESIAN_POINT('Ctrl Pts',(0.00657548352317444,-0.040723354125781,
-0.0136077528087148));
#20478=CARTESIAN_POINT('Ctrl Pts',(0.00645633253597576,-0.040716472909516,
-0.0136533362604753));
#20479=CARTESIAN_POINT('Ctrl Pts',(0.00635798105751931,-0.0407106865879567,
-0.0136801936378314));
#20480=CARTESIAN_POINT('Ctrl Pts',(0.00617678069143139,-0.040700134475921,
-0.0137108895387227));
#20481=CARTESIAN_POINT('Ctrl Pts',(0.00609487396701188,-0.0406954109239253,
-0.0137181205544821));
#20482=CARTESIAN_POINT('Ctrl Pts',(0.00599585040133589,-0.0406900099813477,
-0.0137189405510562));
#20483=CARTESIAN_POINT('Ctrl Pts',(0.00597892209000315,-0.0406890978688332,
-0.0137188021813164));
#20484=CARTESIAN_POINT('Ctrl Pts',(0.00595276283657161,-0.0406877091790826,
-0.0137181577331468));
#20485=CARTESIAN_POINT('Ctrl Pts',(0.00594352883045026,-0.0406872229925691,
-0.0137178472460173));
#20486=CARTESIAN_POINT('Ctrl Pts',(0.00592630323206072,-0.0406863242253804,
-0.0137171131017568));
#20487=CARTESIAN_POINT('Ctrl Pts',(0.00591831167343682,-0.040685910632611,
-0.0137167102074386));
#20488=CARTESIAN_POINT('Ctrl Pts',(0.00589899938271384,-0.0406849188701749,
-0.0137155859051825));
#20489=CARTESIAN_POINT('Ctrl Pts',(0.00588768294064504,-0.0406843440692333,
-0.0137148018088508));
#20490=CARTESIAN_POINT('Ctrl Pts',(0.00584591780513346,-0.0406822428076906,
-0.013711444821988));
#20491=CARTESIAN_POINT('Ctrl Pts',(0.00581553739024073,-0.040680753864107,
-0.0137080923172214));
#20492=CARTESIAN_POINT('Ctrl Pts',(0.00573268109587621,-0.0406767544661384,
-0.0136964486770872));
#20493=CARTESIAN_POINT('Ctrl Pts',(0.00568050128306055,-0.0406743029842307,
-0.0136863468638638));
#20494=CARTESIAN_POINT('Ctrl Pts',(0.00552019613408895,-0.0406667241952723,
-0.0136466317472969));
#20495=CARTESIAN_POINT('Ctrl Pts',(0.00541471472872338,-0.0406616419864291,
-0.0136079288617161));
#20496=CARTESIAN_POINT('Ctrl Pts',(0.00529214236532736,-0.0406549636278507,
-0.0135471305502521));
#20497=CARTESIAN_POINT('Ctrl Pts',(0.00527019991226979,-0.0406537370427915,
-0.013535579550183));
#20498=CARTESIAN_POINT('Ctrl Pts',(0.00523529111460153,-0.0406517300025516,
-0.0135161143203821));
#20499=CARTESIAN_POINT('Ctrl Pts',(0.00522214631399861,-0.0406509611750179,
-0.0135085283933331));
#20500=CARTESIAN_POINT('Ctrl Pts',(0.00519699088545164,-0.0406494634091028,
-0.013493512105536));
#20501=CARTESIAN_POINT('Ctrl Pts',(0.00518496614254834,-0.0406487354857501,
-0.0134861082979582));
#20502=CARTESIAN_POINT('Ctrl Pts',(0.00515687739360278,-0.0406470060111948,
-0.0134682773640541));
#20503=CARTESIAN_POINT('Ctrl Pts',(0.00514090280802337,-0.0406459994918813,
-0.0134577143149038));
#20504=CARTESIAN_POINT('Ctrl Pts',(0.00508516633443893,-0.0406424042933358,
-0.0134193492017226));
#20505=CARTESIAN_POINT('Ctrl Pts',(0.00504652609213745,-0.0406397573343502,
-0.0133899741873596));
#20506=CARTESIAN_POINT('Ctrl Pts',(0.00494495204452492,-0.0406323763439658,
-0.0133049127154077));
#20507=CARTESIAN_POINT('Ctrl Pts',(0.00488508082990064,-0.0406275363409812,
-0.0132458321708397));
#20508=CARTESIAN_POINT('Ctrl Pts',(0.00478795735482854,-0.0406189912885865,
-0.0131329428069117));
#20509=CARTESIAN_POINT('Ctrl Pts',(0.00474874467329652,-0.0406152890207445,
-0.0130810764685347));
#20510=CARTESIAN_POINT('Ctrl Pts',(0.00470353989613774,-0.0406108167308208,
-0.0130127100087736));
#20511=CARTESIAN_POINT('Ctrl Pts',(0.00469439860491936,-0.0406099003905455,
-0.0129983756373753));
#20512=CARTESIAN_POINT('Ctrl Pts',(0.00468067616177849,-0.0406085094900141,
-0.0129760522052363));
#20513=CARTESIAN_POINT('Ctrl Pts',(0.00467592672674916,-0.0406080250971745,
-0.0129681686751539));
#20514=CARTESIAN_POINT('Ctrl Pts',(0.00466718162780741,-0.0406071282183929,
-0.0129533545227395));
#20515=CARTESIAN_POINT('Ctrl Pts',(0.00466316892978935,-0.0406067147234556,
-0.0129464346750234));
#20516=CARTESIAN_POINT('Ctrl Pts',(0.00465361627777243,-0.0406057249895091,
-0.0129296620362231));
#20517=CARTESIAN_POINT('Ctrl Pts',(0.00464813034171527,-0.0406051520537887,
-0.0129197788203857));
#20518=CARTESIAN_POINT('Ctrl Pts',(0.00462849552945023,-0.0406030812901228,
-0.0128834710371234));
#20519=CARTESIAN_POINT('Ctrl Pts',(0.00461500812658388,-0.0406016192119426,
-0.0128566947565149));
#20520=CARTESIAN_POINT('Ctrl Pts',(0.00458055023017565,-0.0405977262078779,
-0.0127830181463181));
#20521=CARTESIAN_POINT('Ctrl Pts',(0.00456112714799178,-0.0405953499949163,
-0.0127354354813212));
#20522=CARTESIAN_POINT('Ctrl Pts',(0.00450608667804092,-0.0405877146426372,
-0.0125786560336434));
#20523=CARTESIAN_POINT('Ctrl Pts',(0.00448026918262782,-0.0405825141736164,
-0.0124664452040318));
#20524=CARTESIAN_POINT('Ctrl Pts',(0.0044643475766838,-0.0405757193609202,
-0.0123282142499272));
#20525=CARTESIAN_POINT('Ctrl Pts',(0.00446213401693944,-0.0405745142893773,
-0.0123039562400101));
#20526=CARTESIAN_POINT('Ctrl Pts',(0.00445948135767097,-0.0405725347763589,
-0.0122646147806767));
#20527=CARTESIAN_POINT('Ctrl Pts',(0.00445868766174779,-0.0405717713111558,
-0.0122495590909445));
#20528=CARTESIAN_POINT('Ctrl Pts',(0.00445773365451917,-0.0405704886291275,
-0.0122244748679434));
#20529=CARTESIAN_POINT('Ctrl Pts',(0.00445745026688442,-0.0405699732731458,
-0.0122144519033791));
#20530=CARTESIAN_POINT('Ctrl Pts',(0.00445708819810097,-0.0405689623995923,
-0.0121949033226106));
#20531=CARTESIAN_POINT('Ctrl Pts',(0.004457,-0.040568467201217,-0.012185378332967));
#20532=CARTESIAN_POINT('Ctrl Pts',(0.004457,-0.0405679692773165,-0.012175853286558));
#20533=CARTESIAN_POINT('Origin',(-0.0125,-0.0375520664398416,-0.0121758532865581));
#20534=CARTESIAN_POINT('',(-0.014043,-0.0304166107246751,-0.0121758532865582));
#20535=CARTESIAN_POINT('',(-0.014043,-0.0303011972027429,-0.0121758532865251));
#20536=CARTESIAN_POINT('',(-0.014043,-0.0375520664398416,-0.012175853286558));
#20537=CARTESIAN_POINT('',(-0.0140434115472061,-0.030301351634873,-0.0121743803418281));
#20538=CARTESIAN_POINT('Ctrl Pts',(-0.014043,-0.0303011972027429,-0.0121758532864921));
#20539=CARTESIAN_POINT('Ctrl Pts',(-0.014043,-0.0303011717518023,-0.0121754036077484));
#20540=CARTESIAN_POINT('Ctrl Pts',(-0.0140429998034242,-0.0303011463056326,
-0.0121749539243807));
#20541=CARTESIAN_POINT('Ctrl Pts',(-0.0140429994102604,-0.0303011208642816,
-0.0121745042365161));
#20542=CARTESIAN_POINT('',(-0.0131954570230097,-0.0302142743898648,-0.0107984686165645));
#20543=CARTESIAN_POINT('Ctrl Pts',(-0.0140434115472061,-0.030301351634873,
-0.0121743803418281));
#20544=CARTESIAN_POINT('Ctrl Pts',(-0.0140434740875886,-0.0302984285463748,
-0.0121215468731317));
#20545=CARTESIAN_POINT('Ctrl Pts',(-0.0140408865195758,-0.030295616371813,
-0.0120687879599));
#20546=CARTESIAN_POINT('Ctrl Pts',(-0.0140354833210815,-0.030292885581712,
-0.0120163446339196));
#20547=CARTESIAN_POINT('Ctrl Pts',(-0.0140053197530325,-0.0302776408385983,
-0.011723577704556));
#20548=CARTESIAN_POINT('Ctrl Pts',(-0.0138865745209328,-0.0302649324214751,
-0.0114393196839804));
#20549=CARTESIAN_POINT('Ctrl Pts',(-0.0137019165735488,-0.0302496228389727,
-0.0112095557337391));
#20550=CARTESIAN_POINT('Ctrl Pts',(-0.0135646906639459,-0.0302382457419439,
-0.0110388099439558));
#20551=CARTESIAN_POINT('Ctrl Pts',(-0.0133911038022161,-0.0302255801464012,
-0.0108972480096383));
#20552=CARTESIAN_POINT('Ctrl Pts',(-0.0131954570230095,-0.0302142743898697,
-0.0107984686165644));
#20553=CARTESIAN_POINT('',(-0.0112093823259403,-0.030215088191226,-0.0113276377436708));
#20554=CARTESIAN_POINT('Origin',(-0.01249999999999,-0.0302142743898623,
-0.0121758532865681));
#20555=CARTESIAN_POINT('Ctrl Pts',(-0.0112106409242372,-0.0302159019925798,
-0.0113282672002234));
#20556=CARTESIAN_POINT('Ctrl Pts',(-0.0112128889480957,-0.0302161112403416,
-0.0113248474768335));
#20557=CARTESIAN_POINT('Ctrl Pts',(-0.0112151505937373,-0.0302163196178771,
-0.011321436671487));
#20558=CARTESIAN_POINT('Ctrl Pts',(-0.0112210324192457,-0.0302168561563185,
-0.0113126424122188));
#20559=CARTESIAN_POINT('Ctrl Pts',(-0.0112246730592058,-0.0302171830508598,
-0.011307272672607));
#20560=CARTESIAN_POINT('Ctrl Pts',(-0.0112417552471371,-0.0302186936789069,
-0.0112824163643799));
#20561=CARTESIAN_POINT('Ctrl Pts',(-0.0112556108209913,-0.0302198531818524,
-0.0112632169578027));
#20562=CARTESIAN_POINT('Ctrl Pts',(-0.0113363765789313,-0.0302262976394441,
-0.0111565625229546));
#20563=CARTESIAN_POINT('Ctrl Pts',(-0.0114120594196726,-0.0302311901234243,
-0.011076143186243));
#20564=CARTESIAN_POINT('Ctrl Pts',(-0.0115503847147757,-0.0302395951819232,
-0.0109575449019186));
#20565=CARTESIAN_POINT('Ctrl Pts',(-0.0116083213402903,-0.0302429855296231,
-0.0109145237014696));
#20566=CARTESIAN_POINT('Ctrl Pts',(-0.011686140488403,-0.0302475289600024,
-0.0108647876252495));
#20567=CARTESIAN_POINT('Ctrl Pts',(-0.0117034458035125,-0.0302485382710704,
-0.0108542021082295));
#20568=CARTESIAN_POINT('Ctrl Pts',(-0.0117300479054118,-0.0302500905181481,
-0.0108386420998857));
#20569=CARTESIAN_POINT('Ctrl Pts',(-0.0117391956082126,-0.0302506244087221,
-0.0108334164515111));
#20570=CARTESIAN_POINT('Ctrl Pts',(-0.011755221200139,-0.0302515601969005,
-0.0108244782036918));
#20571=CARTESIAN_POINT('Ctrl Pts',(-0.0117620751748523,-0.0302519605738842,
-0.0108207233943327));
#20572=CARTESIAN_POINT('Ctrl Pts',(-0.0117775990626936,-0.0302528678627463,
-0.010812371647127));
#20573=CARTESIAN_POINT('Ctrl Pts',(-0.0117862848463781,-0.0302533758191923,
-0.0108078050531642));
#20574=CARTESIAN_POINT('Ctrl Pts',(-0.0118099753534279,-0.0302547623492623,
-0.0107956366714528));
#20575=CARTESIAN_POINT('Ctrl Pts',(-0.011825061483457,-0.0302556464655072,
-0.0107881970298671));
#20576=CARTESIAN_POINT('Ctrl Pts',(-0.0119129398735264,-0.0302608045273133,
-0.010746632362917));
#20577=CARTESIAN_POINT('Ctrl Pts',(-0.0119881799830745,-0.0302652616617878,
-0.0107179954451448));
#20578=CARTESIAN_POINT('Ctrl Pts',(-0.0121503146253649,-0.0302748462115804,
-0.0106703899907418));
#20579=CARTESIAN_POINT('Ctrl Pts',(-0.0122373199868089,-0.0302799787493356,
-0.010652797567));
#20580=CARTESIAN_POINT('Ctrl Pts',(-0.0123500996803343,-0.0302863335257897,
-0.0106399499032247));
#20581=CARTESIAN_POINT('Ctrl Pts',(-0.0123749113486741,-0.0302877125198554,
-0.0106377303254376));
#20582=CARTESIAN_POINT('Ctrl Pts',(-0.0124165652710717,-0.0302899843268226,
-0.0106350187631249));
#20583=CARTESIAN_POINT('Ctrl Pts',(-0.01243338112176,-0.0302908896808708,
-0.0106342001636292));
#20584=CARTESIAN_POINT('Ctrl Pts',(-0.0124571390710527,-0.0302921490056019,
-0.0106334330987397));
#20585=CARTESIAN_POINT('Ctrl Pts',(-0.0124640720731839,-0.0302925141217255,
-0.0106332560343302));
#20586=CARTESIAN_POINT('Ctrl Pts',(-0.0124759986750655,-0.0302931378521079,
-0.0106330318871608));
#20587=CARTESIAN_POINT('Ctrl Pts',(-0.0124809917118446,-0.0302933976588468,
-0.010632962292051));
#20588=CARTESIAN_POINT('Ctrl Pts',(-0.0124914516749318,-0.0302939390487119,
-0.0106328672814104));
#20589=CARTESIAN_POINT('Ctrl Pts',(-0.0124969185598081,-0.0302942203644687,
-0.0106328466785202));
#20590=CARTESIAN_POINT('Ctrl Pts',(-0.0125118384323821,-0.0302949839072028,
-0.0106328697450744));
#20591=CARTESIAN_POINT('Ctrl Pts',(-0.0125212912340889,-0.0302954630580415,
-0.0106329712270566));
#20592=CARTESIAN_POINT('Ctrl Pts',(-0.0125683923754362,-0.0302978301556941,
-0.0106339098563435));
#20593=CARTESIAN_POINT('Ctrl Pts',(-0.0126060046113189,-0.0302996555214584,
-0.0106360382098715));
#20594=CARTESIAN_POINT('Ctrl Pts',(-0.0127448491660251,-0.0303062714341073,
-0.0106490073839222));
#20595=CARTESIAN_POINT('Ctrl Pts',(-0.0128450132129234,-0.0303108171694383,
-0.0106684788984534));
#20596=CARTESIAN_POINT('Ctrl Pts',(-0.0130113085475643,-0.0303188633900924,
-0.0107182640257786));
#20597=CARTESIAN_POINT('Ctrl Pts',(-0.0130785559003934,-0.0303222636577658,
-0.0107436261684833));
#20598=CARTESIAN_POINT('Ctrl Pts',(-0.0131588080123629,-0.0303266406798236,
-0.0107804701562242));
#20599=CARTESIAN_POINT('Ctrl Pts',(-0.013173713863844,-0.0303274675381767,
-0.0107876055850281));
#20600=CARTESIAN_POINT('Ctrl Pts',(-0.0131971681214754,-0.0303287920357033,
-0.0107992998423665));
#20601=CARTESIAN_POINT('Ctrl Pts',(-0.0132057933493018,-0.0303292842278123,
-0.0108037022318877));
#20602=CARTESIAN_POINT('Ctrl Pts',(-0.0132212290482677,-0.0303301745192883,
-0.0108117647887721));
#20603=CARTESIAN_POINT('Ctrl Pts',(-0.0132280545721877,-0.0303305715687269,
-0.0108153955301812));
#20604=CARTESIAN_POINT('Ctrl Pts',(-0.0132440356719109,-0.0303315092894806,
-0.0108240511600488));
#20605=CARTESIAN_POINT('Ctrl Pts',(-0.0132531680111097,-0.030332051445356,
-0.0108291179710081));
#20606=CARTESIAN_POINT('Ctrl Pts',(-0.0132797871363435,-0.0303336505949328,
-0.0108442422521422));
#20607=CARTESIAN_POINT('Ctrl Pts',(-0.0132971285023787,-0.0303347165555468,
-0.0108545501329503));
#20608=CARTESIAN_POINT('Ctrl Pts',(-0.0133754308831641,-0.0303396431246271,
-0.0109031964207954));
#20609=CARTESIAN_POINT('Ctrl Pts',(-0.0134338571581009,-0.0303436450810037,
-0.0109454291875043));
#20610=CARTESIAN_POINT('Ctrl Pts',(-0.0135424034645513,-0.0303516853163875,
-0.0110360882473248));
#20611=CARTESIAN_POINT('Ctrl Pts',(-0.0135926253810445,-0.0303557073647253,
-0.0110841396476955));
#20612=CARTESIAN_POINT('Ctrl Pts',(-0.0136824149249653,-0.030363332887136,
-0.0111824722038504));
#20613=CARTESIAN_POINT('Ctrl Pts',(-0.0137224376692887,-0.0303669352308319,
-0.0112321591360074));
#20614=CARTESIAN_POINT('Ctrl Pts',(-0.0137652657179544,-0.0303709162266439,
-0.0112926437247606));
#20615=CARTESIAN_POINT('Ctrl Pts',(-0.0137711711424191,-0.0303714682133485,
-0.0113011645389617));
#20616=CARTESIAN_POINT('Ctrl Pts',(-0.0137801872895065,-0.0303723149476296,
-0.0113144579412226));
#20617=CARTESIAN_POINT('Ctrl Pts',(-0.013783358111617,-0.0303726135168364,
-0.0113191891770197));
#20618=CARTESIAN_POINT('Ctrl Pts',(-0.0137891462105387,-0.0303731598292146,
-0.0113279299573756));
#20619=CARTESIAN_POINT('Ctrl Pts',(-0.013791771064165,-0.0303734080630411,
-0.0113319341890156));
#20620=CARTESIAN_POINT('Ctrl Pts',(-0.0137977440881499,-0.0303739740860938,
-0.0113411392414262));
#20621=CARTESIAN_POINT('Ctrl Pts',(-0.0138010796582745,-0.0303742910432325,
-0.0113463480238528));
#20622=CARTESIAN_POINT('Ctrl Pts',(-0.013811473055066,-0.0303752818755205,
-0.0113627951499489));
#20623=CARTESIAN_POINT('Ctrl Pts',(-0.0138184174443557,-0.0303759486566424,
-0.0113741048393859));
#20624=CARTESIAN_POINT('Ctrl Pts',(-0.0138541184080652,-0.0303794096330583,
-0.0114339662291199));
#20625=CARTESIAN_POINT('Ctrl Pts',(-0.0138803438739666,-0.0303820691261823,
-0.0114839826899219));
#20626=CARTESIAN_POINT('Ctrl Pts',(-0.01395035767675,-0.0303898718469728,
-0.0116374243898987));
#20627=CARTESIAN_POINT('Ctrl Pts',(-0.013985665331939,-0.0303948723338038,
-0.0117442957161421));
#20628=CARTESIAN_POINT('Ctrl Pts',(-0.0140178041752537,-0.0304022027895388,
-0.0118950095262979));
#20629=CARTESIAN_POINT('Ctrl Pts',(-0.0140248664408474,-0.0304042351083484,
-0.0119363022550097));
#20630=CARTESIAN_POINT('Ctrl Pts',(-0.0140320427969083,-0.0304070201462079,
-0.011991757857305));
#20631=CARTESIAN_POINT('Ctrl Pts',(-0.0140336549765975,-0.0304077254412494,
-0.0120057102446011));
#20632=CARTESIAN_POINT('Ctrl Pts',(-0.0140359948986158,-0.0304088964065686,
-0.0120287104303252));
#20633=CARTESIAN_POINT('Ctrl Pts',(-0.014036833689447,-0.0304093585306091,
-0.0120377462446039));
#20634=CARTESIAN_POINT('Ctrl Pts',(-0.0140382682270244,-0.030410236737763,
-0.0120548364195145));
#20635=CARTESIAN_POINT('Ctrl Pts',(-0.0140388805381732,-0.0304106522778035,
-0.0120628891051825));
#20636=CARTESIAN_POINT('Ctrl Pts',(-0.0140400011847363,-0.030411504526978,
-0.0120793337069593));
#20637=CARTESIAN_POINT('Ctrl Pts',(-0.0140405042043225,-0.0304119413906177,
-0.0120877257034955));
#20638=CARTESIAN_POINT('Ctrl Pts',(-0.014041543983286,-0.0304129922645103,
-0.0121078209656391));
#20639=CARTESIAN_POINT('Ctrl Pts',(-0.0140420160767744,-0.0304136082954006,
-0.0121195269361538));
#20640=CARTESIAN_POINT('Ctrl Pts',(-0.0140427849275548,-0.0304150159869659,
-0.0121461055473814));
#20641=CARTESIAN_POINT('Ctrl Pts',(-0.014043,-0.0304158101282949,-0.0121609792078244));
#20642=CARTESIAN_POINT('Ctrl Pts',(-0.014043,-0.0304166107246751,-0.0121758532865585));
#20643=CARTESIAN_POINT('Origin',(-0.0125,-0.0375520664398416,-0.0121758532865581));
#20644=CARTESIAN_POINT('',(-0.014043,-0.0309187674107451,-0.0121758533048158));
#20645=CARTESIAN_POINT('',(-0.014043,-0.0308032888456207,-0.0121758532865568));
#20646=CARTESIAN_POINT('',(-0.014043,-0.0375520664398416,-0.012175853286558));
#20647=CARTESIAN_POINT('',(-0.0140429998315375,-0.0308032493790877,-0.0121751322628013));
#20648=CARTESIAN_POINT('Ctrl Pts',(-0.014043,-0.0308032888456207,-0.0121758532865555));
#20649=CARTESIAN_POINT('Ctrl Pts',(-0.014043,-0.0308032755095055,-0.0121756096173267));
#20650=CARTESIAN_POINT('Ctrl Pts',(-0.0140429999454013,-0.0308032627183605,
-0.0121753759327705));
#20651=CARTESIAN_POINT('Ctrl Pts',(-0.0140429998315375,-0.0308032493790877,
-0.0121751322628013));
#20652=CARTESIAN_POINT('Ctrl Pts',(-0.0140429998315375,-0.0308032493790877,
-0.0121751322628013));
#20653=CARTESIAN_POINT('Ctrl Pts',(-0.0140429494230278,-0.0307973439656581,
-0.0120672574234215));
#20654=CARTESIAN_POINT('Ctrl Pts',(-0.0140315862929371,-0.0307911149504177,
-0.0119596942407359));
#20655=CARTESIAN_POINT('Ctrl Pts',(-0.0139938756588056,-0.0307807274271626,
-0.0117827611841786));
#20656=CARTESIAN_POINT('Ctrl Pts',(-0.0139735908635154,-0.0307765709606792,
-0.0117124767654398));
#20657=CARTESIAN_POINT('Ctrl Pts',(-0.0139448135370339,-0.0307720887975717,
-0.0116341235815599));
#20658=CARTESIAN_POINT('Ctrl Pts',(-0.0139411281066165,-0.0307715350731643,
-0.0116243942926599));
#20659=CARTESIAN_POINT('Ctrl Pts',(-0.013935300213029,-0.0307706907111287,
-0.011609466585592));
#20660=CARTESIAN_POINT('Ctrl Pts',(-0.0139332273368253,-0.0307703961576646,
-0.0116042415306437));
#20661=CARTESIAN_POINT('Ctrl Pts',(-0.0139293354291963,-0.0307698538238913,
-0.0115945855594669));
#20662=CARTESIAN_POINT('Ctrl Pts',(-0.013927524313414,-0.0307696056024641,
-0.0115901517628385));
#20663=CARTESIAN_POINT('Ctrl Pts',(-0.0139233370211045,-0.0307690410349654,
-0.0115800356499321));
#20664=CARTESIAN_POINT('Ctrl Pts',(-0.0139209474430705,-0.0307687254998222,
-0.0115743590652198));
#20665=CARTESIAN_POINT('Ctrl Pts',(-0.0139132388108628,-0.0307677279934698,
-0.0115563490791319));
#20666=CARTESIAN_POINT('Ctrl Pts',(-0.0139077925512098,-0.030767053299491,
-0.0115440704477702));
#20667=CARTESIAN_POINT('Ctrl Pts',(-0.013859620407409,-0.0307613235492035,
-0.0114391830807388));
#20668=CARTESIAN_POINT('Ctrl Pts',(-0.0138079652272933,-0.0307567183531191,
-0.0113509397503003));
#20669=CARTESIAN_POINT('Ctrl Pts',(-0.0137072622140268,-0.0307488878584575,
-0.011212443082351));
#20670=CARTESIAN_POINT('Ctrl Pts',(-0.0136628308683721,-0.0307457059712628,
-0.0111592585208379));
#20671=CARTESIAN_POINT('Ctrl Pts',(-0.0135962327657241,-0.0307411088261712,
-0.0110896404486581));
#20672=CARTESIAN_POINT('Ctrl Pts',(-0.0135769715949999,-0.0307397975107651,
-0.0110705403487544));
#20673=CARTESIAN_POINT('Ctrl Pts',(-0.0135420153704053,-0.0307374400390593,
-0.0110376579695552));
#20674=CARTESIAN_POINT('Ctrl Pts',(-0.0135265249687069,-0.0307364026865651,
-0.0110236679507206));
#20675=CARTESIAN_POINT('Ctrl Pts',(-0.0135027982186729,-0.0307348219970792,
-0.0110030977037257));
#20676=CARTESIAN_POINT('Ctrl Pts',(-0.0134947701279002,-0.0307342885380063,
-0.0109962803511566));
#20677=CARTESIAN_POINT('Ctrl Pts',(-0.0134801371148019,-0.0307333183483052,
-0.0109841098140687));
#20678=CARTESIAN_POINT('Ctrl Pts',(-0.0134735565062655,-0.0307328828174035,
-0.0109787279826328));
#20679=CARTESIAN_POINT('Ctrl Pts',(-0.0134593177176003,-0.0307319419320742,
-0.0109672781006363));
#20680=CARTESIAN_POINT('Ctrl Pts',(-0.0134516457264063,-0.030731435886214,
-0.0109612278838804));
#20681=CARTESIAN_POINT('Ctrl Pts',(-0.0134306989216477,-0.0307300564533405,
-0.0109450292875952));
#20682=CARTESIAN_POINT('Ctrl Pts',(-0.0134173161417123,-0.0307291775103342,
-0.0109350232153287));
#20683=CARTESIAN_POINT('Ctrl Pts',(-0.0133281770452895,-0.0307233368788353,
-0.0108706057229196));
#20684=CARTESIAN_POINT('Ctrl Pts',(-0.0132477935132545,-0.0307181168976065,
-0.0108229494442921));
#20685=CARTESIAN_POINT('Ctrl Pts',(-0.0131031361488627,-0.030708945922402,
-0.0107540364882219));
#20686=CARTESIAN_POINT('Ctrl Pts',(-0.0130408494877025,-0.030705066069523,
-0.0107291957277703));
#20687=CARTESIAN_POINT('Ctrl Pts',(-0.0129292148328437,-0.0306983982392364,
-0.0106928954607309));
#20688=CARTESIAN_POINT('Ctrl Pts',(-0.0128805447208854,-0.030695582858372,
-0.0106796661776394));
#20689=CARTESIAN_POINT('Ctrl Pts',(-0.0128217893157134,-0.0306923591810636,
-0.0106667490244168));
#20690=CARTESIAN_POINT('Ctrl Pts',(-0.0128122480998191,-0.0306918411466117,
-0.0106647460198662));
#20691=CARTESIAN_POINT('Ctrl Pts',(-0.0127973060332986,-0.0306910390824373,
-0.0106617567735114));
#20692=CARTESIAN_POINT('Ctrl Pts',(-0.0127919179712198,-0.0306907517241886,
-0.0106607087297013));
#20693=CARTESIAN_POINT('Ctrl Pts',(-0.0127817729305266,-0.0306902143185438,
-0.0106587915218718));
#20694=CARTESIAN_POINT('Ctrl Pts',(-0.0127770173567079,-0.0306899639288118,
-0.0106579159470733));
#20695=CARTESIAN_POINT('Ctrl Pts',(-0.0127659386821497,-0.0306893840463748,
-0.0106559299891024));
#20696=CARTESIAN_POINT('Ctrl Pts',(-0.0127596125704511,-0.0306890555078882,
-0.0106548366762317));
#20697=CARTESIAN_POINT('Ctrl Pts',(-0.0127392376551842,-0.0306880051445119,
-0.0106514461940434));
#20698=CARTESIAN_POINT('Ctrl Pts',(-0.0127251634641828,-0.030687291472665,
-0.0106493038832516));
#20699=CARTESIAN_POINT('Ctrl Pts',(-0.0126312431836584,-0.0306825961354117,
-0.0106363349802867));
#20700=CARTESIAN_POINT('Ctrl Pts',(-0.0125506762103103,-0.0306788865497949,
-0.01063158133982));
#20701=CARTESIAN_POINT('Ctrl Pts',(-0.0123601624331091,-0.0306701592498833,
-0.0106352737465537));
#20702=CARTESIAN_POINT('Ctrl Pts',(-0.0122507770236676,-0.0306651636470311,
-0.0106491490349497));
#20703=CARTESIAN_POINT('Ctrl Pts',(-0.0121201739451476,-0.0306586079110084,
-0.0106801358558692));
#20704=CARTESIAN_POINT('Ctrl Pts',(-0.0120966873110969,-0.0306574062505756,
-0.0106862972255519));
#20705=CARTESIAN_POINT('Ctrl Pts',(-0.01206260818613,-0.0306556250520392,
-0.0106961024654139));
#20706=CARTESIAN_POINT('Ctrl Pts',(-0.0120518939316198,-0.0306550595703174,
-0.0106993117075613));
#20707=CARTESIAN_POINT('Ctrl Pts',(-0.0120330202214829,-0.0306540533484992,
-0.0107051892984499));
#20708=CARTESIAN_POINT('Ctrl Pts',(-0.0120248463055414,-0.0306536141938463,
-0.0107078098123495));
#20709=CARTESIAN_POINT('Ctrl Pts',(-0.0120077550872787,-0.0306526886876185,
-0.010713446859534));
#20710=CARTESIAN_POINT('Ctrl Pts',(-0.0119988426941627,-0.0306522018978928,
-0.0107164770631535));
#20711=CARTESIAN_POINT('Ctrl Pts',(-0.0119753903193451,-0.0306509096765467,
-0.0107246910089749));
#20712=CARTESIAN_POINT('Ctrl Pts',(-0.0119608996873145,-0.030650099723648,
-0.0107300116277281));
#20713=CARTESIAN_POINT('Ctrl Pts',(-0.0118949290143646,-0.0306463582493014,
-0.0107553641233125));
#20714=CARTESIAN_POINT('Ctrl Pts',(-0.0118444725404604,-0.0306433425308871,
-0.0107779322920615));
#20715=CARTESIAN_POINT('Ctrl Pts',(-0.0117084441162718,-0.0306347961772676,
-0.0108477611972743));
#20716=CARTESIAN_POINT('Ctrl Pts',(-0.0116259853465121,-0.0306291196217377,
-0.0109005159723672));
#20717=CARTESIAN_POINT('Ctrl Pts',(-0.0115054938057397,-0.0306203765260033,
-0.0109948076630089));
#20718=CARTESIAN_POINT('Ctrl Pts',(-0.0114637760304338,-0.030617255673004,
-0.0110312344862779));
#20719=CARTESIAN_POINT('Ctrl Pts',(-0.0114146650296267,-0.0306135500857657,
-0.0110790076429274));
#20720=CARTESIAN_POINT('Ctrl Pts',(-0.0114053446397557,-0.0306128453806097,
-0.0110883092512143));
#20721=CARTESIAN_POINT('Ctrl Pts',(-0.0113918281553366,-0.0306118228564228,
-0.0111021483371867));
#20722=CARTESIAN_POINT('Ctrl Pts',(-0.0113875386512043,-0.0306114982707693,
-0.0111065933061866));
#20723=CARTESIAN_POINT('Ctrl Pts',(-0.0113799837698613,-0.0306109266485566,
-0.0111145166748831));
#20724=CARTESIAN_POINT('Ctrl Pts',(-0.011376707656632,-0.0306106787951981,
-0.011117984640405));
#20725=CARTESIAN_POINT('Ctrl Pts',(-0.011369594156811,-0.0306101407404914,
-0.011125585021181));
#20726=CARTESIAN_POINT('Ctrl Pts',(-0.0113657632957425,-0.0306098510289648,
-0.0111297233231859));
#20727=CARTESIAN_POINT('Ctrl Pts',(-0.0113549943971347,-0.030609036449744,
-0.0111414851603933));
#20728=CARTESIAN_POINT('Ctrl Pts',(-0.0113481098222761,-0.0306085154811586,
-0.011149157479398));
#20729=CARTESIAN_POINT('Ctrl Pts',(-0.0112981484961286,-0.0306047283158406,
-0.0112059706575476));
#20730=CARTESIAN_POINT('Ctrl Pts',(-0.0112581510031366,-0.0306016589992643,
-0.011257739948259));
#20731=CARTESIAN_POINT('Ctrl Pts',(-0.0111852487920264,-0.0305956568415225,
-0.0113656172204017));
#20732=CARTESIAN_POINT('Ctrl Pts',(-0.0111523657429364,-0.0305927281169855,
-0.0114215752922551));
#20733=CARTESIAN_POINT('Ctrl Pts',(-0.0110864006852365,-0.0305860048597797,
-0.0115519961374219));
#20734=CARTESIAN_POINT('Ctrl Pts',(-0.0110554970487696,-0.0305821856347508,
-0.0116273370579108));
#20735=CARTESIAN_POINT('Ctrl Pts',(-0.0110256835874023,-0.0305773482220927,
-0.0117203235107662));
#20736=CARTESIAN_POINT('Ctrl Pts',(-0.0110209401514166,-0.0305765306276997,
-0.0117359689842479));
#20737=CARTESIAN_POINT('Ctrl Pts',(-0.0110138205785899,-0.0305752223553117,
-0.0117608702000671));
#20738=CARTESIAN_POINT('Ctrl Pts',(-0.0110112802165783,-0.0305747370980337,
-0.0117700779352432));
#20739=CARTESIAN_POINT('Ctrl Pts',(-0.0110066532492773,-0.0305738170960861,
-0.0117874772711904));
#20740=CARTESIAN_POINT('Ctrl Pts',(-0.0110045481435961,-0.0305733829785686,
-0.0117956636121019));
#20741=CARTESIAN_POINT('Ctrl Pts',(-0.0109999407520886,-0.0305723964077133,
-0.0118142113810097));
#20742=CARTESIAN_POINT('Ctrl Pts',(-0.0109974783760361,-0.0305718426742196,
-0.0118245821991285));
#20743=CARTESIAN_POINT('Ctrl Pts',(-0.0109903127649398,-0.0305701469274038,
-0.0118562164764711));
#20744=CARTESIAN_POINT('Ctrl Pts',(-0.010985952191084,-0.0305689939405844,
-0.0118775541004177));
#20745=CARTESIAN_POINT('Ctrl Pts',(-0.0109653526083149,-0.0305628412630669,
-0.0119904895517208));
#20746=CARTESIAN_POINT('Ctrl Pts',(-0.0109569723504914,-0.0305575944876602,
-0.0120833126911311));
#20747=CARTESIAN_POINT('Ctrl Pts',(-0.0109570310556734,-0.0305462854740702,
-0.0122802823658357));
#20748=CARTESIAN_POINT('Ctrl Pts',(-0.0109675701548483,-0.0305402283780848,
-0.0123839872079394));
#20749=CARTESIAN_POINT('Ctrl Pts',(-0.0109908578235556,-0.0305339559971616,
-0.0124975383991549));
#20750=CARTESIAN_POINT('Ctrl Pts',(-0.0109933910287286,-0.0305333163427565,
-0.0125092012202782));
#20751=CARTESIAN_POINT('Ctrl Pts',(-0.0109974016673079,-0.0305323655343222,
-0.0125266855762637));
#20752=CARTESIAN_POINT('Ctrl Pts',(-0.0109987781345088,-0.0305320491088742,
-0.012532529551301));
#20753=CARTESIAN_POINT('Ctrl Pts',(-0.0110013304375527,-0.0305314800344124,
-0.0125430891227222));
#20754=CARTESIAN_POINT('Ctrl Pts',(-0.0110024945079939,-0.030531226728674,
-0.0125478074780214));
#20755=CARTESIAN_POINT('Ctrl Pts',(-0.0110049464103402,-0.0305307059347612,
-0.0125575477186903));
#20756=CARTESIAN_POINT('Ctrl Pts',(-0.0110062372790875,-0.030530438618633,
-0.0125625686995377));
#20757=CARTESIAN_POINT('Ctrl Pts',(-0.0110096743575761,-0.0305297442262051,
-0.0125756635804875));
#20758=CARTESIAN_POINT('Ctrl Pts',(-0.0110118609023418,-0.0305293194148494,
-0.0125837268252921));
#20759=CARTESIAN_POINT('Ctrl Pts',(-0.0110220196005824,-0.0305274182439488,
-0.0126200191953254));
#20760=CARTESIAN_POINT('Ctrl Pts',(-0.0110307306761535,-0.0305259803376887,
-0.0126480368022343));
#20761=CARTESIAN_POINT('Ctrl Pts',(-0.0110587278539433,-0.0305218284427781,
-0.0127297856134861));
#20762=CARTESIAN_POINT('Ctrl Pts',(-0.0110802026541831,-0.0305191956550781,
-0.0127827162446283));
#20763=CARTESIAN_POINT('Ctrl Pts',(-0.011156662585713,-0.0305109887263886,
-0.0129447475557486));
#20764=CARTESIAN_POINT('Ctrl Pts',(-0.0112216765904696,-0.0305054715992893,
-0.0130485736948259));
#20765=CARTESIAN_POINT('Ctrl Pts',(-0.0113098757997528,-0.0304985580437578,
-0.0131580942112467));
#20766=CARTESIAN_POINT('Ctrl Pts',(-0.0113217654382306,-0.0304976368241939,
-0.0131723251261466));
#20767=CARTESIAN_POINT('Ctrl Pts',(-0.0113411685566166,-0.0304961483394291,
-0.0131947161777586));
#20768=CARTESIAN_POINT('Ctrl Pts',(-0.0113485187203051,-0.0304955877483875,
-0.0132030157661547));
#20769=CARTESIAN_POINT('Ctrl Pts',(-0.0113617395626463,-0.030494584783748,
-0.0132176240987487));
#20770=CARTESIAN_POINT('Ctrl Pts',(-0.0113675748990186,-0.0304941439085291,
-0.0132239642706958));
#20771=CARTESIAN_POINT('Ctrl Pts',(-0.0113798954720892,-0.0304932166438202,
-0.0132371277356155));
#20772=CARTESIAN_POINT('Ctrl Pts',(-0.0113863906442239,-0.0304927298350149,
-0.0132439412076329));
#20773=CARTESIAN_POINT('Ctrl Pts',(-0.0114036429511642,-0.0304914418643615,
-0.0132617105326062));
#20774=CARTESIAN_POINT('Ctrl Pts',(-0.0114145017937085,-0.0304906362758869,
-0.013272565809772));
#20775=CARTESIAN_POINT('Ctrl Pts',(-0.0114688045812437,-0.0304866313182435,
-0.0133252541192191));
#20776=CARTESIAN_POINT('Ctrl Pts',(-0.0115145091375823,-0.0304833304183131,
-0.0133646731809641));
#20777=CARTESIAN_POINT('Ctrl Pts',(-0.0116167928359515,-0.0304761087625533,
-0.0134429305290912));
#20778=CARTESIAN_POINT('Ctrl Pts',(-0.0116738946187512,-0.0304721717299995,
-0.0134808776667595));
#20779=CARTESIAN_POINT('Ctrl Pts',(-0.0117408997875379,-0.0304677368945097,
-0.0135192415635791));
#20780=CARTESIAN_POINT('Ctrl Pts',(-0.0117485116987227,-0.0304672357273039,
-0.0135235144194579));
#20781=CARTESIAN_POINT('Ctrl Pts',(-0.0118208725904811,-0.0304624984088769,
-0.0135633296358874));
#20782=CARTESIAN_POINT('Ctrl Pts',(-0.0118880651098639,-0.0304582975430782,
-0.0135942475560951));
#20783=CARTESIAN_POINT('Ctrl Pts',(-0.0119670189529705,-0.0304537690027713,
-0.0136239174433357));
#20784=CARTESIAN_POINT('Ctrl Pts',(-0.0119768562716497,-0.0304532118153955,
-0.0136275003682332));
#20785=CARTESIAN_POINT('Ctrl Pts',(-0.0119921419429425,-0.0304523577512523,
-0.013632892109869));
#20786=CARTESIAN_POINT('Ctrl Pts',(-0.011997565031341,-0.0304520570108528,
-0.0136347710508932));
#20787=CARTESIAN_POINT('Ctrl Pts',(-0.0120071742131388,-0.0304515282905298,
-0.013638040414886));
#20788=CARTESIAN_POINT('Ctrl Pts',(-0.0120113559134437,-0.0304512996033983,
-0.0136394431919941));
#20789=CARTESIAN_POINT('Ctrl Pts',(-0.0120213711478742,-0.0304507551408711,
-0.0136427551564418));
#20790=CARTESIAN_POINT('Ctrl Pts',(-0.0120272102229729,-0.0304504403265547,
-0.0136446475209974));
#20791=CARTESIAN_POINT('Ctrl Pts',(-0.0120449102584731,-0.0304494935025026,
-0.0136502673730838));
#20792=CARTESIAN_POINT('Ctrl Pts',(-0.0120568053751285,-0.0304488673160112,
-0.0136538864776071));
#20793=CARTESIAN_POINT('Ctrl Pts',(-0.0121432858394292,-0.0304443792744698,
-0.0136790603382886));
#20794=CARTESIAN_POINT('Ctrl Pts',(-0.0122193675082449,-0.0304407732031814,
-0.0136951044785367));
#20795=CARTESIAN_POINT('Ctrl Pts',(-0.0124120221433754,-0.030431815569623,
-0.0137207573530174));
#20796=CARTESIAN_POINT('Ctrl Pts',(-0.0125290679802229,-0.0304265009074883,
-0.013722986690178));
#20797=CARTESIAN_POINT('Ctrl Pts',(-0.0126635106112397,-0.0304198540856339,
-0.0137102749700046));
#20798=CARTESIAN_POINT('Ctrl Pts',(-0.0126817436636776,-0.0304189419127957,
-0.0137082223115352));
#20799=CARTESIAN_POINT('Ctrl Pts',(-0.0127109304055275,-0.0304174625238897,
-0.013704408264347));
#20800=CARTESIAN_POINT('Ctrl Pts',(-0.0127219094838851,-0.030416901647396,
-0.0137028530013345));
#20801=CARTESIAN_POINT('Ctrl Pts',(-0.0127414673467393,-0.0304158943082802,
-0.0136998671138763));
#20802=CARTESIAN_POINT('Ctrl Pts',(-0.0127500526574781,-0.0304154492837221,
-0.013698482029835));
#20803=CARTESIAN_POINT('Ctrl Pts',(-0.0127680735993039,-0.0304145090170615,
-0.0136954181547351));
#20804=CARTESIAN_POINT('Ctrl Pts',(-0.0127775061934778,-0.0304140133054916,
-0.0136937238839203));
#20805=CARTESIAN_POINT('Ctrl Pts',(-0.012802478211279,-0.0304126912727064,
-0.013688997888557));
#20806=CARTESIAN_POINT('Ctrl Pts',(-0.012817987526607,-0.0304118602145704,
-0.0136858147307157));
#20807=CARTESIAN_POINT('Ctrl Pts',(-0.0128976761518482,-0.0304075371738706,
-0.0136681771318004));
#20808=CARTESIAN_POINT('Ctrl Pts',(-0.0129609254904815,-0.0304039236816433,
-0.0136498691678098));
#20809=CARTESIAN_POINT('Ctrl Pts',(-0.0130841263647366,-0.0303965468009369,
-0.0136055011220681));
#20810=CARTESIAN_POINT('Ctrl Pts',(-0.0131439814088435,-0.0303927927114002,
-0.0135795568789032));
#20811=CARTESIAN_POINT('Ctrl Pts',(-0.0132700101696556,-0.0303846516667243,
-0.0135151679245038));
#20812=CARTESIAN_POINT('Ctrl Pts',(-0.0133353395666186,-0.0303802770251158,
-0.0134754258988562));
#20813=CARTESIAN_POINT('Ctrl Pts',(-0.0134080169292813,-0.0303754311130047,
-0.0134234600478813));
#20814=CARTESIAN_POINT('Ctrl Pts',(-0.0134184769205675,-0.0303747343583456,
-0.0134157797127629));
#20815=CARTESIAN_POINT('Ctrl Pts',(-0.0134343989358369,-0.0303736764289402,
-0.0134037767807791));
#20816=CARTESIAN_POINT('Ctrl Pts',(-0.0134399304422851,-0.0303733093944198,
-0.0133995477934748));
#20817=CARTESIAN_POINT('Ctrl Pts',(-0.0134492548124156,-0.0303726918248975,
-0.0133923185282897));
#20818=CARTESIAN_POINT('Ctrl Pts',(-0.0134530624926613,-0.0303724399601715,
-0.0133893376373446));
#20819=CARTESIAN_POINT('Ctrl Pts',(-0.0134607591902259,-0.0303719316240073,
-0.0133832536057947));
#20820=CARTESIAN_POINT('Ctrl Pts',(-0.0134646472362987,-0.0303716752555374,
-0.0133801495389822));
#20821=CARTESIAN_POINT('Ctrl Pts',(-0.0134747992607237,-0.0303710069550637,
-0.0133719638403907));
#20822=CARTESIAN_POINT('Ctrl Pts',(-0.0134810384902817,-0.0303705972902913,
-0.0133668518348593));
#20823=CARTESIAN_POINT('Ctrl Pts',(-0.01351012246613,-0.0303686910913438,
-0.0133426387488838));
#20824=CARTESIAN_POINT('Ctrl Pts',(-0.0135324526332497,-0.0303672375738174,
-0.0133229267366824));
#20825=CARTESIAN_POINT('Ctrl Pts',(-0.0135975102589157,-0.0303629840392982,
-0.0132620568278614));
#20826=CARTESIAN_POINT('Ctrl Pts',(-0.0136384512017853,-0.0303602804252429,
-0.0132190678590793));
#20827=CARTESIAN_POINT('Ctrl Pts',(-0.0137582763463087,-0.0303519015165297,
-0.0130777691031764));
#20828=CARTESIAN_POINT('Ctrl Pts',(-0.0138276604041924,-0.0303462875962367,
-0.0129721114137639));
#20829=CARTESIAN_POINT('Ctrl Pts',(-0.013892501448283,-0.0303391167815595,
-0.0128408404528043));
#20830=CARTESIAN_POINT('Ctrl Pts',(-0.0139012024494203,-0.0303381014887717,
-0.0128223050309537));
#20831=CARTESIAN_POINT('Ctrl Pts',(-0.0139136476553152,-0.030336564344782,
-0.0127943608892424));
#20832=CARTESIAN_POINT('Ctrl Pts',(-0.0139176724491935,-0.0303360527362019,
-0.0127850791625988));
#20833=CARTESIAN_POINT('Ctrl Pts',(-0.0139247363448817,-0.0303351279353409,
-0.0127683397334666));
#20834=CARTESIAN_POINT('Ctrl Pts',(-0.0139278089085867,-0.0303347159744179,
-0.0127608964980392));
#20835=CARTESIAN_POINT('Ctrl Pts',(-0.013934237808598,-0.0303338327932478,
-0.0127449702608046));
#20836=CARTESIAN_POINT('Ctrl Pts',(-0.0139375774448333,-0.030333360992527,
-0.0127364808875621));
#20837=CARTESIAN_POINT('Ctrl Pts',(-0.0139464404684414,-0.030332072580007,
-0.0127133510215719));
#20838=CARTESIAN_POINT('Ctrl Pts',(-0.0139518166402862,-0.0303312507887524,
-0.0126986556020744));
#20839=CARTESIAN_POINT('Ctrl Pts',(-0.013982035736537,-0.0303263844984363,
-0.0126119905761492));
#20840=CARTESIAN_POINT('Ctrl Pts',(-0.0140017446732389,-0.0303221620450477,
-0.0125383528249377));
#20841=CARTESIAN_POINT('Ctrl Pts',(-0.0140339403680866,-0.0303123269729252,
-0.0123687181106948));
#20842=CARTESIAN_POINT('Ctrl Pts',(-0.0140430000000041,-0.0303066610915457,
-0.0122723917483003));
#20843=CARTESIAN_POINT('Ctrl Pts',(-0.014043,-0.0303011972027429,-0.0121758532864921));
#20844=CARTESIAN_POINT('',(-0.0140429998425021,-0.0304166482542229,-0.0121765504512336));
#20845=CARTESIAN_POINT('Ctrl Pts',(-0.014043,-0.0304166107246751,-0.0121758532865585));
#20846=CARTESIAN_POINT('Ctrl Pts',(-0.014043,-0.0304166232329507,-0.0121760856746653));
#20847=CARTESIAN_POINT('Ctrl Pts',(-0.0140429999475007,-0.0304166357427992,
-0.0121763180628743));
#20848=CARTESIAN_POINT('Ctrl Pts',(-0.0140429998425021,-0.0304166482542194,
-0.012176550451168));
#20849=CARTESIAN_POINT('Ctrl Pts',(-0.0140429998425021,-0.0304166482542229,
-0.012176550451233));
#20850=CARTESIAN_POINT('Ctrl Pts',(-0.0140429619592719,-0.0304211623406919,
-0.0122603955171862));
#20851=CARTESIAN_POINT('Ctrl Pts',(-0.0140360912751621,-0.0304258834194363,
-0.0123440778667976));
#20852=CARTESIAN_POINT('Ctrl Pts',(-0.0140055671873961,-0.0304366479657113,
-0.0125292716504272));
#20853=CARTESIAN_POINT('Ctrl Pts',(-0.0139783707368846,-0.0304427144881944,
-0.01262979022047));
#20854=CARTESIAN_POINT('Ctrl Pts',(-0.0139350373405486,-0.0304493427776151,
-0.01274314730646));
#20855=CARTESIAN_POINT('Ctrl Pts',(-0.013928517068393,-0.0304502855523705,
-0.0127593716755159));
#20856=CARTESIAN_POINT('Ctrl Pts',(-0.013919037513126,-0.0304515797528431,
-0.0127818477267646));
#20857=CARTESIAN_POINT('Ctrl Pts',(-0.0139163100750219,-0.0304519439065037,
-0.0127881951030303));
#20858=CARTESIAN_POINT('Ctrl Pts',(-0.0139115804684773,-0.0304525613027739,
-0.0127990013161171));
#20859=CARTESIAN_POINT('Ctrl Pts',(-0.0139095996028356,-0.0304528158130124,
-0.0128034692900178));
#20860=CARTESIAN_POINT('Ctrl Pts',(-0.0139054131184268,-0.0304533452192109,
-0.0128127923736308));
#20861=CARTESIAN_POINT('Ctrl Pts',(-0.0139032035354575,-0.0304536198738844,
-0.0128176455222901));
#20862=CARTESIAN_POINT('Ctrl Pts',(-0.0138972261085774,-0.0304543505385233,
-0.0128305959545962));
#20863=CARTESIAN_POINT('Ctrl Pts',(-0.0138934129969186,-0.0304548038494557,
-0.0128386722566403));
#20864=CARTESIAN_POINT('Ctrl Pts',(-0.0138756599279586,-0.0304568589575214,
-0.0128754434912595));
#20865=CARTESIAN_POINT('Ctrl Pts',(-0.0138609014823846,-0.03045841560221,
-0.0129037365874803));
#20866=CARTESIAN_POINT('Ctrl Pts',(-0.0138010752388869,-0.0304642546108091,
-0.0130102375417289));
#20867=CARTESIAN_POINT('Ctrl Pts',(-0.0137500543379166,-0.0304683129173928,
-0.0130848967692267));
#20868=CARTESIAN_POINT('Ctrl Pts',(-0.0136353052765514,-0.0304766106755115,
-0.0132247310601838));
#20869=CARTESIAN_POINT('Ctrl Pts',(-0.0135717575881666,-0.0304808382146522,
-0.0132895839546813));
#20870=CARTESIAN_POINT('Ctrl Pts',(-0.0134901096780616,-0.0304861580368334,
-0.013359413480513));
#20871=CARTESIAN_POINT('Ctrl Pts',(-0.0134771495972244,-0.0304869989658315,
-0.0133701357255105));
#20872=CARTESIAN_POINT('Ctrl Pts',(-0.0134563982816042,-0.03048834131069,
-0.0133867399609093));
#20873=CARTESIAN_POINT('Ctrl Pts',(-0.0134487218921111,-0.0304888370032319,
-0.0133927637092664));
#20874=CARTESIAN_POINT('Ctrl Pts',(-0.0134341755295528,-0.0304897749274503,
-0.0134039571062186));
#20875=CARTESIAN_POINT('Ctrl Pts',(-0.0134273184563056,-0.0304902164907762,
-0.0134091429477865));
#20876=CARTESIAN_POINT('Ctrl Pts',(-0.013411754241254,-0.0304912176370259,
-0.0134207106034591));
#20877=CARTESIAN_POINT('Ctrl Pts',(-0.0134030228031522,-0.0304917785003676,
-0.0134270588431722));
#20878=CARTESIAN_POINT('Ctrl Pts',(-0.0133769584522568,-0.0304934507747414,
-0.0134455941298333));
#20879=CARTESIAN_POINT('Ctrl Pts',(-0.0133594408169735,-0.0304945721935955,
-0.0134575160183573));
#20880=CARTESIAN_POINT('Ctrl Pts',(-0.0132502144236064,-0.0305015514381697,
-0.0135286053184794));
#20881=CARTESIAN_POINT('Ctrl Pts',(-0.0131526997912829,-0.0305077588498726,
-0.0135782569892975));
#20882=CARTESIAN_POINT('Ctrl Pts',(-0.0129910222943623,-0.0305177073603594,
-0.013640038628511));
#20883=CARTESIAN_POINT('Ctrl Pts',(-0.0129298985789664,-0.0305213891917266,
-0.0136591366264577));
#20884=CARTESIAN_POINT('Ctrl Pts',(-0.012847287824246,-0.0305261329955067,
-0.0136794106303462));
#20885=CARTESIAN_POINT('Ctrl Pts',(-0.0128267101150639,-0.0305272956823491,
-0.0136840157750318));
#20886=CARTESIAN_POINT('Ctrl Pts',(-0.0127914889665945,-0.0305292463789131,
-0.0136911432580558));
#20887=CARTESIAN_POINT('Ctrl Pts',(-0.0127768919384072,-0.0305300434060506,
-0.0136938784515484));
#20888=CARTESIAN_POINT('Ctrl Pts',(-0.0127558266730342,-0.0305311749789225,
-0.0136975116894299));
#20889=CARTESIAN_POINT('Ctrl Pts',(-0.012749389070434,-0.0305315182970713,
-0.0136985800106363));
#20890=CARTESIAN_POINT('Ctrl Pts',(-0.0127381399445833,-0.0305321136299855,
-0.0137003735520935));
#20891=CARTESIAN_POINT('Ctrl Pts',(-0.0127333314647548,-0.0305323666415984,
-0.0137011169041322));
#20892=CARTESIAN_POINT('Ctrl Pts',(-0.0127230120705358,-0.0305329064150909,
-0.0137026622552686));
#20893=CARTESIAN_POINT('Ctrl Pts',(-0.0127175002615166,-0.0305331927844787,
-0.0137034571778443));
#20894=CARTESIAN_POINT('Ctrl Pts',(-0.0127023413139607,-0.0305339753546743,
-0.0137055597180189));
#20895=CARTESIAN_POINT('Ctrl Pts',(-0.0126926857650036,-0.030534468235438,
-0.0137068059242885));
#20896=CARTESIAN_POINT('Ctrl Pts',(-0.0126387997979758,-0.0305371910099088,
-0.0137132429057405));
#20897=CARTESIAN_POINT('Ctrl Pts',(-0.0125943692337139,-0.030539331624267,
-0.0137166087139355));
#20898=CARTESIAN_POINT('Ctrl Pts',(-0.0124687799145164,-0.0305452382153818,
-0.0137206684489272));
#20899=CARTESIAN_POINT('Ctrl Pts',(-0.0123876246663945,-0.0305488914232339,
-0.0137168923349803));
#20900=CARTESIAN_POINT('Ctrl Pts',(-0.0122297503350157,-0.0305562073189009,
-0.0136970036247948));
#20901=CARTESIAN_POINT('Ctrl Pts',(-0.012153216827278,-0.0305598546769151,
-0.0136814007288479));
#20902=CARTESIAN_POINT('Ctrl Pts',(-0.0120580667638414,-0.0305647133371462,
-0.0136543599411083));
#20903=CARTESIAN_POINT('Ctrl Pts',(-0.0120380565943718,-0.0305657533452563,
-0.0136482306668853));
#20904=CARTESIAN_POINT('Ctrl Pts',(-0.0120081160877149,-0.030567339712194,
-0.0136383892327033));
#20905=CARTESIAN_POINT('Ctrl Pts',(-0.0119980888296074,-0.0305678761652763,
-0.0136349784856771));
#20906=CARTESIAN_POINT('Ctrl Pts',(-0.0119800170550744,-0.0305688526900691,
-0.0136286230922377));
#20907=CARTESIAN_POINT('Ctrl Pts',(-0.0119719603870234,-0.0305692915572097,
-0.0136257141538498));
#20908=CARTESIAN_POINT('Ctrl Pts',(-0.0119546782030701,-0.0305702407124572,
-0.0136193110971556));
#20909=CARTESIAN_POINT('Ctrl Pts',(-0.0119454611722413,-0.0305707517144472,
-0.0136157952977533));
#20910=CARTESIAN_POINT('Ctrl Pts',(-0.0119205246041696,-0.0305721475255645,
-0.01360600841255));
#20911=CARTESIAN_POINT('Ctrl Pts',(-0.0119048738205827,-0.0305730380541613,
-0.0135995668176128));
#20912=CARTESIAN_POINT('Ctrl Pts',(-0.0118039981726782,-0.0305788741519992,
-0.0135560941437535));
#20913=CARTESIAN_POINT('Ctrl Pts',(-0.0117221723859712,-0.0305840756719932,
-0.0135116912794723));
#20914=CARTESIAN_POINT('Ctrl Pts',(-0.0115573167984598,-0.0305954138837792,
-0.0134019264622939));
#20915=CARTESIAN_POINT('Ctrl Pts',(-0.0114759716208755,-0.0306015553481338,
-0.0133348504458597));
#20916=CARTESIAN_POINT('Ctrl Pts',(-0.0113893643214617,-0.0306082932068849,
-0.013247144498999));
#20917=CARTESIAN_POINT('Ctrl Pts',(-0.0113768762287884,-0.0306092696785555,
-0.0132340449150845));
#20918=CARTESIAN_POINT('Ctrl Pts',(-0.0113598569604872,-0.0306106035290679,
-0.0132155514845421));
#20919=CARTESIAN_POINT('Ctrl Pts',(-0.0113551283242698,-0.0306109744660327,
-0.0132103422151133));
#20920=CARTESIAN_POINT('Ctrl Pts',(-0.0113471469066024,-0.0306116008613769,
-0.0132014277838151));
#20921=CARTESIAN_POINT('Ctrl Pts',(-0.0113438759740372,-0.0306118576527997,
-0.0131977390646101));
#20922=CARTESIAN_POINT('Ctrl Pts',(-0.011337123927671,-0.0306123878049065,
-0.0131900506803082));
#20923=CARTESIAN_POINT('Ctrl Pts',(-0.0113336456799263,-0.0306126609625325,
-0.0131860486710185));
#20924=CARTESIAN_POINT('Ctrl Pts',(-0.0113244423662386,-0.0306133841199227,
-0.0131753486028728));
#20925=CARTESIAN_POINT('Ctrl Pts',(-0.0113187538491829,-0.0306138315092047,
-0.0131686192085097));
#20926=CARTESIAN_POINT('Ctrl Pts',(-0.0112935203378516,-0.0306158198128638,
-0.0131382445289321));
#20927=CARTESIAN_POINT('Ctrl Pts',(-0.0112746243640372,-0.0306173190145845,
-0.0131140669385898));
#20928=CARTESIAN_POINT('Ctrl Pts',(-0.0112025494906394,-0.030623149254895,
-0.013015950711378));
#20929=CARTESIAN_POINT('Ctrl Pts',(-0.0111552375424365,-0.030627243638966,
-0.0129379278292193));
#20930=CARTESIAN_POINT('Ctrl Pts',(-0.0110749422758685,-0.0306355951768532,
-0.0127744742140938));
#20931=CARTESIAN_POINT('Ctrl Pts',(-0.0110421162633324,-0.0306398394525619,
-0.0126893795270005));
#20932=CARTESIAN_POINT('Ctrl Pts',(-0.0110123478014286,-0.0306451775304189,
-0.0125857579484948));
#20933=CARTESIAN_POINT('Ctrl Pts',(-0.0110079757565,-0.0306460168988562,
-0.012569546726585));
#20934=CARTESIAN_POINT('Ctrl Pts',(-0.0110014893245516,-0.0306473562455791,
-0.012543833483475));
#20935=CARTESIAN_POINT('Ctrl Pts',(-0.0109991987531483,-0.0306478504992553,
-0.0125343770396436));
#20936=CARTESIAN_POINT('Ctrl Pts',(-0.0109950601030574,-0.0306487853506769,
-0.0125165559136453));
#20937=CARTESIAN_POINT('Ctrl Pts',(-0.0109931919416164,-0.030649225278308,
-0.0125081962491017));
#20938=CARTESIAN_POINT('Ctrl Pts',(-0.0109891373545825,-0.0306502221907669,
-0.0124893154617643));
#20939=CARTESIAN_POINT('Ctrl Pts',(-0.0109869910518902,-0.0306507804446034,
-0.012478786255466));
#20940=CARTESIAN_POINT('Ctrl Pts',(-0.0109808300539897,-0.0306524803556776,
-0.0124468616590358));
#20941=CARTESIAN_POINT('Ctrl Pts',(-0.0109771580966731,-0.0306536328500733,
-0.0124254035516808));
#20942=CARTESIAN_POINT('Ctrl Pts',(-0.0109595680137425,-0.0306600116332963,
-0.0123076804651647));
#20943=CARTESIAN_POINT('Ctrl Pts',(-0.0109543241034389,-0.0306655090689206,
-0.0122103547704631));
#20944=CARTESIAN_POINT('Ctrl Pts',(-0.0109612556957566,-0.0306753151036192,
-0.0120397967497272));
#20945=CARTESIAN_POINT('Ctrl Pts',(-0.010969476643053,-0.0306795673559181,
-0.0119667019448935));
#20946=CARTESIAN_POINT('Ctrl Pts',(-0.010987018548352,-0.0306849504049318,
-0.0118721219714775));
#20947=CARTESIAN_POINT('Ctrl Pts',(-0.0109916568000309,-0.0306862077229858,
-0.0118498679125829));
#20948=CARTESIAN_POINT('Ctrl Pts',(-0.0110003256509675,-0.0306882978728411,
-0.0118124360475416));
#20949=CARTESIAN_POINT('Ctrl Pts',(-0.0110040992278845,-0.0306891414710078,
-0.0117972028407568));
#20950=CARTESIAN_POINT('Ctrl Pts',(-0.0110098017706814,-0.0306903251657888,
-0.0117756003048406));
#20951=CARTESIAN_POINT('Ctrl Pts',(-0.0110115404366519,-0.0306906752394195,
-0.0117691822358206));
#20952=CARTESIAN_POINT('Ctrl Pts',(-0.0110146232150849,-0.0306912773937334,
-0.0117580872233235));
#20953=CARTESIAN_POINT('Ctrl Pts',(-0.0110159480480263,-0.0306915305617535,
-0.0117534050850856));
#20954=CARTESIAN_POINT('Ctrl Pts',(-0.0110188097995528,-0.0306920656357347,
-0.0117434708938957));
#20955=CARTESIAN_POINT('Ctrl Pts',(-0.0110203525251162,-0.0306923472066169,
-0.0117382206834991));
#20956=CARTESIAN_POINT('Ctrl Pts',(-0.011024670551673,-0.0306931170189241,
-0.0117238094362247));
#20957=CARTESIAN_POINT('Ctrl Pts',(-0.0110275032615779,-0.0306936020335336,
-0.0117146657022878));
#20958=CARTESIAN_POINT('Ctrl Pts',(-0.0110426153138818,-0.0306960918336743,
-0.011667444483677));
#20959=CARTESIAN_POINT('Ctrl Pts',(-0.0110562879786035,-0.0306980248142775,
-0.0116298260922532));
#20960=CARTESIAN_POINT('Ctrl Pts',(-0.0111033029854586,-0.0307039044634106,
-0.0115146344757925));
#20961=CARTESIAN_POINT('Ctrl Pts',(-0.0111415567760878,-0.0307077024841035,
-0.0114392352185974));
#20962=CARTESIAN_POINT('Ctrl Pts',(-0.0112274929545942,-0.0307152357200265,
-0.0112995485770479));
#20963=CARTESIAN_POINT('Ctrl Pts',(-0.0112743787907372,-0.0307189517511015,
-0.0112350902162897));
#20964=CARTESIAN_POINT('Ctrl Pts',(-0.0113397333074098,-0.030723896382847,
-0.0111584661777838));
#20965=CARTESIAN_POINT('Ctrl Pts',(-0.0113537713148073,-0.0307249460144424,
-0.0111426761119587));
#20966=CARTESIAN_POINT('Ctrl Pts',(-0.0113753531124075,-0.0307265441084047,
-0.0111193820975619));
#20967=CARTESIAN_POINT('Ctrl Pts',(-0.0113826578108055,-0.0307270824316285,
-0.0111116594978831));
#20968=CARTESIAN_POINT('Ctrl Pts',(-0.0113959929561588,-0.0307280608851821,
-0.0110978501101519));
#20969=CARTESIAN_POINT('Ctrl Pts',(-0.0114019954527315,-0.0307284997866218,
-0.0110917368668703));
#20970=CARTESIAN_POINT('Ctrl Pts',(-0.0114149967993361,-0.030729447352476,
-0.0110787143845922));
#20971=CARTESIAN_POINT('Ctrl Pts',(-0.0114220113940059,-0.0307299567116823,
-0.0110718214595818));
#20972=CARTESIAN_POINT('Ctrl Pts',(-0.0114411804004771,-0.0307313438491194,
-0.0110533418049822));
#20973=CARTESIAN_POINT('Ctrl Pts',(-0.0114534586045064,-0.0307322272300015,
-0.0110418858937261));
#20974=CARTESIAN_POINT('Ctrl Pts',(-0.0115348687414218,-0.0307380531965798,
-0.0109683764485705));
#20975=CARTESIAN_POINT('Ctrl Pts',(-0.0116092877460205,-0.0307432517697466,
-0.0109124824317057));
#20976=CARTESIAN_POINT('Ctrl Pts',(-0.0117777427553323,-0.0307545884299237,
-0.0108082780066903));
#20977=CARTESIAN_POINT('Ctrl Pts',(-0.0118726434709606,-0.0307607315589126,
-0.010762225704277));
#20978=CARTESIAN_POINT('Ctrl Pts',(-0.0119883950716518,-0.030767464384224,
-0.0107200260264546));
#20979=CARTESIAN_POINT('Ctrl Pts',(-0.0120054033895746,-0.0307684348701076,
-0.0107141601375789));
#20980=CARTESIAN_POINT('Ctrl Pts',(-0.0120291885079166,-0.0307697621975758,
-0.0107064197736644));
#20981=CARTESIAN_POINT('Ctrl Pts',(-0.012035880805606,-0.0307701324089196,
-0.0107042923170377));
#20982=CARTESIAN_POINT('Ctrl Pts',(-0.0120472965931817,-0.0307707581089296,
-0.0107007489047131));
#20983=CARTESIAN_POINT('Ctrl Pts',(-0.0120520127416988,-0.0307710149191941,
-0.0106993097786609));
#20984=CARTESIAN_POINT('Ctrl Pts',(-0.0120618273026738,-0.0307715457612612,
-0.0106963662328868));
#20985=CARTESIAN_POINT('Ctrl Pts',(-0.0120669266884168,-0.030771819583202,
-0.010694865520531));
#20986=CARTESIAN_POINT('Ctrl Pts',(-0.0120805421215145,-0.0307725456422034,
-0.0106909349343394));
#20987=CARTESIAN_POINT('Ctrl Pts',(-0.0120890716209946,-0.0307729952389376,
-0.0106885519388215));
#20988=CARTESIAN_POINT('Ctrl Pts',(-0.0121276388578793,-0.0307750064555578,
-0.0106781340281651));
#20989=CARTESIAN_POINT('Ctrl Pts',(-0.0121578964739101,-0.0307765252451901,
-0.0106709342820215));
#20990=CARTESIAN_POINT('Ctrl Pts',(-0.012277221589053,-0.0307823564303481,
-0.0106463264540505));
#20991=CARTESIAN_POINT('Ctrl Pts',(-0.0123675392354059,-0.0307864369814528,
-0.0106358731519739));
#20992=CARTESIAN_POINT('Ctrl Pts',(-0.0125490537754813,-0.0307947659468167,
-0.0106309607689021));
#20993=CARTESIAN_POINT('Ctrl Pts',(-0.0126398834516143,-0.0307990017912982,
-0.0106365256891552));
#20994=CARTESIAN_POINT('Ctrl Pts',(-0.0127462966141307,-0.0308043302083165,
-0.0106525447049422));
#20995=CARTESIAN_POINT('Ctrl Pts',(-0.0127628616879551,-0.030805169853775,
-0.0106553156309625));
#20996=CARTESIAN_POINT('Ctrl Pts',(-0.0127889539324155,-0.0308065098558042,
-0.0106601193274885));
#20997=CARTESIAN_POINT('Ctrl Pts',(-0.0127985129744181,-0.0308070044923971,
-0.0106619729054995));
#20998=CARTESIAN_POINT('Ctrl Pts',(-0.0128164560618017,-0.0308079402117008,
-0.0106656287696141));
#20999=CARTESIAN_POINT('Ctrl Pts',(-0.0128248438973218,-0.0308083806253845,
-0.0106674107225067));
#21000=CARTESIAN_POINT('Ctrl Pts',(-0.0128437235527055,-0.0308093788468724,
-0.0106715863815443));
#21001=CARTESIAN_POINT('Ctrl Pts',(-0.0128542059869155,-0.0308099379277745,
-0.0106740201023731));
#21002=CARTESIAN_POINT('Ctrl Pts',(-0.0128851609110074,-0.03081160359428,
-0.0106815490540761));
#21003=CARTESIAN_POINT('Ctrl Pts',(-0.0129055547445077,-0.0308127201236252,
-0.0106869545807193));
#21004=CARTESIAN_POINT('Ctrl Pts',(-0.0130325293218204,-0.0308197945049652,
-0.0107234123468547));
#21005=CARTESIAN_POINT('Ctrl Pts',(-0.0131355953217276,-0.0308261170557336,
-0.0107654690165223));
#21006=CARTESIAN_POINT('Ctrl Pts',(-0.0132890159889861,-0.0308361480421952,
-0.0108483289663659));
#21007=CARTESIAN_POINT('Ctrl Pts',(-0.0133428826814456,-0.0308397973145065,
-0.0108818608243822));
#21008=CARTESIAN_POINT('Ctrl Pts',(-0.0134116219889735,-0.0308445030601893,
-0.0109307693202668));
#21009=CARTESIAN_POINT('Ctrl Pts',(-0.0134284593864447,-0.0308456596245896,
-0.0109432738882543));
#21010=CARTESIAN_POINT('Ctrl Pts',(-0.0134567215558228,-0.0308476006057915,
-0.0109651711068409));
#21011=CARTESIAN_POINT('Ctrl Pts',(-0.0134682755582404,-0.0308483939966565,
-0.0109743916972974));
#21012=CARTESIAN_POINT('Ctrl Pts',(-0.0134847150887634,-0.0308495204899492,
-0.010987902359445));
#21013=CARTESIAN_POINT('Ctrl Pts',(-0.0134897084787755,-0.0308498623307743,
-0.0109920592414255));
#21014=CARTESIAN_POINT('Ctrl Pts',(-0.0134983819025579,-0.0308504553007776,
-0.0109993729079864));
#21015=CARTESIAN_POINT('Ctrl Pts',(-0.013502073536278,-0.0308507074190815,
-0.0110025156818494));
#21016=CARTESIAN_POINT('Ctrl Pts',(-0.0135099648380958,-0.0308512457214186,
-0.0110092981410806));
#21017=CARTESIAN_POINT('Ctrl Pts',(-0.0135141597046751,-0.0308515315098546,
-0.0110129431537756));
#21018=CARTESIAN_POINT('Ctrl Pts',(-0.0135256275228104,-0.0308523120799809,
-0.0110230170417338));
#21019=CARTESIAN_POINT('Ctrl Pts',(-0.0135328597583993,-0.0308528035570709,
-0.0110294921080602));
#21020=CARTESIAN_POINT('Ctrl Pts',(-0.013572648899753,-0.0308555061701469,
-0.0110657978330293));
#21021=CARTESIAN_POINT('Ctrl Pts',(-0.013603977222896,-0.0308576293819689,
-0.0110969493681308));
#21022=CARTESIAN_POINT('Ctrl Pts',(-0.0136891656692589,-0.0308635356374126,
-0.0111892592360783));
#21023=CARTESIAN_POINT('Ctrl Pts',(-0.0137395790253832,-0.0308672026279364,
-0.0112533958816029));
#21024=CARTESIAN_POINT('Ctrl Pts',(-0.013828008975108,-0.0308745408381592,
-0.0113863239956194));
#21025=CARTESIAN_POINT('Ctrl Pts',(-0.0138663073724793,-0.0308781963844657,
-0.0114546272955443));
#21026=CARTESIAN_POINT('Ctrl Pts',(-0.0139080908935563,-0.0308830653584843,
-0.011544530967795));
#21027=CARTESIAN_POINT('Ctrl Pts',(-0.0139165318193202,-0.0308841063692228,
-0.0115637051127779));
#21028=CARTESIAN_POINT('Ctrl Pts',(-0.0139286487403395,-0.0308856937539192,
-0.0115928233061177));
#21029=CARTESIAN_POINT('Ctrl Pts',(-0.0139326170781135,-0.0308862301864663,
-0.0116026434806445));
#21030=CARTESIAN_POINT('Ctrl Pts',(-0.0139396093889504,-0.0308872064059661,
-0.0116204731555862));
#21031=CARTESIAN_POINT('Ctrl Pts',(-0.0139426684200045,-0.0308876449847313,
-0.0116284684962802));
#21032=CARTESIAN_POINT('Ctrl Pts',(-0.0139491048155499,-0.0308885932070914,
-0.0116457199913139));
#21033=CARTESIAN_POINT('Ctrl Pts',(-0.0139524603565234,-0.0308891035605338,
-0.0116549838366586));
#21034=CARTESIAN_POINT('Ctrl Pts',(-0.0139613261152707,-0.0308904968068033,
-0.0116802120876568));
#21035=CARTESIAN_POINT('Ctrl Pts',(-0.0139666632167006,-0.0308913853925636,
-0.0116962355311076));
#21036=CARTESIAN_POINT('Ctrl Pts',(-0.0140000051271375,-0.03089728200354,
-0.0118021026232651));
#21037=CARTESIAN_POINT('Ctrl Pts',(-0.0140199994568309,-0.0309025532529568,
-0.0118942471776128));
#21038=CARTESIAN_POINT('Ctrl Pts',(-0.0140391534379602,-0.0309115449730766,
-0.0120500901012688));
#21039=CARTESIAN_POINT('Ctrl Pts',(-0.0140430000007467,-0.0309151869899036,
-0.0121129498483668));
#21040=CARTESIAN_POINT('Ctrl Pts',(-0.014043,-0.0309187674097093,-0.0121758533048748));
#21041=CARTESIAN_POINT('Origin',(-0.0125,-0.0375520664398416,-0.0121758532865581));
#21042=CARTESIAN_POINT('',(-0.014043,-0.0314187998068562,-0.0121758533148101));
#21043=CARTESIAN_POINT('',(-0.014043,-0.0313028240247934,-0.012175853286558));
#21044=CARTESIAN_POINT('',(-0.014043,-0.0375520664398416,-0.012175853286558));
#21045=CARTESIAN_POINT('Ctrl Pts',(-0.014043,-0.0313028240247934,-0.012175853286558));
#21046=CARTESIAN_POINT('Ctrl Pts',(-0.014043,-0.0313005190170936,-0.0121265275259863));
#21047=CARTESIAN_POINT('Ctrl Pts',(-0.0140406347849488,-0.0312981692539751,
-0.0120772051756399));
#21048=CARTESIAN_POINT('Ctrl Pts',(-0.0140338217440674,-0.0312946809599502,
-0.0120064041507614));
#21049=CARTESIAN_POINT('Ctrl Pts',(-0.0140312806644925,-0.0312936011312428,
-0.0119847993155959));
#21050=CARTESIAN_POINT('Ctrl Pts',(-0.0140268066319898,-0.0312919676677619,
-0.0119526371310362));
#21051=CARTESIAN_POINT('Ctrl Pts',(-0.0140252188406569,-0.031291424927535,
-0.0119420340740226));
#21052=CARTESIAN_POINT('Ctrl Pts',(-0.0140221682962787,-0.0312904436278096,
-0.0119230182053871));
#21053=CARTESIAN_POINT('Ctrl Pts',(-0.0140207459527931,-0.0312900063722433,
-0.0119145993035507));
#21054=CARTESIAN_POINT('Ctrl Pts',(-0.0140175605185017,-0.0312890681217481,
-0.0118966527277991));
#21055=CARTESIAN_POINT('Ctrl Pts',(-0.0140157774145337,-0.0312885665028,
-0.0118871290181793));
#21056=CARTESIAN_POINT('Ctrl Pts',(-0.0140106781529482,-0.0312871927391396,
-0.0118612436754009));
#21057=CARTESIAN_POINT('Ctrl Pts',(-0.0140071860355736,-0.0312863149998045,
-0.0118449183778706));
#21058=CARTESIAN_POINT('Ctrl Pts',(-0.0139834471966939,-0.0312807148054992,
-0.0117421255008378));
#21059=CARTESIAN_POINT('Ctrl Pts',(-0.0139560348964219,-0.0312757595954976,
-0.0116574964101312));
#21060=CARTESIAN_POINT('Ctrl Pts',(-0.0138875438819905,-0.0312656985551237,
-0.0114952698372967));
#21061=CARTESIAN_POINT('Ctrl Pts',(-0.0138468197716936,-0.0312606167738904,
-0.0114178634818881));
#21062=CARTESIAN_POINT('Ctrl Pts',(-0.0137803875331701,-0.0312536983617118,
-0.0113140238327408));
#21063=CARTESIAN_POINT('Ctrl Pts',(-0.0137599529244731,-0.031251714526073,
-0.0112844155522293));
#21064=CARTESIAN_POINT('Ctrl Pts',(-0.0137329721680036,-0.0312492939318396,
-0.0112481062528848));
#21065=CARTESIAN_POINT('Ctrl Pts',(-0.0137273763371305,-0.0312488019098052,
-0.0112407157240016));
#21066=CARTESIAN_POINT('Ctrl Pts',(-0.0137184210559769,-0.0312480307572239,
-0.0112291071766932));
#21067=CARTESIAN_POINT('Ctrl Pts',(-0.0137151056003922,-0.0312477486939512,
-0.0112248556799171));
#21068=CARTESIAN_POINT('Ctrl Pts',(-0.0137087556794671,-0.0312472151110408,
-0.0112168004298651));
#21069=CARTESIAN_POINT('Ctrl Pts',(-0.0137057254418329,-0.0312469633209034,
-0.0112129935700234));
#21070=CARTESIAN_POINT('Ctrl Pts',(-0.0136984538037513,-0.0312463657082569,
-0.011203946434757));
#21071=CARTESIAN_POINT('Ctrl Pts',(-0.0136941959271362,-0.0312460210537556,
-0.0111987194476353));
#21072=CARTESIAN_POINT('Ctrl Pts',(-0.0136795084245081,-0.0312448494325104,
-0.0111809284147174));
#21073=CARTESIAN_POINT('Ctrl Pts',(-0.0136689133758189,-0.0312440336178028,
-0.011168501717371));
#21074=CARTESIAN_POINT('Ctrl Pts',(-0.0136422593199032,-0.0312420458234462,
-0.0111382266894987));
#21075=CARTESIAN_POINT('Ctrl Pts',(-0.0136259769468366,-0.0312408869670091,
-0.0111205801846117));
#21076=CARTESIAN_POINT('Ctrl Pts',(-0.0135524081518246,-0.0312358524697818,
-0.0110444901932278));
#21077=CARTESIAN_POINT('Ctrl Pts',(-0.0134909347650257,-0.0312321580340759,
-0.0109902753235302));
#21078=CARTESIAN_POINT('Ctrl Pts',(-0.0133559939598241,-0.0312244326390659,
-0.010889129713864));
#21079=CARTESIAN_POINT('Ctrl Pts',(-0.0132822749709674,-0.0312204048739834,
-0.01084302651057));
#21080=CARTESIAN_POINT('Ctrl Pts',(-0.0131858139626322,-0.0312150855436296,
-0.0107934722996522));
#21081=CARTESIAN_POINT('Ctrl Pts',(-0.0131663455494081,-0.0312140103464438,
-0.0107839834884451));
#21082=CARTESIAN_POINT('Ctrl Pts',(-0.0131369669927512,-0.0312123825279386,
-0.0107704221782014));
#21083=CARTESIAN_POINT('Ctrl Pts',(-0.01312720327993,-0.0312118406869284,
-0.0107660378417762));
#21084=CARTESIAN_POINT('Ctrl Pts',(-0.0131095713611014,-0.0312108603544565,
-0.0107583397483868));
#21085=CARTESIAN_POINT('Ctrl Pts',(-0.0131017197167644,-0.0312104231556606,
-0.0107549890236042));
#21086=CARTESIAN_POINT('Ctrl Pts',(-0.0130848864820876,-0.0312094843018567,
-0.0107479699147983));
#21087=CARTESIAN_POINT('Ctrl Pts',(-0.0130758973173038,-0.0312089820147118,
-0.0107443207530781));
#21088=CARTESIAN_POINT('Ctrl Pts',(-0.0130512943288748,-0.0312076045266062,
-0.0107346023788394));
#21089=CARTESIAN_POINT('Ctrl Pts',(-0.0130356154374764,-0.031206723680201,
-0.0107287023997226));
#21090=CARTESIAN_POINT('Ctrl Pts',(-0.0129342466001967,-0.031201007907147,
-0.0106924302429863));
#21091=CARTESIAN_POINT('Ctrl Pts',(-0.0128461220448033,-0.031195928251443,
-0.0106694305730379));
#21092=CARTESIAN_POINT('Ctrl Pts',(-0.0126669335673251,-0.0311855366367846,
-0.0106392232659509));
#21093=CARTESIAN_POINT('Ctrl Pts',(-0.0125762113815732,-0.0311802471659527,
-0.0106320622022023));
#21094=CARTESIAN_POINT('Ctrl Pts',(-0.0124543255623496,-0.0311734452865964,
-0.0106332166961741));
#21095=CARTESIAN_POINT('Ctrl Pts',(-0.0124232795539096,-0.0311717406208604,
-0.0106344487245602));
#21096=CARTESIAN_POINT('Ctrl Pts',(-0.0123834825228855,-0.0311696089553695,
-0.0106372335706211));
#21097=CARTESIAN_POINT('Ctrl Pts',(-0.0123746802217776,-0.0311691408530085,
-0.0106379254881434));
#21098=CARTESIAN_POINT('Ctrl Pts',(-0.0123606093942982,-0.0311683985144417,
-0.0106391531551615));
#21099=CARTESIAN_POINT('Ctrl Pts',(-0.0123553369690545,-0.0311681216923717,
-0.010639640526576));
#21100=CARTESIAN_POINT('Ctrl Pts',(-0.0123451854952486,-0.0311675914182987,
-0.0106406316328125));
#21101=CARTESIAN_POINT('Ctrl Pts',(-0.0123403062233601,-0.0311673377695546,
-0.0106411315023298));
#21102=CARTESIAN_POINT('Ctrl Pts',(-0.0123284948285749,-0.0311667265721093,
-0.0106423984885686));
#21103=CARTESIAN_POINT('Ctrl Pts',(-0.0123215652740173,-0.0311663703395413,
-0.010643189365978));
#21104=CARTESIAN_POINT('Ctrl Pts',(-0.0122969636725558,-0.0311651132311436,
-0.0106461662858608));
#21105=CARTESIAN_POINT('Ctrl Pts',(-0.0122793237856051,-0.0311642258140123,
-0.0106486112855031));
#21106=CARTESIAN_POINT('Ctrl Pts',(-0.0121583326540826,-0.0311582114863341,
-0.0106675215962063));
#21107=CARTESIAN_POINT('Ctrl Pts',(-0.0120568375989976,-0.031153516538237,
-0.0106941607960075));
#21108=CARTESIAN_POINT('Ctrl Pts',(-0.011870697009067,-0.0311444087027044,
-0.0107638758042902));
#21109=CARTESIAN_POINT('Ctrl Pts',(-0.0117857906274547,-0.0311400321842557,
-0.0108048663533));
#21110=CARTESIAN_POINT('Ctrl Pts',(-0.0116908961306411,-0.0311345506455391,
-0.0108618987205334));
#21111=CARTESIAN_POINT('Ctrl Pts',(-0.0116767792295656,-0.0311337192033832,
-0.0108706968939959));
#21112=CARTESIAN_POINT('Ctrl Pts',(-0.0116545998468666,-0.0311323859911732,
-0.0108850229120981));
#21113=CARTESIAN_POINT('Ctrl Pts',(-0.0116464427123398,-0.0311318897542957,
-0.0108904022274014));
#21114=CARTESIAN_POINT('Ctrl Pts',(-0.0116312619504509,-0.0311309548612989,
-0.0109006215631267));
#21115=CARTESIAN_POINT('Ctrl Pts',(-0.0116242262729878,-0.0311305169182789,
-0.0109054430684162));
#21116=CARTESIAN_POINT('Ctrl Pts',(-0.0116085343097703,-0.0311295294932626,
-0.0109163889730781));
#21117=CARTESIAN_POINT('Ctrl Pts',(-0.0115999005113475,-0.0311289788167575,
-0.0109225447304792));
#21118=CARTESIAN_POINT('Ctrl Pts',(-0.0115742441204289,-0.0311273198262368,
-0.0109412391678987));
#21119=CARTESIAN_POINT('Ctrl Pts',(-0.0115574155588669,-0.0311262014037959,
-0.0109540388644997));
#21120=CARTESIAN_POINT('Ctrl Pts',(-0.0114781619539282,-0.0311207854773813,
-0.0110169306531468));
#21121=CARTESIAN_POINT('Ctrl Pts',(-0.0114194415795425,-0.0311163109085506,
-0.0110714777212019));
#21122=CARTESIAN_POINT('Ctrl Pts',(-0.0113074279156442,-0.031106870717989,
-0.0111930533605935));
#21123=CARTESIAN_POINT('Ctrl Pts',(-0.0112549350824193,-0.031101908248443,
-0.0112604641424284));
#21124=CARTESIAN_POINT('Ctrl Pts',(-0.0111870507173682,-0.0310949224586195,
-0.0113643609691927));
#21125=CARTESIAN_POINT('Ctrl Pts',(-0.0111670518366827,-0.0310927752266633,
-0.0113976468630364));
#21126=CARTESIAN_POINT('Ctrl Pts',(-0.0111437602459878,-0.0310901894747661,
-0.011439950822192));
#21127=CARTESIAN_POINT('Ctrl Pts',(-0.0111392685022474,-0.0310896864884867,
-0.0114482898822647));
#21128=CARTESIAN_POINT('Ctrl Pts',(-0.0111323202740601,-0.0310889021407934,
-0.0114614789367094));
#21129=CARTESIAN_POINT('Ctrl Pts',(-0.0111298122170721,-0.0310886176822952,
-0.0114663013252655));
#21130=CARTESIAN_POINT('Ctrl Pts',(-0.0111251139595864,-0.0310880824073191,
-0.011475452750135));
#21131=CARTESIAN_POINT('Ctrl Pts',(-0.0111229186460618,-0.0310878312878547,
-0.0114797789511274));
#21132=CARTESIAN_POINT('Ctrl Pts',(-0.0111177632486421,-0.031087239042276,
-0.0114900583000764));
#21133=CARTESIAN_POINT('Ctrl Pts',(-0.0111148211425578,-0.0310868990256422,
-0.0114960204127502));
#21134=CARTESIAN_POINT('Ctrl Pts',(-0.0111050326269539,-0.031085760227282,
-0.0115161839940852));
#21135=CARTESIAN_POINT('Ctrl Pts',(-0.0110983651551519,-0.0310849717737282,
-0.0115304717364148));
#21136=CARTESIAN_POINT('Ctrl Pts',(-0.0110825561425577,-0.0310830640951102,
-0.0115657500526432));
#21137=CARTESIAN_POINT('Ctrl Pts',(-0.011073660356683,-0.0310819566575063,
-0.0115868470458324));
#21138=CARTESIAN_POINT('Ctrl Pts',(-0.0110377984019296,-0.0310773091971512,
-0.0116774789781477));
#21139=CARTESIAN_POINT('Ctrl Pts',(-0.0110154216321738,-0.03107392375148,
-0.0117487247801976));
#21140=CARTESIAN_POINT('Ctrl Pts',(-0.01097626581616,-0.0310661315592871,
-0.0119145757500195));
#21141=CARTESIAN_POINT('Ctrl Pts',(-0.0109629844860348,-0.0310617159960887,
-0.0120096817091262));
#21142=CARTESIAN_POINT('Ctrl Pts',(-0.0109576162560431,-0.0310559503038506,
-0.0121271249687789));
#21143=CARTESIAN_POINT('Ctrl Pts',(-0.0109570826618411,-0.0310548705814258,
-0.0121488701201978));
#21144=CARTESIAN_POINT('Ctrl Pts',(-0.0109569725114194,-0.0310532372833294,
-0.0121813386347357));
#21145=CARTESIAN_POINT('Ctrl Pts',(-0.0109570478613904,-0.0310526946015177,
-0.0121920585324064));
#21146=CARTESIAN_POINT('Ctrl Pts',(-0.0109573838690453,-0.0310517134114333,
-0.0122113125077997));
#21147=CARTESIAN_POINT('Ctrl Pts',(-0.0109576036693031,-0.031051276207012,
-0.012219846911247));
#21148=CARTESIAN_POINT('Ctrl Pts',(-0.0109582240675939,-0.0310503380719188,
-0.0122380612446153));
#21149=CARTESIAN_POINT('Ctrl Pts',(-0.0109586450312573,-0.0310498365173575,
-0.0122477400750566));
#21150=CARTESIAN_POINT('Ctrl Pts',(-0.0109600393977087,-0.0310484629485315,
-0.0122740823602664));
#21151=CARTESIAN_POINT('Ctrl Pts',(-0.0109611920708989,-0.0310475853407344,
-0.0122907346830704));
#21152=CARTESIAN_POINT('Ctrl Pts',(-0.0109701797365539,-0.031041987693695,
-0.012395801729819));
#21153=CARTESIAN_POINT('Ctrl Pts',(-0.0109853604041931,-0.031037035122964,
-0.0124834087278465));
#21154=CARTESIAN_POINT('Ctrl Pts',(-0.0110302204661157,-0.0310269812824074,
-0.0126535625986533));
#21155=CARTESIAN_POINT('Ctrl Pts',(-0.0110595705451287,-0.0310219041063863,
-0.0127358722422504));
#21156=CARTESIAN_POINT('Ctrl Pts',(-0.0111106681819876,-0.0310149827822227,
-0.0128480940182276));
#21157=CARTESIAN_POINT('Ctrl Pts',(-0.0111267659440434,-0.0310129923785422,
-0.0128803950497096));
#21158=CARTESIAN_POINT('Ctrl Pts',(-0.0111484092874477,-0.031010565137391,
-0.0129202574921695));
#21159=CARTESIAN_POINT('Ctrl Pts',(-0.011152909743729,-0.0310100726732616,
-0.0129283710108423));
#21160=CARTESIAN_POINT('Ctrl Pts',(-0.011160141437612,-0.0310093010078231,
-0.0129411356619324));
#21161=CARTESIAN_POINT('Ctrl Pts',(-0.0111628242807973,-0.0310090188667659,
-0.0129458137913819));
#21162=CARTESIAN_POINT('Ctrl Pts',(-0.0111679737966436,-0.0310084852567781,
-0.0129546850130064));
#21163=CARTESIAN_POINT('Ctrl Pts',(-0.0111704358242123,-0.0310082335159733,
-0.0129588805959455));
#21164=CARTESIAN_POINT('Ctrl Pts',(-0.0111763546002404,-0.0310076361981139,
-0.0129688584808408));
#21165=CARTESIAN_POINT('Ctrl Pts',(-0.011179829488834,-0.031007291786187,
-0.0129746299807336));
#21166=CARTESIAN_POINT('Ctrl Pts',(-0.0111918409033299,-0.0310061218476698,
-0.0129942874388786));
#21167=CARTESIAN_POINT('Ctrl Pts',(-0.0112005598606468,-0.0310053074309449,
-0.0130080612220807));
#21168=CARTESIAN_POINT('Ctrl Pts',(-0.0112226240601629,-0.0310033237572431,
-0.0130417246730382));
#21169=CARTESIAN_POINT('Ctrl Pts',(-0.0112362174672482,-0.0310021675538656,
-0.0130614470730105));
#21170=CARTESIAN_POINT('Ctrl Pts',(-0.0112980277246355,-0.0309971540684869,
-0.0131468029614563));
#21171=CARTESIAN_POINT('Ctrl Pts',(-0.0113509394552251,-0.0309934765240861,
-0.0132088789021195));
#21172=CARTESIAN_POINT('Ctrl Pts',(-0.0114758488817147,-0.0309853823298892,
-0.0133338864009991));
#21173=CARTESIAN_POINT('Ctrl Pts',(-0.0115492838821746,-0.0309809558937707,
-0.0133948949450062));
#21174=CARTESIAN_POINT('Ctrl Pts',(-0.0116416731843121,-0.0309754121445663,
-0.0134581964913626));
#21175=CARTESIAN_POINT('Ctrl Pts',(-0.0116556301136451,-0.0309745758274465,
-0.0134674292560259));
#21176=CARTESIAN_POINT('Ctrl Pts',(-0.011677988908923,-0.0309732365604675,
-0.013481702695055));
#21177=CARTESIAN_POINT('Ctrl Pts',(-0.0116862935610924,-0.0309727392322758,
-0.0134868936127972));
#21178=CARTESIAN_POINT('Ctrl Pts',(-0.0117019200456593,-0.0309718033949768,
-0.0134964554562701));
#21179=CARTESIAN_POINT('Ctrl Pts',(-0.0117092298122922,-0.0309713656136902,
-0.0135008454414439));
#21180=CARTESIAN_POINT('Ctrl Pts',(-0.0117256832486443,-0.0309703800294736,
-0.0135105421382006));
#21181=CARTESIAN_POINT('Ctrl Pts',(-0.0117348457680845,-0.0309698310511575,
-0.0135158158815605));
#21182=CARTESIAN_POINT('Ctrl Pts',(-0.0117623517470979,-0.0309681823257206,
-0.0135312736031221));
#21183=CARTESIAN_POINT('Ctrl Pts',(-0.0117808489710853,-0.0309670726544111,
-0.0135411777602971));
#21184=CARTESIAN_POINT('Ctrl Pts',(-0.0118696968007565,-0.030961736442912,
-0.0135864439912578));
#21185=CARTESIAN_POINT('Ctrl Pts',(-0.0119424760997342,-0.0309573388393052,
-0.0136167601913685));
#21186=CARTESIAN_POINT('Ctrl Pts',(-0.0120956776001367,-0.0309481341353171,
-0.0136672258043267));
#21187=CARTESIAN_POINT('Ctrl Pts',(-0.0121760589441339,-0.0309433324564841,
-0.0136867241320808));
#21188=CARTESIAN_POINT('Ctrl Pts',(-0.0122997019858036,-0.0309362604012892,
-0.0137063910731471));
#21189=CARTESIAN_POINT('Ctrl Pts',(-0.0123420526491352,-0.0309338943701879,
-0.0137113396619697));
#21190=CARTESIAN_POINT('Ctrl Pts',(-0.0123941313120377,-0.030931095948976,
-0.0137152470008867));
#21191=CARTESIAN_POINT('Ctrl Pts',(-0.0124037125345544,-0.0309305857104295,
-0.0137158759876751));
#21192=CARTESIAN_POINT('Ctrl Pts',(-0.0124188104996167,-0.0309297896015973,
-0.0137167256807697));
#21193=CARTESIAN_POINT('Ctrl Pts',(-0.0124243234717443,-0.0309295005659932,
-0.0137170062754458));
#21194=CARTESIAN_POINT('Ctrl Pts',(-0.0124346659409761,-0.0309289615968069,
-0.0137174770470344));
#21195=CARTESIAN_POINT('Ctrl Pts',(-0.0124394948270623,-0.0309287113066356,
-0.0137176741200312));
#21196=CARTESIAN_POINT('Ctrl Pts',(-0.0124508169665904,-0.0309281275309323,
-0.0137180829170477));
#21197=CARTESIAN_POINT('Ctrl Pts',(-0.0124573107200674,-0.0309277950628319,
-0.013718276325883));
#21198=CARTESIAN_POINT('Ctrl Pts',(-0.0124786578030399,-0.0309267093106307,
-0.01371877720549));
#21199=CARTESIAN_POINT('Ctrl Pts',(-0.0124935147706009,-0.0309259650759251,
-0.0137189111861308));
#21200=CARTESIAN_POINT('Ctrl Pts',(-0.012529504346246,-0.0309241850212241,
-0.0137187159144776));
#21201=CARTESIAN_POINT('Ctrl Pts',(-0.0125506330762215,-0.0309231590068975,
-0.0137181671182491));
#21202=CARTESIAN_POINT('Ctrl Pts',(-0.0126360418514792,-0.0309190654877355,
-0.0137141915793627));
#21203=CARTESIAN_POINT('Ctrl Pts',(-0.012700092534102,-0.0309161174221325,
-0.0137071782008028));
#21204=CARTESIAN_POINT('Ctrl Pts',(-0.012871342986869,-0.0309081699097549,
-0.0136774951502817));
#21205=CARTESIAN_POINT('Ctrl Pts',(-0.0129768606266926,-0.0309031799190236,
-0.0136473917860184));
#21206=CARTESIAN_POINT('Ctrl Pts',(-0.0130979618606991,-0.0308967704333187,
-0.0135984355095743));
#21207=CARTESIAN_POINT('Ctrl Pts',(-0.0131174528354949,-0.0308957176050501,
-0.0135900847065962));
#21208=CARTESIAN_POINT('Ctrl Pts',(-0.0131465645792169,-0.0308941100558627,
-0.0135768953946216));
#21209=CARTESIAN_POINT('Ctrl Pts',(-0.0131563173006883,-0.030893565478811,
-0.0135723533176647));
#21210=CARTESIAN_POINT('Ctrl Pts',(-0.0131737293795579,-0.0308925820122013,
-0.0135640214092683));
#21211=CARTESIAN_POINT('Ctrl Pts',(-0.0131814063120283,-0.0308921444469597,
-0.0135602692095438));
#21212=CARTESIAN_POINT('Ctrl Pts',(-0.0131977057952542,-0.030891206788878,
-0.0135521342080454));
#21213=CARTESIAN_POINT('Ctrl Pts',(-0.0132063190667737,-0.0308907060857857,
-0.0135477337193074));
#21214=CARTESIAN_POINT('Ctrl Pts',(-0.0132296036359554,-0.0308893380728076,
-0.0135355603097986));
#21215=CARTESIAN_POINT('Ctrl Pts',(-0.0132441914788461,-0.0308884652523189,
-0.0135276312521803));
#21216=CARTESIAN_POINT('Ctrl Pts',(-0.0133332288349783,-0.0308830385571604,
-0.0134773579121625));
#21217=CARTESIAN_POINT('Ctrl Pts',(-0.0134041636691832,-0.0308782693275541,
-0.0134291166730617));
#21218=CARTESIAN_POINT('Ctrl Pts',(-0.0135340838198056,-0.030868733716134,
-0.0133239665058592));
#21219=CARTESIAN_POINT('Ctrl Pts',(-0.0135932805261852,-0.0308639952928679,
-0.0132677465442893));
#21220=CARTESIAN_POINT('Ctrl Pts',(-0.0136772695135252,-0.0308568873207405,
-0.0131742695953239));
#21221=CARTESIAN_POINT('Ctrl Pts',(-0.0137053592258453,-0.0308544324730081,
-0.0131401708623074));
#21222=CARTESIAN_POINT('Ctrl Pts',(-0.0137377792462662,-0.0308515465744558,
-0.0130971812862224));
#21223=CARTESIAN_POINT('Ctrl Pts',(-0.0137435362833015,-0.0308510319370611,
-0.0130893959877722));
#21224=CARTESIAN_POINT('Ctrl Pts',(-0.0137524705225291,-0.0308502305148623,
-0.0130770731601995));
#21225=CARTESIAN_POINT('Ctrl Pts',(-0.0137556971352038,-0.030849940497253,
-0.0130725719587064));
#21226=CARTESIAN_POINT('Ctrl Pts',(-0.013761408353671,-0.0308494262564917,
-0.0130645133967215));
#21227=CARTESIAN_POINT('Ctrl Pts',(-0.0137639022094597,-0.0308492014100959,
-0.0130609629020573));
#21228=CARTESIAN_POINT('Ctrl Pts',(-0.0137699038301692,-0.0308486595189075,
-0.0130523413240749));
#21229=CARTESIAN_POINT('Ctrl Pts',(-0.0137733962086973,-0.0308483435160092,
-0.0130472596877231));
#21230=CARTESIAN_POINT('Ctrl Pts',(-0.0137841950752339,-0.0308473638266477,
-0.0130313430788124));
#21231=CARTESIAN_POINT('Ctrl Pts',(-0.0137913946134809,-0.0308467069408973,
-0.0130204358755078));
#21232=CARTESIAN_POINT('Ctrl Pts',(-0.013827828768116,-0.0308433559756539,
-0.0129636832785706));
#21233=CARTESIAN_POINT('Ctrl Pts',(-0.0138547661281363,-0.030840786408751,
-0.0129164037821995));
#21234=CARTESIAN_POINT('Ctrl Pts',(-0.0139248674980924,-0.0308335386331882,
-0.0127766807744706));
#21235=CARTESIAN_POINT('Ctrl Pts',(-0.013961439716183,-0.0308289842246961,
-0.0126812595850956));
#21236=CARTESIAN_POINT('Ctrl Pts',(-0.0140021511263143,-0.0308217251250766,
-0.0125324114727777));
#21237=CARTESIAN_POINT('Ctrl Pts',(-0.0140133858916283,-0.030819206517818,
-0.0124812288204585));
#21238=CARTESIAN_POINT('Ctrl Pts',(-0.014024495316186,-0.0308158496982509,
-0.0124145873610451));
#21239=CARTESIAN_POINT('Ctrl Pts',(-0.0140267724902431,-0.0308150879787133,
-0.0123995621812588));
#21240=CARTESIAN_POINT('Ctrl Pts',(-0.0140300931750389,-0.030813845652624,
-0.0123752310809937));
#21241=CARTESIAN_POINT('Ctrl Pts',(-0.0140312745770285,-0.0308133694373306,
-0.0123659448273697));
#21242=CARTESIAN_POINT('Ctrl Pts',(-0.0140333367189323,-0.0308124690384065,
-0.0123484666725585));
#21243=CARTESIAN_POINT('Ctrl Pts',(-0.0140342364899137,-0.0308120454762187,
-0.0123402773241824));
#21244=CARTESIAN_POINT('Ctrl Pts',(-0.0140359147144746,-0.0308111890925589,
-0.0123237873637089));
#21245=CARTESIAN_POINT('Ctrl Pts',(-0.0140366915631573,-0.0308107562353505,
-0.012315486869047));
#21246=CARTESIAN_POINT('Ctrl Pts',(-0.014038320504432,-0.0308097575942595,
-0.0122964174451424));
#21247=CARTESIAN_POINT('Ctrl Pts',(-0.0140391268413355,-0.030809190389752,
-0.0122856451302186));
#21248=CARTESIAN_POINT('Ctrl Pts',(-0.014041939566174,-0.0308068743987195,
-0.0122419021072547));
#21249=CARTESIAN_POINT('Ctrl Pts',(-0.0140430000000001,-0.030805096474939,
-0.0122088811687427));
#21250=CARTESIAN_POINT('Ctrl Pts',(-0.014043,-0.0308032888456207,-0.0121758532865555));
#21251=CARTESIAN_POINT('Ctrl Pts',(-0.014043,-0.0309187674097093,-0.0121758533048748));
#21252=CARTESIAN_POINT('Ctrl Pts',(-0.0140429999997999,-0.0309197267292913,
-0.0121927073390054));
#21253=CARTESIAN_POINT('Ctrl Pts',(-0.0140427238577457,-0.0309206814208278,
-0.0122095645227286));
#21254=CARTESIAN_POINT('Ctrl Pts',(-0.0140413384621183,-0.0309230574164513,
-0.0122518175606727));
#21255=CARTESIAN_POINT('Ctrl Pts',(-0.0140398782586855,-0.0309244690359173,
-0.0122771937571986));
#21256=CARTESIAN_POINT('Ctrl Pts',(-0.0140363931382051,-0.0309267847732897,
-0.0123195035874159));
#21257=CARTESIAN_POINT('Ctrl Pts',(-0.0140347132494167,-0.0309277026349426,
-0.012336460176902));
#21258=CARTESIAN_POINT('Ctrl Pts',(-0.014031962124351,-0.030928970686247,
-0.0123602123718667));
#21259=CARTESIAN_POINT('Ctrl Pts',(-0.0140311258586705,-0.0309293327863993,
-0.0123670333880292));
#21260=CARTESIAN_POINT('Ctrl Pts',(-0.0140296149479145,-0.0309299489013664,
-0.0123787107393482));
#21261=CARTESIAN_POINT('Ctrl Pts',(-0.0140289626800033,-0.0309302041436871,
-0.0123835698257165));
#21262=CARTESIAN_POINT('Ctrl Pts',(-0.0140275471559694,-0.0309307362609983,
-0.0123937467129794));
#21263=CARTESIAN_POINT('Ctrl Pts',(-0.0140267792772837,-0.0309310128789367,
-0.0123990637234993));
#21264=CARTESIAN_POINT('Ctrl Pts',(-0.0140246335990807,-0.0309317547926685,
-0.0124133916641692));
#21265=CARTESIAN_POINT('Ctrl Pts',(-0.0140232036731765,-0.0309322172402755,
-0.0124223947029267));
#21266=CARTESIAN_POINT('Ctrl Pts',(-0.0140160595552021,-0.0309343870014191,
-0.012464938041969));
#21267=CARTESIAN_POINT('Ctrl Pts',(-0.0140093164845565,-0.0309360427540956,
-0.0124982980427139));
#21268=CARTESIAN_POINT('Ctrl Pts',(-0.0139810469113904,-0.030941888174126,
-0.0126176772879945));
#21269=CARTESIAN_POINT('Ctrl Pts',(-0.0139532205792408,-0.0309458753313444,
-0.0127020283231891));
#21270=CARTESIAN_POINT('Ctrl Pts',(-0.0138830248715679,-0.0309540546000406,
-0.0128658643282637));
#21271=CARTESIAN_POINT('Ctrl Pts',(-0.0138406470350087,-0.030958236270876,
-0.0129449672449545));
#21272=CARTESIAN_POINT('Ctrl Pts',(-0.0137824822075436,-0.0309635013414945,
-0.0130339729371519));
#21273=CARTESIAN_POINT('Ctrl Pts',(-0.0137730851630063,-0.0309643393753712,
-0.0130478533366812));
#21274=CARTESIAN_POINT('Ctrl Pts',(-0.0137578787239697,-0.0309656773985198,
-0.0130695449510751));
#21275=CARTESIAN_POINT('Ctrl Pts',(-0.0137522182108292,-0.0309661716973291,
-0.0130774591994918));
#21276=CARTESIAN_POINT('Ctrl Pts',(-0.0137414283646035,-0.0309671071460843,
-0.0130922473977398));
#21277=CARTESIAN_POINT('Ctrl Pts',(-0.0137363158197064,-0.0309675476317604,
-0.0130991331690595));
#21278=CARTESIAN_POINT('Ctrl Pts',(-0.0137246525950884,-0.0309685465186392,
-0.0131145710639826));
#21279=CARTESIAN_POINT('Ctrl Pts',(-0.0137180692685168,-0.0309691061996272,
-0.0131230978660948));
#21280=CARTESIAN_POINT('Ctrl Pts',(-0.0136982971299149,-0.0309707753298544,
-0.0131481599935476));
#21281=CARTESIAN_POINT('Ctrl Pts',(-0.0136848573908443,-0.0309718947833409,
-0.0131644933865907));
#21282=CARTESIAN_POINT('Ctrl Pts',(-0.013599607983548,-0.0309789066292323,
-0.013263861633095));
#21283=CARTESIAN_POINT('Ctrl Pts',(-0.0135194521904476,-0.0309851545951428,
-0.0133393009105908));
#21284=CARTESIAN_POINT('Ctrl Pts',(-0.0133808170987185,-0.0309951608916098,
-0.0134443691810781));
#21285=CARTESIAN_POINT('Ctrl Pts',(-0.0133272741725891,-0.0309988588622458,
-0.0134799197867874));
#21286=CARTESIAN_POINT('Ctrl Pts',(-0.0132533798821043,-0.0310036199124827,
-0.0135225952334969));
#21287=CARTESIAN_POINT('Ctrl Pts',(-0.0132348737252259,-0.0310047851272844,
-0.0135327820979586));
#21288=CARTESIAN_POINT('Ctrl Pts',(-0.0132030001029772,-0.0310067390190267,
-0.0135494837710494));
#21289=CARTESIAN_POINT('Ctrl Pts',(-0.0131897372243734,-0.0310075368144819,
-0.0135561910879665));
#21290=CARTESIAN_POINT('Ctrl Pts',(-0.0131705263658104,-0.0310086683968085,
-0.01356556037592));
#21291=CARTESIAN_POINT('Ctrl Pts',(-0.0131646555701357,-0.0310090110245991,
-0.0135683777486628));
#21292=CARTESIAN_POINT('Ctrl Pts',(-0.0131543807138519,-0.0310096049105123,
-0.013573228830074));
#21293=CARTESIAN_POINT('Ctrl Pts',(-0.0131499846347196,-0.031009857166506,
-0.0135752790634877));
#21294=CARTESIAN_POINT('Ctrl Pts',(-0.0131405376316122,-0.0310103952635411,
-0.0135796308146671));
#21295=CARTESIAN_POINT('Ctrl Pts',(-0.0131354839011096,-0.0310106807144809,
-0.0135819258377602));
#21296=CARTESIAN_POINT('Ctrl Pts',(-0.0131215875496647,-0.0310114593267562,
-0.0135881462857946));
#21297=CARTESIAN_POINT('Ctrl Pts',(-0.0131127200845871,-0.0310119492118839,
-0.013592015955395));
#21298=CARTESIAN_POINT('Ctrl Pts',(-0.013063767907049,-0.0310146185447421,
-0.0136128322959929));
#21299=CARTESIAN_POINT('Ctrl Pts',(-0.0130230134595776,-0.0310167126499927,
-0.0136281619406473));
#21300=CARTESIAN_POINT('Ctrl Pts',(-0.01290386020267,-0.0310226143502235,
-0.0136673131991004));
#21301=CARTESIAN_POINT('Ctrl Pts',(-0.0128241435143882,-0.0310263011890831,
-0.0136866437324693));
#21302=CARTESIAN_POINT('Ctrl Pts',(-0.012665844421335,-0.0310336686199884,
-0.0137119169659547));
#21303=CARTESIAN_POINT('Ctrl Pts',(-0.0125875982687394,-0.0310373329892026,
-0.0137183580556447));
#21304=CARTESIAN_POINT('Ctrl Pts',(-0.0124882326912814,-0.0310422129895159,
-0.013718950971472));
#21305=CARTESIAN_POINT('Ctrl Pts',(-0.0124672587562583,-0.0310432552753258,
-0.0137186484423189));
#21306=CARTESIAN_POINT('Ctrl Pts',(-0.0124357069778531,-0.0310448442603338,
-0.0137175496624171));
#21307=CARTESIAN_POINT('Ctrl Pts',(-0.0124251201090016,-0.0310453809899061,
-0.0137170717339816));
#21308=CARTESIAN_POINT('Ctrl Pts',(-0.0124059903499639,-0.031046357579604,
-0.013716010581419));
#21309=CARTESIAN_POINT('Ctrl Pts',(-0.0123974457426624,-0.03104679622856,
-0.0137154652271415));
#21310=CARTESIAN_POINT('Ctrl Pts',(-0.0123790810876162,-0.0310477444113113,
-0.013714139558045));
#21311=CARTESIAN_POINT('Ctrl Pts',(-0.0123692631224394,-0.0310482546528639,
-0.013713336261814));
#21312=CARTESIAN_POINT('Ctrl Pts',(-0.0123426482946646,-0.0310496471127105,
-0.0137109018930533));
#21313=CARTESIAN_POINT('Ctrl Pts',(-0.0123258697440226,-0.031050535011485,
-0.0137090892132329));
#21314=CARTESIAN_POINT('Ctrl Pts',(-0.012216813550849,-0.031056373395258,
-0.0136954941044142));
#21315=CARTESIAN_POINT('Ctrl Pts',(-0.0121257454425382,-0.0310615806010856,
-0.0136756638961651));
#21316=CARTESIAN_POINT('Ctrl Pts',(-0.0119600813405946,-0.0310715218734116,
-0.0136235561292637));
#21317=CARTESIAN_POINT('Ctrl Pts',(-0.0118851501116786,-0.0310762074079022,
-0.0135933565807054));
#21318=CARTESIAN_POINT('Ctrl Pts',(-0.0117900448187887,-0.0310821782538876,
-0.0135460596560954));
#21319=CARTESIAN_POINT('Ctrl Pts',(-0.0117674517988811,-0.0310835978162309,
-0.0135341150823386));
#21320=CARTESIAN_POINT('Ctrl Pts',(-0.0117302459833056,-0.0310859250798677,
-0.0135132464042558));
#21321=CARTESIAN_POINT('Ctrl Pts',(-0.011715466625256,-0.0310868466852827,
-0.0135046305549598));
#21322=CARTESIAN_POINT('Ctrl Pts',(-0.0116949451066805,-0.0310881189824366,
-0.0134922054412082));
#21323=CARTESIAN_POINT('Ctrl Pts',(-0.01168908100374,-0.0310884816851732,
-0.0134886010770101));
#21324=CARTESIAN_POINT('Ctrl Pts',(-0.0116790798933332,-0.031089098515078,
-0.0134823613173361));
#21325=CARTESIAN_POINT('Ctrl Pts',(-0.0116749310045456,-0.0310893538766728,
-0.0134797452342304));
#21326=CARTESIAN_POINT('Ctrl Pts',(-0.011666267956283,-0.0310898858840773,
-0.0134742248394573));
#21327=CARTESIAN_POINT('Ctrl Pts',(-0.0116617564013197,-0.0310901622765562,
-0.0134713167098475));
#21328=CARTESIAN_POINT('Ctrl Pts',(-0.0116496410565979,-0.0310909029549704,
-0.0134634174184723));
#21329=CARTESIAN_POINT('Ctrl Pts',(-0.0116420659629052,-0.0310913644087414,
-0.0134583823981348));
#21330=CARTESIAN_POINT('Ctrl Pts',(-0.0116065589249322,-0.0310935217388308,
-0.0134343261755774));
#21331=CARTESIAN_POINT('Ctrl Pts',(-0.0115792105544783,-0.0310951667641105,
-0.0134144565560531));
#21332=CARTESIAN_POINT('Ctrl Pts',(-0.0114824342448742,-0.0311010109886243,
-0.0133391663908452));
#21333=CARTESIAN_POINT('Ctrl Pts',(-0.0114171692275707,-0.031105005431088,
-0.0132786754863899));
#21334=CARTESIAN_POINT('Ctrl Pts',(-0.0112971988020621,-0.0311131963200409,
-0.0131465023820683));
#21335=CARTESIAN_POINT('Ctrl Pts',(-0.0112428369460793,-0.0311173821542475,
-0.0130749801744246));
#21336=CARTESIAN_POINT('Ctrl Pts',(-0.0111860523406025,-0.0311226520673691,
-0.0129849710500098));
#21337=CARTESIAN_POINT('Ctrl Pts',(-0.0111773398722174,-0.0311234901848296,
-0.0129706489618191));
#21338=CARTESIAN_POINT('Ctrl Pts',(-0.0111639419606316,-0.0311248282860984,
-0.012947794080044));
#21339=CARTESIAN_POINT('Ctrl Pts',(-0.0111591008255313,-0.0311253225772011,
-0.0129393538245042));
#21340=CARTESIAN_POINT('Ctrl Pts',(-0.0111501438200613,-0.0311262579761414,
-0.0129233897948665));
#21341=CARTESIAN_POINT('Ctrl Pts',(-0.0111460102048364,-0.0311266984193158,
-0.0129158763729574));
#21342=CARTESIAN_POINT('Ctrl Pts',(-0.0111368266679554,-0.0311276971607501,
-0.0128988494615704));
#21343=CARTESIAN_POINT('Ctrl Pts',(-0.0111318133316558,-0.0311282567380392,
-0.0128893168349656));
#21344=CARTESIAN_POINT('Ctrl Pts',(-0.0111169256987649,-0.031129963151428,
-0.0128602746366784));
#21345=CARTESIAN_POINT('Ctrl Pts',(-0.0111073662144627,-0.0311311209257603,
-0.012840607512082));
#21346=CARTESIAN_POINT('Ctrl Pts',(-0.0110607219278723,-0.031137102606807,
-0.0127392188744835));
#21347=CARTESIAN_POINT('Ctrl Pts',(-0.0110304041011302,-0.0311421528906475,
-0.0126545872917843));
#21348=CARTESIAN_POINT('Ctrl Pts',(-0.0109903420781809,-0.0311511948352812,
-0.0125020507816218));
#21349=CARTESIAN_POINT('Ctrl Pts',(-0.0109774359771608,-0.0311551327015931,
-0.0124352195095036));
#21350=CARTESIAN_POINT('Ctrl Pts',(-0.0109651997208015,-0.0311606998811778,
-0.0123375965698176));
#21351=CARTESIAN_POINT('Ctrl Pts',(-0.0109623113754691,-0.031162399786375,
-0.0123073320358549));
#21352=CARTESIAN_POINT('Ctrl Pts',(-0.0109590484480718,-0.031165127141809,
-0.0122576632037539));
#21353=CARTESIAN_POINT('Ctrl Pts',(-0.0109581424565425,-0.0311661747410972,
-0.0122383027164186));
#21354=CARTESIAN_POINT('Ctrl Pts',(-0.0109573997453987,-0.0311675877622278,
-0.0122117089779379));
#21355=CARTESIAN_POINT('Ctrl Pts',(-0.010957248792155,-0.0311679688627185,
-0.0122044870225952));
#21356=CARTESIAN_POINT('Ctrl Pts',(-0.0109570796508526,-0.0311686072878051,
-0.0121922988135003));
#21357=CARTESIAN_POINT('Ctrl Pts',(-0.0109570347133661,-0.0311688660655803,
-0.0121873330838899));
#21358=CARTESIAN_POINT('Ctrl Pts',(-0.0109569916181838,-0.0311693952042206,
-0.0121771247251873));
#21359=CARTESIAN_POINT('Ctrl Pts',(-0.0109569962038278,-0.0311696654148973,
-0.0121718822021046));
#21360=CARTESIAN_POINT('Ctrl Pts',(-0.0109570784197879,-0.0311703712887587,
-0.0121581136928511));
#21361=CARTESIAN_POINT('Ctrl Pts',(-0.0109572000003191,-0.0311708045647993,
-0.0121495880395073));
#21362=CARTESIAN_POINT('Ctrl Pts',(-0.0109580187732477,-0.0311726349978654,
-0.0121132828204177));
#21363=CARTESIAN_POINT('Ctrl Pts',(-0.010959395680332,-0.0311739982119459,
-0.0120855223909404));
#21364=CARTESIAN_POINT('Ctrl Pts',(-0.0109686508018625,-0.0311798198603566,
-0.0119648959344783));
#21365=CARTESIAN_POINT('Ctrl Pts',(-0.0109841832778093,-0.0311840101716126,
-0.0118728094945433));
#21366=CARTESIAN_POINT('Ctrl Pts',(-0.0110314466607925,-0.0311925138532889,
-0.0116934467709577));
#21367=CARTESIAN_POINT('Ctrl Pts',(-0.0110629169821904,-0.0311968121845459,
-0.0116065072015876));
#21368=CARTESIAN_POINT('Ctrl Pts',(-0.0111090846695419,-0.0312022138392394,
-0.0115076565783938));
#21369=CARTESIAN_POINT('Ctrl Pts',(-0.0111164560409825,-0.0312030552750401,
-0.0114925243886525));
#21370=CARTESIAN_POINT('Ctrl Pts',(-0.0111284836261574,-0.0312043974756499,
-0.0114688265567624));
#21371=CARTESIAN_POINT('Ctrl Pts',(-0.0111329760998269,-0.0312048924871565,
-0.0114601790512941));
#21372=CARTESIAN_POINT('Ctrl Pts',(-0.011141574594219,-0.0312058285074883,
-0.011444004309123));
#21373=CARTESIAN_POINT('Ctrl Pts',(-0.0111456620439648,-0.0312062688419898,
-0.0114364675917224));
#21374=CARTESIAN_POINT('Ctrl Pts',(-0.0111550150009916,-0.0312072663301049,
-0.01141955976564));
#21375=CARTESIAN_POINT('Ctrl Pts',(-0.011160316010977,-0.0312078247494321,
-0.0114102088919434));
#21376=CARTESIAN_POINT('Ctrl Pts',(-0.0111766388626056,-0.0312095239808521,
-0.0113821042925125));
#21377=CARTESIAN_POINT('Ctrl Pts',(-0.0111879596588067,-0.0312106755962077,
-0.0113635280786875));
#21378=CARTESIAN_POINT('Ctrl Pts',(-0.0112528187808207,-0.0312171317976559,
-0.0112619957958249));
#21379=CARTESIAN_POINT('Ctrl Pts',(-0.0113138241330732,-0.0312227164045157,
-0.0111840981045602));
#21380=CARTESIAN_POINT('Ctrl Pts',(-0.0114316282162692,-0.0312325385762263,
-0.0110602141609473));
#21381=CARTESIAN_POINT('Ctrl Pts',(-0.0114850322445972,-0.0312367177322726,
-0.0110114177966349));
#21382=CARTESIAN_POINT('Ctrl Pts',(-0.0115593191796873,-0.0312420197606286,
-0.0109525478163445));
#21383=CARTESIAN_POINT('Ctrl Pts',(-0.0115772833932574,-0.0312432657176012,
-0.0109389414752818));
#21384=CARTESIAN_POINT('Ctrl Pts',(-0.0116081740004673,-0.0312453392971401,
-0.0109165921695208));
#21385=CARTESIAN_POINT('Ctrl Pts',(-0.0116209464427121,-0.0312461774619369,
-0.0109076431090239));
#21386=CARTESIAN_POINT('Ctrl Pts',(-0.0116393454923739,-0.0312473552021274,
-0.0108951632897102));
#21387=CARTESIAN_POINT('Ctrl Pts',(-0.0116448622419863,-0.031247704604537,
-0.010891473098485));
#21388=CARTESIAN_POINT('Ctrl Pts',(-0.0116544654328692,-0.0312483061370609,
-0.0108851387624942));
#21389=CARTESIAN_POINT('Ctrl Pts',(-0.0116585408457478,-0.0312485593448531,
-0.010882478174338));
#21390=CARTESIAN_POINT('Ctrl Pts',(-0.0116672333130352,-0.0312490949490242,
-0.0108768618717511));
#21391=CARTESIAN_POINT('Ctrl Pts',(-0.0116718535883144,-0.0312493770050019,
-0.0108739114394363));
#21392=CARTESIAN_POINT('Ctrl Pts',(-0.0116846238486616,-0.0312501496512385,
-0.010865852045191));
#21393=CARTESIAN_POINT('Ctrl Pts',(-0.0116928061608303,-0.0312506369741942,
-0.0108607944911011));
#21394=CARTESIAN_POINT('Ctrl Pts',(-0.0117357025130474,-0.0312531545595775,
-0.0108348311298225));
#21395=CARTESIAN_POINT('Ctrl Pts',(-0.0117711853453037,-0.031255111143097,
-0.0108152208042713));
#21396=CARTESIAN_POINT('Ctrl Pts',(-0.0118824743987821,-0.0312609925952532,
-0.0107593190983834));
#21397=CARTESIAN_POINT('Ctrl Pts',(-0.0119605045893482,-0.0312647732333334,
-0.0107278018578865));
#21398=CARTESIAN_POINT('Ctrl Pts',(-0.0121165116196277,-0.031272279977967,
-0.0106791605316225));
#21399=CARTESIAN_POINT('Ctrl Pts',(-0.0121940131859898,-0.0312759873359157,
-0.0106614151083494));
#21400=CARTESIAN_POINT('Ctrl Pts',(-0.0122933978351906,-0.0312809209924038,
-0.0106466019452003));
#21401=CARTESIAN_POINT('Ctrl Pts',(-0.0123143260863358,-0.031281969229822,
-0.0106439201080648));
#21402=CARTESIAN_POINT('Ctrl Pts',(-0.0123458631698375,-0.0312835654911346,
-0.0106405345384491));
#21403=CARTESIAN_POINT('Ctrl Pts',(-0.0123564354451908,-0.0312841034040758,
-0.0106395098900538));
#21404=CARTESIAN_POINT('Ctrl Pts',(-0.012375549059105,-0.031285081251584,
-0.0106378564402917));
#21405=CARTESIAN_POINT('Ctrl Pts',(-0.0123840867072331,-0.0312855199601821,
-0.0106371894374848));
#21406=CARTESIAN_POINT('Ctrl Pts',(-0.0124024385166975,-0.0312864672622507,
-0.010635909311979));
#21407=CARTESIAN_POINT('Ctrl Pts',(-0.0124122538382186,-0.0312869765519656,
-0.0106353188685943));
#21408=CARTESIAN_POINT('Ctrl Pts',(-0.0124388490866719,-0.0312883638656256,
-0.0106339740145444));
#21409=CARTESIAN_POINT('Ctrl Pts',(-0.0124556364473477,-0.0312892475002527,
-0.0106333997317607));
#21410=CARTESIAN_POINT('Ctrl Pts',(-0.0125704938159743,-0.0312953492017711,
-0.0106313471124719));
#21411=CARTESIAN_POINT('Ctrl Pts',(-0.012668487372212,-0.0313008553547883,
-0.0106389487559617));
#21412=CARTESIAN_POINT('Ctrl Pts',(-0.0128429466235424,-0.0313110090258485,
-0.0106693727204599));
#21413=CARTESIAN_POINT('Ctrl Pts',(-0.0129196526182226,-0.0313155950207616,
-0.0106889140619312));
#21414=CARTESIAN_POINT('Ctrl Pts',(-0.0130168898550949,-0.0313213476946538,
-0.0107218136260671));
#21415=CARTESIAN_POINT('Ctrl Pts',(-0.0130390792974556,-0.0313226555674681,
-0.0107298933754122));
#21416=CARTESIAN_POINT('Ctrl Pts',(-0.0130761133177147,-0.0313248201810509,
-0.0107443495181992));
#21417=CARTESIAN_POINT('Ctrl Pts',(-0.0130910587182855,-0.0313256886165501,
-0.0107504553682053));
#21418=CARTESIAN_POINT('Ctrl Pts',(-0.0131120939334941,-0.0313269007924542,
-0.0107594369331056));
#21419=CARTESIAN_POINT('Ctrl Pts',(-0.0131182645298868,-0.0313272551293908,
-0.0107621194912024));
#21420=CARTESIAN_POINT('Ctrl Pts',(-0.013128880205169,-0.0313278622994748,
-0.0107668172673062));
#21421=CARTESIAN_POINT('Ctrl Pts',(-0.0131333335911517,-0.0313281162683805,
-0.0107688133508342));
#21422=CARTESIAN_POINT('Ctrl Pts',(-0.0131427281013041,-0.0313286503610117,
-0.0107730777716749));
#21423=CARTESIAN_POINT('Ctrl Pts',(-0.0131476667777454,-0.0313289301780944,
-0.0107753511251391));
#21424=CARTESIAN_POINT('Ctrl Pts',(-0.0131611214909912,-0.0313296901569358,
-0.0107816309421281));
#21425=CARTESIAN_POINT('Ctrl Pts',(-0.0131696131809573,-0.031330167226973,
-0.0107856893509535));
#21426=CARTESIAN_POINT('Ctrl Pts',(-0.0132118066745237,-0.0313325273371271,
-0.0108063310933569));
#21427=CARTESIAN_POINT('Ctrl Pts',(-0.0132449344289738,-0.0313343472715819,
-0.0108240645205944));
#21428=CARTESIAN_POINT('Ctrl Pts',(-0.0133517755032359,-0.0313402109989266,
-0.0108863789230458));
#21429=CARTESIAN_POINT('Ctrl Pts',(-0.0134224073458359,-0.0313440852657322,
-0.0109359210994207));
#21430=CARTESIAN_POINT('Ctrl Pts',(-0.0135502929232256,-0.0313517326713571,
-0.0110426267863424));
#21431=CARTESIAN_POINT('Ctrl Pts',(-0.0136079193139404,-0.0313554846830447,
-0.0110988989378598));
#21432=CARTESIAN_POINT('Ctrl Pts',(-0.0136748757773923,-0.0313604741009463,
-0.0111753702043208));
#21433=CARTESIAN_POINT('Ctrl Pts',(-0.0136885261557252,-0.0313615284658871,
-0.0111916251562969));
#21434=CARTESIAN_POINT('Ctrl Pts',(-0.013708513501919,-0.0313631322157503,
-0.0112164485420964));
#21435=CARTESIAN_POINT('Ctrl Pts',(-0.0137151043714358,-0.0313636713432469,
-0.0112248098032431));
#21436=CARTESIAN_POINT('Ctrl Pts',(-0.0137267926811872,-0.031364646481713,
-0.0112399575957178));
#21437=CARTESIAN_POINT('Ctrl Pts',(-0.013731921686652,-0.0313650812109238,
-0.0112467192914424));
#21438=CARTESIAN_POINT('Ctrl Pts',(-0.0137428446459158,-0.0313660220366368,
-0.0112613687502036));
#21439=CARTESIAN_POINT('Ctrl Pts',(-0.0137486198364894,-0.031366528842055,
-0.0112692699869681));
#21440=CARTESIAN_POINT('Ctrl Pts',(-0.0137639816519964,-0.0313679027444263,
-0.0112907122608906));
#21441=CARTESIAN_POINT('Ctrl Pts',(-0.0137734255022911,-0.0313687752719427,
-0.0113043535946737));
#21442=CARTESIAN_POINT('Ctrl Pts',(-0.0138262623926238,-0.0313738218903273,
-0.0113833676767165));
#21443=CARTESIAN_POINT('Ctrl Pts',(-0.0138648334690308,-0.0313781741396072,
-0.0114518144486001));
#21444=CARTESIAN_POINT('Ctrl Pts',(-0.0139383546983522,-0.031388052756501,
-0.0116092272285832));
#21445=CARTESIAN_POINT('Ctrl Pts',(-0.0139705940672988,-0.031393613462857,
-0.011699112259949));
#21446=CARTESIAN_POINT('Ctrl Pts',(-0.0140007705764022,-0.0314004243894994,
-0.0118164043836479));
#21447=CARTESIAN_POINT('Ctrl Pts',(-0.0140065762251424,-0.0314018596450021,
-0.0118415719137731));
#21448=CARTESIAN_POINT('Ctrl Pts',(-0.014015199515888,-0.031404209607931,
-0.0118837632711088));
#21449=CARTESIAN_POINT('Ctrl Pts',(-0.0140183682408435,-0.0314051385426463,
-0.0119007095351413));
#21450=CARTESIAN_POINT('Ctrl Pts',(-0.0140224074768403,-0.031406419095244,
-0.011924512604793));
#21451=CARTESIAN_POINT('Ctrl Pts',(-0.0140235168407667,-0.0314067829250573,
-0.0119313270030986));
#21452=CARTESIAN_POINT('Ctrl Pts',(-0.0140253365821976,-0.03140740106837,
-0.011942998392169));
#21453=CARTESIAN_POINT('Ctrl Pts',(-0.0140260695839526,-0.0314076566295594,
-0.01194785171153));
#21454=CARTESIAN_POINT('Ctrl Pts',(-0.0140275544431892,-0.0314081884094914,
-0.0119580112748559));
#21455=CARTESIAN_POINT('Ctrl Pts',(-0.0140283018302413,-0.0314084643816878,
-0.0119633180274747));
#21456=CARTESIAN_POINT('Ctrl Pts',(-0.0140302378378962,-0.0314092026785807,
-0.0119776029958386));
#21457=CARTESIAN_POINT('Ctrl Pts',(-0.0140313751044238,-0.0314096622026436,
-0.0119865880879898));
#21458=CARTESIAN_POINT('Ctrl Pts',(-0.0140363282943189,-0.0314117950472679,
-0.0120286939042389));
#21459=CARTESIAN_POINT('Ctrl Pts',(-0.0140391494611381,-0.031413418910114,
-0.012061924657053));
#21460=CARTESIAN_POINT('Ctrl Pts',(-0.0140422975768346,-0.0314162923121628,
-0.0121220867706215));
#21461=CARTESIAN_POINT('Ctrl Pts',(-0.0140430000004932,-0.0314175525195978,
-0.0121489728247115));
#21462=CARTESIAN_POINT('Ctrl Pts',(-0.014043,-0.0314187998055481,-0.0121758533148708));
#21463=CARTESIAN_POINT('Origin',(-0.0125,-0.0375520664398416,-0.0121758532865581));
#21464=CARTESIAN_POINT('',(-0.014043,-0.0319166517728185,-0.012175853290423));
#21465=CARTESIAN_POINT('',(-0.014043,-0.0318006569328344,-0.0121758532865509));
#21466=CARTESIAN_POINT('',(-0.014043,-0.0375520664398416,-0.012175853286558));
#21467=CARTESIAN_POINT('Ctrl Pts',(-0.014043,-0.0318006569328344,-0.0121758532865438));
#21468=CARTESIAN_POINT('Ctrl Pts',(-0.014043,-0.031800630291104,-0.0121753151222929));
#21469=CARTESIAN_POINT('Ctrl Pts',(-0.0140429997179574,-0.0318006036615213,
-0.0121747769564973));
#21470=CARTESIAN_POINT('Ctrl Pts',(-0.0140429240554956,-0.0317970272351956,
-0.0121024653297101));
#21471=CARTESIAN_POINT('Ctrl Pts',(-0.0140378411364186,-0.0317936999177665,
-0.0120307775798329));
#21472=CARTESIAN_POINT('Ctrl Pts',(-0.014010173087722,-0.0317846413065578,
-0.0118352191775621));
#21473=CARTESIAN_POINT('Ctrl Pts',(-0.0139774172398278,-0.0317789769893868,
-0.0117133701000584));
#21474=CARTESIAN_POINT('Ctrl Pts',(-0.0139234868784111,-0.0317719059281056,
-0.0115801533805521));
#21475=CARTESIAN_POINT('Ctrl Pts',(-0.0139164380903339,-0.031771010882243,
-0.0115635817996873));
#21476=CARTESIAN_POINT('Ctrl Pts',(-0.0139046028958629,-0.0317695513497367,
-0.0115370563120314));
#21477=CARTESIAN_POINT('Ctrl Pts',(-0.013899996738649,-0.0317689930075452,
-0.0115270235760002));
#21478=CARTESIAN_POINT('Ctrl Pts',(-0.0138916235517631,-0.0317679945020514,
-0.0115092901880454));
#21479=CARTESIAN_POINT('Ctrl Pts',(-0.0138878992316142,-0.0317675558367389,
-0.0115015698201503));
#21480=CARTESIAN_POINT('Ctrl Pts',(-0.0138799117831603,-0.031766626197059,
-0.0114853587308294));
#21481=CARTESIAN_POINT('Ctrl Pts',(-0.0138756341846108,-0.0317661347267244,
-0.0114768755719674));
#21482=CARTESIAN_POINT('Ctrl Pts',(-0.0138640274006613,-0.0317648176722115,
-0.0114543767475489));
#21483=CARTESIAN_POINT('Ctrl Pts',(-0.0138565607304269,-0.0317639872469671,
-0.0114404336066681));
#21484=CARTESIAN_POINT('Ctrl Pts',(-0.0138159213544144,-0.0317595527490682,
-0.0113672697233371));
#21485=CARTESIAN_POINT('Ctrl Pts',(-0.0137790857770913,-0.0317558172180877,
-0.0113101777448214));
#21486=CARTESIAN_POINT('Ctrl Pts',(-0.0136808040824151,-0.0317465152106493,
-0.0111778809278317));
#21487=CARTESIAN_POINT('Ctrl Pts',(-0.0136157912680871,-0.0317408619446796,
-0.0111056871540145));
#21488=CARTESIAN_POINT('Ctrl Pts',(-0.0135094033908899,-0.0317326642940279,
-0.0110078553862304));
#21489=CARTESIAN_POINT('Ctrl Pts',(-0.013472894301811,-0.0317300099144168,
-0.0109772742436927));
#21490=CARTESIAN_POINT('Ctrl Pts',(-0.0134271763829065,-0.0317269277677483,
-0.0109424472890075));
#21491=CARTESIAN_POINT('Ctrl Pts',(-0.0134192682859518,-0.031726402955929,
-0.0109365420955482));
#21492=CARTESIAN_POINT('Ctrl Pts',(-0.0134068010642203,-0.0317255892474744,
-0.0109274174788518));
#21493=CARTESIAN_POINT('Ctrl Pts',(-0.0134022803366845,-0.0317252969600848,
-0.0109241463192546));
#21494=CARTESIAN_POINT('Ctrl Pts',(-0.0133942162168097,-0.0317247806297561,
-0.0109183775813838));
#21495=CARTESIAN_POINT('Ctrl Pts',(-0.0133906800132446,-0.0317245559367038,
-0.0109158703874805));
#21496=CARTESIAN_POINT('Ctrl Pts',(-0.0133821331609715,-0.0317240169503172,
-0.0109098645698703));
#21497=CARTESIAN_POINT('Ctrl Pts',(-0.0133771122493237,-0.0317237036638611,
-0.0109063807783821));
#21498=CARTESIAN_POINT('Ctrl Pts',(-0.01336154471605,-0.0317227421597699,
-0.0108957155984358));
#21499=CARTESIAN_POINT('Ctrl Pts',(-0.0133509293759966,-0.0317221003717403,
-0.0108886349619036));
#21500=CARTESIAN_POINT('Ctrl Pts',(-0.0132968948368375,-0.0317188964377486,
-0.0108535534804574));
#21501=CARTESIAN_POINT('Ctrl Pts',(-0.0132521733054764,-0.0317164468002304,
-0.0108276120894787));
#21502=CARTESIAN_POINT('Ctrl Pts',(-0.0131036592332028,-0.0317086819026316,
-0.0107511590444323));
#21503=CARTESIAN_POINT('Ctrl Pts',(-0.0129954912974291,-0.0317035537289001,
-0.0107100267541059));
#21504=CARTESIAN_POINT('Ctrl Pts',(-0.012841333060349,-0.0316959959845422,
-0.0106704436115146));
#21505=CARTESIAN_POINT('Ctrl Pts',(-0.0127984774933241,-0.0316938737939708,
-0.0106613641597208));
#21506=CARTESIAN_POINT('Ctrl Pts',(-0.0127411594453574,-0.0316909800703432,
-0.0106517481108439));
#21507=CARTESIAN_POINT('Ctrl Pts',(-0.0127269909217542,-0.0316902604120932,
-0.0106495736370227));
#21508=CARTESIAN_POINT('Ctrl Pts',(-0.0127037001825489,-0.0316890694806828,
-0.0106463306339442));
#21509=CARTESIAN_POINT('Ctrl Pts',(-0.0126945949243015,-0.0316886019217213,
-0.010645145567928));
#21510=CARTESIAN_POINT('Ctrl Pts',(-0.0126768648209758,-0.0316876874322071,
-0.010642998714074));
#21511=CARTESIAN_POINT('Ctrl Pts',(-0.0126682413588322,-0.0316872407946655,
-0.0106420282814334));
#21512=CARTESIAN_POINT('Ctrl Pts',(-0.0126479001148416,-0.0316861827262866,
-0.010639912803571));
#21513=CARTESIAN_POINT('Ctrl Pts',(-0.0126361766183313,-0.0316855693820485,
-0.0106388290416337));
#21514=CARTESIAN_POINT('Ctrl Pts',(-0.0125968527884696,-0.0316834998003213,
-0.0106356472322416));
#21515=CARTESIAN_POINT('Ctrl Pts',(-0.0125692097402094,-0.0316820246536008,
-0.0106341577813421));
#21516=CARTESIAN_POINT('Ctrl Pts',(-0.0124382744380537,-0.031674939488645,
-0.0106306312862919));
#21517=CARTESIAN_POINT('Ctrl Pts',(-0.0123350002987807,-0.031669038477402,
-0.0106382281837397));
#21518=CARTESIAN_POINT('Ctrl Pts',(-0.012151237794049,-0.0316583054104492,
-0.010670479162199));
#21519=CARTESIAN_POINT('Ctrl Pts',(-0.0120704952807793,-0.0316535128762213,
-0.0106914968401289));
#21520=CARTESIAN_POINT('Ctrl Pts',(-0.011978320373973,-0.0316482187122544,
-0.0107236465618568));
#21521=CARTESIAN_POINT('Ctrl Pts',(-0.0119648669779445,-0.031647450799211,
-0.0107285500422606));
#21522=CARTESIAN_POINT('Ctrl Pts',(-0.0119455658713085,-0.0316463580742347,
-0.0107358908292815));
#21523=CARTESIAN_POINT('Ctrl Pts',(-0.0119396622196268,-0.0316460250643994,
-0.010738177851672));
#21524=CARTESIAN_POINT('Ctrl Pts',(-0.0119292850441425,-0.0316454420928893,
-0.0107422715092035));
#21525=CARTESIAN_POINT('Ctrl Pts',(-0.0119248056701419,-0.0316451912436498,
-0.0107440628835124));
#21526=CARTESIAN_POINT('Ctrl Pts',(-0.0119151927200352,-0.0316446546751647,
-0.0107479596530128));
#21527=CARTESIAN_POINT('Ctrl Pts',(-0.0119100620423893,-0.0316443693588579,
-0.0107500717494829));
#21528=CARTESIAN_POINT('Ctrl Pts',(-0.0118957223472363,-0.0316435746227282,
-0.010756065489688));
#21529=CARTESIAN_POINT('Ctrl Pts',(-0.0118865393314773,-0.0316430688056284,
-0.0107600090550408));
#21530=CARTESIAN_POINT('Ctrl Pts',(-0.0118260182016705,-0.0316397518980771,
-0.0107866987026908));
#21531=CARTESIAN_POINT('Ctrl Pts',(-0.0117759115280193,-0.0316370850688512,
-0.010812145494282));
#21532=CARTESIAN_POINT('Ctrl Pts',(-0.0116275742199918,-0.0316291182848472,
-0.0108979658418662));
#21533=CARTESIAN_POINT('Ctrl Pts',(-0.0115346259594284,-0.031623996726177,
-0.0109666482075573));
#21534=CARTESIAN_POINT('Ctrl Pts',(-0.0114179772714879,-0.0316164399769792,
-0.0110749411839614));
#21535=CARTESIAN_POINT('Ctrl Pts',(-0.0113870617992448,-0.0316143103092429,
-0.0111062043809193));
#21536=CARTESIAN_POINT('Ctrl Pts',(-0.0113478781340771,-0.0316114078491724,
-0.0111493689143198));
#21537=CARTESIAN_POINT('Ctrl Pts',(-0.011338380987994,-0.0316106873466154,
-0.0111601288093045));
#21538=CARTESIAN_POINT('Ctrl Pts',(-0.0113230535894728,-0.0316094953790479,
-0.0111779903080915));
#21539=CARTESIAN_POINT('Ctrl Pts',(-0.0113171341261726,-0.0316090276412316,
-0.0111850144011765));
#21540=CARTESIAN_POINT('Ctrl Pts',(-0.0113057462058952,-0.0316081130660162,
-0.01119877491156));
#21541=CARTESIAN_POINT('Ctrl Pts',(-0.0113002711489813,-0.0316076665246123,
-0.0112055054337023));
#21542=CARTESIAN_POINT('Ctrl Pts',(-0.0112875075440424,-0.0316066091055477,
-0.0112214689773933));
#21543=CARTESIAN_POINT('Ctrl Pts',(-0.0112802673097772,-0.031605996321064,
-0.0112307397910558));
#21544=CARTESIAN_POINT('Ctrl Pts',(-0.0112563863377993,-0.0316039307063774,
-0.011262049874944));
#21545=CARTESIAN_POINT('Ctrl Pts',(-0.0112402320462533,-0.0316024590656478,
-0.0112844520379224));
#21546=CARTESIAN_POINT('Ctrl Pts',(-0.0111665650985857,-0.031595380844297,
-0.0113926153348836));
#21547=CARTESIAN_POINT('Ctrl Pts',(-0.0111171619164245,-0.0315894833894227,
-0.0114835643690004));
#21548=CARTESIAN_POINT('Ctrl Pts',(-0.0110675418461785,-0.0315821068386753,
-0.0116017997303886));
#21549=CARTESIAN_POINT('Ctrl Pts',(-0.0110584301087489,-0.031580668887265,
-0.0116250809976767));
#21550=CARTESIAN_POINT('Ctrl Pts',(-0.0110278663839119,-0.0315755474997315,
-0.0117091366087032));
#21551=CARTESIAN_POINT('Ctrl Pts',(-0.011009658438675,-0.0315719038614914,
-0.0117710257013392));
#21552=CARTESIAN_POINT('Ctrl Pts',(-0.0109930773146484,-0.0315678858214653,
-0.0118439792902322));
#21553=CARTESIAN_POINT('Ctrl Pts',(-0.010990882965122,-0.0315673342759804,
-0.0118541047582145));
#21554=CARTESIAN_POINT('Ctrl Pts',(-0.0109876416896197,-0.0315664883202947,
-0.0118698243430674));
#21555=CARTESIAN_POINT('Ctrl Pts',(-0.0109865234855263,-0.0315661900910179,
-0.0118754032650795));
#21556=CARTESIAN_POINT('Ctrl Pts',(-0.010984518280851,-0.0315656433627924,
-0.0118857029309605));
#21557=CARTESIAN_POINT('Ctrl Pts',(-0.010983622453974,-0.0315653943879511,
-0.0118904216685973));
#21558=CARTESIAN_POINT('Ctrl Pts',(-0.0109816158611639,-0.0315648255243191,
-0.0119012674562572));
#21559=CARTESIAN_POINT('Ctrl Pts',(-0.010980520136464,-0.0315645064845513,
-0.0119073971110363));
#21560=CARTESIAN_POINT('Ctrl Pts',(-0.0109771883120504,-0.0315635085460924,
-0.0119267100421606));
#21561=CARTESIAN_POINT('Ctrl Pts',(-0.0109750863987945,-0.0315628368008368,
-0.0119399161660624));
#21562=CARTESIAN_POINT('Ctrl Pts',(-0.0109649245214153,-0.0315593411971617,
-0.0120095850233701));
#21563=CARTESIAN_POINT('Ctrl Pts',(-0.0109598274102922,-0.0315566538427666,
-0.0120664396776707));
#21564=CARTESIAN_POINT('Ctrl Pts',(-0.0109545142260599,-0.0315494153022565,
-0.0122227950051354));
#21565=CARTESIAN_POINT('Ctrl Pts',(-0.0109607458248166,-0.0315449654078458,
-0.0123222318213382));
#21566=CARTESIAN_POINT('Ctrl Pts',(-0.010984675190863,-0.0315378572209813,
-0.0124713219394031));
#21567=CARTESIAN_POINT('Ctrl Pts',(-0.0109954009256225,-0.0315353746771646,
-0.0125218185770298));
#21568=CARTESIAN_POINT('Ctrl Pts',(-0.0110125450983386,-0.0315320542911416,
-0.0125864129636788));
#21569=CARTESIAN_POINT('Ctrl Pts',(-0.0110166732559227,-0.0315312902798499,
-0.0126010862606229));
#21570=CARTESIAN_POINT('Ctrl Pts',(-0.0110236909792046,-0.0315300448295888,
-0.0126246835458702));
#21571=CARTESIAN_POINT('Ctrl Pts',(-0.011026445765568,-0.031529567811064,
-0.0126336467330491));
#21572=CARTESIAN_POINT('Ctrl Pts',(-0.0110318845674109,-0.031528647916297,
-0.0126507849696059));
#21573=CARTESIAN_POINT('Ctrl Pts',(-0.0110345556072107,-0.0315282054829589,
-0.0126589637859304));
#21574=CARTESIAN_POINT('Ctrl Pts',(-0.0110408889312757,-0.0315271772916329,
-0.0126778207336216));
#21575=CARTESIAN_POINT('Ctrl Pts',(-0.0110446002438786,-0.0315265899214682,
-0.0126884817772992));
#21576=CARTESIAN_POINT('Ctrl Pts',(-0.0110568474233639,-0.0315246981823385,
-0.0127224573921279));
#21577=CARTESIAN_POINT('Ctrl Pts',(-0.0110658288473158,-0.0315233790617733,
-0.0127456062293459));
#21578=CARTESIAN_POINT('Ctrl Pts',(-0.0111179710884246,-0.0315160679038513,
-0.0128709426998285));
#21579=CARTESIAN_POINT('Ctrl Pts',(-0.0111714917336044,-0.0315097234847948,
-0.0129684517790176));
#21580=CARTESIAN_POINT('Ctrl Pts',(-0.0112806622102527,-0.0314987561664895,
-0.013124761480192));
#21581=CARTESIAN_POINT('Ctrl Pts',(-0.0113313406802289,-0.0314941765764891,
-0.0131865207481635));
#21582=CARTESIAN_POINT('Ctrl Pts',(-0.0113965066813918,-0.0314890714234106,
-0.0132544437859607));
#21583=CARTESIAN_POINT('Ctrl Pts',(-0.0114065868246255,-0.03148830165795,
-0.0132646611789313));
#21584=CARTESIAN_POINT('Ctrl Pts',(-0.0114213213747563,-0.0314872068035573,
-0.0132791853217146));
#21585=CARTESIAN_POINT('Ctrl Pts',(-0.0114258617893619,-0.0314868734739981,
-0.013283606085507));
#21586=CARTESIAN_POINT('Ctrl Pts',(-0.0114339070495687,-0.0314862901444335,
-0.0132913433587082));
#21587=CARTESIAN_POINT('Ctrl Pts',(-0.0114374004072367,-0.0314860392531805,
-0.0132946715862134));
#21588=CARTESIAN_POINT('Ctrl Pts',(-0.0114449417030782,-0.0314855028281203,
-0.0133017892228587));
#21589=CARTESIAN_POINT('Ctrl Pts',(-0.0114489944971222,-0.0314852176946538,
-0.013305573241834));
#21590=CARTESIAN_POINT('Ctrl Pts',(-0.0114603962918709,-0.0314844239995374,
-0.0133161044249919));
#21591=CARTESIAN_POINT('Ctrl Pts',(-0.011467790581762,-0.0314839190254278,
-0.0133228023941833));
#21592=CARTESIAN_POINT('Ctrl Pts',(-0.0115168794162522,-0.0314806262338454,
-0.0133664092732175));
#21593=CARTESIAN_POINT('Ctrl Pts',(-0.0115604846098879,-0.031477980269098,
-0.0134011130887091));
#21594=CARTESIAN_POINT('Ctrl Pts',(-0.0116985704139045,-0.0314701005952718,
-0.0134992943016249));
#21595=CARTESIAN_POINT('Ctrl Pts',(-0.0117982678455839,-0.0314650432427232,
-0.0135547508225012));
#21596=CARTESIAN_POINT('Ctrl Pts',(-0.0119451645025708,-0.0314574943013234,
-0.0136163676654415));
#21597=CARTESIAN_POINT('Ctrl Pts',(-0.0119879288441348,-0.0314552901873211,
-0.0136321179503589));
#21598=CARTESIAN_POINT('Ctrl Pts',(-0.0120451693595663,-0.0314523002917368,
-0.0136503665053269));
#21599=CARTESIAN_POINT('Ctrl Pts',(-0.0120590749664324,-0.0314515710219752,
-0.0136545842425752));
#21600=CARTESIAN_POINT('Ctrl Pts',(-0.0120819016179637,-0.0314503682950758,
-0.0136611572370011));
#21601=CARTESIAN_POINT('Ctrl Pts',(-0.0120907880374488,-0.0314498987012237,
-0.0136636300329526));
#21602=CARTESIAN_POINT('Ctrl Pts',(-0.0121080585018323,-0.0314489832053343,
-0.0136682693948805));
#21603=CARTESIAN_POINT('Ctrl Pts',(-0.0121164396775446,-0.0314485376299861,
-0.013670445355758));
#21604=CARTESIAN_POINT('Ctrl Pts',(-0.0121361459330668,-0.0314474867756949,
-0.0136753849156557));
#21605=CARTESIAN_POINT('Ctrl Pts',(-0.0121474847910617,-0.0314468796561892,
-0.0136780909195834));
#21606=CARTESIAN_POINT('Ctrl Pts',(-0.0121851607319519,-0.0314448538103778,
-0.0136866321919951));
#21607=CARTESIAN_POINT('Ctrl Pts',(-0.0122116190984518,-0.0314434172474533,
-0.0136919050659516));
#21608=CARTESIAN_POINT('Ctrl Pts',(-0.0122757551059123,-0.0314399006285472,
-0.0137029470427694));
#21609=CARTESIAN_POINT('Ctrl Pts',(-0.0123135335768134,-0.0314378006839648,
-0.0137080187715643));
#21610=CARTESIAN_POINT('Ctrl Pts',(-0.012457617621782,-0.0314296992537254,
-0.0137219541182271));
#21611=CARTESIAN_POINT('Ctrl Pts',(-0.0125645521885388,-0.0314234725606537,
-0.0137211863448015));
#21612=CARTESIAN_POINT('Ctrl Pts',(-0.0127197598683049,-0.0314146025089491,
-0.0137039263207496));
#21613=CARTESIAN_POINT('Ctrl Pts',(-0.0127686924796418,-0.0314118358566056,
-0.0136960857583644));
#21614=CARTESIAN_POINT('Ctrl Pts',(-0.0128269234237763,-0.031408643907022,
-0.0136838550991895));
#21615=CARTESIAN_POINT('Ctrl Pts',(-0.0128366602484997,-0.0314081136287711,
-0.0136817112742818));
#21616=CARTESIAN_POINT('Ctrl Pts',(-0.0128518354416466,-0.0314072933158411,
-0.0136782154968239));
#21617=CARTESIAN_POINT('Ctrl Pts',(-0.0128572882227633,-0.0314069998045459,
-0.0136769280737221));
#21618=CARTESIAN_POINT('Ctrl Pts',(-0.012866944239757,-0.0314064824055297,
-0.0136745926529453));
#21619=CARTESIAN_POINT('Ctrl Pts',(-0.0128711501188199,-0.0314062578524647,
-0.0136735566461199));
#21620=CARTESIAN_POINT('Ctrl Pts',(-0.0128812487181822,-0.0314057205870529,
-0.0136710239713124));
#21621=CARTESIAN_POINT('Ctrl Pts',(-0.0128871370070363,-0.0314054088625491,
-0.0136695101754966));
#21622=CARTESIAN_POINT('Ctrl Pts',(-0.0129051965450461,-0.0314044571203294,
-0.0136647533541457));
#21623=CARTESIAN_POINT('Ctrl Pts',(-0.0129173374299002,-0.0314038233447224,
-0.0136613959955447));
#21624=CARTESIAN_POINT('Ctrl Pts',(-0.0129457587835721,-0.0314023510811008,
-0.013653160601575));
#21625=CARTESIAN_POINT('Ctrl Pts',(-0.0129620026687948,-0.0314015184722565,
-0.0136481614638394));
#21626=CARTESIAN_POINT('Ctrl Pts',(-0.0130206555641337,-0.0313985335677542,
-0.0136290443927013));
#21627=CARTESIAN_POINT('Ctrl Pts',(-0.0130625305068071,-0.0313964432331087,
-0.0136133533619526));
#21628=CARTESIAN_POINT('Ctrl Pts',(-0.0131982379464647,-0.0313896356981413,
-0.013555662234645));
#21629=CARTESIAN_POINT('Ctrl Pts',(-0.0132885534290213,-0.0313850331117796,
-0.0135061135931963));
#21630=CARTESIAN_POINT('Ctrl Pts',(-0.0134112576859686,-0.0313779840296989,
-0.0134218794208967));
#21631=CARTESIAN_POINT('Ctrl Pts',(-0.013448052116485,-0.0313757558167005,
-0.0133941177908969));
#21632=CARTESIAN_POINT('Ctrl Pts',(-0.0134947858151831,-0.0313727377552565,
-0.0133554561483445));
#21633=CARTESIAN_POINT('Ctrl Pts',(-0.0135058912837954,-0.0313720058249217,
-0.0133460004723073));
#21634=CARTESIAN_POINT('Ctrl Pts',(-0.013523807265752,-0.0313707998273471,
-0.0133303024977436));
#21635=CARTESIAN_POINT('Ctrl Pts',(-0.013530698836923,-0.0313703296649524,
-0.0133241538575348));
#21636=CARTESIAN_POINT('Ctrl Pts',(-0.0135439403209284,-0.0313694138634025,
-0.0133121246016416));
#21637=CARTESIAN_POINT('Ctrl Pts',(-0.0135502967841283,-0.0313689685601055,
-0.0133062516925681));
#21638=CARTESIAN_POINT('Ctrl Pts',(-0.0135650762338339,-0.0313679196056958,
-0.0132923642757343));
#21639=CARTESIAN_POINT('Ctrl Pts',(-0.013573458629085,-0.0313673141332777,
-0.0132843074960202));
#21640=CARTESIAN_POINT('Ctrl Pts',(-0.013600853366855,-0.0313652997611933,
-0.0132573747199841));
#21641=CARTESIAN_POINT('Ctrl Pts',(-0.0136194644230901,-0.0313638733011536,
-0.0132380990352257));
#21642=CARTESIAN_POINT('Ctrl Pts',(-0.0136630699305331,-0.0313603867760978,
-0.0131905170504403));
#21643=CARTESIAN_POINT('Ctrl Pts',(-0.0136875447775516,-0.031358307270234,
-0.0131617596279088));
#21644=CARTESIAN_POINT('Ctrl Pts',(-0.0138019066580386,-0.0313479849574463,
-0.0130169432312744));
#21645=CARTESIAN_POINT('Ctrl Pts',(-0.0138759629044949,-0.0313392533197594,
-0.0128893755103561));
#21646=CARTESIAN_POINT('Ctrl Pts',(-0.0139370121809736,-0.0313303600388513,
-0.0127380926822364));
#21647=CARTESIAN_POINT('Ctrl Pts',(-0.0139428982562188,-0.0313294780530571,
-0.0127228101499231));
#21648=CARTESIAN_POINT('Ctrl Pts',(-0.0139509387763527,-0.031328239789845,
-0.0127009000863227));
#21649=CARTESIAN_POINT('Ctrl Pts',(-0.0139532931812631,-0.031327872779829,
-0.0126943476525835));
#21650=CARTESIAN_POINT('Ctrl Pts',(-0.0139572136048589,-0.0313272542821306,
-0.0126832003773575));
#21651=CARTESIAN_POINT('Ctrl Pts',(-0.0139588024282121,-0.0313270014754814,
-0.0126786137051423));
#21652=CARTESIAN_POINT('Ctrl Pts',(-0.0139620753876551,-0.0313264762451874,
-0.012669019054479));
#21653=CARTESIAN_POINT('Ctrl Pts',(-0.0139637554792521,-0.0313262040545563,
-0.012664009831563));
#21654=CARTESIAN_POINT('Ctrl Pts',(-0.0139681582703751,-0.0313254835558807,
-0.0126506557095259));
#21655=CARTESIAN_POINT('Ctrl Pts',(-0.0139708355850721,-0.0313250378356614,
-0.0126422959264484));
#21656=CARTESIAN_POINT('Ctrl Pts',(-0.0139835680918285,-0.0313228780206909,
-0.0126013393005177));
#21657=CARTESIAN_POINT('Ctrl Pts',(-0.0139926123972976,-0.0313212164221712,
-0.0125684359760995));
#21658=CARTESIAN_POINT('Ctrl Pts',(-0.0140179558701629,-0.0313160286083413,
-0.0124626238067398));
#21659=CARTESIAN_POINT('Ctrl Pts',(-0.0140300569968736,-0.0313126382639009,
-0.0123888184736796));
#21660=CARTESIAN_POINT('Ctrl Pts',(-0.0140409219831004,-0.0313071059622067,
-0.0122683242487341));
#21661=CARTESIAN_POINT('Ctrl Pts',(-0.014043,-0.0313049845530144,-0.0122220872743005));
#21662=CARTESIAN_POINT('Ctrl Pts',(-0.014043,-0.0313028240247934,-0.012175853286558));
#21663=CARTESIAN_POINT('Ctrl Pts',(-0.014043,-0.0314187998055481,-0.0121758533148708));
#21664=CARTESIAN_POINT('Ctrl Pts',(-0.0140429999988588,-0.0314216855929924,
-0.0122380454537156));
#21665=CARTESIAN_POINT('Ctrl Pts',(-0.0140392399449419,-0.0314245042001014,
-0.0123002077166543));
#21666=CARTESIAN_POINT('Ctrl Pts',(-0.0140208889864976,-0.0314314837974405,
-0.0124512110731899));
#21667=CARTESIAN_POINT('Ctrl Pts',(-0.014002275293269,-0.0314356780248151,
-0.012539297740629));
#21668=CARTESIAN_POINT('Ctrl Pts',(-0.0139712207534049,-0.0314409577605894,
-0.012641298972176));
#21669=CARTESIAN_POINT('Ctrl Pts',(-0.0139660757433579,-0.031441796146914,
-0.0126572596414093));
#21670=CARTESIAN_POINT('Ctrl Pts',(-0.0139575355393169,-0.0314431345853968,
-0.012682344994258));
#21671=CARTESIAN_POINT('Ctrl Pts',(-0.0139543122951916,-0.031443628940107,
-0.0126915270601004));
#21672=CARTESIAN_POINT('Ctrl Pts',(-0.0139480856770548,-0.0314445644024562,
-0.012708742027167));
#21673=CARTESIAN_POINT('Ctrl Pts',(-0.0139451017595287,-0.0314450048446786,
-0.0127167815984485));
#21674=CARTESIAN_POINT('Ctrl Pts',(-0.0139382198245729,-0.031446003506652,
-0.0127348601796778));
#21675=CARTESIAN_POINT('Ctrl Pts',(-0.0139342834387855,-0.0314465630044302,
-0.0127448840235487));
#21676=CARTESIAN_POINT('Ctrl Pts',(-0.0139220405319888,-0.0314482688950765,
-0.0127751257354399));
#21677=CARTESIAN_POINT('Ctrl Pts',(-0.0139134092916564,-0.0314494262159711,
-0.0127952084759897));
#21678=CARTESIAN_POINT('Ctrl Pts',(-0.0138656667541817,-0.0314556027049977,
-0.0129000935037362));
#21679=CARTESIAN_POINT('Ctrl Pts',(-0.0138193481733023,-0.0314608691567798,
-0.0129813877187382));
#21680=CARTESIAN_POINT('Ctrl Pts',(-0.013706683963106,-0.0314721789603007,
-0.0131430750946339));
#21681=CARTESIAN_POINT('Ctrl Pts',(-0.0136389643303889,-0.0314782151913641,
-0.0132219731957544));
#21682=CARTESIAN_POINT('Ctrl Pts',(-0.0135543627053837,-0.0314845312773765,
-0.0133025029334424));
#21683=CARTESIAN_POINT('Ctrl Pts',(-0.0135447724057623,-0.0314852313616164,
-0.0133114019573471));
#21684=CARTESIAN_POINT('Ctrl Pts',(-0.0135304805762694,-0.0314862499360126,
-0.0133243292653996));
#21685=CARTESIAN_POINT('Ctrl Pts',(-0.013525866360791,-0.0314865750786379,
-0.0133284527418921));
#21686=CARTESIAN_POINT('Ctrl Pts',(-0.0135179594372508,-0.031487125754598,
-0.0133354336365533));
#21687=CARTESIAN_POINT('Ctrl Pts',(-0.0135146792651424,-0.0314873523150126,
-0.0133383050035641));
#21688=CARTESIAN_POINT('Ctrl Pts',(-0.01350717894198,-0.0314878660443637,
-0.0133448146302843));
#21689=CARTESIAN_POINT('Ctrl Pts',(-0.0135029512197482,-0.0314881525584564,
-0.0133484439640745));
#21690=CARTESIAN_POINT('Ctrl Pts',(-0.0134912567842693,-0.0314889369990052,
-0.0133583736587378));
#21691=CARTESIAN_POINT('Ctrl Pts',(-0.013483749633373,-0.0314894315678469,
-0.0133646262300369));
#21692=CARTESIAN_POINT('Ctrl Pts',(-0.0134410412539979,-0.0314921980381885,
-0.0133995156181787));
#21693=CARTESIAN_POINT('Ctrl Pts',(-0.0134046468821151,-0.031494377009065,
-0.0134266621483671));
#21694=CARTESIAN_POINT('Ctrl Pts',(-0.0132853666425809,-0.0315011482257995,
-0.0135076991616854));
#21695=CARTESIAN_POINT('Ctrl Pts',(-0.0131984798373307,-0.0315055587226969,
-0.0135552522752469));
#21696=CARTESIAN_POINT('Ctrl Pts',(-0.0130448705970116,-0.0315133184102152,
-0.0136210619488648));
#21697=CARTESIAN_POINT('Ctrl Pts',(-0.0129803920588518,-0.0315165622782346,
-0.013643754580357));
#21698=CARTESIAN_POINT('Ctrl Pts',(-0.0128993289897697,-0.0315207376173863,
-0.0136663691636852));
#21699=CARTESIAN_POINT('Ctrl Pts',(-0.012883967019409,-0.0315215327998017,
-0.0136704002166832));
#21700=CARTESIAN_POINT('Ctrl Pts',(-0.0128592813512121,-0.0315228179743021,
-0.0136764721374574));
#21701=CARTESIAN_POINT('Ctrl Pts',(-0.0128499959959254,-0.0315233030360891,
-0.0136786649256138));
#21702=CARTESIAN_POINT('Ctrl Pts',(-0.0128322943177223,-0.0315242311219549,
-0.013682672321702));
#21703=CARTESIAN_POINT('Ctrl Pts',(-0.0128238819549973,-0.0315246736108308,
-0.0136845028792327));
#21704=CARTESIAN_POINT('Ctrl Pts',(-0.0128045985912559,-0.0315256913505688,
-0.0136885302834647));
#21705=CARTESIAN_POINT('Ctrl Pts',(-0.0127937184265435,-0.0315262680758019,
-0.0136906804965072));
#21706=CARTESIAN_POINT('Ctrl Pts',(-0.01276502335477,-0.0315277959497924,
-0.0136960306488351));
#21707=CARTESIAN_POINT('Ctrl Pts',(-0.0127471740453338,-0.0315287532568627,
-0.0136990346759671));
#21708=CARTESIAN_POINT('Ctrl Pts',(-0.0126055737809395,-0.0315364040525736,
-0.0137203114565959));
#21709=CARTESIAN_POINT('Ctrl Pts',(-0.0124800872303128,-0.0315435797212047,
-0.013723784297865));
#21710=CARTESIAN_POINT('Ctrl Pts',(-0.0122769806300937,-0.0315553065791207,
-0.0137046909230675));
#21711=CARTESIAN_POINT('Ctrl Pts',(-0.0121990524657633,-0.0315598178928486,
-0.0136912789580564));
#21712=CARTESIAN_POINT('Ctrl Pts',(-0.0121122597943697,-0.0315646262399087,
-0.013669378581585));
#21713=CARTESIAN_POINT('Ctrl Pts',(-0.0121020581902953,-0.0315651878494193,
-0.0136666928493729));
#21714=CARTESIAN_POINT('Ctrl Pts',(-0.0120864060407903,-0.0315660431511267,
-0.0136624000601014));
#21715=CARTESIAN_POINT('Ctrl Pts',(-0.0120809356730253,-0.0315663408723307,
-0.0136608672140737));
#21716=CARTESIAN_POINT('Ctrl Pts',(-0.0120708318770773,-0.0315668883691417,
-0.0136579757627627));
#21717=CARTESIAN_POINT('Ctrl Pts',(-0.0120661963298796,-0.0315671386014761,
-0.0136566256149808));
#21718=CARTESIAN_POINT('Ctrl Pts',(-0.0120556232049555,-0.0315677072362739,
-0.0136534921787438));
#21719=CARTESIAN_POINT('Ctrl Pts',(-0.0120496899720474,-0.0315680248214863,
-0.0136516948474849));
#21720=CARTESIAN_POINT('Ctrl Pts',(-0.0120308744763391,-0.0315690276065104,
-0.013645871110256));
#21721=CARTESIAN_POINT('Ctrl Pts',(-0.0120180338164882,-0.0315697054688908,
-0.0136417113220724));
#21722=CARTESIAN_POINT('Ctrl Pts',(-0.011909283972561,-0.0315754038128945,
-0.0136048977846261));
#21723=CARTESIAN_POINT('Ctrl Pts',(-0.0118167405790377,-0.0315799811809506,
-0.0135630356141383));
#21724=CARTESIAN_POINT('Ctrl Pts',(-0.0116507180950171,-0.0315887461816521,
-0.0134672590627352));
#21725=CARTESIAN_POINT('Ctrl Pts',(-0.0115765930058636,-0.031592907270975,
-0.0134153396254213));
#21726=CARTESIAN_POINT('Ctrl Pts',(-0.0114882928262972,-0.0315985317671662,
-0.0133411528032266));
#21727=CARTESIAN_POINT('Ctrl Pts',(-0.0114695407594927,-0.0315997681887071,
-0.0133246039272904));
#21728=CARTESIAN_POINT('Ctrl Pts',(-0.0114428755826538,-0.0316015932368798,
-0.013299893216345));
#21729=CARTESIAN_POINT('Ctrl Pts',(-0.0114346369432065,-0.0316021667873117,
-0.0132920877358709));
#21730=CARTESIAN_POINT('Ctrl Pts',(-0.0114202772051401,-0.0316031840721613,
-0.0132781791835554));
#21731=CARTESIAN_POINT('Ctrl Pts',(-0.011414119831395,-0.0316036261341294,
-0.0132721141826644));
#21732=CARTESIAN_POINT('Ctrl Pts',(-0.0114013635139283,-0.0316045544583557,
-0.013259336315536));
#21733=CARTESIAN_POINT('Ctrl Pts',(-0.0113947744096335,-0.0316050411283271,
-0.0132526141661086));
#21734=CARTESIAN_POINT('Ctrl Pts',(-0.0113776456897686,-0.0316063254153682,
-0.0132348167131437));
#21735=CARTESIAN_POINT('Ctrl Pts',(-0.0113672086351464,-0.0316071274270104,
-0.013223644505026));
#21736=CARTESIAN_POINT('Ctrl Pts',(-0.0113222320731733,-0.0316106710319972,
-0.0131740423693049));
#21737=CARTESIAN_POINT('Ctrl Pts',(-0.011289472193382,-0.0316134855826697,
-0.0131340496840499));
#21738=CARTESIAN_POINT('Ctrl Pts',(-0.0112006689691173,-0.0316218155595446,
-0.0130138015137302));
#21739=CARTESIAN_POINT('Ctrl Pts',(-0.0111501738805981,-0.0316274929481046,
-0.0129297664808525));
#21740=CARTESIAN_POINT('Ctrl Pts',(-0.0110828562279666,-0.031636423064715,
-0.0127889953812587));
#21741=CARTESIAN_POINT('Ctrl Pts',(-0.0110607267242149,-0.0316397154109402,
-0.0127350788423439));
#21742=CARTESIAN_POINT('Ctrl Pts',(-0.0110372773487158,-0.0316436002356902,
-0.0126672537134824));
#21743=CARTESIAN_POINT('Ctrl Pts',(-0.011033025996539,-0.0316443246282052,
-0.0126544128249562));
#21744=CARTESIAN_POINT('Ctrl Pts',(-0.011027051346591,-0.0316453714782436,
-0.0126355386036348));
#21745=CARTESIAN_POINT('Ctrl Pts',(-0.0110251952250376,-0.0316457011070212,
-0.0126295483435721));
#21746=CARTESIAN_POINT('Ctrl Pts',(-0.0110219755849809,-0.0316462806238918,
-0.012618929028264));
#21747=CARTESIAN_POINT('Ctrl Pts',(-0.0110205971952142,-0.0316465313568009,
-0.0126143046833669));
#21748=CARTESIAN_POINT('Ctrl Pts',(-0.011017636666745,-0.031647075684922,
-0.0126041995107628));
#21749=CARTESIAN_POINT('Ctrl Pts',(-0.0110160632115682,-0.0316473687820653,
-0.0125987163253028));
#21750=CARTESIAN_POINT('Ctrl Pts',(-0.0110117176444677,-0.0316481894854295,
-0.0125832498706483));
#21751=CARTESIAN_POINT('Ctrl Pts',(-0.0110090155767339,-0.0316487132087248,
-0.0125732470549029));
#21752=CARTESIAN_POINT('Ctrl Pts',(-0.0109906081618817,-0.0316523842815274,
-0.0125022723833809));
#21753=CARTESIAN_POINT('Ctrl Pts',(-0.0109785454291245,-0.0316553510898768,
-0.0124404107412925));
#21754=CARTESIAN_POINT('Ctrl Pts',(-0.0109614573369846,-0.0316613814771096,
-0.0123110872576325));
#21755=CARTESIAN_POINT('Ctrl Pts',(-0.0109570156799674,-0.0316644317685996,
-0.0122436865241268));
#21756=CARTESIAN_POINT('Ctrl Pts',(-0.0109569816722006,-0.0316711948049043,
-0.0120969527910919));
#21757=CARTESIAN_POINT('Ctrl Pts',(-0.010963070016228,-0.0316749233671426,
-0.0120178175974637));
#21758=CARTESIAN_POINT('Ctrl Pts',(-0.0109777527841392,-0.0316796695635056,
-0.0119230919205409));
#21759=CARTESIAN_POINT('Ctrl Pts',(-0.0109805618209704,-0.0316804998709306,
-0.0119067204429781));
#21760=CARTESIAN_POINT('Ctrl Pts',(-0.0109854459026682,-0.0316818329524735,
-0.0118807757495471));
#21761=CARTESIAN_POINT('Ctrl Pts',(-0.0109873487846232,-0.0316823302282132,
-0.0118711712204072));
#21762=CARTESIAN_POINT('Ctrl Pts',(-0.0109910713672093,-0.0316832640090688,
-0.0118532770942604));
#21763=CARTESIAN_POINT('Ctrl Pts',(-0.0109928683066127,-0.031683699766836,
-0.0118449831101408));
#21764=CARTESIAN_POINT('Ctrl Pts',(-0.0109970722828062,-0.0316846868900492,
-0.0118263243261713));
#21765=CARTESIAN_POINT('Ctrl Pts',(-0.0109995182829033,-0.0316852394964143,
-0.0118159688241762));
#21766=CARTESIAN_POINT('Ctrl Pts',(-0.0110071560672459,-0.031686903189005,
-0.011785065433712));
#21767=CARTESIAN_POINT('Ctrl Pts',(-0.0110126641422153,-0.0316880244259015,
-0.0117645989379319));
#21768=CARTESIAN_POINT('Ctrl Pts',(-0.0110410173594783,-0.0316934510274061,
-0.0116672804403995));
#21769=CARTESIAN_POINT('Ctrl Pts',(-0.0110694050539009,-0.0316979340238511,
-0.0115921821460593));
#21770=CARTESIAN_POINT('Ctrl Pts',(-0.0111399017405879,-0.0317074009861696,
-0.0114421569168597));
#21771=CARTESIAN_POINT('Ctrl Pts',(-0.01118269381291,-0.0317123820749236,
-0.0113678420665893));
#21772=CARTESIAN_POINT('Ctrl Pts',(-0.0112532272501905,-0.0317193527880609,
-0.0112659780185449));
#21773=CARTESIAN_POINT('Ctrl Pts',(-0.0112761921383354,-0.0317214701386228,
-0.0112353161852541));
#21774=CARTESIAN_POINT('Ctrl Pts',(-0.0113062256179998,-0.0317240272589316,
-0.0111981819475763));
#21775=CARTESIAN_POINT('Ctrl Pts',(-0.011312243238261,-0.0317245297064263,
-0.0111908799844202));
#21776=CARTESIAN_POINT('Ctrl Pts',(-0.0113218308849708,-0.0317253141558594,
-0.0111794616901454));
#21777=CARTESIAN_POINT('Ctrl Pts',(-0.0113253561033934,-0.0317255992391111,
-0.0111753082376082));
#21778=CARTESIAN_POINT('Ctrl Pts',(-0.01133207872757,-0.0317261364439579,
-0.0111674720663748));
#21779=CARTESIAN_POINT('Ctrl Pts',(-0.0113352716623891,-0.0317263888622535,
-0.0111637857573716));
#21780=CARTESIAN_POINT('Ctrl Pts',(-0.011342896161655,-0.0317269852962187,
-0.0111550669867109));
#21781=CARTESIAN_POINT('Ctrl Pts',(-0.0113473431960032,-0.0317273281753524,
-0.0111500481110629));
#21782=CARTESIAN_POINT('Ctrl Pts',(-0.0113625144457699,-0.0317284817601491,
-0.0111331492301612));
#21783=CARTESIAN_POINT('Ctrl Pts',(-0.0113733910411831,-0.0317292818058187,
-0.0111214067838658));
#21784=CARTESIAN_POINT('Ctrl Pts',(-0.0114005710316521,-0.0317312220403453,
-0.0110929638574415));
#21785=CARTESIAN_POINT('Ctrl Pts',(-0.0114170746473165,-0.0317323499411187,
-0.0110764596620695));
#21786=CARTESIAN_POINT('Ctrl Pts',(-0.0114897944134372,-0.0317371412862598,
-0.0110069644607968));
#21787=CARTESIAN_POINT('Ctrl Pts',(-0.0115495740244434,-0.0317406407346818,
-0.0109578597792837));
#21788=CARTESIAN_POINT('Ctrl Pts',(-0.0116880512975171,-0.0317483843806724,
-0.0108605389232706));
#21789=CARTESIAN_POINT('Ctrl Pts',(-0.0117678951791015,-0.0317526346948226,
-0.0108144815196708));
#21790=CARTESIAN_POINT('Ctrl Pts',(-0.0118712875394283,-0.0317582209022481,
-0.0107665797076639));
#21791=CARTESIAN_POINT('Ctrl Pts',(-0.0118914099420664,-0.0317593108955528,
-0.0107577737898283));
#21792=CARTESIAN_POINT('Ctrl Pts',(-0.0119216871275012,-0.0317609581386278,
-0.0107452870948034));
#21793=CARTESIAN_POINT('Ctrl Pts',(-0.0119317041149455,-0.0317615042593862,
-0.0107412783715227));
#21794=CARTESIAN_POINT('Ctrl Pts',(-0.011949758379731,-0.0317624909408469,
-0.0107342719574853));
#21795=CARTESIAN_POINT('Ctrl Pts',(-0.0119577802259509,-0.0317629301730841,
-0.0107312355926018));
#21796=CARTESIAN_POINT('Ctrl Pts',(-0.0119749439893212,-0.0317638718940798,
-0.0107249020033856));
#21797=CARTESIAN_POINT('Ctrl Pts',(-0.0119840925476679,-0.0317643750033485,
-0.0107216239596289));
#21798=CARTESIAN_POINT('Ctrl Pts',(-0.0120090515854803,-0.0317657509490294,
-0.0107129459846599));
#21799=CARTESIAN_POINT('Ctrl Pts',(-0.0120249194718407,-0.0317666293757518,
-0.0107077161738364));
#21800=CARTESIAN_POINT('Ctrl Pts',(-0.0121246045041788,-0.0317721721395204,
-0.010676646821809));
#21801=CARTESIAN_POINT('Ctrl Pts',(-0.0122104013007253,-0.0317770630400579,
-0.0106577391190128));
#21802=CARTESIAN_POINT('Ctrl Pts',(-0.0123820202042009,-0.0317869496649744,
-0.0106350001679799));
#21803=CARTESIAN_POINT('Ctrl Pts',(-0.0124674965099922,-0.0317919203460436,
-0.0106308318749435));
#21804=CARTESIAN_POINT('Ctrl Pts',(-0.0125913970206836,-0.0317988969046917,
-0.0106350804242895));
#21805=CARTESIAN_POINT('Ctrl Pts',(-0.0126298556022816,-0.0318010285394772,
-0.0106378440581973));
#21806=CARTESIAN_POINT('Ctrl Pts',(-0.0126775947549223,-0.0318036000286029,
-0.0106430783709083));
#21807=CARTESIAN_POINT('Ctrl Pts',(-0.0126870071505291,-0.0318041033853816,
-0.0106441982426557));
#21808=CARTESIAN_POINT('Ctrl Pts',(-0.0127018158172239,-0.0318048889279331,
-0.0106460987008032));
#21809=CARTESIAN_POINT('Ctrl Pts',(-0.0127072191454741,-0.0318051742088032,
-0.0106468212580266));
#21810=CARTESIAN_POINT('Ctrl Pts',(-0.0127174478545807,-0.0318057115568389,
-0.0106482443040263));
#21811=CARTESIAN_POINT('Ctrl Pts',(-0.0127222738468022,-0.0318059639233734,
-0.0106489390419921));
#21812=CARTESIAN_POINT('Ctrl Pts',(-0.0127337215038839,-0.0318065599275467,
-0.0106506424418905));
#21813=CARTESIAN_POINT('Ctrl Pts',(-0.0127403401075631,-0.0318069024333957,
-0.0106516713755119));
#21814=CARTESIAN_POINT('Ctrl Pts',(-0.0127627051048666,-0.031808053377305,
-0.0106552975609974));
#21815=CARTESIAN_POINT('Ctrl Pts',(-0.0127784183023889,-0.031808851221472,
-0.010658096068466));
#21816=CARTESIAN_POINT('Ctrl Pts',(-0.0128169063445851,-0.0318107850220818,
-0.0106655686193845));
#21817=CARTESIAN_POINT('Ctrl Pts',(-0.012839624779767,-0.0318119087968367,
-0.0106705146189658));
#21818=CARTESIAN_POINT('Ctrl Pts',(-0.0129367571694401,-0.0318166695232632,
-0.0106939722459075));
#21819=CARTESIAN_POINT('Ctrl Pts',(-0.013009849350703,-0.031820144561209,
-0.0107175038186367));
#21820=CARTESIAN_POINT('Ctrl Pts',(-0.0131668980918235,-0.0318278993658513,
-0.0107813231004393));
#21821=CARTESIAN_POINT('Ctrl Pts',(-0.0132495690237774,-0.0318321861072869,
-0.0108239613746075));
#21822=CARTESIAN_POINT('Ctrl Pts',(-0.0133463750261516,-0.0318378106396406,
-0.0108855131817872));
#21823=CARTESIAN_POINT('Ctrl Pts',(-0.0133645964665641,-0.0318388972158917,
-0.01089765097047));
#21824=CARTESIAN_POINT('Ctrl Pts',(-0.013391391948244,-0.0318405402915505,
-0.0109163353195115));
#21825=CARTESIAN_POINT('Ctrl Pts',(-0.013400165969161,-0.0318410857470344,
-0.0109225910095268));
#21826=CARTESIAN_POINT('Ctrl Pts',(-0.0134158039776208,-0.0318420717059085,
-0.0109339895168248));
#21827=CARTESIAN_POINT('Ctrl Pts',(-0.013422692017339,-0.0318425108891388,
-0.0109390986685371));
#21828=CARTESIAN_POINT('Ctrl Pts',(-0.0134373008046071,-0.0318434530307015,
-0.0109501245995892));
#21829=CARTESIAN_POINT('Ctrl Pts',(-0.0134450088862328,-0.031843956615434,
-0.0109560574792675));
#21830=CARTESIAN_POINT('Ctrl Pts',(-0.0134658350799753,-0.0318453352274491,
-0.0109724032046639));
#21831=CARTESIAN_POINT('Ctrl Pts',(-0.0134788403150553,-0.0318462158815942,
-0.0109829571850283));
#21832=CARTESIAN_POINT('Ctrl Pts',(-0.0135599560775883,-0.0318518367961169,
-0.0110510038017946));
#21833=CARTESIAN_POINT('Ctrl Pts',(-0.0136231399884212,-0.0318568115473902,
-0.0111140878365509));
#21834=CARTESIAN_POINT('Ctrl Pts',(-0.0137371225708579,-0.0318669267327057,
-0.0112495145873098));
#21835=CARTESIAN_POINT('Ctrl Pts',(-0.0137878748009157,-0.0318720434887797,
-0.0113214796170112));
#21836=CARTESIAN_POINT('Ctrl Pts',(-0.0138499070741362,-0.0318789373447697,
-0.0114276364890068));
#21837=CARTESIAN_POINT('Ctrl Pts',(-0.0138665555018071,-0.0318808691789927,
-0.0114584943213541));
#21838=CARTESIAN_POINT('Ctrl Pts',(-0.0138862393816572,-0.0318832380413681,
-0.0114981553964777));
#21839=CARTESIAN_POINT('Ctrl Pts',(-0.013890265281936,-0.031883727492543,
-0.0115064531763914));
#21840=CARTESIAN_POINT('Ctrl Pts',(-0.0138965281904415,-0.0318844963049612,
-0.0115196619091663));
#21841=CARTESIAN_POINT('Ctrl Pts',(-0.0138988141917251,-0.0318847785531938,
-0.0115245492337199));
#21842=CARTESIAN_POINT('Ctrl Pts',(-0.0139031249124826,-0.0318853137806134,
-0.0115338926690531));
#21843=CARTESIAN_POINT('Ctrl Pts',(-0.0139051541117647,-0.0318855670177228,
-0.0115383465204142));
#21844=CARTESIAN_POINT('Ctrl Pts',(-0.0139099595100629,-0.0318861699647982,
-0.0115490282139574));
#21845=CARTESIAN_POINT('Ctrl Pts',(-0.013912715715472,-0.0318865184664609,
-0.0115552650154181));
#21846=CARTESIAN_POINT('Ctrl Pts',(-0.013922078927995,-0.031887712405295,
-0.0115768379581493));
#21847=CARTESIAN_POINT('Ctrl Pts',(-0.0139284784774628,-0.0318885461455529,
-0.0115922634278809));
#21848=CARTESIAN_POINT('Ctrl Pts',(-0.0139437284609508,-0.0318905856554026,
-0.0116307768201803));
#21849=CARTESIAN_POINT('Ctrl Pts',(-0.0139522769493644,-0.0318917774295723,
-0.0116539797495911));
#21850=CARTESIAN_POINT('Ctrl Pts',(-0.0139882901032485,-0.0318970719356118,
-0.0117594791351609));
#21851=CARTESIAN_POINT('Ctrl Pts',(-0.0140093433701723,-0.0319009749002342,
-0.0118438004972352));
#21852=CARTESIAN_POINT('Ctrl Pts',(-0.0140363806581955,-0.0319087461953,
-0.0120109363637244));
#21853=CARTESIAN_POINT('Ctrl Pts',(-0.0140430000004134,-0.031912595402268,
-0.0120933357057804));
#21854=CARTESIAN_POINT('Ctrl Pts',(-0.014043,-0.0319166517728185,-0.012175853294288));
#21855=CARTESIAN_POINT('Origin',(-0.0125,-0.0375520664398416,-0.0121758532865581));
#21856=CARTESIAN_POINT('',(-0.014043,-0.0324174341340783,-0.0121758532914128));
#21857=CARTESIAN_POINT('',(-0.014043,-0.0323021764224865,-0.0121758532515513));
#21858=CARTESIAN_POINT('',(-0.014043,-0.0375520664398416,-0.012175853286558));
#21859=CARTESIAN_POINT('Ctrl Pts',(-0.014043,-0.0323021764244909,-0.0121758532514363));
#21860=CARTESIAN_POINT('Ctrl Pts',(-0.0140429999996933,-0.0323014024090168,
-0.0121623792514412));
#21861=CARTESIAN_POINT('Ctrl Pts',(-0.0140428235103971,-0.0323006271566412,
-0.0121489018304193));
#21862=CARTESIAN_POINT('Ctrl Pts',(-0.0140408270881201,-0.0322962438293193,
-0.0120727329270992));
#21863=CARTESIAN_POINT('Ctrl Pts',(-0.0140353633656632,-0.032292635035969,
-0.0120101972794149));
#21864=CARTESIAN_POINT('Ctrl Pts',(-0.0140230358114081,-0.0322879765861664,
-0.0119275701132655));
#21865=CARTESIAN_POINT('Ctrl Pts',(-0.0140195463323506,-0.0322868284354249,
-0.0119070380506838));
#21866=CARTESIAN_POINT('Ctrl Pts',(-0.0140128878450054,-0.032284900661059,
-0.0118721507694607));
#21867=CARTESIAN_POINT('Ctrl Pts',(-0.0140099274416961,-0.0322841121881339,
-0.0118577589574257));
#21868=CARTESIAN_POINT('Ctrl Pts',(-0.0140053688660552,-0.0322829922003959,
-0.0118370976558387));
#21869=CARTESIAN_POINT('Ctrl Pts',(-0.0140039362113176,-0.032282652052595,
-0.0118307928926249));
#21870=CARTESIAN_POINT('Ctrl Pts',(-0.0140013647676637,-0.0322820618640116,
-0.0118197969211683));
#21871=CARTESIAN_POINT('Ctrl Pts',(-0.0140002435303095,-0.0322818108450363,
-0.0118151017753191));
#21872=CARTESIAN_POINT('Ctrl Pts',(-0.013997789552853,-0.0322812748217816,
-0.01180503516218));
#21873=CARTESIAN_POINT('Ctrl Pts',(-0.0139964499356728,-0.0322809902103484,
-0.0117996655436832));
#21874=CARTESIAN_POINT('Ctrl Pts',(-0.0139926912207524,-0.0322802128617021,
-0.011784937242925));
#21875=CARTESIAN_POINT('Ctrl Pts',(-0.0139902129889699,-0.0322797234015583,
-0.0117755937579562));
#21876=CARTESIAN_POINT('Ctrl Pts',(-0.0139760053679398,-0.0322770374793962,
-0.0117239897731068));
#21877=CARTESIAN_POINT('Ctrl Pts',(-0.013962565230283,-0.032274927781438,
-0.0116822177737148));
#21878=CARTESIAN_POINT('Ctrl Pts',(-0.0139190434010339,-0.0322690209717205,
-0.0115644277510888));
#21879=CARTESIAN_POINT('Ctrl Pts',(-0.0138846801153873,-0.0322653423961703,
-0.0114901511835274));
#21880=CARTESIAN_POINT('Ctrl Pts',(-0.0138061657954547,-0.0322579859731393,
-0.011350676282501));
#21881=CARTESIAN_POINT('Ctrl Pts',(-0.0137625961580761,-0.0322543240921222,
-0.0112854401602769));
#21882=CARTESIAN_POINT('Ctrl Pts',(-0.0137013501291463,-0.0322494488460696,
-0.0112073260525811));
#21883=CARTESIAN_POINT('Ctrl Pts',(-0.0136881015250762,-0.0322484086226143,
-0.0111911188811897));
#21884=CARTESIAN_POINT('Ctrl Pts',(-0.0136676780585777,-0.0322468235214271,
-0.0111671469333451));
#21885=CARTESIAN_POINT('Ctrl Pts',(-0.013660746145708,-0.0322462885816627,
-0.0111591778548133));
#21886=CARTESIAN_POINT('Ctrl Pts',(-0.0136480718860771,-0.0322453156526887,
-0.0111449058425988));
#21887=CARTESIAN_POINT('Ctrl Pts',(-0.0136423580375394,-0.0322448788703348,
-0.0111385781070625));
#21888=CARTESIAN_POINT('Ctrl Pts',(-0.0136299642480799,-0.0322439352084256,
-0.0111250793635263));
#21889=CARTESIAN_POINT('Ctrl Pts',(-0.0136232678644398,-0.0322434276324282,
-0.0111179240176503));
#21890=CARTESIAN_POINT('Ctrl Pts',(-0.013604933054889,-0.0322420437799935,
-0.0110987028936592));
#21891=CARTESIAN_POINT('Ctrl Pts',(-0.0135931656490724,-0.032241161906209,
-0.011086762446262));
#21892=CARTESIAN_POINT('Ctrl Pts',(-0.0135145892371655,-0.0322353122326807,
-0.0110095872392964));
#21893=CARTESIAN_POINT('Ctrl Pts',(-0.0134421802690433,-0.0322300853874455,
-0.0109503494476973));
#21894=CARTESIAN_POINT('Ctrl Pts',(-0.0132962289054131,-0.0322199963196308,
-0.0108515651732669));
#21895=CARTESIAN_POINT('Ctrl Pts',(-0.0132239530049224,-0.0322151795230815,
-0.010810711575507));
#21896=CARTESIAN_POINT('Ctrl Pts',(-0.0131268248095656,-0.0322091751821878,
-0.0107657031799728));
#21897=CARTESIAN_POINT('Ctrl Pts',(-0.0131046682162367,-0.0322078358229432,
-0.0107560613594998));
#21898=CARTESIAN_POINT('Ctrl Pts',(-0.0130671014424623,-0.0322056259069295,
-0.0107407525663575));
#21899=CARTESIAN_POINT('Ctrl Pts',(-0.0130518110852945,-0.0322047430254511,
-0.0107348041230554));
#21900=CARTESIAN_POINT('Ctrl Pts',(-0.0130300954901301,-0.0322035153834349,
-0.0107267523971341));
#21901=CARTESIAN_POINT('Ctrl Pts',(-0.0130237473259522,-0.0322031596364759,
-0.0107244459149776));
#21902=CARTESIAN_POINT('Ctrl Pts',(-0.0130127983454962,-0.0322025516975174,
-0.010720549005675));
#21903=CARTESIAN_POINT('Ctrl Pts',(-0.0130082048110785,-0.0322022983446181,
-0.0107189385445465));
#21904=CARTESIAN_POINT('Ctrl Pts',(-0.0129985127033996,-0.0322017674475736,
-0.0107155919772538));
#21905=CARTESIAN_POINT('Ctrl Pts',(-0.0129934125866443,-0.0322014901870418,
-0.0107138608009521));
#21906=CARTESIAN_POINT('Ctrl Pts',(-0.0129795343760125,-0.0322007411634398,
-0.0107092308958848));
#21907=CARTESIAN_POINT('Ctrl Pts',(-0.0129707389993778,-0.0322002723613871,
-0.0107063842473956));
#21908=CARTESIAN_POINT('Ctrl Pts',(-0.0129279224990572,-0.032198016373534,
-0.0106929504496126));
#21909=CARTESIAN_POINT('Ctrl Pts',(-0.0128935650285831,-0.0321962858672358,
-0.010683464129016));
#21910=CARTESIAN_POINT('Ctrl Pts',(-0.0127737697465406,-0.0321904305936913,
-0.0106548134393784));
#21911=CARTESIAN_POINT('Ctrl Pts',(-0.0126870491266767,-0.0321864932091093,
-0.0106417325660733));
#21912=CARTESIAN_POINT('Ctrl Pts',(-0.0125109318388377,-0.0321783922995229,
-0.0106303309326174));
#21913=CARTESIAN_POINT('Ctrl Pts',(-0.012421856794486,-0.0321742379998419,
-0.0106322697170178));
#21914=CARTESIAN_POINT('Ctrl Pts',(-0.0123168511923568,-0.0321690070947061,
-0.0106436704194866));
#21915=CARTESIAN_POINT('Ctrl Pts',(-0.0123002815129674,-0.032168172158224,
-0.0106457420741262));
#21916=CARTESIAN_POINT('Ctrl Pts',(-0.0122741546431794,-0.0321668392922129,
-0.0106494402451697));
#21917=CARTESIAN_POINT('Ctrl Pts',(-0.0122645733314575,-0.0321663470123645,
-0.0106508886390163));
#21918=CARTESIAN_POINT('Ctrl Pts',(-0.0122465765331201,-0.0321654155456725,
-0.0106537828389171));
#21919=CARTESIAN_POINT('Ctrl Pts',(-0.0122381581429432,-0.0321649770190096,
-0.0106552084433648));
#21920=CARTESIAN_POINT('Ctrl Pts',(-0.012219197687725,-0.0321639828298705,
-0.0106585813982888));
#21921=CARTESIAN_POINT('Ctrl Pts',(-0.0122086632869483,-0.0321634259017085,
-0.0106605688798174));
#21922=CARTESIAN_POINT('Ctrl Pts',(-0.0121775280171883,-0.0321617660248295,
-0.0106667797179403));
#21923=CARTESIAN_POINT('Ctrl Pts',(-0.0121569923994884,-0.0321606531911222,
-0.0106713145059951));
#21924=CARTESIAN_POINT('Ctrl Pts',(-0.012028020395348,-0.0321535475888209,
-0.0107025724913517));
#21925=CARTESIAN_POINT('Ctrl Pts',(-0.0119226761109214,-0.0321471850232166,
-0.0107405794132459));
#21926=CARTESIAN_POINT('Ctrl Pts',(-0.0117657791738965,-0.0321371385022699,
-0.0108172743186234));
#21927=CARTESIAN_POINT('Ctrl Pts',(-0.011710931187045,-0.0321335130317843,
-0.0108483789565857));
#21928=CARTESIAN_POINT('Ctrl Pts',(-0.0116406414486539,-0.0321288356149218,
-0.0108941404923349));
#21929=CARTESIAN_POINT('Ctrl Pts',(-0.0116233786649854,-0.0321276844641987,
-0.0109058848175271));
#21930=CARTESIAN_POINT('Ctrl Pts',(-0.0115943592308539,-0.0321257522141839,
-0.0109265012690223));
#21931=CARTESIAN_POINT('Ctrl Pts',(-0.0115824817568368,-0.0321249622150257,
-0.0109351978263089));
#21932=CARTESIAN_POINT('Ctrl Pts',(-0.0115655649451977,-0.0321238404745172,
-0.0109479599722));
#21933=CARTESIAN_POINT('Ctrl Pts',(-0.0115604242233197,-0.0321235000641672,
-0.0109518891425114));
#21934=CARTESIAN_POINT('Ctrl Pts',(-0.0115514911714856,-0.0321229095813506,
-0.0109588063240946));
#21935=CARTESIAN_POINT('Ctrl Pts',(-0.0115476879231135,-0.0321226585276164,
-0.0109617799703976));
#21936=CARTESIAN_POINT('Ctrl Pts',(-0.0115395571341245,-0.0321221226115552,
-0.0109681989087729));
#21937=CARTESIAN_POINT('Ctrl Pts',(-0.0115352341138763,-0.0321218381400629,
-0.0109716496569232));
#21938=CARTESIAN_POINT('Ctrl Pts',(-0.0115234173981948,-0.0321210615560551,
-0.010981186548432));
#21939=CARTESIAN_POINT('Ctrl Pts',(-0.0115159620002614,-0.0321205727100189,
-0.0109873199814207));
#21940=CARTESIAN_POINT('Ctrl Pts',(-0.0114751411846417,-0.0321178992648421,
-0.0110215500197178));
#21941=CARTESIAN_POINT('Ctrl Pts',(-0.0114429186950757,-0.0321158004714033,
-0.0110509838181382));
#21942=CARTESIAN_POINT('Ctrl Pts',(-0.0113539269842558,-0.032109895319126,
-0.0111394800000965));
#21943=CARTESIAN_POINT('Ctrl Pts',(-0.0113005548730207,-0.0321062092793998,
-0.0112017458049318));
#21944=CARTESIAN_POINT('Ctrl Pts',(-0.0112062339021968,-0.0320988418406193,
-0.0113313608100745));
#21945=CARTESIAN_POINT('Ctrl Pts',(-0.0111649973353384,-0.0320951766149079,
-0.0113981871873302));
#21946=CARTESIAN_POINT('Ctrl Pts',(-0.0111194116557756,-0.0320902971958638,
-0.0114864598123865));
#21947=CARTESIAN_POINT('Ctrl Pts',(-0.011110182906361,-0.0320892565078004,
-0.0115052595706263));
#21948=CARTESIAN_POINT('Ctrl Pts',(-0.0110968787278661,-0.0320876708385675,
-0.0115338164565803));
#21949=CARTESIAN_POINT('Ctrl Pts',(-0.0110925161102953,-0.0320871358063374,
-0.0115434375306079));
#21950=CARTESIAN_POINT('Ctrl Pts',(-0.0110848116882396,-0.0320861627790461,
-0.0115609030997182));
#21951=CARTESIAN_POINT('Ctrl Pts',(-0.0110814354390259,-0.0320857259919911,
-0.0115687319868926));
#21952=CARTESIAN_POINT('Ctrl Pts',(-0.0110743187512896,-0.0320847823987675,
-0.0115856177494684));
#21953=CARTESIAN_POINT('Ctrl Pts',(-0.0110705993703399,-0.032084274897052,
-0.0115946830480476));
#21954=CARTESIAN_POINT('Ctrl Pts',(-0.0110607537182774,-0.0320828914462587,
-0.0116193463606848));
#21955=CARTESIAN_POINT('Ctrl Pts',(-0.011054794920006,-0.0320820099052575,
-0.0116350094414325));
#21956=CARTESIAN_POINT('Ctrl Pts',(-0.0110177761448494,-0.0320762323051437,
-0.0117372987639338));
#21957=CARTESIAN_POINT('Ctrl Pts',(-0.0109942680790685,-0.0320710852195581,
-0.0118264470815429));
#21958=CARTESIAN_POINT('Ctrl Pts',(-0.0109647616807814,-0.0320610157007253,
-0.0119999402523358));
#21959=CARTESIAN_POINT('Ctrl Pts',(-0.0109574635849771,-0.032056133265962,
-0.0120837456160181));
#21960=CARTESIAN_POINT('Ctrl Pts',(-0.0109568933609971,-0.0320500572486341,
-0.0121920443636418));
#21961=CARTESIAN_POINT('Ctrl Pts',(-0.0109573401127474,-0.0320487088891805,
-0.0122163604111844));
#21962=CARTESIAN_POINT('Ctrl Pts',(-0.0109590536773698,-0.0320464858426147,
-0.0122571251699337));
#21963=CARTESIAN_POINT('Ctrl Pts',(-0.0109600098025389,-0.032045598654852,
-0.0122735821097014));
#21964=CARTESIAN_POINT('Ctrl Pts',(-0.0109617301546598,-0.0320443661384221,
-0.0122967692483317));
#21965=CARTESIAN_POINT('Ctrl Pts',(-0.0109622752140964,-0.0320440097099208,
-0.0123035140599565));
#21966=CARTESIAN_POINT('Ctrl Pts',(-0.0109632887936613,-0.0320434009845412,
-0.012315106224637));
#21967=CARTESIAN_POINT('Ctrl Pts',(-0.0109637359201621,-0.032043147518766,
-0.0123199553054482));
#21968=CARTESIAN_POINT('Ctrl Pts',(-0.0109647253659352,-0.0320426167946495,
-0.0123301573491021));
#21969=CARTESIAN_POINT('Ctrl Pts',(-0.0109652727324225,-0.0320423398155694,
-0.0123355096725717));
#21970=CARTESIAN_POINT('Ctrl Pts',(-0.0109668338688409,-0.0320415923790633,
-0.0123500244361822));
#21971=CARTESIAN_POINT('Ctrl Pts',(-0.010967901783508,-0.032041124861347,
-0.0123591809659832));
#21972=CARTESIAN_POINT('Ctrl Pts',(-0.0109734549035827,-0.0320388866200802,
-0.0124033507051559));
#21973=CARTESIAN_POINT('Ctrl Pts',(-0.0109790589215706,-0.0320371715013044,
-0.01243821482079));
#21974=CARTESIAN_POINT('Ctrl Pts',(-0.0110027495082845,-0.0320313180628234,
-0.0125589906133852));
#21975=CARTESIAN_POINT('Ctrl Pts',(-0.0110269641510058,-0.0320273702158028,
-0.0126435287443692));
#21976=CARTESIAN_POINT('Ctrl Pts',(-0.0110899706560847,-0.0320192526330271,
-0.0128087834626587));
#21977=CARTESIAN_POINT('Ctrl Pts',(-0.0111288488893611,-0.0320150923741797,
-0.0128891034036025));
#21978=CARTESIAN_POINT('Ctrl Pts',(-0.0111829827757266,-0.0320098545022367,
-0.0129799637173531));
#21979=CARTESIAN_POINT('Ctrl Pts',(-0.0111917635861749,-0.0320090193762505,
-0.0129941719360176));
#21980=CARTESIAN_POINT('Ctrl Pts',(-0.0112060009354054,-0.0320076862766123,
-0.0130163943831706));
#21981=CARTESIAN_POINT('Ctrl Pts',(-0.0112113054498348,-0.0320071939560945,
-0.0130245047256277));
#21982=CARTESIAN_POINT('Ctrl Pts',(-0.0112214264970593,-0.0320062624552239,
-0.013039665590713));
#21983=CARTESIAN_POINT('Ctrl Pts',(-0.0112262258540188,-0.0320058239356048,
-0.0130467271697072));
#21984=CARTESIAN_POINT('Ctrl Pts',(-0.0112371820506617,-0.0320048298206117,
-0.0130625633413006));
#21985=CARTESIAN_POINT('Ctrl Pts',(-0.0112433721724092,-0.0320042729603208,
-0.0130713142792607));
#21986=CARTESIAN_POINT('Ctrl Pts',(-0.0112623915357128,-0.0320025760020515,
-0.0130976162162919));
#21987=CARTESIAN_POINT('Ctrl Pts',(-0.011275500610095,-0.0320014250975602,
-0.0131149607290215));
#21988=CARTESIAN_POINT('Ctrl Pts',(-0.0113491114112831,-0.0319950598003242,
-0.0132081919729491));
#21989=CARTESIAN_POINT('Ctrl Pts',(-0.0114162954365855,-0.0319895757749732,
-0.0132785079835967));
#21990=CARTESIAN_POINT('Ctrl Pts',(-0.0115452768988058,-0.031979773896115,
-0.0133902561919174));
#21991=CARTESIAN_POINT('Ctrl Pts',(-0.0116043083131546,-0.0319755120036411,
-0.0134344269360474));
#21992=CARTESIAN_POINT('Ctrl Pts',(-0.0116854032086831,-0.0319701192544387,
-0.0134865012690919));
#21993=CARTESIAN_POINT('Ctrl Pts',(-0.0117048071894857,-0.031968861450865,
-0.0134983639854986));
#21994=CARTESIAN_POINT('Ctrl Pts',(-0.0117380292250366,-0.0319667711180667,
-0.0135176787747676));
#21995=CARTESIAN_POINT('Ctrl Pts',(-0.0117517113655891,-0.0319659278084603,
-0.0135253566246823));
#21996=CARTESIAN_POINT('Ctrl Pts',(-0.0117713445580545,-0.0319647451036616,
-0.0135359835309754));
#21997=CARTESIAN_POINT('Ctrl Pts',(-0.011777200816211,-0.031964395739545,
-0.0135391046859483));
#21998=CARTESIAN_POINT('Ctrl Pts',(-0.0117873716285336,-0.0319637951248527,
-0.0135444413635362));
#21999=CARTESIAN_POINT('Ctrl Pts',(-0.0117916767836761,-0.0319635427881837,
-0.0135466744797905));
#22000=CARTESIAN_POINT('Ctrl Pts',(-0.0118008351341862,-0.0319630100786934,
-0.0135513703188797));
#22001=CARTESIAN_POINT('Ctrl Pts',(-0.0118056908919372,-0.03196273003183,
-0.013553827698524));
#22002=CARTESIAN_POINT('Ctrl Pts',(-0.0118190602724995,-0.0319619652660586,
-0.0135605050023124));
#22003=CARTESIAN_POINT('Ctrl Pts',(-0.0118276001633642,-0.0319614837230102,
-0.0135646721209505));
#22004=CARTESIAN_POINT('Ctrl Pts',(-0.0118716424635831,-0.0319590331655217,
-0.013585661491315));
#22005=CARTESIAN_POINT('Ctrl Pts',(-0.0119077418968354,-0.0319571333865021,
-0.0136012034711843));
#22006=CARTESIAN_POINT('Ctrl Pts',(-0.0120236538055205,-0.0319512561800969,
-0.0136459419296564));
#22007=CARTESIAN_POINT('Ctrl Pts',(-0.0121053042773844,-0.0319474337372591,
-0.0136699359365906));
#22008=CARTESIAN_POINT('Ctrl Pts',(-0.0122741850631011,-0.0319395143527983,
-0.0137047441389993));
#22009=CARTESIAN_POINT('Ctrl Pts',(-0.0123611914895947,-0.0319354237535049,
-0.0137150834938936));
#22010=CARTESIAN_POINT('Ctrl Pts',(-0.0124652440825787,-0.0319302672733225,
-0.0137185517071799));
#22011=CARTESIAN_POINT('Ctrl Pts',(-0.012481897348991,-0.0319294344280181,
-0.0137188369733155));
#22012=CARTESIAN_POINT('Ctrl Pts',(-0.0125082324792094,-0.0319281041401937,
-0.0137188616942558));
#22013=CARTESIAN_POINT('Ctrl Pts',(-0.0125179131024213,-0.0319276123093079,
-0.0137187796733674));
#22014=CARTESIAN_POINT('Ctrl Pts',(-0.0125361302775812,-0.0319266812190894,
-0.0137184538588422));
#22015=CARTESIAN_POINT('Ctrl Pts',(-0.0125446668504504,-0.0319262426138277,
-0.0137182302803985));
#22016=CARTESIAN_POINT('Ctrl Pts',(-0.012563928827658,-0.0319252476018939,
-0.0137175657525926));
#22017=CARTESIAN_POINT('Ctrl Pts',(-0.0125746522955975,-0.0319246899210072,
-0.0137170837202814));
#22018=CARTESIAN_POINT('Ctrl Pts',(-0.0126064345943363,-0.0319230256569791,
-0.0137153226009946));
#22019=CARTESIAN_POINT('Ctrl Pts',(-0.0126274725934355,-0.031921909111367,
-0.0137137234928307));
#22020=CARTESIAN_POINT('Ctrl Pts',(-0.0127582702136378,-0.0319148721889959,
-0.0137010792155449));
#22021=CARTESIAN_POINT('Ctrl Pts',(-0.0128665996690467,-0.0319085921787821,
-0.0136787223706112));
#22022=CARTESIAN_POINT('Ctrl Pts',(-0.0130324786803932,-0.0318985703388443,
-0.0136254750177988));
#22023=CARTESIAN_POINT('Ctrl Pts',(-0.0130920834450007,-0.0318948885563024,
-0.0136021683154359));
#22024=CARTESIAN_POINT('Ctrl Pts',(-0.0131691645023182,-0.0318901471835159,
-0.0135663607653334));
#22025=CARTESIAN_POINT('Ctrl Pts',(-0.0131880741132712,-0.0318889859838773,
-0.0135571013694842));
#22026=CARTESIAN_POINT('Ctrl Pts',(-0.0132199560174419,-0.0318870387537765,
-0.0135406725924551));
#22027=CARTESIAN_POINT('Ctrl Pts',(-0.0132330250925264,-0.0318862436531303,
-0.0135336981415434));
#22028=CARTESIAN_POINT('Ctrl Pts',(-0.013251670079468,-0.0318851160569593,
-0.013523400378333));
#22029=CARTESIAN_POINT('Ctrl Pts',(-0.0132573282642186,-0.0318847747715767,
-0.0135202285972891));
#22030=CARTESIAN_POINT('Ctrl Pts',(-0.0132671643151485,-0.0318841833068554,
-0.0135146330441754));
#22031=CARTESIAN_POINT('Ctrl Pts',(-0.0132713510550923,-0.0318839321360027,
-0.013512225195068));
#22032=CARTESIAN_POINT('Ctrl Pts',(-0.0132803003765,-0.0318833965713724,
-0.013507022251915));
#22033=CARTESIAN_POINT('Ctrl Pts',(-0.0132850593136585,-0.0318831125617741,
-0.0135042212204468));
#22034=CARTESIAN_POINT('Ctrl Pts',(-0.0132980610852545,-0.03188233850035,
-0.013496474317329));
#22035=CARTESIAN_POINT('Ctrl Pts',(-0.0133062730271159,-0.031881851680172,
-0.0134914767955324));
#22036=CARTESIAN_POINT('Ctrl Pts',(-0.0133508280585645,-0.0318792187936029,
-0.0134637881742982));
#22037=CARTESIAN_POINT('Ctrl Pts',(-0.0133862633597354,-0.0318771554557466,
-0.0134396659599712));
#22038=CARTESIAN_POINT('Ctrl Pts',(-0.0134867964851076,-0.0318712556472463,
-0.0133649182943407));
#22039=CARTESIAN_POINT('Ctrl Pts',(-0.0135488972606294,-0.0318675453688137,
-0.013310515586894));
#22040=CARTESIAN_POINT('Ctrl Pts',(-0.0136611935207123,-0.0318601421039148,
-0.0131950036282095));
#22041=CARTESIAN_POINT('Ctrl Pts',(-0.0137116321733821,-0.0318564659579765,
-0.0131344896602007));
#22042=CARTESIAN_POINT('Ctrl Pts',(-0.0137693929830662,-0.0318515729131813,
-0.0130533100132674));
#22043=CARTESIAN_POINT('Ctrl Pts',(-0.0137812017001961,-0.0318505307102753,
-0.0130359759540137));
#22044=CARTESIAN_POINT('Ctrl Pts',(-0.0137984248661999,-0.0318489431890256,
-0.0130095520284163));
#22045=CARTESIAN_POINT('Ctrl Pts',(-0.0138041053777642,-0.0318484078554346,
-0.0130006380353296));
#22046=CARTESIAN_POINT('Ctrl Pts',(-0.0138142017696548,-0.0318474345075051,
-0.0129844294462429));
#22047=CARTESIAN_POINT('Ctrl Pts',(-0.0138186496473569,-0.0318469977049215,
-0.0129771552277894));
#22048=CARTESIAN_POINT('Ctrl Pts',(-0.0138280767564826,-0.0318460543346053,
-0.0129614467266122));
#22049=CARTESIAN_POINT('Ctrl Pts',(-0.0138330364100274,-0.0318455470742361,
-0.0129530011796582));
#22050=CARTESIAN_POINT('Ctrl Pts',(-0.0138462531932358,-0.0318441649282978,
-0.0129299961686877));
#22051=CARTESIAN_POINT('Ctrl Pts',(-0.0138543542076786,-0.0318432844684109,
-0.0129153489236433));
#22052=CARTESIAN_POINT('Ctrl Pts',(-0.0139061215541963,-0.0318374308466215,
-0.0128180447586783));
#22053=CARTESIAN_POINT('Ctrl Pts',(-0.0139424311107755,-0.0318321979428736,
-0.0127317091060275));
#22054=CARTESIAN_POINT('Ctrl Pts',(-0.0139910963525862,-0.0318229885074964,
-0.0125783767836752));
#22055=CARTESIAN_POINT('Ctrl Pts',(-0.0140072568250182,-0.0318190829830428,
-0.0125128553779215));
#22056=CARTESIAN_POINT('Ctrl Pts',(-0.0140278290876955,-0.031812422048736,
-0.0123973822912105));
#22057=CARTESIAN_POINT('Ctrl Pts',(-0.0140341920576218,-0.0318096367507819,
-0.0123478776869965));
#22058=CARTESIAN_POINT('Ctrl Pts',(-0.0140389177835271,-0.0318064415575806,
-0.0122884405341281));
#22059=CARTESIAN_POINT('Ctrl Pts',(-0.0140395977153843,-0.0318059240643805,
-0.0122787256205836));
#22060=CARTESIAN_POINT('Ctrl Pts',(-0.0140405172755869,-0.031805122299086,
-0.0122635214099575));
#22061=CARTESIAN_POINT('Ctrl Pts',(-0.0140408196282058,-0.0318048347066493,
-0.0122580363226576));
#22062=CARTESIAN_POINT('Ctrl Pts',(-0.0140413330832879,-0.031804297025581,
-0.0122477192516973));
#22063=CARTESIAN_POINT('Ctrl Pts',(-0.0140415507622473,-0.0318040465978552,
-0.0122428878919822));
#22064=CARTESIAN_POINT('Ctrl Pts',(-0.0140420046998314,-0.0318034664649263,
-0.0122316365662889));
#22065=CARTESIAN_POINT('Ctrl Pts',(-0.0140422235856369,-0.0318031377252097,
-0.0122252160593249));
#22066=CARTESIAN_POINT('Ctrl Pts',(-0.0140428007586163,-0.0318020831670447,
-0.012204484510068));
#22067=CARTESIAN_POINT('Ctrl Pts',(-0.0140430000000001,-0.0318013656520773,
-0.0121901694497616));
#22068=CARTESIAN_POINT('Ctrl Pts',(-0.014043,-0.0318006569328344,-0.0121758532865438));
#22069=CARTESIAN_POINT('Ctrl Pts',(-0.014043,-0.0319166517728185,-0.012175853294288));
#22070=CARTESIAN_POINT('Ctrl Pts',(-0.0140429999999704,-0.0319169422534939,
-0.0121817624597713));
#22071=CARTESIAN_POINT('Ctrl Pts',(-0.0140429660548091,-0.0319172337445512,
-0.0121876722341942));
#22072=CARTESIAN_POINT('Ctrl Pts',(-0.0140427051512635,-0.0319183575977179,
-0.0122103777823771));
#22073=CARTESIAN_POINT('Ctrl Pts',(-0.0140422379333357,-0.0319191969743863,
-0.0122271685248212));
#22074=CARTESIAN_POINT('Ctrl Pts',(-0.0140410627718577,-0.0319205413333712,
-0.0122537713290109));
#22075=CARTESIAN_POINT('Ctrl Pts',(-0.01404053494283,-0.0319210406534681,
-0.012263590235529));
#22076=CARTESIAN_POINT('Ctrl Pts',(-0.0140393719069067,-0.0319219803902146,
-0.012281949790573));
#22077=CARTESIAN_POINT('Ctrl Pts',(-0.0140387593723613,-0.0319224200743601,
-0.012290491526098));
#22078=CARTESIAN_POINT('Ctrl Pts',(-0.0140372278659085,-0.0319234101772051,
-0.0123096154226401));
#22079=CARTESIAN_POINT('Ctrl Pts',(-0.0140362706686662,-0.03192396178414,
-0.0123201940145537));
#22080=CARTESIAN_POINT('Ctrl Pts',(-0.0140330862384887,-0.0319256194078617,
-0.012351752990122));
#22081=CARTESIAN_POINT('Ctrl Pts',(-0.0140305379026275,-0.0319267354658688,
-0.0123726978684155));
#22082=CARTESIAN_POINT('Ctrl Pts',(-0.0140163573164733,-0.0319321145826708,
-0.0124721867527332));
#22083=CARTESIAN_POINT('Ctrl Pts',(-0.0139991047897372,-0.0319365516829508,
-0.0125497986723084));
#22084=CARTESIAN_POINT('Ctrl Pts',(-0.0139514649066583,-0.031945879745736,
-0.0127060959049457));
#22085=CARTESIAN_POINT('Ctrl Pts',(-0.0139204468957665,-0.0319507665606939,
-0.0127843253274699));
#22086=CARTESIAN_POINT('Ctrl Pts',(-0.0138652568777996,-0.0319577884795798,
-0.0128959677289772));
#22087=CARTESIAN_POINT('Ctrl Pts',(-0.0138458731720214,-0.0319600340530743,
-0.0129315761544118));
#22088=CARTESIAN_POINT('Ctrl Pts',(-0.0138201805120936,-0.0319627204035708,
-0.0129746429565677));
#22089=CARTESIAN_POINT('Ctrl Pts',(-0.0138151752260996,-0.031963231396606,
-0.0129828574100301));
#22090=CARTESIAN_POINT('Ctrl Pts',(-0.0138071972516023,-0.0319640261151596,
-0.0129956791193369));
#22091=CARTESIAN_POINT('Ctrl Pts',(-0.0138042763461494,-0.031964313052479,
-0.0130003181223142));
#22092=CARTESIAN_POINT('Ctrl Pts',(-0.0137987156101211,-0.0319648516270746,
-0.0130090462121896));
#22093=CARTESIAN_POINT('Ctrl Pts',(-0.0137960811021365,-0.0319651035859133,
-0.0130131384615522));
#22094=CARTESIAN_POINT('Ctrl Pts',(-0.0137898083069323,-0.0319656961064391,
-0.0130227816064802));
#22095=CARTESIAN_POINT('Ctrl Pts',(-0.0137861534562582,-0.0319660355748878,
-0.0130283216659042));
#22096=CARTESIAN_POINT('Ctrl Pts',(-0.0137737921095495,-0.0319671652006882,
-0.0130467986470862));
#22097=CARTESIAN_POINT('Ctrl Pts',(-0.013764925022248,-0.0319679452898744,
-0.0130596275126013));
#22098=CARTESIAN_POINT('Ctrl Pts',(-0.0137427744656077,-0.0319698274324029,
-0.0130906583301425));
#22099=CARTESIAN_POINT('Ctrl Pts',(-0.0137292836388706,-0.031970918139689,
-0.0131087082895254));
#22100=CARTESIAN_POINT('Ctrl Pts',(-0.0136708955153006,-0.031975440632618,
-0.0131833608826115));
#22101=CARTESIAN_POINT('Ctrl Pts',(-0.0136224453854206,-0.0319787263198167,
-0.0132370721023809));
#22102=CARTESIAN_POINT('Ctrl Pts',(-0.0134992967630453,-0.0319865425461815,
-0.0133556850161962));
#22103=CARTESIAN_POINT('Ctrl Pts',(-0.0134217799183298,-0.0319910816732149,
-0.0134171898733728));
#22104=CARTESIAN_POINT('Ctrl Pts',(-0.0133206694192779,-0.0319969898729515,
-0.0134826906383517));
#22105=CARTESIAN_POINT('Ctrl Pts',(-0.0133021657511994,-0.0319980696954103,
-0.0134941295127196));
#22106=CARTESIAN_POINT('Ctrl Pts',(-0.0132741667858537,-0.0319997045317629,
-0.0135106305426203));
#22107=CARTESIAN_POINT('Ctrl Pts',(-0.0132648499467091,-0.0320002486689731,
-0.0135159909985312));
#22108=CARTESIAN_POINT('Ctrl Pts',(-0.0132480023222733,-0.0320012331992971,
-0.0135254513872195));
#22109=CARTESIAN_POINT('Ctrl Pts',(-0.0132404918790416,-0.0320016722887083,
-0.0135295867465001));
#22110=CARTESIAN_POINT('Ctrl Pts',(-0.0132243723881314,-0.0320026152795823,
-0.0135382880928566));
#22111=CARTESIAN_POINT('Ctrl Pts',(-0.013215753795921,-0.0320031198192404,
-0.0135428355307223));
#22112=CARTESIAN_POINT('Ctrl Pts',(-0.0131921329600889,-0.0320045037901023,
-0.013555013993079));
#22113=CARTESIAN_POINT('Ctrl Pts',(-0.0131770483068297,-0.0320053889219412,
-0.0135624815167361));
#22114=CARTESIAN_POINT('Ctrl Pts',(-0.013078484710178,-0.032011182453819,
-0.0136092827796161));
#22115=CARTESIAN_POINT('Ctrl Pts',(-0.0129917537958947,-0.032016343456613,
-0.0136413015193974));
#22116=CARTESIAN_POINT('Ctrl Pts',(-0.0128127401473149,-0.0320269541029228,
-0.0136896979822628));
#22117=CARTESIAN_POINT('Ctrl Pts',(-0.0127207672858566,-0.0320323822922919,
-0.0137058188526549));
#22118=CARTESIAN_POINT('Ctrl Pts',(-0.0126001934017919,-0.0320391054182371,
-0.0137158478645137));
#22119=CARTESIAN_POINT('Ctrl Pts',(-0.0125724269560706,-0.0320406258176822,
-0.0137174033299859));
#22120=CARTESIAN_POINT('Ctrl Pts',(-0.0125361078259006,-0.0320425652275291,
-0.0137184543202629));
#22121=CARTESIAN_POINT('Ctrl Pts',(-0.0125275814496023,-0.0320430169774265,
-0.0137186303263275));
#22122=CARTESIAN_POINT('Ctrl Pts',(-0.0125138114984911,-0.0320437403275864,
-0.013718800378684));
#22123=CARTESIAN_POINT('Ctrl Pts',(-0.0125085687592662,-0.0320440142790308,
-0.0137188384013834));
#22124=CARTESIAN_POINT('Ctrl Pts',(-0.0124983601186337,-0.0320445447452104,
-0.0137188604055981));
#22125=CARTESIAN_POINT('Ctrl Pts',(-0.0124933943547235,-0.0320448013974494,
-0.0137188471376502));
#22126=CARTESIAN_POINT('Ctrl Pts',(-0.0124812066377706,-0.0320454280943007,
-0.013718755736726));
#22127=CARTESIAN_POINT('Ctrl Pts',(-0.0124739849020089,-0.0320457966692349,
-0.0137186508688197));
#22128=CARTESIAN_POINT('Ctrl Pts',(-0.0124473971903043,-0.032047144279301,
-0.0137180780409634));
#22129=CARTESIAN_POINT('Ctrl Pts',(-0.0124280390797191,-0.032048107201025,
-0.0137172960974338));
#22130=CARTESIAN_POINT('Ctrl Pts',(-0.0123783766262372,-0.0320505420554229,
-0.0137143523908195));
#22131=CARTESIAN_POINT('Ctrl Pts',(-0.0123481114512134,-0.0320519919471633,
-0.0137116598435217));
#22132=CARTESIAN_POINT('Ctrl Pts',(-0.0122505129668877,-0.0320566112387483,
-0.0137000633715691));
#22133=CARTESIAN_POINT('Ctrl Pts',(-0.0121836818544641,-0.0320596898314799,
-0.0136876084454355));
#22134=CARTESIAN_POINT('Ctrl Pts',(-0.0120229158364813,-0.0320672850412203,
-0.0136465158741246));
#22135=CARTESIAN_POINT('Ctrl Pts',(-0.011930484834166,-0.0320718285865343,
-0.0136132494119354));
#22136=CARTESIAN_POINT('Ctrl Pts',(-0.0118266446090333,-0.0320775108559329,
-0.013564278175693));
#22137=CARTESIAN_POINT('Ctrl Pts',(-0.0118115702840447,-0.0320783502771295,
-0.0135568658330794));
#22138=CARTESIAN_POINT('Ctrl Pts',(-0.0117878682210418,-0.032079694691472,
-0.01354472655373));
#22139=CARTESIAN_POINT('Ctrl Pts',(-0.011779159296538,-0.0320801940215883,
-0.0135401605710662));
#22140=CARTESIAN_POINT('Ctrl Pts',(-0.0117629486601084,-0.0320811337671448,
-0.0135314629862703));
#22141=CARTESIAN_POINT('Ctrl Pts',(-0.0117554365231385,-0.0320815734499467,
-0.013527351551659));
#22142=CARTESIAN_POINT('Ctrl Pts',(-0.0117386846254669,-0.0320825635364429,
-0.0135180010858926));
#22143=CARTESIAN_POINT('Ctrl Pts',(-0.0117294640141239,-0.0320831151282,
-0.0135127287862278));
#22144=CARTESIAN_POINT('Ctrl Pts',(-0.0117020938763298,-0.0320847726599055,
-0.0134967014523874));
#22145=CARTESIAN_POINT('Ctrl Pts',(-0.0116841102276577,-0.0320858886394198,
-0.0134856692580569));
#22146=CARTESIAN_POINT('Ctrl Pts',(-0.0115995562540498,-0.03209126703914,
-0.0134313819550415));
#22147=CARTESIAN_POINT('Ctrl Pts',(-0.0115361712344603,-0.0320957034469407,
-0.0133834055945569));
#22148=CARTESIAN_POINT('Ctrl Pts',(-0.0114138978568064,-0.032105029388017,
-0.0132750737526457));
#22149=CARTESIAN_POINT('Ctrl Pts',(-0.0113556848857642,-0.0321099147532679,
-0.0132143360332975));
#22150=CARTESIAN_POINT('Ctrl Pts',(-0.0112771204596531,-0.0321169374722964,
-0.0131176916970582));
#22151=CARTESIAN_POINT('Ctrl Pts',(-0.0112527855390189,-0.0321191850388395,
-0.0130852214994991));
#22152=CARTESIAN_POINT('Ctrl Pts',(-0.0112242949873362,-0.0321218733759114,
-0.0130439075950904));
#22153=CARTESIAN_POINT('Ctrl Pts',(-0.0112189071713629,-0.0321223844833262,
-0.0130359362683328));
#22154=CARTESIAN_POINT('Ctrl Pts',(-0.0112105667440473,-0.03212317933925,
-0.0130233442506023));
#22155=CARTESIAN_POINT('Ctrl Pts',(-0.011207563687886,-0.0321234663013213,
-0.0130187574546923));
#22156=CARTESIAN_POINT('Ctrl Pts',(-0.011201940978569,-0.0321240048945783,
-0.0130100687640944));
#22157=CARTESIAN_POINT('Ctrl Pts',(-0.0111993162298553,-0.0321242568476558,
-0.0130059703966385));
#22158=CARTESIAN_POINT('Ctrl Pts',(-0.0111931584837095,-0.0321248493176249,
-0.0129962545830056));
#22159=CARTESIAN_POINT('Ctrl Pts',(-0.0111896422235246,-0.0321251887418385,
-0.0129906265904009));
#22160=CARTESIAN_POINT('Ctrl Pts',(-0.0111779880860844,-0.0321263180594005,
-0.0129717028290849));
#22161=CARTESIAN_POINT('Ctrl Pts',(-0.0111700151646058,-0.0321270978920825,
-0.0129583060759418));
#22162=CARTESIAN_POINT('Ctrl Pts',(-0.0111510234573555,-0.0321289792913082,
-0.0129252653659614));
#22163=CARTESIAN_POINT('Ctrl Pts',(-0.0111402289115818,-0.0321300695235784,
-0.0129054962441676));
#22164=CARTESIAN_POINT('Ctrl Pts',(-0.011096674195217,-0.0321345886825178,
-0.0128214039259133));
#22165=CARTESIAN_POINT('Ctrl Pts',(-0.0110680141644286,-0.0321378717271535,
-0.0127550567583075));
#22166=CARTESIAN_POINT('Ctrl Pts',(-0.0110113731883091,-0.032145688809762,
-0.0125937088234088));
#22167=CARTESIAN_POINT('Ctrl Pts',(-0.0109876766916429,-0.0321502314013961,
-0.0124975504302443));
#22168=CARTESIAN_POINT('Ctrl Pts',(-0.0109701803805182,-0.0321561435539088,
-0.0123782737419149));
#22169=CARTESIAN_POINT('Ctrl Pts',(-0.0109674790815342,-0.0321572233199449,
-0.012356689357217));
#22170=CARTESIAN_POINT('Ctrl Pts',(-0.0109641260040787,-0.0321588580874549,
-0.0123243645636871));
#22171=CARTESIAN_POINT('Ctrl Pts',(-0.0109631287621924,-0.0321594022136373,
-0.0123136622906007));
#22172=CARTESIAN_POINT('Ctrl Pts',(-0.0109615372199236,-0.0321603867320347,
-0.0122944061499693));
#22173=CARTESIAN_POINT('Ctrl Pts',(-0.0109609022454603,-0.0321608258206849,
-0.0122858560371255));
#22174=CARTESIAN_POINT('Ctrl Pts',(-0.0109596978758653,-0.0321617688187711,
-0.0122675774786374));
#22175=CARTESIAN_POINT('Ctrl Pts',(-0.010959149322553,-0.0321622733665018,
-0.0122578480728074));
#22176=CARTESIAN_POINT('Ctrl Pts',(-0.0109579047110446,-0.0321636573826688,
-0.0122313008497113));
#22177=CARTESIAN_POINT('Ctrl Pts',(-0.0109573916382353,-0.0321645425523657,
-0.0122144761339798));
#22178=CARTESIAN_POINT('Ctrl Pts',(-0.0109558501300154,-0.0321703376501135,
-0.0121053470060591));
#22179=CARTESIAN_POINT('Ctrl Pts',(-0.0109628316203562,-0.0321755003490587,
-0.0120131296779549));
#22180=CARTESIAN_POINT('Ctrl Pts',(-0.0109933409255827,-0.0321861156027621,
-0.0118301368019082));
#22181=CARTESIAN_POINT('Ctrl Pts',(-0.0110169770976427,-0.0321915467249982,
-0.0117397510100458));
#22182=CARTESIAN_POINT('Ctrl Pts',(-0.0110580443883101,-0.0321982683749375,
-0.0116259602098475));
#22183=CARTESIAN_POINT('Ctrl Pts',(-0.0110681629142342,-0.0321997850792603,
-0.0116001266821526));
#22184=CARTESIAN_POINT('Ctrl Pts',(-0.0110822933137908,-0.0322017205603752,
-0.0115667314981259));
#22185=CARTESIAN_POINT('Ctrl Pts',(-0.0110856786444253,-0.0322021719189494,
-0.0115589118704271));
#22186=CARTESIAN_POINT('Ctrl Pts',(-0.0110912507092514,-0.0322028947967239,
-0.0115463281434806));
#22187=CARTESIAN_POINT('Ctrl Pts',(-0.0110933972028274,-0.0322031686617601,
-0.0115415465448679));
#22188=CARTESIAN_POINT('Ctrl Pts',(-0.0110976251436653,-0.0322036990882563,
-0.0115322552518551));
#22189=CARTESIAN_POINT('Ctrl Pts',(-0.0110997040558569,-0.0322039557858975,
-0.0115277445478319));
#22190=CARTESIAN_POINT('Ctrl Pts',(-0.0111048614540886,-0.0322045827758229,
-0.0115166949823676));
#22191=CARTESIAN_POINT('Ctrl Pts',(-0.0111079642141444,-0.0322049515951886,
-0.0115101674694237));
#22192=CARTESIAN_POINT('Ctrl Pts',(-0.0111195667612765,-0.0322063011771879,
-0.0114861941946474));
#22193=CARTESIAN_POINT('Ctrl Pts',(-0.0111283498874238,-0.0322072657648647,
-0.0114688867928833));
#22194=CARTESIAN_POINT('Ctrl Pts',(-0.0111517487311405,-0.0322097058792018,
-0.0114248573387118));
#22195=CARTESIAN_POINT('Ctrl Pts',(-0.0111668335932105,-0.0322111592442367,
-0.0113983933818991));
#22196=CARTESIAN_POINT('Ctrl Pts',(-0.011218245431407,-0.032215799021166,
-0.0113141015688734));
#22197=CARTESIAN_POINT('Ctrl Pts',(-0.0112576293993007,-0.0322188937404567,
-0.0112582331258105));
#22198=CARTESIAN_POINT('Ctrl Pts',(-0.0113569037998826,-0.0322261176008592,
-0.0111355676082758));
#22199=CARTESIAN_POINT('Ctrl Pts',(-0.0114191674707024,-0.0322302625613331,
-0.0110710174130741));
#22200=CARTESIAN_POINT('Ctrl Pts',(-0.0115030776349032,-0.0322357192888351,
-0.010997944910605));
#22201=CARTESIAN_POINT('Ctrl Pts',(-0.0115197846167669,-0.0322367993157329,
-0.0109840059441173));
#22202=CARTESIAN_POINT('Ctrl Pts',(-0.0115451780432855,-0.0322384344015361,
-0.0109637148521648));
#22203=CARTESIAN_POINT('Ctrl Pts',(-0.0115536456085968,-0.0322389785787183,
-0.0109570924767839));
#22204=CARTESIAN_POINT('Ctrl Pts',(-0.0115689899199205,-0.032239963152296,
-0.0109453482116252));
#22205=CARTESIAN_POINT('Ctrl Pts',(-0.0115758415173753,-0.0322404022444899,
-0.0109401941087521));
#22206=CARTESIAN_POINT('Ctrl Pts',(-0.0115905710423415,-0.0322413452093064,
-0.0109293048845732));
#22207=CARTESIAN_POINT('Ctrl Pts',(-0.0115984610302843,-0.0322418497197641,
-0.010923586770301));
#22208=CARTESIAN_POINT('Ctrl Pts',(-0.0116201238511323,-0.0322432335266724,
-0.0109081979051512));
#22209=CARTESIAN_POINT('Ctrl Pts',(-0.0116340013053723,-0.032244118521495,
-0.0108986773261174));
#22210=CARTESIAN_POINT('Ctrl Pts',(-0.0117248834550524,-0.0322499064025573,
-0.0108384902259258));
#22211=CARTESIAN_POINT('Ctrl Pts',(-0.0118061304776674,-0.0322550612853422,
-0.0107945906897392));
#22212=CARTESIAN_POINT('Ctrl Pts',(-0.0119762458062526,-0.0322656553284739,
-0.0107214873447004));
#22213=CARTESIAN_POINT('Ctrl Pts',(-0.01206483966933,-0.0322710729570748,
-0.0106925681206186));
#22214=CARTESIAN_POINT('Ctrl Pts',(-0.0121828310401409,-0.0322778014209382,
-0.0106655423719038));
#22215=CARTESIAN_POINT('Ctrl Pts',(-0.0122103299047898,-0.0322793351559365,
-0.0106600278907194));
#22216=CARTESIAN_POINT('Ctrl Pts',(-0.0122463948042114,-0.0322812887332433,
-0.0106538130206249));
#22217=CARTESIAN_POINT('Ctrl Pts',(-0.0122548364234306,-0.0322817418870856,
-0.0106524304976524));
#22218=CARTESIAN_POINT('Ctrl Pts',(-0.0122684756223713,-0.0322824669319866,
-0.0106503130514614));
#22219=CARTESIAN_POINT('Ctrl Pts',(-0.0122736661062311,-0.0322827411934426,
-0.0106495343433195));
#22220=CARTESIAN_POINT('Ctrl Pts',(-0.0122837717217313,-0.0322832718039773,
-0.0106480709207708));
#22221=CARTESIAN_POINT('Ctrl Pts',(-0.0122886863140448,-0.0322835282952914,
-0.01064738341375));
#22222=CARTESIAN_POINT('Ctrl Pts',(-0.0123007441942925,-0.0322841539498816,
-0.0106457558933926));
#22223=CARTESIAN_POINT('Ctrl Pts',(-0.0123078910134248,-0.0322845216549992,
-0.0106448421664524));
#22224=CARTESIAN_POINT('Ctrl Pts',(-0.0123341540218158,-0.0322858622687672,
-0.0106416712165045));
#22225=CARTESIAN_POINT('Ctrl Pts',(-0.0123533062680993,-0.0322868192813766,
-0.0106397216108868));
#22226=CARTESIAN_POINT('Ctrl Pts',(-0.0124024935538336,-0.0322892355134744,
-0.010635642960321));
#22227=CARTESIAN_POINT('Ctrl Pts',(-0.0124325641655228,-0.0322906731164171,
-0.0106340336040558));
#22228=CARTESIAN_POINT('Ctrl Pts',(-0.0125292533641203,-0.0322952207938548,
-0.0106316933225697));
#22229=CARTESIAN_POINT('Ctrl Pts',(-0.0125958796663092,-0.0322982431290773,
-0.0106343950511176));
#22230=CARTESIAN_POINT('Ctrl Pts',(-0.0127612711648686,-0.0323058529334065,
-0.0106518696511979));
#22231=CARTESIAN_POINT('Ctrl Pts',(-0.0128591577506311,-0.0323104675815919,
-0.0106719278231339));
#22232=CARTESIAN_POINT('Ctrl Pts',(-0.0129705046211916,-0.0323162338886589,
-0.0107062418997138));
#22233=CARTESIAN_POINT('Ctrl Pts',(-0.0129865049967269,-0.0323170748592469,
-0.0107114608913793));
#22234=CARTESIAN_POINT('Ctrl Pts',(-0.0130117205299129,-0.0323184212001292,
-0.0107201445478324));
#22235=CARTESIAN_POINT('Ctrl Pts',(-0.0130209936233605,-0.0323189208791938,
-0.0107234375501757));
#22236=CARTESIAN_POINT('Ctrl Pts',(-0.013038275914345,-0.0323198609326567,
-0.0107297615315659));
#22237=CARTESIAN_POINT('Ctrl Pts',(-0.013046292635808,-0.0323203005697546,
-0.0107327709341124));
#22238=CARTESIAN_POINT('Ctrl Pts',(-0.0130641871037121,-0.0323212900913802,
-0.0107396588294172));
#22239=CARTESIAN_POINT('Ctrl Pts',(-0.0130740506592899,-0.0323218411579902,
-0.010743572783411));
#22240=CARTESIAN_POINT('Ctrl Pts',(-0.0131033543346783,-0.0323234955058182,
-0.0107555520867022));
#22241=CARTESIAN_POINT('Ctrl Pts',(-0.0131226700925024,-0.0323246087694194,
-0.0107639135398794));
#22242=CARTESIAN_POINT('Ctrl Pts',(-0.0132136337266458,-0.0323299624000507,
-0.0108055197128482));
#22243=CARTESIAN_POINT('Ctrl Pts',(-0.0132828221127666,-0.0323343748988194,
-0.0108438344934591));
#22244=CARTESIAN_POINT('Ctrl Pts',(-0.0134181972058184,-0.0323436271259771,
-0.0109330037934953));
#22245=CARTESIAN_POINT('Ctrl Pts',(-0.0134838165852728,-0.0323484619563676,
-0.0109842720454189));
#22246=CARTESIAN_POINT('Ctrl Pts',(-0.0135757289940174,-0.0323555134702802,
-0.0110688745059318));
#22247=CARTESIAN_POINT('Ctrl Pts',(-0.0136053122046139,-0.0323578315518118,
-0.011098411707659));
#22248=CARTESIAN_POINT('Ctrl Pts',(-0.013640153666218,-0.0323605833376665,
-0.0111361465028885));
#22249=CARTESIAN_POINT('Ctrl Pts',(-0.0136465801365082,-0.0323610918480808,
-0.0111432378798205));
#22250=CARTESIAN_POINT('Ctrl Pts',(-0.01365661317641,-0.0323618865789594,
-0.011154518130326));
#22251=CARTESIAN_POINT('Ctrl Pts',(-0.0136602638261778,-0.0323621759315623,
-0.0111586672678074));
#22252=CARTESIAN_POINT('Ctrl Pts',(-0.0136670800446404,-0.0323627163734295,
-0.0111664986674117));
#22253=CARTESIAN_POINT('Ctrl Pts',(-0.0136702505251697,-0.032362967811008,
-0.0111701762576503));
#22254=CARTESIAN_POINT('Ctrl Pts',(-0.0136776591715056,-0.0323635556007237,
-0.0111788523739204));
#22255=CARTESIAN_POINT('Ctrl Pts',(-0.0136818829145273,-0.0323638909071585,
-0.0111838630026428));
#22256=CARTESIAN_POINT('Ctrl Pts',(-0.0136957348818779,-0.0323649918051742,
-0.0112005096625076));
#22257=CARTESIAN_POINT('Ctrl Pts',(-0.0137052244605922,-0.0323657480149955,
-0.011212260465689));
#22258=CARTESIAN_POINT('Ctrl Pts',(-0.0137278523818071,-0.0323675613209275,
-0.0112411376347031));
#22259=CARTESIAN_POINT('Ctrl Pts',(-0.0137408070774015,-0.0323686081332972,
-0.0112584042739884));
#22260=CARTESIAN_POINT('Ctrl Pts',(-0.0137923220884857,-0.0323728321358293,
-0.0113301539952048));
#22261=CARTESIAN_POINT('Ctrl Pts',(-0.0138276919353843,-0.0323758820507518,
-0.0113868420124714));
#22262=CARTESIAN_POINT('Ctrl Pts',(-0.0139095396231259,-0.032383787597368,
-0.0115392012996929));
#22263=CARTESIAN_POINT('Ctrl Pts',(-0.0139500007379712,-0.032388642164868,
-0.0116376867040619));
#22264=CARTESIAN_POINT('Ctrl Pts',(-0.0139860484821259,-0.0323948962800243,
-0.0117599659943611));
#22265=CARTESIAN_POINT('Ctrl Pts',(-0.0139916454875632,-0.0323959533441385,
-0.0117805103782178));
#22266=CARTESIAN_POINT('Ctrl Pts',(-0.0139994382659481,-0.0323975673383834,
-0.011811641058401));
#22267=CARTESIAN_POINT('Ctrl Pts',(-0.0140019509509674,-0.0323981140334458,
-0.0118221457891512));
#22268=CARTESIAN_POINT('Ctrl Pts',(-0.0140062609982421,-0.0323991013395911,
-0.0118410393193961));
#22269=CARTESIAN_POINT('Ctrl Pts',(-0.0140080990893304,-0.0323995406150394,
-0.0118494184228482));
#22270=CARTESIAN_POINT('Ctrl Pts',(-0.0140118687026241,-0.0324004819773254,
-0.0118673142784492));
#22271=CARTESIAN_POINT('Ctrl Pts',(-0.0140137804400154,-0.0324009846796224,
-0.011876834780237));
#22272=CARTESIAN_POINT('Ctrl Pts',(-0.0140187298901506,-0.0324023583439381,
-0.0119027480668268));
#22273=CARTESIAN_POINT('Ctrl Pts',(-0.0140215919319507,-0.0324032348650724,
-0.0119191727391614));
#22274=CARTESIAN_POINT('Ctrl Pts',(-0.014036712830561,-0.0324083904766337,
-0.0120151170314925));
#22275=CARTESIAN_POINT('Ctrl Pts',(-0.0140430000005061,-0.0324128571794188,
-0.0120954324537772));
#22276=CARTESIAN_POINT('Ctrl Pts',(-0.014043,-0.0324174341340783,-0.0121758532962676));
#22277=CARTESIAN_POINT('Origin',(-0.0125,-0.0375520664398416,-0.0121758532865581));
#22278=CARTESIAN_POINT('',(-0.014043,-0.0329194567307744,-0.012175853286558));
#22279=CARTESIAN_POINT('',(-0.014043,-0.0328035263970765,-0.012175853286558));
#22280=CARTESIAN_POINT('',(-0.014043,-0.0375520664398416,-0.012175853286558));
#22281=CARTESIAN_POINT('',(-0.0140429999983096,-0.0328035227368026,-0.0121757810608236));
#22282=CARTESIAN_POINT('Ctrl Pts',(-0.014043,-0.0328035263970765,-0.012175853286558));
#22283=CARTESIAN_POINT('Ctrl Pts',(-0.014043,-0.0328035250082943,-0.0121758258822526));
#22284=CARTESIAN_POINT('Ctrl Pts',(-0.0140429999992699,-0.0328035236194892,
-0.0121757984779469));
#22285=CARTESIAN_POINT('Ctrl Pts',(-0.0140429999978098,-0.0328035222306614,
-0.0121757710736408));
#22286=CARTESIAN_POINT('Ctrl Pts',(-0.0140429999983096,-0.0328035227368026,
-0.0121757810608236));
#22287=CARTESIAN_POINT('Ctrl Pts',(-0.0140429997244644,-0.032803226248909,
-0.0121699307479627));
#22288=CARTESIAN_POINT('Ctrl Pts',(-0.0140429662544466,-0.0328029292367222,
-0.0121640905248185));
#22289=CARTESIAN_POINT('Ctrl Pts',(-0.0140428326113774,-0.0328023317104684,
-0.0121523831128644));
#22290=CARTESIAN_POINT('Ctrl Pts',(-0.0140427323894257,-0.0328020317059399,
-0.0121465260101399));
#22291=CARTESIAN_POINT('Ctrl Pts',(-0.0140423926184721,-0.0328012658944575,
-0.0121316290106755));
#22292=CARTESIAN_POINT('Ctrl Pts',(-0.0140421069495067,-0.0328007986457035,
-0.0121225904693319));
#22293=CARTESIAN_POINT('Ctrl Pts',(-0.0140411769421325,-0.0327996020335943,
-0.0120995748553997));
#22294=CARTESIAN_POINT('Ctrl Pts',(-0.0140404219178594,-0.0327988692188615,
-0.0120856032807187));
#22295=CARTESIAN_POINT('Ctrl Pts',(-0.014036550875133,-0.0327958427418227,
-0.0120284165045126));
#22296=CARTESIAN_POINT('Ctrl Pts',(-0.0140318055634194,-0.0327934986844895,
-0.0119853344806585));
#22297=CARTESIAN_POINT('Ctrl Pts',(-0.0140199972636875,-0.0327891861370116,
-0.0119081486292883));
#22298=CARTESIAN_POINT('Ctrl Pts',(-0.0140135806720148,-0.0327872363642042,
-0.011873974482153));
#22299=CARTESIAN_POINT('Ctrl Pts',(-0.0139837811262394,-0.0327794733027683,
-0.0117403299865484));
#22300=CARTESIAN_POINT('Ctrl Pts',(-0.0139516989191298,-0.0327734991223908,
-0.0116430715414537));
#22301=CARTESIAN_POINT('Ctrl Pts',(-0.0139001588968634,-0.0327663675661505,
-0.0115269917098509));
#22302=CARTESIAN_POINT('Ctrl Pts',(-0.013889529205442,-0.0327649887308705,
-0.0115045299815642));
#22303=CARTESIAN_POINT('Ctrl Pts',(-0.0138708348424866,-0.0327627213181017,
-0.0114673751691735));
#22304=CARTESIAN_POINT('Ctrl Pts',(-0.013863065111816,-0.0327618196361788,
-0.0114525394169333));
#22305=CARTESIAN_POINT('Ctrl Pts',(-0.0138517984869085,-0.0327605707356656,
-0.0114318531459254));
#22306=CARTESIAN_POINT('Ctrl Pts',(-0.0138485022640765,-0.0327602120316526,
-0.0114258952839585));
#22307=CARTESIAN_POINT('Ctrl Pts',(-0.0138427778257623,-0.0327596006749833,
-0.011415708241936));
#22308=CARTESIAN_POINT('Ctrl Pts',(-0.0138403688191471,-0.0327593468267121,
-0.0114114684297682));
#22309=CARTESIAN_POINT('Ctrl Pts',(-0.0138352689187748,-0.0327588166531116,
-0.0114025909371715));
#22310=CARTESIAN_POINT('Ctrl Pts',(-0.0138325739117848,-0.0327585405927337,
-0.0113979557883235));
#22311=CARTESIAN_POINT('Ctrl Pts',(-0.0138252227961144,-0.0327577983336406,
-0.0113854629012682));
#22312=CARTESIAN_POINT('Ctrl Pts',(-0.0138205209230791,-0.0327573350055703,
-0.0113776321894092));
#22313=CARTESIAN_POINT('Ctrl Pts',(-0.013797749268969,-0.0327551425741716,
-0.0113404591951907));
#22314=CARTESIAN_POINT('Ctrl Pts',(-0.0137787683345102,-0.0327534664295224,
-0.0113116841417433));
#22315=CARTESIAN_POINT('Ctrl Pts',(-0.013707724800304,-0.0327476163614296,
-0.0112114558279984));
#22316=CARTESIAN_POINT('Ctrl Pts',(-0.0136505067409734,-0.0327436410706501,
-0.0111438660428199));
#22317=CARTESIAN_POINT('Ctrl Pts',(-0.0135243824325406,-0.0327354796503313,
-0.0110184903610312));
#22318=CARTESIAN_POINT('Ctrl Pts',(-0.0134555945387388,-0.0327313036492548,
-0.0109610754836151));
#22319=CARTESIAN_POINT('Ctrl Pts',(-0.0133685166019989,-0.0327260473694893,
-0.0109003897604941));
#22320=CARTESIAN_POINT('Ctrl Pts',(-0.0133546516847554,-0.0327252117478388,
-0.0108910580637586));
#22321=CARTESIAN_POINT('Ctrl Pts',(-0.0133325099890432,-0.0327238780371024,
-0.0108766727468868));
#22322=CARTESIAN_POINT('Ctrl Pts',(-0.0133243322634616,-0.0327233856101872,
-0.010871468653743));
#22323=CARTESIAN_POINT('Ctrl Pts',(-0.0133088603065355,-0.0327224540197819,
-0.0108618263086129));
#22324=CARTESIAN_POINT('Ctrl Pts',(-0.0133015771911879,-0.032722015518471,
-0.0108573708646372));
#22325=CARTESIAN_POINT('Ctrl Pts',(-0.0132850706713883,-0.0327210215969352,
-0.0108474603234615));
#22326=CARTESIAN_POINT('Ctrl Pts',(-0.0132758267262926,-0.0327204649138006,
-0.0108420404412043));
#22327=CARTESIAN_POINT('Ctrl Pts',(-0.0132476748534127,-0.0327187690472513,
-0.0108259261865134));
#22328=CARTESIAN_POINT('Ctrl Pts',(-0.0132285973984482,-0.0327176190776858,
-0.010815534710689));
#22329=CARTESIAN_POINT('Ctrl Pts',(-0.0131303402214902,-0.0327116905567254,
-0.0107646740380959));
#22330=CARTESIAN_POINT('Ctrl Pts',(-0.0130479976322164,-0.0327066898361415,
-0.0107307060445875));
#22331=CARTESIAN_POINT('Ctrl Pts',(-0.0128868339071897,-0.032697006236147,
-0.0106799863916181));
#22332=CARTESIAN_POINT('Ctrl Pts',(-0.0128087131819163,-0.0326923591923312,
-0.0106619329192578));
#22333=CARTESIAN_POINT('Ctrl Pts',(-0.0127060641022901,-0.0326865408525819,
-0.0106464905632975));
#22334=CARTESIAN_POINT('Ctrl Pts',(-0.0126825053440603,-0.0326852253882661,
-0.0106435006341352));
#22335=CARTESIAN_POINT('Ctrl Pts',(-0.0126427753067765,-0.032683050396092,
-0.010639387683986));
#22336=CARTESIAN_POINT('Ctrl Pts',(-0.0126266387098334,-0.0326821790053556,
-0.0106379735727623));
#22337=CARTESIAN_POINT('Ctrl Pts',(-0.0126037793719043,-0.0326809643850252,
-0.0106363325813264));
#22338=CARTESIAN_POINT('Ctrl Pts',(-0.0125970733164945,-0.0326806104690602,
-0.0106358951915498));
#22339=CARTESIAN_POINT('Ctrl Pts',(-0.012585510544212,-0.0326800046388432,
-0.0106352168632663));
#22340=CARTESIAN_POINT('Ctrl Pts',(-0.012580655196328,-0.0326797515851657,
-0.0106349550473385));
#22341=CARTESIAN_POINT('Ctrl Pts',(-0.0125704036744945,-0.032679220204491,
-0.0106344508415677));
#22342=CARTESIAN_POINT('Ctrl Pts',(-0.0125650073885619,-0.0326789421729556,
-0.0106342138293644));
#22343=CARTESIAN_POINT('Ctrl Pts',(-0.0125503014755309,-0.0326781887991145,
-0.0106336452793051));
#22344=CARTESIAN_POINT('Ctrl Pts',(-0.0125409897741537,-0.0326777164765595,
-0.0106333696974533));
#22345=CARTESIAN_POINT('Ctrl Pts',(-0.0124951126938798,-0.0326754101701503,
-0.0106324276977446));
#22346=CARTESIAN_POINT('Ctrl Pts',(-0.0124585317443909,-0.032673635977473,
-0.0106329770171757));
#22347=CARTESIAN_POINT('Ctrl Pts',(-0.0123352407819245,-0.0326677753268966,
-0.010639217255425));
#22348=CARTESIAN_POINT('Ctrl Pts',(-0.0122490006785074,-0.0326638676144234,
-0.010650928101743));
#22349=CARTESIAN_POINT('Ctrl Pts',(-0.0120777731806125,-0.0326558138624723,
-0.0106891069510247));
#22350=CARTESIAN_POINT('Ctrl Pts',(-0.0119931714857072,-0.0326516763249778,
-0.010715780421183));
#22351=CARTESIAN_POINT('Ctrl Pts',(-0.0118959055696372,-0.0326464650123408,
-0.0107559246356871));
#22352=CARTESIAN_POINT('Ctrl Pts',(-0.0118805854294431,-0.0326456306145429,
-0.0107625405056147));
#22353=CARTESIAN_POINT('Ctrl Pts',(-0.0118565455573148,-0.0326442984126594,
-0.0107733878743638));
#22354=CARTESIAN_POINT('Ctrl Pts',(-0.0118477530101154,-0.0326438062484429,
-0.0107774553779504));
#22355=CARTESIAN_POINT('Ctrl Pts',(-0.0118312840929762,-0.032642874878877,
-0.0107852631448178));
#22356=CARTESIAN_POINT('Ctrl Pts',(-0.0118235993105306,-0.0326424363321358,
-0.0107889848681468));
#22357=CARTESIAN_POINT('Ctrl Pts',(-0.011806333575241,-0.0326414419318973,
-0.010797524265604));
#22358=CARTESIAN_POINT('Ctrl Pts',(-0.0117967712285257,-0.0326408848105252,
-0.0108023783920016));
#22359=CARTESIAN_POINT('Ctrl Pts',(-0.0117679565917114,-0.0326391862427176,
-0.0108173853401912));
#22360=CARTESIAN_POINT('Ctrl Pts',(-0.0117488683643744,-0.0326380339597172,
-0.0108278459002554));
#22361=CARTESIAN_POINT('Ctrl Pts',(-0.0116527594557584,-0.0326320908328485,
-0.0108831898943557));
#22362=CARTESIAN_POINT('Ctrl Pts',(-0.0115795205881838,-0.0326270766925603,
-0.0109342780358299));
#22363=CARTESIAN_POINT('Ctrl Pts',(-0.0114498302371968,-0.0326173926887576,
-0.0110425550282222));
#22364=CARTESIAN_POINT('Ctrl Pts',(-0.0113926136139859,-0.0326127594332519,
-0.0110983945447478));
#22365=CARTESIAN_POINT('Ctrl Pts',(-0.0113243403033009,-0.0326069562425437,
-0.0111762356619507));
#22366=CARTESIAN_POINT('Ctrl Pts',(-0.011309118951816,-0.0326056427589277,
-0.0111944188541949));
#22367=CARTESIAN_POINT('Ctrl Pts',(-0.0112842253070289,-0.0326034706658091,
-0.0112255887597121));
#22368=CARTESIAN_POINT('Ctrl Pts',(-0.011274327606889,-0.0326026002313648,
-0.011238389686991));
#22369=CARTESIAN_POINT('Ctrl Pts',(-0.0112606079694354,-0.032601386695724,
-0.0112567224382293));
#22370=CARTESIAN_POINT('Ctrl Pts',(-0.0112566183136278,-0.0326010329329584,
-0.0112621267918926));
#22371=CARTESIAN_POINT('Ctrl Pts',(-0.0112498020408711,-0.0326004272789098,
-0.0112714873757067));
#22372=CARTESIAN_POINT('Ctrl Pts',(-0.0112469586225496,-0.0326001742499973,
-0.0112754311930397));
#22373=CARTESIAN_POINT('Ctrl Pts',(-0.011240994894217,-0.0325996428275759,
-0.0112837858380411));
#22374=CARTESIAN_POINT('Ctrl Pts',(-0.0112378790635814,-0.0325993647305307,
-0.0112881996758034));
#22375=CARTESIAN_POINT('Ctrl Pts',(-0.0112294507906448,-0.0325986109868777,
-0.0113002731385966));
#22376=CARTESIAN_POINT('Ctrl Pts',(-0.0112241843916177,-0.0325981383650359,
-0.0113079647968963));
#22377=CARTESIAN_POINT('Ctrl Pts',(-0.0111985554069844,-0.032595827662577,
-0.0113461337935123));
#22378=CARTESIAN_POINT('Ctrl Pts',(-0.0111792122399681,-0.0325940496495128,
-0.011377284237655));
#22379=CARTESIAN_POINT('Ctrl Pts',(-0.0111178553037901,-0.0325881885176848,
-0.011484433144876));
#22380=CARTESIAN_POINT('Ctrl Pts',(-0.0110811477855629,-0.0325842833984268,
-0.0115632802324847));
#22381=CARTESIAN_POINT('Ctrl Pts',(-0.0110208009578662,-0.0325762337584024,
-0.0117279086460154));
#22382=CARTESIAN_POINT('Ctrl Pts',(-0.0109975465615405,-0.0325720976757051,
-0.0118134782931668));
#22383=CARTESIAN_POINT('Ctrl Pts',(-0.0109787793125266,-0.0325668880632285,
-0.011916980649851));
#22384=CARTESIAN_POINT('Ctrl Pts',(-0.0109760689136149,-0.0325660537125726,
-0.0119334456987578));
#22385=CARTESIAN_POINT('Ctrl Pts',(-0.0109722078318142,-0.0325647215688092,
-0.0119595342189157));
#22386=CARTESIAN_POINT('Ctrl Pts',(-0.0109708798368436,-0.0325642294147125,
-0.0119691303579224));
#22387=CARTESIAN_POINT('Ctrl Pts',(-0.010968551528085,-0.032563298053641,
-0.0119872068316185));
#22388=CARTESIAN_POINT('Ctrl Pts',(-0.0109675310725281,-0.0325628595051369,
-0.0119956842284084));
#22389=CARTESIAN_POINT('Ctrl Pts',(-0.0109653878181927,-0.0325618650863954,
-0.0120148270245111));
#22390=CARTESIAN_POINT('Ctrl Pts',(-0.0109643057519314,-0.0325613079480914,
-0.0120254964635249));
#22391=CARTESIAN_POINT('Ctrl Pts',(-0.0109614296813406,-0.0325596468470826,
-0.0120571376949412));
#22392=CARTESIAN_POINT('Ctrl Pts',(-0.0109599535229632,-0.0325585329777989,
-0.0120781352913499));
#22393=CARTESIAN_POINT('Ctrl Pts',(-0.0109533742755317,-0.0325514455818761,
-0.0122103330444433));
#22394=CARTESIAN_POINT('Ctrl Pts',(-0.0109598889094037,-0.0325451049800559,
-0.0123217669462785));
#22395=CARTESIAN_POINT('Ctrl Pts',(-0.0109888058462719,-0.0325350650839862,
-0.0124938796035878));
#22396=CARTESIAN_POINT('Ctrl Pts',(-0.0110031091522276,-0.0325314247238606,
-0.0125555465236941));
#22397=CARTESIAN_POINT('Ctrl Pts',(-0.0110271277663615,-0.0325267303830084,
-0.0126362163418378));
#22398=CARTESIAN_POINT('Ctrl Pts',(-0.0110335057639658,-0.032525576563121,
-0.0126561464117112));
#22399=CARTESIAN_POINT('Ctrl Pts',(-0.0110450660151565,-0.0325236403323662,
-0.0126898897568675));
#22400=CARTESIAN_POINT('Ctrl Pts',(-0.0110500445025095,-0.0325228489765341,
-0.0127037694537943));
#22401=CARTESIAN_POINT('Ctrl Pts',(-0.0110574944376209,-0.0325217256783336,
-0.0127236384829956));
#22402=CARTESIAN_POINT('Ctrl Pts',(-0.0110598057005549,-0.0325213850348982,
-0.0127296865662819));
#22403=CARTESIAN_POINT('Ctrl Pts',(-0.0110639068894313,-0.0325207942907258,
-0.0127402192046221));
#22404=CARTESIAN_POINT('Ctrl Pts',(-0.0110656798977015,-0.0325205432059915,
-0.0127447101736816));
#22405=CARTESIAN_POINT('Ctrl Pts',(-0.0110695283732042,-0.0325200073844477,
-0.0127543258374588));
#22406=CARTESIAN_POINT('Ctrl Pts',(-0.0110716103251592,-0.0325197230366926,
-0.0127594477569554));
#22407=CARTESIAN_POINT('Ctrl Pts',(-0.0110773987902469,-0.0325189471285778,
-0.0127734717092702));
#22408=CARTESIAN_POINT('Ctrl Pts',(-0.0110811613476847,-0.0325184588253497,
-0.0127823504991152));
#22409=CARTESIAN_POINT('Ctrl Pts',(-0.0111023185562571,-0.0325157963382542,
-0.0128310021143866));
#22410=CARTESIAN_POINT('Ctrl Pts',(-0.011121303723076,-0.0325137071229543,
-0.0128700654705278));
#22411=CARTESIAN_POINT('Ctrl Pts',(-0.0111808480780025,-0.032507803420902,
-0.0129804745734806));
#22412=CARTESIAN_POINT('Ctrl Pts',(-0.0112254798547442,-0.0325041108284196,
-0.013049453122762));
#22413=CARTESIAN_POINT('Ctrl Pts',(-0.0113276439434469,-0.0324963929152494,
-0.0131827341911131));
#22414=CARTESIAN_POINT('Ctrl Pts',(-0.0113855001258628,-0.0324923704458758,
-0.0132464212615704));
#22415=CARTESIAN_POINT('Ctrl Pts',(-0.011460501472027,-0.0324872934748917,
-0.0133162775856155));
#22416=CARTESIAN_POINT('Ctrl Pts',(-0.011472834962371,-0.0324864629990781,
-0.0133273986525901));
#22417=CARTESIAN_POINT('Ctrl Pts',(-0.0114926307967935,-0.0324851356325864,
-0.0133446773993336));
#22418=CARTESIAN_POINT('Ctrl Pts',(-0.0114999758491315,-0.0324846443105656,
-0.0133509678385413));
#22419=CARTESIAN_POINT('Ctrl Pts',(-0.0115139184607852,-0.032483713644786,
-0.0133626831587809));
#22420=CARTESIAN_POINT('Ctrl Pts',(-0.0115205028986772,-0.0324832749481566,
-0.0133681231268906));
#22421=CARTESIAN_POINT('Ctrl Pts',(-0.0115354762927348,-0.0324822789926153,
-0.013380286176647));
#22422=CARTESIAN_POINT('Ctrl Pts',(-0.011543890970961,-0.0324817204497219,
-0.0133869767671743));
#22423=CARTESIAN_POINT('Ctrl Pts',(-0.011569086375589,-0.0324800511541379,
-0.0134065836508996));
#22424=CARTESIAN_POINT('Ctrl Pts',(-0.0115860633531154,-0.0324789303497482,
-0.0134192426668818));
#22425=CARTESIAN_POINT('Ctrl Pts',(-0.0116915941436823,-0.0324719851637537,
-0.0134946033438365));
#22426=CARTESIAN_POINT('Ctrl Pts',(-0.011786285673404,-0.0324658143181881,
-0.013548160498309));
#22427=CARTESIAN_POINT('Ctrl Pts',(-0.0119456088858079,-0.0324558243318147,
-0.0136172938886583));
#22428=CARTESIAN_POINT('Ctrl Pts',(-0.0120070114391975,-0.0324520667593339,
-0.0136394322758185));
#22429=CARTESIAN_POINT('Ctrl Pts',(-0.0120900727109608,-0.0324472395209694,
-0.0136635567748357));
#22430=CARTESIAN_POINT('Ctrl Pts',(-0.0121106345482471,-0.0324460649912443,
-0.0136690701732354));
#22431=CARTESIAN_POINT('Ctrl Pts',(-0.0121458068770551,-0.0324440979176854,
-0.0136777252120749));
#22432=CARTESIAN_POINT('Ctrl Pts',(-0.0121603606636426,-0.0324432960755124,
-0.0136810832366418));
#22433=CARTESIAN_POINT('Ctrl Pts',(-0.0121813230510829,-0.0324421607483455,
-0.0136856004017363));
#22434=CARTESIAN_POINT('Ctrl Pts',(-0.0121876934003862,-0.0324418183126306,
-0.0136869310279051));
#22435=CARTESIAN_POINT('Ctrl Pts',(-0.0121988085144354,-0.0324412255542373,
-0.013689179438025));
#22436=CARTESIAN_POINT('Ctrl Pts',(-0.0122035494616066,-0.0324409742265764,
-0.0136901152956575));
#22437=CARTESIAN_POINT('Ctrl Pts',(-0.0122137054581072,-0.0324404391109127,
-0.0136920705514625));
#22438=CARTESIAN_POINT('Ctrl Pts',(-0.0122191216327169,-0.0324401556984485,
-0.0136930832308128));
#22439=CARTESIAN_POINT('Ctrl Pts',(-0.0122339492827184,-0.0324393848949003,
-0.0136957734827298));
#22440=CARTESIAN_POINT('Ctrl Pts',(-0.0122433712510885,-0.0324389006907258,
-0.0136973926652461));
#22441=CARTESIAN_POINT('Ctrl Pts',(-0.0122941413774278,-0.0324363186966429,
-0.0137056325802603));
#22442=CARTESIAN_POINT('Ctrl Pts',(-0.0123357340323474,-0.0324342998576002,
-0.0137106560996469));
#22443=CARTESIAN_POINT('Ctrl Pts',(-0.0124603304710097,-0.0324284066491825,
-0.0137205806679845));
#22444=CARTESIAN_POINT('Ctrl Pts',(-0.0125435793494546,-0.0324246660088853,
-0.0137204756885645));
#22445=CARTESIAN_POINT('Ctrl Pts',(-0.0127051396550983,-0.0324172177402809,
-0.0137071944590896));
#22446=CARTESIAN_POINT('Ctrl Pts',(-0.012783243030385,-0.0324135277774321,
-0.0136946883165602));
#22447=CARTESIAN_POINT('Ctrl Pts',(-0.0128804727332715,-0.0324086174898915,
-0.0136713568852446));
#22448=CARTESIAN_POINT('Ctrl Pts',(-0.0129008019995967,-0.0324075733750139,
-0.0136660372410511));
#22449=CARTESIAN_POINT('Ctrl Pts',(-0.0129311921174884,-0.0324059835165886,
-0.0136574180833613));
#22450=CARTESIAN_POINT('Ctrl Pts',(-0.0129413384001461,-0.0324054478030911,
-0.0136544273626967));
#22451=CARTESIAN_POINT('Ctrl Pts',(-0.0129596066641425,-0.0324044740507557,
-0.0136488378149771));
#22452=CARTESIAN_POINT('Ctrl Pts',(-0.0129677394254137,-0.0324040372284005,
-0.0136462755159603));
#22453=CARTESIAN_POINT('Ctrl Pts',(-0.0129851617722922,-0.0324030941378602,
-0.0136406272856353));
#22454=CARTESIAN_POINT('Ctrl Pts',(-0.0129944440342363,-0.0324025871806956,
-0.0136375201106764));
#22455=CARTESIAN_POINT('Ctrl Pts',(-0.0130194928668625,-0.0324012066730194,
-0.0136288692764909));
#22456=CARTESIAN_POINT('Ctrl Pts',(-0.0130351996469986,-0.0324003275702542,
-0.0136231575440893));
#22457=CARTESIAN_POINT('Ctrl Pts',(-0.0131324138541097,-0.0323948006898061,
-0.0135860069610628));
#22458=CARTESIAN_POINT('Ctrl Pts',(-0.0132112105052648,-0.0323899285015497,
-0.013547952614839));
#22459=CARTESIAN_POINT('Ctrl Pts',(-0.0133619244911491,-0.03237992469363,
-0.0134586819281539));
#22460=CARTESIAN_POINT('Ctrl Pts',(-0.0134335328699816,-0.0323748114634214,
-0.0134075511645289));
#22461=CARTESIAN_POINT('Ctrl Pts',(-0.013519319976915,-0.0323684844588378,
-0.0133344961086026));
#22462=CARTESIAN_POINT('Ctrl Pts',(-0.0135378465294945,-0.0323671054819359,
-0.0133179308216092));
#22463=CARTESIAN_POINT('Ctrl Pts',(-0.0135681763908311,-0.0323648378633378,
-0.01328946392179));
#22464=CARTESIAN_POINT('Ctrl Pts',(-0.0135802002123302,-0.0323639361143729,
-0.0132778047351143));
#22465=CARTESIAN_POINT('Ctrl Pts',(-0.0135968426480222,-0.0323626871381552,
-0.0132611327743329));
#22466=CARTESIAN_POINT('Ctrl Pts',(-0.0136016211373579,-0.0323623284236823,
-0.0132562820136126));
#22467=CARTESIAN_POINT('Ctrl Pts',(-0.013609766483034,-0.0323617170548982,
-0.0132479032535201));
#22468=CARTESIAN_POINT('Ctrl Pts',(-0.0136131489844963,-0.032361463204849,
-0.0132443906603794));
#22469=CARTESIAN_POINT('Ctrl Pts',(-0.0136202154902349,-0.0323609330336838,
-0.0132369824026247));
#22470=CARTESIAN_POINT('Ctrl Pts',(-0.0136238959011567,-0.0323606569774543,
-0.0132330835124756));
#22471=CARTESIAN_POINT('Ctrl Pts',(-0.0136337905808048,-0.0323599147417337,
-0.0132224913961231));
#22472=CARTESIAN_POINT('Ctrl Pts',(-0.0136399659577281,-0.0323594514325772,
-0.013215761953922));
#22473=CARTESIAN_POINT('Ctrl Pts',(-0.0136691515799494,-0.0323572591902006,
-0.0131833853204877));
#22474=CARTESIAN_POINT('Ctrl Pts',(-0.0136913596375806,-0.032355583205021,
-0.0131570254128175));
#22475=CARTESIAN_POINT('Ctrl Pts',(-0.0137673233547661,-0.0323497331482562,
-0.0130604738930858));
#22476=CARTESIAN_POINT('Ctrl Pts',(-0.0138159115028095,-0.0323457577434689,
-0.0129864338199178));
#22477=CARTESIAN_POINT('Ctrl Pts',(-0.0139003702802725,-0.0323375961407567,
-0.012829926416516));
#22478=CARTESIAN_POINT('Ctrl Pts',(-0.0139359188354758,-0.0323334200739767,
-0.0127476779122721));
#22479=CARTESIAN_POINT('Ctrl Pts',(-0.0139694163163981,-0.0323281637173709,
-0.0126469625995437));
#22480=CARTESIAN_POINT('Ctrl Pts',(-0.0139744325090918,-0.032327328093665,
-0.0126310203375714));
#22481=CARTESIAN_POINT('Ctrl Pts',(-0.0139819473688683,-0.0323259943803933,
-0.0126057078580092));
#22482=CARTESIAN_POINT('Ctrl Pts',(-0.0139846184244454,-0.0323255019530356,
-0.0125963899495029));
#22483=CARTESIAN_POINT('Ctrl Pts',(-0.0139894767132811,-0.0323245703622555,
-0.0125788185640078));
#22484=CARTESIAN_POINT('Ctrl Pts',(-0.0139916835854576,-0.0323241318610183,
-0.0125705708706653));
#22485=CARTESIAN_POINT('Ctrl Pts',(-0.0139965056315262,-0.0323231379402778,
-0.0125519313608952));
#22486=CARTESIAN_POINT('Ctrl Pts',(-0.0139990812110588,-0.0323225812578732,
-0.0125415298349163));
#22487=CARTESIAN_POINT('Ctrl Pts',(-0.0140063846163501,-0.0323209228120207,
-0.0125106601955618));
#22488=CARTESIAN_POINT('Ctrl Pts',(-0.014010802899698,-0.0323198111887906,
-0.0124901219903299));
#22489=CARTESIAN_POINT('Ctrl Pts',(-0.0140335651968874,-0.0323134072121081,
-0.0123727010909512));
#22490=CARTESIAN_POINT('Ctrl Pts',(-0.0140430000022424,-0.032307835615159,
-0.0122743679938294));
#22491=CARTESIAN_POINT('Ctrl Pts',(-0.014043,-0.0323021764244909,-0.0121758532514363));
#22492=CARTESIAN_POINT('',(-0.0140429999980935,-0.0329194527355552,-0.0121757765831131));
#22493=CARTESIAN_POINT('Ctrl Pts',(-0.014043,-0.0324174341340783,-0.0121758532962676));
#22494=CARTESIAN_POINT('Ctrl Pts',(-0.0140429999999617,-0.0324177808943133,
-0.0121819461576369));
#22495=CARTESIAN_POINT('Ctrl Pts',(-0.0140429639115131,-0.0324181282307381,
-0.0121880396273339));
#22496=CARTESIAN_POINT('Ctrl Pts',(-0.0140419046234089,-0.0324232318073101,
-0.0122774465068135));
#22497=CARTESIAN_POINT('Ctrl Pts',(-0.0140341711796612,-0.0324280773472333,
-0.0123605416903952));
#22498=CARTESIAN_POINT('Ctrl Pts',(-0.0140125876239106,-0.0324351230456924,
-0.0124835094666267));
#22499=CARTESIAN_POINT('Ctrl Pts',(-0.0140037591473482,-0.0324374264332629,
-0.0125241098010196));
#22500=CARTESIAN_POINT('Ctrl Pts',(-0.0139908971430643,-0.0324401636230692,
-0.012573554180475));
#22501=CARTESIAN_POINT('Ctrl Pts',(-0.0139884058274866,-0.032440671318938,
-0.0125827788251411));
#22502=CARTESIAN_POINT('Ctrl Pts',(-0.0139843394442716,-0.0324414650629874,
-0.0125972983218125));
#22503=CARTESIAN_POINT('Ctrl Pts',(-0.0139828213964599,-0.0324417542309827,
-0.0126026087336661));
#22504=CARTESIAN_POINT('Ctrl Pts',(-0.013979914969254,-0.0324422945272259,
-0.0126125731846274));
#22505=CARTESIAN_POINT('Ctrl Pts',(-0.0139785331325594,-0.032442546001343,
-0.0126172288203762));
#22506=CARTESIAN_POINT('Ctrl Pts',(-0.0139752332176127,-0.0324431341391227,
-0.0126281573643367));
#22507=CARTESIAN_POINT('Ctrl Pts',(-0.0139732970943684,-0.032443469753171,
-0.0126344246548958));
#22508=CARTESIAN_POINT('Ctrl Pts',(-0.0139667605406211,-0.0324445727557668,
-0.0126551149007491));
#22509=CARTESIAN_POINT('Ctrl Pts',(-0.013961987693389,-0.032445330713125,
-0.0126694828998101));
#22510=CARTESIAN_POINT('Ctrl Pts',(-0.0139498766783522,-0.0324471490320271,
-0.0127042238135634));
#22511=CARTESIAN_POINT('Ctrl Pts',(-0.0139423195314849,-0.0324481990344315,
-0.0127245173354993));
#22512=CARTESIAN_POINT('Ctrl Pts',(-0.0139095917812991,-0.0324524441066034,
-0.0128070476695066));
#22513=CARTESIAN_POINT('Ctrl Pts',(-0.0138807987633129,-0.0324555106095279,
-0.0128677717206334));
#22514=CARTESIAN_POINT('Ctrl Pts',(-0.0137967414498903,-0.0324634090795341,
-0.0130187504035597));
#22515=CARTESIAN_POINT('Ctrl Pts',(-0.0137360007520845,-0.0324682410838825,
-0.0131055380670655));
#22516=CARTESIAN_POINT('Ctrl Pts',(-0.0136529287288984,-0.0324744695459774,
-0.0132015522961771));
#22517=CARTESIAN_POINT('Ctrl Pts',(-0.013638653784388,-0.0324755274946351,
-0.0132173765057506));
#22518=CARTESIAN_POINT('Ctrl Pts',(-0.0136166542635667,-0.0324771425786297,
-0.0132407706529972));
#22519=CARTESIAN_POINT('Ctrl Pts',(-0.0136091700568949,-0.0324776894577568,
-0.0132485636476857));
#22520=CARTESIAN_POINT('Ctrl Pts',(-0.0135955978805996,-0.0324786769642786,
-0.0132624018944978));
#22521=CARTESIAN_POINT('Ctrl Pts',(-0.0135895401288239,-0.0324791162537408,
-0.0132684762302694));
#22522=CARTESIAN_POINT('Ctrl Pts',(-0.0135765197807536,-0.0324800575018689,
-0.0132813162702421));
#22523=CARTESIAN_POINT('Ctrl Pts',(-0.0135695433750145,-0.0324805600743814,
-0.0132880673890639));
#22524=CARTESIAN_POINT('Ctrl Pts',(-0.0135504227140547,-0.0324819330113688,
-0.0133062243259164));
#22525=CARTESIAN_POINT('Ctrl Pts',(-0.0135381569252161,-0.0324828089250301,
-0.0133174997878952));
#22526=CARTESIAN_POINT('Ctrl Pts',(-0.0134613172970779,-0.0324882683933732,
-0.013385873039758));
#22527=CARTESIAN_POINT('Ctrl Pts',(-0.0133922442729897,-0.0324930702459721,
-0.0134376675824383));
#22528=CARTESIAN_POINT('Ctrl Pts',(-0.0132491825625166,-0.0325027046666989,
-0.0135272987180643));
#22529=CARTESIAN_POINT('Ctrl Pts',(-0.0131757362757509,-0.0325075102839964,
-0.013565479022581));
#22530=CARTESIAN_POINT('Ctrl Pts',(-0.0130604591241145,-0.0325145767457728,
-0.0136140944927583));
#22531=CARTESIAN_POINT('Ctrl Pts',(-0.0130206644780057,-0.0325169340987139,
-0.0136289744986511));
#22532=CARTESIAN_POINT('Ctrl Pts',(-0.0129711636299716,-0.0325197253521151,
-0.0136451886263051));
#22533=CARTESIAN_POINT('Ctrl Pts',(-0.0129619953984455,-0.0325202364941967,
-0.0136480970733859));
#22534=CARTESIAN_POINT('Ctrl Pts',(-0.0129475067367539,-0.0325210344126728,
-0.0136525446501887));
#22535=CARTESIAN_POINT('Ctrl Pts',(-0.0129422043352802,-0.0325213243611548,
-0.0136541411443886));
#22536=CARTESIAN_POINT('Ctrl Pts',(-0.0129322388107494,-0.0325218652763522,
-0.0136570832362048));
#22537=CARTESIAN_POINT('Ctrl Pts',(-0.0129275779324979,-0.0325221165992554,
-0.0136584353804902));
#22538=CARTESIAN_POINT('Ctrl Pts',(-0.0129166273318506,-0.0325227032802055,
-0.0136615562690325));
#22539=CARTESIAN_POINT('Ctrl Pts',(-0.012910332668483,-0.0325230376050304,
-0.0136633070807751));
#22540=CARTESIAN_POINT('Ctrl Pts',(-0.0128895613395232,-0.0325241318068259,
-0.0136689425739873));
#22541=CARTESIAN_POINT('Ctrl Pts',(-0.0128750387855278,-0.0325248824584113,
-0.0136726564126512));
#22542=CARTESIAN_POINT('Ctrl Pts',(-0.0128396904560963,-0.0325266798456656,
-0.0136811492180981));
#22543=CARTESIAN_POINT('Ctrl Pts',(-0.0128188147461368,-0.0325277165349856,
-0.013685708470305));
#22544=CARTESIAN_POINT('Ctrl Pts',(-0.0127335509036351,-0.0325318742835031,
-0.013702482713648));
#22545=CARTESIAN_POINT('Ctrl Pts',(-0.0126685072039677,-0.0325348720916436,
-0.0137110241936687));
#22546=CARTESIAN_POINT('Ctrl Pts',(-0.0124954567473541,-0.0325428006478178,
-0.0137226145925197));
#22547=CARTESIAN_POINT('Ctrl Pts',(-0.0123873503650151,-0.0325477264178684,
-0.0137185129836419));
#22548=CARTESIAN_POINT('Ctrl Pts',(-0.0122595450338619,-0.0325540614977239,
-0.0137001502063682));
#22549=CARTESIAN_POINT('Ctrl Pts',(-0.0122385965895038,-0.0325551155661509,
-0.0136966977535008));
#22550=CARTESIAN_POINT('Ctrl Pts',(-0.0122071204858661,-0.0325567258693322,
-0.013690840737277));
#22551=CARTESIAN_POINT('Ctrl Pts',(-0.0121965354970523,-0.0325572719404621,
-0.0136887560175417));
#22552=CARTESIAN_POINT('Ctrl Pts',(-0.0121775757708738,-0.0325582585679991,
-0.0136848149109564));
#22553=CARTESIAN_POINT('Ctrl Pts',(-0.012169192949372,-0.0325586977965608,
-0.0136829993507281));
#22554=CARTESIAN_POINT('Ctrl Pts',(-0.0121513448073806,-0.032559639548806,
-0.0136789777025424));
#22555=CARTESIAN_POINT('Ctrl Pts',(-0.0121418843504614,-0.0325601426934379,
-0.0136767518937284));
#22556=CARTESIAN_POINT('Ctrl Pts',(-0.0121162167577163,-0.0325615188373242,
-0.0136704564597074));
#22557=CARTESIAN_POINT('Ctrl Pts',(-0.0121000540087729,-0.0325623974296017,
-0.01366621277227));
#22558=CARTESIAN_POINT('Ctrl Pts',(-0.0119994044083191,-0.0325679458533994,
-0.0136380310854544));
#22559=CARTESIAN_POINT('Ctrl Pts',(-0.0119170322623532,-0.0325728428169011,
-0.0136071829817816));
#22560=CARTESIAN_POINT('Ctrl Pts',(-0.0117604114638662,-0.0325827462484919,
-0.0135327570164667));
#22561=CARTESIAN_POINT('Ctrl Pts',(-0.011686276429226,-0.0325877277857869,
-0.0134896390262423));
#22562=CARTESIAN_POINT('Ctrl Pts',(-0.0115847225035555,-0.0325946982489978,
-0.0134186652507507));
#22563=CARTESIAN_POINT('Ctrl Pts',(-0.0115541690903881,-0.0325968149861419,
-0.0133955740710582));
#22564=CARTESIAN_POINT('Ctrl Pts',(-0.0115171739800513,-0.0325993714889418,
-0.0133653874487364));
#22565=CARTESIAN_POINT('Ctrl Pts',(-0.0115098986709613,-0.032599873897062,
-0.0133593387640804));
#22566=CARTESIAN_POINT('Ctrl Pts',(-0.0114985226211263,-0.0326006582991061,
-0.0133497023973405));
#22567=CARTESIAN_POINT('Ctrl Pts',(-0.0114943845729975,-0.0326009433737483,
-0.0133461593533875));
#22568=CARTESIAN_POINT('Ctrl Pts',(-0.0114865776302015,-0.0326014805723252,
-0.013339402978093));
#22569=CARTESIAN_POINT('Ctrl Pts',(-0.0114829051272995,-0.0326017329928445,
-0.0133361941004829));
#22570=CARTESIAN_POINT('Ctrl Pts',(-0.0114742191309836,-0.0326023294453778,
-0.0133285317221074));
#22571=CARTESIAN_POINT('Ctrl Pts',(-0.0114692192928218,-0.0326026723406502,
-0.0133240628074794));
#22572=CARTESIAN_POINT('Ctrl Pts',(-0.0114523844923257,-0.0326038260397585,
-0.0133088170751233));
#22573=CARTESIAN_POINT('Ctrl Pts',(-0.0114406877850518,-0.0326046261807342,
-0.013297888431824));
#22574=CARTESIAN_POINT('Ctrl Pts',(-0.0114123585830405,-0.0326065666939424,
-0.0132705815181657));
#22575=CARTESIAN_POINT('Ctrl Pts',(-0.0113959233188129,-0.0326076947734705,
-0.0132540037973761));
#22576=CARTESIAN_POINT('Ctrl Pts',(-0.0113267243139725,-0.0326124874498326,
-0.0131809624494235));
#22577=CARTESIAN_POINT('Ctrl Pts',(-0.0112778649772784,-0.0326159879599315,
-0.0131209498722869));
#22578=CARTESIAN_POINT('Ctrl Pts',(-0.0111811589440617,-0.0326237311146279,
-0.0129820567978842));
#22579=CARTESIAN_POINT('Ctrl Pts',(-0.011135467511743,-0.0326279798353588,
-0.0129020453472362));
#22580=CARTESIAN_POINT('Ctrl Pts',(-0.0110880260708171,-0.0326335643731067,
-0.0127984776858735));
#22581=CARTESIAN_POINT('Ctrl Pts',(-0.0110793058263517,-0.0326346545212671,
-0.0127783145082686));
#22582=CARTESIAN_POINT('Ctrl Pts',(-0.0110669486024995,-0.0326363019531987,
-0.012747980119422));
#22583=CARTESIAN_POINT('Ctrl Pts',(-0.0110629829701518,-0.0326368481040948,
-0.0127379453333044));
#22584=CARTESIAN_POINT('Ctrl Pts',(-0.0110560543977237,-0.0326378348183345,
-0.0127198603339765));
#22585=CARTESIAN_POINT('Ctrl Pts',(-0.0110530527060399,-0.0326382740528369,
-0.0127118253889376));
#22586=CARTESIAN_POINT('Ctrl Pts',(-0.0110467934629567,-0.0326392157549688,
-0.0126946347371269));
#22587=CARTESIAN_POINT('Ctrl Pts',(-0.0110435551126964,-0.032639718842843,
-0.0126854724749631));
#22588=CARTESIAN_POINT('Ctrl Pts',(-0.0110349857874414,-0.0326410946685077,
-0.0126604783112454));
#22589=CARTESIAN_POINT('Ctrl Pts',(-0.0110298251291063,-0.0326419729949649,
-0.0126445897550293));
#22590=CARTESIAN_POINT('Ctrl Pts',(-0.0109992051731233,-0.0326475123413992,
-0.0125448326862552));
#22591=CARTESIAN_POINT('Ctrl Pts',(-0.010980676026657,-0.0326523995820292,
-0.012459017216906));
#22592=CARTESIAN_POINT('Ctrl Pts',(-0.0109586794845246,-0.0326622760399338,
-0.0122874761640966));
#22593=CARTESIAN_POINT('Ctrl Pts',(-0.010954865690689,-0.0326672401449363,
-0.0122020950875256));
#22594=CARTESIAN_POINT('Ctrl Pts',(-0.0109596091936112,-0.0326742203875233,
-0.0120781663327876));
#22595=CARTESIAN_POINT('Ctrl Pts',(-0.0109625437130375,-0.0326763610460147,
-0.0120395624830163));
#22596=CARTESIAN_POINT('Ctrl Pts',(-0.0109680016151335,-0.0326789416044001,
-0.0119916794927017));
#22597=CARTESIAN_POINT('Ctrl Pts',(-0.0109691632003269,-0.0326794455302104,
-0.0119822616048896));
#22598=CARTESIAN_POINT('Ctrl Pts',(-0.0109711290972703,-0.0326802317568371,
-0.0119674486216061));
#22599=CARTESIAN_POINT('Ctrl Pts',(-0.0109718752432203,-0.0326805171613873,
-0.0119620461980114));
#22600=CARTESIAN_POINT('Ctrl Pts',(-0.0109733426014132,-0.0326810545994463,
-0.011951822142272));
#22601=CARTESIAN_POINT('Ctrl Pts',(-0.0109740580350851,-0.0326813069339909,
-0.0119469998700646));
#22602=CARTESIAN_POINT('Ctrl Pts',(-0.0109758099470793,-0.0326819026710148,
-0.0119355649553286));
#22603=CARTESIAN_POINT('Ctrl Pts',(-0.0109768666299908,-0.0326822449446563,
-0.0119289554536394));
#22604=CARTESIAN_POINT('Ctrl Pts',(-0.0109805835797715,-0.0326833942479967,
-0.0119066386306476));
#22605=CARTESIAN_POINT('Ctrl Pts',(-0.0109834441573704,-0.0326841907247585,
-0.0118909652339224));
#22606=CARTESIAN_POINT('Ctrl Pts',(-0.0109910637827476,-0.032686120532288,
-0.0118525912815925));
#22607=CARTESIAN_POINT('Ctrl Pts',(-0.0109960929496927,-0.0326872417471431,
-0.0118299479481645));
#22608=CARTESIAN_POINT('Ctrl Pts',(-0.0110198547796943,-0.032691983580424,
-0.0117333102471039));
#22609=CARTESIAN_POINT('Ctrl Pts',(-0.0110435536591722,-0.0326954435644003,
-0.01166064502976));
#22610=CARTESIAN_POINT('Ctrl Pts',(-0.0111079724699095,-0.0327032047436342,
-0.0115036770522244));
#22611=CARTESIAN_POINT('Ctrl Pts',(-0.0111511710667793,-0.0327075133650244,
-0.0114207241683673));
#22612=CARTESIAN_POINT('Ctrl Pts',(-0.0112134049155082,-0.0327131612647455,
-0.0113237970705941));
#22613=CARTESIAN_POINT('Ctrl Pts',(-0.011225602763543,-0.0327142461164853,
-0.0113056588654261));
#22614=CARTESIAN_POINT('Ctrl Pts',(-0.0112443793212655,-0.0327158870886356,
-0.0112789800078663));
#22615=CARTESIAN_POINT('Ctrl Pts',(-0.0112506691681248,-0.0327164322079441,
-0.0112702388919093));
#22616=CARTESIAN_POINT('Ctrl Pts',(-0.0112621311625699,-0.0327174178021129,
-0.0112546566306558));
#22617=CARTESIAN_POINT('Ctrl Pts',(-0.0112672698573007,-0.0327178569610101,
-0.0112477913657454));
#22618=CARTESIAN_POINT('Ctrl Pts',(-0.0112783615668921,-0.0327187993171647,
-0.0112332275715205));
#22619=CARTESIAN_POINT('Ctrl Pts',(-0.0112843307023872,-0.0327193031438145,
-0.011225541836087));
#22620=CARTESIAN_POINT('Ctrl Pts',(-0.0113007828619445,-0.0327206831129039,
-0.0112047670588319));
#22621=CARTESIAN_POINT('Ctrl Pts',(-0.0113114069942638,-0.0327215649008488,
-0.0111917918847195));
#22622=CARTESIAN_POINT('Ctrl Pts',(-0.0113803126264655,-0.0327272273863249,
-0.0111103820167889));
#22623=CARTESIAN_POINT('Ctrl Pts',(-0.0114442609884801,-0.0327322468603228,
-0.0110469866249132));
#22624=CARTESIAN_POINT('Ctrl Pts',(-0.0115819114031304,-0.0327424810909635,
-0.0109325055699087));
#22625=CARTESIAN_POINT('Ctrl Pts',(-0.0116552824548097,-0.0327476727498928,
-0.010881537712132));
#22626=CARTESIAN_POINT('Ctrl Pts',(-0.0117615386664768,-0.0327545259767972,
-0.0108206289413296));
#22627=CARTESIAN_POINT('Ctrl Pts',(-0.0117909630646408,-0.0327563581860617,
-0.010805004976924));
#22628=CARTESIAN_POINT('Ctrl Pts',(-0.0118290012093397,-0.0327586233443108,
-0.0107863600026639));
#22629=CARTESIAN_POINT('Ctrl Pts',(-0.0118371656007931,-0.0327591036113302,
-0.0107824468383063));
#22630=CARTESIAN_POINT('Ctrl Pts',(-0.0118502163364397,-0.0327598613609656,
-0.0107763323319675));
#22631=CARTESIAN_POINT('Ctrl Pts',(-0.0118550804041916,-0.032760141596235,
-0.0107740842512208));
#22632=CARTESIAN_POINT('Ctrl Pts',(-0.0118644225726241,-0.0327606755157795,
-0.0107698253961913));
#22633=CARTESIAN_POINT('Ctrl Pts',(-0.0118688986597354,-0.0327609294298043,
-0.0107678106049485));
#22634=CARTESIAN_POINT('Ctrl Pts',(-0.0118796947980605,-0.0327615374383849,
-0.0107630128345269));
#22635=CARTESIAN_POINT('Ctrl Pts',(-0.0118860241395326,-0.0327618902689997,
-0.0107602508237543));
#22636=CARTESIAN_POINT('Ctrl Pts',(-0.0119082266795699,-0.03276311603792,
-0.0107507389588601));
#22637=CARTESIAN_POINT('Ctrl Pts',(-0.0119241948405835,-0.032763976425662,
-0.01074421262814));
#22638=CARTESIAN_POINT('Ctrl Pts',(-0.0119643539121354,-0.0327660955354746,
-0.0107285799143478));
#22639=CARTESIAN_POINT('Ctrl Pts',(-0.0119886709526783,-0.0327673388034294,
-0.01071981081942));
#22640=CARTESIAN_POINT('Ctrl Pts',(-0.0121037832715948,-0.032773087197665,
-0.0106815393746914));
#22641=CARTESIAN_POINT('Ctrl Pts',(-0.0121969719264597,-0.0327773579174847,
-0.0106598923281588));
#22642=CARTESIAN_POINT('Ctrl Pts',(-0.0123691074703633,-0.0327853693868554,
-0.0106364247099558));
#22643=CARTESIAN_POINT('Ctrl Pts',(-0.012447332898459,-0.032789053757119,
-0.0106317685655158));
#22644=CARTESIAN_POINT('Ctrl Pts',(-0.0125421513020828,-0.0327937494306661,
-0.0106333399669067));
#22645=CARTESIAN_POINT('Ctrl Pts',(-0.0125587284274799,-0.0327945785354581,
-0.0106338821394445));
#22646=CARTESIAN_POINT('Ctrl Pts',(-0.0125850671367133,-0.0327959101214111,
-0.0106351689126419));
#22647=CARTESIAN_POINT('Ctrl Pts',(-0.0125948361536064,-0.032796407125762,
-0.0106357393764921));
#22648=CARTESIAN_POINT('Ctrl Pts',(-0.0126130664320088,-0.0327973406722879,
-0.0106369780442519));
#22649=CARTESIAN_POINT('Ctrl Pts',(-0.0126215289170978,-0.0327977764707723,
-0.0106376232166725));
#22650=CARTESIAN_POINT('Ctrl Pts',(-0.0126405959430574,-0.0327987640530906,
-0.0106392351927735));
#22651=CARTESIAN_POINT('Ctrl Pts',(-0.012651196591259,-0.0327993170826376,
-0.0106402420178862));
#22652=CARTESIAN_POINT('Ctrl Pts',(-0.0126829024536885,-0.0328009833492266,
-0.0106435848497243));
#22653=CARTESIAN_POINT('Ctrl Pts',(-0.0127039701414622,-0.0328021067835447,
-0.0106462468042387));
#22654=CARTESIAN_POINT('Ctrl Pts',(-0.0128046186569758,-0.0328075536333466,
-0.010661080274502));
#22655=CARTESIAN_POINT('Ctrl Pts',(-0.0128832112915167,-0.0328120562245261,
-0.0106790312885555));
#22656=CARTESIAN_POINT('Ctrl Pts',(-0.0130421918661889,-0.0328215700421989,
-0.0107286888424951));
#22657=CARTESIAN_POINT('Ctrl Pts',(-0.0131220551897563,-0.0328265784254938,
-0.0107611786217417));
#22658=CARTESIAN_POINT('Ctrl Pts',(-0.0132322551602566,-0.0328335270169368,
-0.0108171553750811));
#22659=CARTESIAN_POINT('Ctrl Pts',(-0.0132650886670807,-0.0328356007848239,
-0.0108353692798452));
#22660=CARTESIAN_POINT('Ctrl Pts',(-0.0133052833941123,-0.0328381139623187,
-0.0108596252708577));
#22661=CARTESIAN_POINT('Ctrl Pts',(-0.0133132949983306,-0.0328386135641192,
-0.0108645604937411));
#22662=CARTESIAN_POINT('Ctrl Pts',(-0.0133258634042756,-0.0328393945915308,
-0.0108724622515164));
#22663=CARTESIAN_POINT('Ctrl Pts',(-0.0133304504072629,-0.0328396790554818,
-0.0108753800359229));
#22664=CARTESIAN_POINT('Ctrl Pts',(-0.0133391259879381,-0.032840215815753,
-0.010880963177334));
#22665=CARTESIAN_POINT('Ctrl Pts',(-0.0133432174288135,-0.0328404684003856,
-0.0108836237455743));
#22666=CARTESIAN_POINT('Ctrl Pts',(-0.0133529201297948,-0.0328410661999849,
-0.0108899988878199));
#22667=CARTESIAN_POINT('Ctrl Pts',(-0.013358519897868,-0.0328414102633424,
-0.010893730877907));
#22668=CARTESIAN_POINT('Ctrl Pts',(-0.0133774740956578,-0.032842572257485,
-0.0109065428477252));
#22669=CARTESIAN_POINT('Ctrl Pts',(-0.0133907107283158,-0.0328433793163547,
-0.0109157960593147));
#22670=CARTESIAN_POINT('Ctrl Pts',(-0.0134229456072659,-0.0328453400896089,
-0.0109390920326783));
#22671=CARTESIAN_POINT('Ctrl Pts',(-0.0134417716285728,-0.0328464811728091,
-0.0109533667694848));
#22672=CARTESIAN_POINT('Ctrl Pts',(-0.0135221867171937,-0.0328513717640358,
-0.0110173017218181));
#22673=CARTESIAN_POINT('Ctrl Pts',(-0.0135802355540582,-0.0328549504506304,
-0.0110712266880717));
#22674=CARTESIAN_POINT('Ctrl Pts',(-0.013700364442488,-0.0328630579585532,
-0.0112013896027806));
#22675=CARTESIAN_POINT('Ctrl Pts',(-0.013759813755502,-0.0328676008757561,
-0.0112795715416857));
#22676=CARTESIAN_POINT('Ctrl Pts',(-0.0138202878194713,-0.0328732816843213,
-0.0113771226022248));
#22677=CARTESIAN_POINT('Ctrl Pts',(-0.013828896551105,-0.0328741203482622,
-0.0113915290162322));
#22678=CARTESIAN_POINT('Ctrl Pts',(-0.0138421723004847,-0.032875463821008,
-0.0114145917419387));
#22679=CARTESIAN_POINT('Ctrl Pts',(-0.0138469946144851,-0.0328759629805441,
-0.0114231573810236));
#22680=CARTESIAN_POINT('Ctrl Pts',(-0.0138558645071177,-0.0328769025759237,
-0.0114392707862286));
#22681=CARTESIAN_POINT('Ctrl Pts',(-0.0138599317404098,-0.0328773422814102,
-0.0114468073353758));
#22682=CARTESIAN_POINT('Ctrl Pts',(-0.013868904590534,-0.0328783326456948,
-0.0114637703285601));
#22683=CARTESIAN_POINT('Ctrl Pts',(-0.013873775959069,-0.0328788844954938,
-0.0114732143154514));
#22684=CARTESIAN_POINT('Ctrl Pts',(-0.0138880372903935,-0.0328805435929272,
-0.0115015776912613));
#22685=CARTESIAN_POINT('Ctrl Pts',(-0.0138971364804514,-0.0328816609083075,
-0.0115206398151141));
#22686=CARTESIAN_POINT('Ctrl Pts',(-0.0139386436631161,-0.032887051523899,
-0.0116123931994035));
#22687=CARTESIAN_POINT('Ctrl Pts',(-0.0139657830044827,-0.0328914997311912,
-0.0116873245635427));
#22688=CARTESIAN_POINT('Ctrl Pts',(-0.0140183362770819,-0.0329027411556628,
-0.0118770741745044));
#22689=CARTESIAN_POINT('Ctrl Pts',(-0.0140366543374166,-0.0329096254192521,
-0.0119933458369967));
#22690=CARTESIAN_POINT('Ctrl Pts',(-0.0140422074617452,-0.0329167382459104,
-0.0121244821376552));
#22691=CARTESIAN_POINT('Ctrl Pts',(-0.0140426082344107,-0.0329174845899751,
-0.0121384004940174));
#22692=CARTESIAN_POINT('Ctrl Pts',(-0.0140428857751294,-0.0329184474911976,
-0.012156597996416));
#22693=CARTESIAN_POINT('Ctrl Pts',(-0.0140429332088814,-0.0329186727920838,
-0.0121608734644583));
#22694=CARTESIAN_POINT('Ctrl Pts',(-0.0140429874690276,-0.032919083176937,
-0.012168694850362));
#22695=CARTESIAN_POINT('Ctrl Pts',(-0.0140429998218256,-0.0329192680377374,
-0.0121722307005113));
#22696=CARTESIAN_POINT('Ctrl Pts',(-0.0140429999980935,-0.0329194527355552,
-0.0121757765831131));
#22697=CARTESIAN_POINT('Ctrl Pts',(-0.0140429999975648,-0.0329194522153789,
-0.0121757665966515));
#22698=CARTESIAN_POINT('Ctrl Pts',(-0.0140429999990012,-0.032919453720546,
-0.012175795493288));
#22699=CARTESIAN_POINT('Ctrl Pts',(-0.014043,-0.0329194552256883,-0.012175824389923));
#22700=CARTESIAN_POINT('Ctrl Pts',(-0.014043,-0.0329194567307744,-0.012175853286558));
#22701=CARTESIAN_POINT('Origin',(-0.0125,-0.0375520664398416,-0.0121758532865581));
#22702=CARTESIAN_POINT('',(-0.014043,-0.0334176320149228,-0.0121758533032418));
#22703=CARTESIAN_POINT('',(-0.014043,-0.0333016781458831,-0.0121758532817056));
#22704=CARTESIAN_POINT('',(-0.014043,-0.0375520664398416,-0.012175853286558));
#22705=CARTESIAN_POINT('Ctrl Pts',(-0.014043,-0.033301678145883,-0.0121758532768531));
#22706=CARTESIAN_POINT('Ctrl Pts',(-0.014042999999241,-0.033296152169727,
-0.0120551830319892));
#22707=CARTESIAN_POINT('Ctrl Pts',(-0.0140288457417181,-0.0332906903108907,
-0.0119349225769698));
#22708=CARTESIAN_POINT('Ctrl Pts',(-0.0139966325516127,-0.0332838656524112,
-0.0118000014907481));
#22709=CARTESIAN_POINT('Ctrl Pts',(-0.0139921423245643,-0.0332829702098229,
-0.0117825533799734));
#22710=CARTESIAN_POINT('Ctrl Pts',(-0.0139844089798668,-0.0332815101562521,
-0.0117545447263159));
#22711=CARTESIAN_POINT('Ctrl Pts',(-0.0139813561101524,-0.0332809516970285,
-0.011743933167611));
#22712=CARTESIAN_POINT('Ctrl Pts',(-0.0139757314063109,-0.0332799530605089,
-0.0117251435179896));
#22713=CARTESIAN_POINT('Ctrl Pts',(-0.0139732047965941,-0.0332795143826616,
-0.0117169523142201));
#22714=CARTESIAN_POINT('Ctrl Pts',(-0.0139677346345415,-0.0332785847981094,
-0.0116997290599259));
#22715=CARTESIAN_POINT('Ctrl Pts',(-0.0139647756697856,-0.0332780933963267,
-0.0116907023117127));
#22716=CARTESIAN_POINT('Ctrl Pts',(-0.0139566703640938,-0.0332767767238189,
-0.0116667261811201));
#22717=CARTESIAN_POINT('Ctrl Pts',(-0.0139513773794409,-0.0332759466169526,
-0.0116518278707558));
#22718=CARTESIAN_POINT('Ctrl Pts',(-0.0139221889122559,-0.0332715180028544,
-0.0115735070654471));
#22719=CARTESIAN_POINT('Ctrl Pts',(-0.013894365681829,-0.0332677884639099,
-0.0115116358488667));
#22720=CARTESIAN_POINT('Ctrl Pts',(-0.0138174143498841,-0.0332585334771182,
-0.011366824163526));
#22721=CARTESIAN_POINT('Ctrl Pts',(-0.0137644127396292,-0.0332529236212528,
-0.0112862647760647));
#22722=CARTESIAN_POINT('Ctrl Pts',(-0.0136740383076148,-0.0332447201061352,
-0.0111734466349453));
#22723=CARTESIAN_POINT('Ctrl Pts',(-0.0136420623434125,-0.0332420227577066,
-0.0111371620818609));
#22724=CARTESIAN_POINT('Ctrl Pts',(-0.0136015312225119,-0.0332388977514583,
-0.0110953087936099));
#22725=CARTESIAN_POINT('Ctrl Pts',(-0.0135945604091944,-0.0332383700911428,
-0.0110882481394156));
#22726=CARTESIAN_POINT('Ctrl Pts',(-0.0135835550348256,-0.0332375529407202,
-0.0110773139134795));
#22727=CARTESIAN_POINT('Ctrl Pts',(-0.0135795668106827,-0.0332372600152216,
-0.0110733943209213));
#22728=CARTESIAN_POINT('Ctrl Pts',(-0.0135724503514152,-0.03323674313081,
-0.0110664759746853));
#22729=CARTESIAN_POINT('Ctrl Pts',(-0.0135693307625849,-0.0332365185138221,
-0.0110634686871448));
#22730=CARTESIAN_POINT('Ctrl Pts',(-0.0135617929739524,-0.0332359804373121,
-0.011056263262125));
#22731=CARTESIAN_POINT('Ctrl Pts',(-0.0135573625317489,-0.0332356679746439,
-0.0110520781216601));
#22732=CARTESIAN_POINT('Ctrl Pts',(-0.0135436433875685,-0.0332347116196893,
-0.01103927153246));
#22733=CARTESIAN_POINT('Ctrl Pts',(-0.0135342729675937,-0.0332340740578503,
-0.0110307379857063));
#22734=CARTESIAN_POINT('Ctrl Pts',(-0.0134867184240696,-0.0332309098259927,
-0.0109884905393795));
#22735=CARTESIAN_POINT('Ctrl Pts',(-0.0134469836643739,-0.0332284925796322,
-0.0109565640261634));
#22736=CARTESIAN_POINT('Ctrl Pts',(-0.0133142590940587,-0.033220866288037,
-0.0108603308489456));
#22737=CARTESIAN_POINT('Ctrl Pts',(-0.0132157712838526,-0.0332158413491706,
-0.0108042521872334));
#22738=CARTESIAN_POINT('Ctrl Pts',(-0.0130694227664543,-0.0332082935853901,
-0.0107410145810245));
#22739=CARTESIAN_POINT('Ctrl Pts',(-0.0130259984901731,-0.033206048986665,
-0.0107245333712017));
#22740=CARTESIAN_POINT('Ctrl Pts',(-0.0129680087563431,-0.0332030117683303,
-0.0107054687749478));
#22741=CARTESIAN_POINT('Ctrl Pts',(-0.0129540541024748,-0.0332022780351559,
-0.0107010998626277));
#22742=CARTESIAN_POINT('Ctrl Pts',(-0.0129311800476335,-0.0332010698260814,
-0.0106942939019389));
#22743=CARTESIAN_POINT('Ctrl Pts',(-0.0129222969583428,-0.0332005992834258,
-0.0106917374832196));
#22744=CARTESIAN_POINT('Ctrl Pts',(-0.012905056972069,-0.0331996832850976,
-0.0106869433878798));
#22745=CARTESIAN_POINT('Ctrl Pts',(-0.0128967031576967,-0.0331992381715063,
-0.0106846958711251));
#22746=CARTESIAN_POINT('Ctrl Pts',(-0.0128770990768917,-0.0331981905139784,
-0.0106795979697089));
#22747=CARTESIAN_POINT('Ctrl Pts',(-0.0128658347779109,-0.0331975861617243,
-0.0106768040571065));
#22748=CARTESIAN_POINT('Ctrl Pts',(-0.012828587192449,-0.0331955795278258,
-0.0106680102706161));
#22749=CARTESIAN_POINT('Ctrl Pts',(-0.0128024808630634,-0.033194159870343,
-0.0106625571120584));
#22750=CARTESIAN_POINT('Ctrl Pts',(-0.0127393392062007,-0.0331906935492558,
-0.0106510670502018));
#22751=CARTESIAN_POINT('Ctrl Pts',(-0.0127022005491562,-0.0331886277416685,
-0.0106456993854977));
#22752=CARTESIAN_POINT('Ctrl Pts',(-0.0125228879134571,-0.0331785426351897,
-0.0106264253128829));
#22753=CARTESIAN_POINT('Ctrl Pts',(-0.0123794560510369,-0.0331700629168765,
-0.0106309536660835));
#22754=CARTESIAN_POINT('Ctrl Pts',(-0.0122193872987455,-0.0331611545540931,
-0.0106584576307248));
#22755=CARTESIAN_POINT('Ctrl Pts',(-0.0122001368681476,-0.0331600940283299,
-0.0106621441876746));
#22756=CARTESIAN_POINT('Ctrl Pts',(-0.0121736682899321,-0.0331586557360306,
-0.0106677378483833));
#22757=CARTESIAN_POINT('Ctrl Pts',(-0.0121663866318791,-0.0331582621475538,
-0.0106693319010822));
#22758=CARTESIAN_POINT('Ctrl Pts',(-0.0121547273851938,-0.0331576356276604,
-0.0106719729469641));
#22759=CARTESIAN_POINT('Ctrl Pts',(-0.0121503424172609,-0.0331574008367902,
-0.0106729864161349));
#22760=CARTESIAN_POINT('Ctrl Pts',(-0.0121410762691838,-0.0331569065573037,
-0.0106751707914174));
#22761=CARTESIAN_POINT('Ctrl Pts',(-0.0121361962496979,-0.0331566473516613,
-0.0106763463582545));
#22762=CARTESIAN_POINT('Ctrl Pts',(-0.0121239753659187,-0.0331560008153209,
-0.0106793534651212));
#22763=CARTESIAN_POINT('Ctrl Pts',(-0.0121166419780126,-0.0331556151921408,
-0.0106812152459307));
#22764=CARTESIAN_POINT('Ctrl Pts',(-0.012087969008273,-0.0331541155907492,
-0.0106887195791152));
#22765=CARTESIAN_POINT('Ctrl Pts',(-0.0120667369238895,-0.0331530228913737,
-0.0106947660502066));
#22766=CARTESIAN_POINT('Ctrl Pts',(-0.0120105755842982,-0.0331501626028183,
-0.0107120708379579));
#22767=CARTESIAN_POINT('Ctrl Pts',(-0.0119759049515203,-0.0331484280663903,
-0.0107241232949017));
#22768=CARTESIAN_POINT('Ctrl Pts',(-0.0118429268132295,-0.0331417856479386,
-0.0107757359221877));
#22769=CARTESIAN_POINT('Ctrl Pts',(-0.011748369474188,-0.0331370647311215,
-0.0108241409225991));
#22770=CARTESIAN_POINT('Ctrl Pts',(-0.0116147830261486,-0.0331295780527243,
-0.0109109085821144));
#22771=CARTESIAN_POINT('Ctrl Pts',(-0.0115715905166981,-0.0331270148741966,
-0.0109422612457511));
#22772=CARTESIAN_POINT('Ctrl Pts',(-0.0115182038036025,-0.0331236049908651,
-0.0109854081652544));
#22773=CARTESIAN_POINT('Ctrl Pts',(-0.0115064415724431,-0.0331228377457005,
-0.0109952072821043));
#22774=CARTESIAN_POINT('Ctrl Pts',(-0.0114877022356755,-0.0331215883127571,
-0.0110112973921178));
#22775=CARTESIAN_POINT('Ctrl Pts',(-0.0114806332307526,-0.0331211105987463,
-0.0110174800394696));
#22776=CARTESIAN_POINT('Ctrl Pts',(-0.0114671999910074,-0.0331201902407994,
-0.0110294471211287));
#22777=CARTESIAN_POINT('Ctrl Pts',(-0.011460826800954,-0.0331197480501957,
-0.0110352210000202));
#22778=CARTESIAN_POINT('Ctrl Pts',(-0.0114462227531703,-0.0331187217275783,
-0.0110486757271219));
#22779=CARTESIAN_POINT('Ctrl Pts',(-0.0114380270948717,-0.0331181360022596,
-0.011056393918768));
#22780=CARTESIAN_POINT('Ctrl Pts',(-0.0114121546808937,-0.0331162551347873,
-0.0110812988605483));
#22781=CARTESIAN_POINT('Ctrl Pts',(-0.0113948056805476,-0.0331149454778611,
-0.0110988192799597));
#22782=CARTESIAN_POINT('Ctrl Pts',(-0.0113113018554094,-0.0331083951899383,
-0.0111872909957439));
#22783=CARTESIAN_POINT('Ctrl Pts',(-0.0112515282733817,-0.0331028933737157,
-0.0112639473365652));
#22784=CARTESIAN_POINT('Ctrl Pts',(-0.0111485094637647,-0.0330918868883044,
-0.011425351829882));
#22785=CARTESIAN_POINT('Ctrl Pts',(-0.0111050893947673,-0.0330864133788897,
-0.0115095156814365));
#22786=CARTESIAN_POINT('Ctrl Pts',(-0.0110644683691668,-0.033080544567881,
-0.0116099132101176));
#22787=CARTESIAN_POINT('Ctrl Pts',(-0.0110594667646659,-0.0330798051885138,
-0.0116227680698562));
#22788=CARTESIAN_POINT('Ctrl Pts',(-0.0110524208953178,-0.0330787401342785,
-0.0116416212705606));
#22789=CARTESIAN_POINT('Ctrl Pts',(-0.0110502402635295,-0.0330784069972564,
-0.0116475675490016));
#22790=CARTESIAN_POINT('Ctrl Pts',(-0.0110464631061732,-0.0330778238832217,
-0.0116580668689895));
#22791=CARTESIAN_POINT('Ctrl Pts',(-0.0110448512311633,-0.0330775730171807,
-0.0116626142207783));
#22792=CARTESIAN_POINT('Ctrl Pts',(-0.0110414320188788,-0.033077036505556,
-0.0116724059589919));
#22793=CARTESIAN_POINT('Ctrl Pts',(-0.0110396316109885,-0.0330767512618778,
-0.0116776525866035));
#22794=CARTESIAN_POINT('Ctrl Pts',(-0.0110346690425709,-0.0330759569394036,
-0.0116923722431352));
#22795=CARTESIAN_POINT('Ctrl Pts',(-0.0110315704470788,-0.0330754514572935,
-0.0117018665860989));
#22796=CARTESIAN_POINT('Ctrl Pts',(-0.011011718255126,-0.0330721441819817,
-0.0117647590981194));
#22797=CARTESIAN_POINT('Ctrl Pts',(-0.0109977867187983,-0.0330694856854163,
-0.0118190096687034));
#22798=CARTESIAN_POINT('Ctrl Pts',(-0.0109644113418268,-0.0330615558892467,
-0.0119862633187186));
#22799=CARTESIAN_POINT('Ctrl Pts',(-0.0109545743677489,-0.0330564620125295,
-0.0121007706075571));
#22800=CARTESIAN_POINT('Ctrl Pts',(-0.0109586460915655,-0.0330489090233292,
-0.0122599315010698));
#22801=CARTESIAN_POINT('Ctrl Pts',(-0.010961722743937,-0.0330467476622815,
-0.0123044754470868));
#22802=CARTESIAN_POINT('Ctrl Pts',(-0.0109683424438608,-0.0330438081090372,
-0.0123631557808283));
#22803=CARTESIAN_POINT('Ctrl Pts',(-0.0109701604180367,-0.0330430839848228,
-0.0123774666025577));
#22804=CARTESIAN_POINT('Ctrl Pts',(-0.0109734662095251,-0.0330418875741503,
-0.0124008605179066));
#22805=CARTESIAN_POINT('Ctrl Pts',(-0.0109748351353497,-0.0330414190708893,
-0.0124099596692897));
#22806=CARTESIAN_POINT('Ctrl Pts',(-0.0109776516505458,-0.0330405041262296,
-0.0124276064444926));
#22807=CARTESIAN_POINT('Ctrl Pts',(-0.0109790900548561,-0.0330400579935811,
-0.0124361551964145));
#22808=CARTESIAN_POINT('Ctrl Pts',(-0.0109826421209544,-0.0330390033333457,
-0.0124562305144706));
#22809=CARTESIAN_POINT('Ctrl Pts',(-0.0109848151900985,-0.0330383929267915,
-0.0124677459117464));
#22810=CARTESIAN_POINT('Ctrl Pts',(-0.0109924957788973,-0.0330363440785638,
-0.0125060468579444));
#22811=CARTESIAN_POINT('Ctrl Pts',(-0.0109985839199138,-0.0330348872402636,
-0.0125327095558795));
#22812=CARTESIAN_POINT('Ctrl Pts',(-0.0110309772842716,-0.0330278377748488,
-0.0126590089468896));
#22813=CARTESIAN_POINT('Ctrl Pts',(-0.0110665086202501,-0.0330219547106032,
-0.012755994984683));
#22814=CARTESIAN_POINT('Ctrl Pts',(-0.0111480942304945,-0.0330111915779412,
-0.0129243641307971));
#22815=CARTESIAN_POINT('Ctrl Pts',(-0.0111908820708974,-0.0330063516450282,
-0.0129969074872464));
#22816=CARTESIAN_POINT('Ctrl Pts',(-0.0112476075637781,-0.0330010171067081,
-0.0130772778498566));
#22817=CARTESIAN_POINT('Ctrl Pts',(-0.0112560067434965,-0.0330002510111807,
-0.0130888340442841));
#22818=CARTESIAN_POINT('Ctrl Pts',(-0.0112683549198031,-0.0329991603767217,
-0.0131053366936856));
#22819=CARTESIAN_POINT('Ctrl Pts',(-0.0112721755274159,-0.0329988276816825,
-0.0131103778046844));
#22820=CARTESIAN_POINT('Ctrl Pts',(-0.0112789641621737,-0.0329982450633999,
-0.013119221586375));
#22821=CARTESIAN_POINT('Ctrl Pts',(-0.011281919180256,-0.0329979942562031,
-0.0131230340428408));
#22822=CARTESIAN_POINT('Ctrl Pts',(-0.0112883138634745,-0.032997457549047,
-0.0131312048081595));
#22823=CARTESIAN_POINT('Ctrl Pts',(-0.0112917592084221,-0.0329971720545742,
-0.013135558457285));
#22824=CARTESIAN_POINT('Ctrl Pts',(-0.0113014822670362,-0.0329963762978074,
-0.0131477094739646));
#22825=CARTESIAN_POINT('Ctrl Pts',(-0.0113078125736036,-0.032995869653209,
-0.0131554646153989));
#22826=CARTESIAN_POINT('Ctrl Pts',(-0.0113504464243476,-0.0329925286058322,
-0.0132066691322122));
#22827=CARTESIAN_POINT('Ctrl Pts',(-0.0113890457330661,-0.0329898408982329,
-0.0132481575847098));
#22828=CARTESIAN_POINT('Ctrl Pts',(-0.011514181234861,-0.03298176909845,
-0.013368630062464));
#22829=CARTESIAN_POINT('Ctrl Pts',(-0.0116074853011914,-0.0329765667088619,
-0.013439963034965));
#22830=CARTESIAN_POINT('Ctrl Pts',(-0.0117440273664582,-0.0329689961016864,
-0.013521632071756));
#22831=CARTESIAN_POINT('Ctrl Pts',(-0.0117809579514357,-0.0329669561624363,
-0.0135417205273295));
#22832=CARTESIAN_POINT('Ctrl Pts',(-0.0118313514045219,-0.0329641584066854,
-0.0135665215149725));
#22833=CARTESIAN_POINT('Ctrl Pts',(-0.0118441272053702,-0.0329634480126654,
-0.0135725923194883));
#22834=CARTESIAN_POINT('Ctrl Pts',(-0.0118652944906967,-0.0329622684372074,
-0.0135822961355113));
#22835=CARTESIAN_POINT('Ctrl Pts',(-0.0118736381516352,-0.0329618028283095,
-0.0135860317862855));
#22836=CARTESIAN_POINT('Ctrl Pts',(-0.0118899840936412,-0.032960889206223,
-0.0135931765542023));
#22837=CARTESIAN_POINT('Ctrl Pts',(-0.0118979829868851,-0.0329604414528551,
-0.0135965925880454));
#22838=CARTESIAN_POINT('Ctrl Pts',(-0.011916985876345,-0.0329593759791014,
-0.0136045187317482));
#22839=CARTESIAN_POINT('Ctrl Pts',(-0.011928013867272,-0.0329587562703609,
-0.0136089695679277));
#22840=CARTESIAN_POINT('Ctrl Pts',(-0.0119655619976626,-0.0329566411941367,
-0.0136236213513849));
#22841=CARTESIAN_POINT('Ctrl Pts',(-0.0119923109507173,-0.0329551257665596,
-0.0136332166705206));
#22842=CARTESIAN_POINT('Ctrl Pts',(-0.0120581938271205,-0.0329513713343882,
-0.0136548160656322));
#22843=CARTESIAN_POINT('Ctrl Pts',(-0.0120975685265146,-0.0329491086984023,
-0.013666011709668));
#22844=CARTESIAN_POINT('Ctrl Pts',(-0.0122030850394115,-0.0329430110253012,
-0.0136915266441084));
#22845=CARTESIAN_POINT('Ctrl Pts',(-0.0122698018796857,-0.0329391177373856,
-0.013703083518909));
#22846=CARTESIAN_POINT('Ctrl Pts',(-0.0123438199066056,-0.0329348369247644,
-0.0137109438446322));
#22847=CARTESIAN_POINT('Ctrl Pts',(-0.0123505867931309,-0.0329344459609326,
-0.0137116172453002));
#22848=CARTESIAN_POINT('Ctrl Pts',(-0.0124330278122191,-0.0329296889413775,
-0.0137192712514353));
#22849=CARTESIAN_POINT('Ctrl Pts',(-0.0125091205728446,-0.0329253553718529,
-0.0137206973512007));
#22850=CARTESIAN_POINT('Ctrl Pts',(-0.0125954496246285,-0.0329207106154944,
-0.0137159336742156));
#22851=CARTESIAN_POINT('Ctrl Pts',(-0.0126058792891594,-0.0329201540881409,
-0.0137152518116621));
#22852=CARTESIAN_POINT('Ctrl Pts',(-0.0126219952401571,-0.0329193021375521,
-0.0137140336288337));
#22853=CARTESIAN_POINT('Ctrl Pts',(-0.0126276866447654,-0.0329190028130942,
-0.01371357163749));
#22854=CARTESIAN_POINT('Ctrl Pts',(-0.0126381585326451,-0.0329184550843414,
-0.0137126630568392));
#22855=CARTESIAN_POINT('Ctrl Pts',(-0.0126429395401884,-0.0329182061904306,
-0.0137122257475079));
#22856=CARTESIAN_POINT('Ctrl Pts',(-0.0126538895050607,-0.0329176387833459,
-0.0137111726188893));
#22857=CARTESIAN_POINT('Ctrl Pts',(-0.0126600568555555,-0.0329173211019334,
-0.0137105419317078));
#22858=CARTESIAN_POINT('Ctrl Pts',(-0.0126793686295204,-0.0329163318439331,
-0.013708449385348));
#22859=CARTESIAN_POINT('Ctrl Pts',(-0.0126924984764923,-0.0329156672447565,
-0.0137068556594882));
#22860=CARTESIAN_POINT('Ctrl Pts',(-0.0127608272772352,-0.0329122429023933,
-0.0136976688387602));
#22861=CARTESIAN_POINT('Ctrl Pts',(-0.0128156100796063,-0.0329096135837406,
-0.0136872581774954));
#22862=CARTESIAN_POINT('Ctrl Pts',(-0.0129649152554317,-0.03290249052404,
-0.0136504102436105));
#22863=CARTESIAN_POINT('Ctrl Pts',(-0.0130576593490872,-0.0328981012696692,
-0.0136178938039853));
#22864=CARTESIAN_POINT('Ctrl Pts',(-0.0131958712734373,-0.0328909526596439,
-0.0135540935395386));
#22865=CARTESIAN_POINT('Ctrl Pts',(-0.0132438176649994,-0.0328883517338971,
-0.0135288194993583));
#22866=CARTESIAN_POINT('Ctrl Pts',(-0.0133035606075861,-0.0328848969701308,
-0.0134931901948779));
#22867=CARTESIAN_POINT('Ctrl Pts',(-0.0133166684933199,-0.0328841252425706,
-0.0134851044963859));
#22868=CARTESIAN_POINT('Ctrl Pts',(-0.0133375877116235,-0.0328828702892249,
-0.0134717639288243));
#22869=CARTESIAN_POINT('Ctrl Pts',(-0.0133454759792513,-0.0328823916115646,
-0.0134666313196696));
#22870=CARTESIAN_POINT('Ctrl Pts',(-0.0133604769657345,-0.0328814706014864,
-0.0134566742144954));
#22871=CARTESIAN_POINT('Ctrl Pts',(-0.0133675973107815,-0.0328810287367656,
-0.013451861813306));
#22872=CARTESIAN_POINT('Ctrl Pts',(-0.0133839168246122,-0.0328800049496955,
-0.013440632257663));
#22873=CARTESIAN_POINT('Ctrl Pts',(-0.0133930868912302,-0.0328794214596371,
-0.0134341738316986));
#22874=CARTESIAN_POINT('Ctrl Pts',(-0.0134219964039928,-0.0328775552894878,
-0.0134133378197421));
#22875=CARTESIAN_POINT('Ctrl Pts',(-0.0134414646539318,-0.0328762584115564,
-0.0133985918326946));
#22876=CARTESIAN_POINT('Ctrl Pts',(-0.0135243603918976,-0.0328705572458573,
-0.0133326497747992));
#22877=CARTESIAN_POINT('Ctrl Pts',(-0.0135840185090255,-0.0328659761684123,
-0.0132769406511241));
#22878=CARTESIAN_POINT('Ctrl Pts',(-0.013703765963006,-0.0328558137271099,
-0.0131459127545683));
#22879=CARTESIAN_POINT('Ctrl Pts',(-0.0137617835849164,-0.0328502190270702,
-0.013069145510338));
#22880=CARTESIAN_POINT('Ctrl Pts',(-0.0138250427961349,-0.0328435712401595,
-0.0129668642335203));
#22881=CARTESIAN_POINT('Ctrl Pts',(-0.0138373078725187,-0.0328422512351829,
-0.0129459471180647));
#22882=CARTESIAN_POINT('Ctrl Pts',(-0.0138530011160535,-0.0328405280150102,
-0.0129176769838345));
#22883=CARTESIAN_POINT('Ctrl Pts',(-0.0138568711142915,-0.0328401000875645,
-0.0129105744599875));
#22884=CARTESIAN_POINT('Ctrl Pts',(-0.0138631050811206,-0.0328394062463213,
-0.0128989161292336));
#22885=CARTESIAN_POINT('Ctrl Pts',(-0.0138655024378823,-0.0328391382916245,
-0.0128943784637747));
#22886=CARTESIAN_POINT('Ctrl Pts',(-0.0138701924285461,-0.0328386119678611,
-0.0128853930988605));
#22887=CARTESIAN_POINT('Ctrl Pts',(-0.0138724861399803,-0.0328383535381095,
-0.0128809460697477));
#22888=CARTESIAN_POINT('Ctrl Pts',(-0.0138781587854846,-0.0328377116394678,
-0.0128698154239936));
#22889=CARTESIAN_POINT('Ctrl Pts',(-0.0138815108142272,-0.0328373298260715,
-0.0128631181268945));
#22890=CARTESIAN_POINT('Ctrl Pts',(-0.0138942850700447,-0.0328358639294411,
-0.012837124234716));
#22891=CARTESIAN_POINT('Ctrl Pts',(-0.0139033532252393,-0.0328347999244533,
-0.0128176553858556));
#22892=CARTESIAN_POINT('Ctrl Pts',(-0.013926224460689,-0.0328320357980582,
-0.0127657474880569));
#22893=CARTESIAN_POINT('Ctrl Pts',(-0.0139393278280347,-0.0328303660408524,
-0.0127330130776393));
#22894=CARTESIAN_POINT('Ctrl Pts',(-0.0139917105688196,-0.0328231694238316,
-0.0125879320291054));
#22895=CARTESIAN_POINT('Ctrl Pts',(-0.0140190391198761,-0.0328178951815481,
-0.012471709497576));
#22896=CARTESIAN_POINT('Ctrl Pts',(-0.0140373546116113,-0.0328103457982441,
-0.0123136809524147));
#22897=CARTESIAN_POINT('Ctrl Pts',(-0.0140404158572249,-0.0328084080817642,
-0.0122737018312358));
#22898=CARTESIAN_POINT('Ctrl Pts',(-0.0140423272384866,-0.0328058804702862,
-0.0122227100333379));
#22899=CARTESIAN_POINT('Ctrl Pts',(-0.0140426208761371,-0.0328053347200742,
-0.0122117655427823));
#22900=CARTESIAN_POINT('Ctrl Pts',(-0.0140429326708424,-0.0328043677931774,
-0.0121924976864138));
#22901=CARTESIAN_POINT('Ctrl Pts',(-0.014043,-0.0328039481464066,-0.0121841755036127));
#22902=CARTESIAN_POINT('Ctrl Pts',(-0.014043,-0.0328035263970765,-0.012175853286558));
#22903=CARTESIAN_POINT('Ctrl Pts',(-0.014043,-0.0329194567307744,-0.012175853286558));
#22904=CARTESIAN_POINT('Ctrl Pts',(-0.014043,-0.0329195999341371,-0.0121786026942404));
#22905=CARTESIAN_POINT('Ctrl Pts',(-0.0140429926515305,-0.0329197427213959,
-0.0121813520976706));
#22906=CARTESIAN_POINT('Ctrl Pts',(-0.0140429619707811,-0.0329200399154781,
-0.0121870914667029));
#22907=CARTESIAN_POINT('Ctrl Pts',(-0.0140429372967764,-0.0329201942468374,
-0.0121900813744717));
#22908=CARTESIAN_POINT('Ctrl Pts',(-0.0140428360710219,-0.0329206610219979,
-0.0121991522450127));
#22909=CARTESIAN_POINT('Ctrl Pts',(-0.0140427322590762,-0.0329209719621453,
-0.0122052329173575));
#22910=CARTESIAN_POINT('Ctrl Pts',(-0.0140422594856282,-0.0329220174968526,
-0.0122257998779618));
#22911=CARTESIAN_POINT('Ctrl Pts',(-0.014041722401065,-0.032922743339528,
-0.0122402819253537));
#22912=CARTESIAN_POINT('Ctrl Pts',(-0.0140367797607974,-0.0329275248478707,
-0.0123368139459897));
#22913=CARTESIAN_POINT('Ctrl Pts',(-0.0140260297645205,-0.0329312979608478,
-0.012418414989397));
#22914=CARTESIAN_POINT('Ctrl Pts',(-0.0139871455167143,-0.0329397967123801,
-0.0126000974179127));
#22915=CARTESIAN_POINT('Ctrl Pts',(-0.0139553108782099,-0.0329445061163852,
-0.0126989722561689));
#22916=CARTESIAN_POINT('Ctrl Pts',(-0.0139026943126495,-0.0329508845023387,
-0.0128193344209594));
#22917=CARTESIAN_POINT('Ctrl Pts',(-0.0138908936270081,-0.0329522524208113,
-0.0128444593776491));
#22918=CARTESIAN_POINT('Ctrl Pts',(-0.0138731125759079,-0.0329542358861596,
-0.0128798067357444));
#22919=CARTESIAN_POINT('Ctrl Pts',(-0.013867681949484,-0.0329548323029073,
-0.0128903004013197));
#22920=CARTESIAN_POINT('Ctrl Pts',(-0.0138580377772868,-0.0329558760007039,
-0.0129084229609032));
#22921=CARTESIAN_POINT('Ctrl Pts',(-0.0138538790841758,-0.0329563213172082,
-0.0129160805176271));
#22922=CARTESIAN_POINT('Ctrl Pts',(-0.0138451844818609,-0.0329572429074834,
-0.0129317718132345));
#22923=CARTESIAN_POINT('Ctrl Pts',(-0.0138406409435228,-0.0329577194444046,
-0.0129398009057024));
#22924=CARTESIAN_POINT('Ctrl Pts',(-0.0138288143456409,-0.0329589472875306,
-0.0129602697685481));
#22925=CARTESIAN_POINT('Ctrl Pts',(-0.0138214285801439,-0.0329597023082833,
-0.0129726489133671));
#22926=CARTESIAN_POINT('Ctrl Pts',(-0.013790692239611,-0.032962798411707,
-0.0130225625361672));
#22927=CARTESIAN_POINT('Ctrl Pts',(-0.0137659088770554,-0.032965191816156,
-0.0130591862922433));
#22928=CARTESIAN_POINT('Ctrl Pts',(-0.0136711795036043,-0.0329739867068987,
-0.0131869838270116));
#22929=CARTESIAN_POINT('Ctrl Pts',(-0.0135926801614238,-0.0329806827048526,
-0.0132713401750666));
#22930=CARTESIAN_POINT('Ctrl Pts',(-0.0134630178788468,-0.0329904300486842,
-0.0133827467251288));
#22931=CARTESIAN_POINT('Ctrl Pts',(-0.0134185081556305,-0.0329935791001491,
-0.0134169572659047));
#22932=CARTESIAN_POINT('Ctrl Pts',(-0.013363965201739,-0.0329971253974243,
-0.0134543342323532));
#22933=CARTESIAN_POINT('Ctrl Pts',(-0.0133556446117909,-0.0329976582109083,
-0.0134599178126856));
#22934=CARTESIAN_POINT('Ctrl Pts',(-0.013342616163237,-0.0329984790999736,
-0.0134684777521611));
#22935=CARTESIAN_POINT('Ctrl Pts',(-0.0133379457253415,-0.0329987707303358,
-0.013471510251547));
#22936=CARTESIAN_POINT('Ctrl Pts',(-0.0133291798075773,-0.0329993130076031,
-0.0134771347072217));
#22937=CARTESIAN_POINT('Ctrl Pts',(-0.0133250885276702,-0.0329995640327805,
-0.013479732656352));
#22938=CARTESIAN_POINT('Ctrl Pts',(-0.0133155927122235,-0.0330001419785699,
-0.0134856998750939));
#22939=CARTESIAN_POINT('Ctrl Pts',(-0.0133101794889474,-0.0330004679770742,
-0.0134890550060902));
#22940=CARTESIAN_POINT('Ctrl Pts',(-0.0132924250257821,-0.0330015264303756,
-0.0134999077007458));
#22941=CARTESIAN_POINT('Ctrl Pts',(-0.0132799989623827,-0.0330022503496351,
-0.0135072657546555));
#22942=CARTESIAN_POINT('Ctrl Pts',(-0.0132005855368806,-0.0330067824600841,
-0.0135527966970516));
#22943=CARTESIAN_POINT('Ctrl Pts',(-0.0131309130594329,-0.0330103411939344,
-0.0135860817231761));
#22944=CARTESIAN_POINT('Ctrl Pts',(-0.012994618020904,-0.0330170381419621,
-0.0136390617723327));
#22945=CARTESIAN_POINT('Ctrl Pts',(-0.012928588319169,-0.0330201747633333,
-0.0136597460937967));
#22946=CARTESIAN_POINT('Ctrl Pts',(-0.0128226904031785,-0.0330252666629476,
-0.0136852588003124));
#22947=CARTESIAN_POINT('Ctrl Pts',(-0.0127836398937354,-0.0330271561274909,
-0.0136930817626132));
#22948=CARTESIAN_POINT('Ctrl Pts',(-0.0127168092452417,-0.0330304420367926,
-0.0137037995368402));
#22949=CARTESIAN_POINT('Ctrl Pts',(-0.0126891729729697,-0.0330318156964838,
-0.0137074666382348));
#22950=CARTESIAN_POINT('Ctrl Pts',(-0.0126496834413369,-0.0330338060527694,
-0.0137116214774584));
#22951=CARTESIAN_POINT('Ctrl Pts',(-0.0126378997052687,-0.0330344034310928,
-0.0137127243709459));
#22952=CARTESIAN_POINT('Ctrl Pts',(-0.0126174166645416,-0.0330354482528905,
-0.0137144040057708));
#22953=CARTESIAN_POINT('Ctrl Pts',(-0.012608722916222,-0.033035893719385,
-0.0137150427849832));
#22954=CARTESIAN_POINT('Ctrl Pts',(-0.0125908251323664,-0.0330368150930682,
-0.013716205446885));
#22955=CARTESIAN_POINT('Ctrl Pts',(-0.01258162089507,-0.0330372912578075,
-0.0137167205770884));
#22956=CARTESIAN_POINT('Ctrl Pts',(-0.0125580461718774,-0.0330385170193999,
-0.013717828155152));
#22957=CARTESIAN_POINT('Ctrl Pts',(-0.0125436712294385,-0.0330392703064992,
-0.013718302202476));
#22958=CARTESIAN_POINT('Ctrl Pts',(-0.0124853957293894,-0.033042348631409,
-0.0137194086951833));
#22959=CARTESIAN_POINT('Ctrl Pts',(-0.0124414871536661,-0.0330447252279825,
-0.0137183682182671));
#22960=CARTESIAN_POINT('Ctrl Pts',(-0.0122827748385063,-0.0330535163660108,
-0.0137078209683911));
#22961=CARTESIAN_POINT('Ctrl Pts',(-0.0121690868453822,-0.033060228775654,
-0.0136873436842773));
#22962=CARTESIAN_POINT('Ctrl Pts',(-0.0120049295896913,-0.0330699971878748,
-0.0136383543126339));
#22963=CARTESIAN_POINT('Ctrl Pts',(-0.0119520183292706,-0.0330731508227526,
-0.0136193633028095));
#22964=CARTESIAN_POINT('Ctrl Pts',(-0.0118910220392996,-0.0330767014860323,
-0.0135936315833082));
#22965=CARTESIAN_POINT('Ctrl Pts',(-0.0118818253204101,-0.0330772344536998,
-0.0135896458920154));
#22966=CARTESIAN_POINT('Ctrl Pts',(-0.011867579849828,-0.0330780555274094,
-0.0135833065781637));
#22967=CARTESIAN_POINT('Ctrl Pts',(-0.0118625040576128,-0.0330783471907059,
-0.0135810148216686));
#22968=CARTESIAN_POINT('Ctrl Pts',(-0.0118530345009027,-0.0330788894950169,
-0.0135766773764606));
#22969=CARTESIAN_POINT('Ctrl Pts',(-0.0118486379596951,-0.0330791405147342,
-0.0135746384668961));
#22970=CARTESIAN_POINT('Ctrl Pts',(-0.01183848705678,-0.0330797184050798,
-0.0135698727164946));
#22971=CARTESIAN_POINT('Ctrl Pts',(-0.0118327398934341,-0.0330800443542148,
-0.0135671309360713));
#22972=CARTESIAN_POINT('Ctrl Pts',(-0.0118140207415016,-0.0330811024748431,
-0.0135580579771797));
#22973=CARTESIAN_POINT('Ctrl Pts',(-0.011801120249478,-0.0330818261182355,
-0.0135515801753165));
#22974=CARTESIAN_POINT('Ctrl Pts',(-0.0117198965951304,-0.0330863584258906,
-0.0135093573960194));
#22975=CARTESIAN_POINT('Ctrl Pts',(-0.0116542362045179,-0.0330899175452863,
-0.013468710748643));
#22976=CARTESIAN_POINT('Ctrl Pts',(-0.0115360069820772,-0.0330966148742783,
-0.0133826438735455));
#22977=CARTESIAN_POINT('Ctrl Pts',(-0.0114829253133027,-0.0330997514956493,
-0.0133382580750814));
#22978=CARTESIAN_POINT('Ctrl Pts',(-0.0114042395231014,-0.0331048433952636,
-0.0132629333565266));
#22979=CARTESIAN_POINT('Ctrl Pts',(-0.0113765573810259,-0.033106732859807,
-0.0132343005076058));
#22980=CARTESIAN_POINT('Ctrl Pts',(-0.0113314294628993,-0.033110018769109,
-0.0131838557133378));
#22981=CARTESIAN_POINT('Ctrl Pts',(-0.0113134115642216,-0.0331113924288003,
-0.0131625821028058));
#22982=CARTESIAN_POINT('Ctrl Pts',(-0.0112885788147417,-0.033113382785086,
-0.0131315979076253));
#22983=CARTESIAN_POINT('Ctrl Pts',(-0.011281283895528,-0.0331139801634094,
-0.0131222781992908));
#22984=CARTESIAN_POINT('Ctrl Pts',(-0.0112688033457407,-0.0331150249852071,
-0.0131059499413432));
#22985=CARTESIAN_POINT('Ctrl Pts',(-0.0112635685145531,-0.0331154704517016,
-0.0130989795868927));
#22986=CARTESIAN_POINT('Ctrl Pts',(-0.0112529198203433,-0.0331163918253848,
-0.0130845474089121));
#22987=CARTESIAN_POINT('Ctrl Pts',(-0.011247513213227,-0.0331168679901241,
-0.0130770806865507));
#22988=CARTESIAN_POINT('Ctrl Pts',(-0.0112338435624034,-0.0331180937517165,
-0.0130578417949739));
#22989=CARTESIAN_POINT('Ctrl Pts',(-0.0112256777408025,-0.0331188470388158,
-0.0130460019027213));
#22990=CARTESIAN_POINT('Ctrl Pts',(-0.0111932598222739,-0.0331219253637252,
-0.0129975629020136));
#22991=CARTESIAN_POINT('Ctrl Pts',(-0.0111704111002564,-0.0331243019602983,
-0.0129600531497367));
#22992=CARTESIAN_POINT('Ctrl Pts',(-0.0110935323815902,-0.0331330930983265,
-0.0128208033523248));
#22993=CARTESIAN_POINT('Ctrl Pts',(-0.0110493365457318,-0.03313980550797,
-0.0127140746915099));
#22994=CARTESIAN_POINT('Ctrl Pts',(-0.0110018636076939,-0.0331495739201912,
-0.0125494724944212));
#22995=CARTESIAN_POINT('Ctrl Pts',(-0.010989255406508,-0.0331527275550691,
-0.0124946884347279));
#22996=CARTESIAN_POINT('Ctrl Pts',(-0.0109779508597921,-0.0331562782183488,
-0.0124294590241645));
#22997=CARTESIAN_POINT('Ctrl Pts',(-0.0109763356030537,-0.0331568111860163,
-0.0124195667888718));
#22998=CARTESIAN_POINT('Ctrl Pts',(-0.0109739729479484,-0.033157632259726,
-0.012404154514767));
#22999=CARTESIAN_POINT('Ctrl Pts',(-0.0109731588811264,-0.0331579239230225,
-0.0123986451491363));
#23000=CARTESIAN_POINT('Ctrl Pts',(-0.0109716921962995,-0.0331584662273335,
-0.0123883332739022));
#23001=CARTESIAN_POINT('Ctrl Pts',(-0.0109710323735861,-0.0331587172470508,
-0.0123835320906325));
#23002=CARTESIAN_POINT('Ctrl Pts',(-0.010969557954751,-0.0331592951373964,
-0.0123724154681247));
#23003=CARTESIAN_POINT('Ctrl Pts',(-0.0109687598191304,-0.0331596210865314,
-0.012366098014053));
#23004=CARTESIAN_POINT('Ctrl Pts',(-0.0109662802579694,-0.0331606792071597,
-0.0123454442732641));
#23005=CARTESIAN_POINT('Ctrl Pts',(-0.0109647608413423,-0.0331614028505521,
-0.0123310889263665));
#23006=CARTESIAN_POINT('Ctrl Pts',(-0.0109564039104447,-0.0331659351582133,
-0.0122399285904424));
#23007=CARTESIAN_POINT('Ctrl Pts',(-0.0109551297071341,-0.0331694942776144,
-0.0121627158112966));
#23008=CARTESIAN_POINT('Ctrl Pts',(-0.010963671607677,-0.0331761916066194,
-0.0120167271403392));
#23009=CARTESIAN_POINT('Ctrl Pts',(-0.0109723401835273,-0.0331793282279981,
-0.0119480786262911));
#23010=CARTESIAN_POINT('Ctrl Pts',(-0.0109932086416718,-0.0331844201276134,
-0.0118411685039492));
#23011=CARTESIAN_POINT('Ctrl Pts',(-0.0110023452679362,-0.0331863095921493,
-0.0118024043055921));
#23012=CARTESIAN_POINT('Ctrl Pts',(-0.0110204097744286,-0.0331895955014393,
-0.0117371748656594));
#23013=CARTESIAN_POINT('Ctrl Pts',(-0.011028575540593,-0.0331909691611265,
-0.0117105190701174));
#23014=CARTESIAN_POINT('Ctrl Pts',(-0.0110412303003652,-0.0331929595174073,
-0.0116728820823938));
#23015=CARTESIAN_POINT('Ctrl Pts',(-0.0110451309990397,-0.03319355689573,
-0.0116617081234135));
#23016=CARTESIAN_POINT('Ctrl Pts',(-0.0110521273049904,-0.0331946017175269,
-0.0116423838424964));
#23017=CARTESIAN_POINT('Ctrl Pts',(-0.0110551641887478,-0.0331950471840213,
-0.0116342127571505));
#23018=CARTESIAN_POINT('Ctrl Pts',(-0.0110615547780563,-0.0331959685577046,
-0.0116174543915371));
#23019=CARTESIAN_POINT('Ctrl Pts',(-0.0110649165262468,-0.0331964447224443,
-0.0116088705699796));
#23020=CARTESIAN_POINT('Ctrl Pts',(-0.0110737195480242,-0.0331976704840381,
-0.0115869730561571));
#23021=CARTESIAN_POINT('Ctrl Pts',(-0.0110792703383311,-0.0331984237711386,
-0.0115737045815427));
#23022=CARTESIAN_POINT('Ctrl Pts',(-0.011102514379402,-0.0332015020960607,
-0.0115202539237943));
#23023=CARTESIAN_POINT('Ctrl Pts',(-0.0111217321636346,-0.0332038786926459,
-0.0114807606028172));
#23024=CARTESIAN_POINT('Ctrl Pts',(-0.01119736777905,-0.0332126698306768,
-0.0113408317024874));
#23025=CARTESIAN_POINT('Ctrl Pts',(-0.0112632968571075,-0.0332193822403086,
-0.0112459758351642));
#23026=CARTESIAN_POINT('Ctrl Pts',(-0.0113761538947043,-0.0332291506525148,
-0.011117092740428));
#23027=CARTESIAN_POINT('Ctrl Pts',(-0.0114154404776327,-0.0332323042873894,
-0.0110768829862725));
#23028=CARTESIAN_POINT('Ctrl Pts',(-0.0114642208455187,-0.0332358549506661,
-0.011032126484172));
#23029=CARTESIAN_POINT('Ctrl Pts',(-0.011471672085274,-0.0332363879183335,
-0.0110254224257381));
#23030=CARTESIAN_POINT('Ctrl Pts',(-0.0114833644229151,-0.033237208992043,
-0.0110151069241687));
#23031=CARTESIAN_POINT('Ctrl Pts',(-0.0114875605180411,-0.0332375006553395,
-0.0110114451486249));
#23032=CARTESIAN_POINT('Ctrl Pts',(-0.0114954451454344,-0.0332380429596505,
-0.0110046393726883));
#23033=CARTESIAN_POINT('Ctrl Pts',(-0.0114991286688594,-0.0332382939793677,
-0.0110014900264106));
#23034=CARTESIAN_POINT('Ctrl Pts',(-0.0115076862849315,-0.0332388718697134,
-0.0109942429294712));
#23035=CARTESIAN_POINT('Ctrl Pts',(-0.0115125709667679,-0.0332391978188484,
-0.0109901579411259));
#23036=CARTESIAN_POINT('Ctrl Pts',(-0.0115286106547145,-0.0332402559394769,
-0.0109769120495777));
#23037=CARTESIAN_POINT('Ctrl Pts',(-0.0115398692343731,-0.0332409795828695,
-0.0109678771729534));
#23038=CARTESIAN_POINT('Ctrl Pts',(-0.0116120622211135,-0.0332455118905934,
-0.0109115902469658));
#23039=CARTESIAN_POINT('Ctrl Pts',(-0.0116763456830407,-0.0332490710100485,
-0.0108687992014549));
#23040=CARTESIAN_POINT('Ctrl Pts',(-0.0118038054591141,-0.033255768339187,
-0.0107971077621977));
#23041=CARTESIAN_POINT('Ctrl Pts',(-0.0118662545682228,-0.0332589049606438,
-0.010767310586225));
#23042=CARTESIAN_POINT('Ctrl Pts',(-0.0119674912369483,-0.0332639968602696,
-0.0107271060627891));
#23043=CARTESIAN_POINT('Ctrl Pts',(-0.0120050466006367,-0.0332658863247279,
-0.0107138495347917));
#23044=CARTESIAN_POINT('Ctrl Pts',(-0.0120696953875809,-0.0332691722338961,
-0.0106938060764293));
#23045=CARTESIAN_POINT('Ctrl Pts',(-0.0120965373776007,-0.0332705458935413,
-0.0106862748948614));
#23046=CARTESIAN_POINT('Ctrl Pts',(-0.0121350451156411,-0.0332725362497718,
-0.0106765877993376));
#23047=CARTESIAN_POINT('Ctrl Pts',(-0.0121465552086665,-0.0332731336280875,
-0.0106738327014075));
#23048=CARTESIAN_POINT('Ctrl Pts',(-0.0121665961081347,-0.0332741784498762,
-0.010669278750204));
#23049=CARTESIAN_POINT('Ctrl Pts',(-0.0121751126573689,-0.0332746239163695,
-0.0106674192644108));
#23050=CARTESIAN_POINT('Ctrl Pts',(-0.0121926671517927,-0.0332755452900544,
-0.0106637420132362));
#23051=CARTESIAN_POINT('Ctrl Pts',(-0.0122017065321154,-0.0332760214547967,
-0.0106619328842395));
#23052=CARTESIAN_POINT('Ctrl Pts',(-0.0122248889067874,-0.0332772472164056,
-0.0106575088790393));
#23053=CARTESIAN_POINT('Ctrl Pts',(-0.0122390530250158,-0.0332780005035187,
-0.0106550105889884));
#23054=CARTESIAN_POINT('Ctrl Pts',(-0.0122965889274273,-0.0332810788285701,
-0.0106456897266794));
#23055=CARTESIAN_POINT('Ctrl Pts',(-0.0123402047784401,-0.0332834554252774,
-0.0106405221968228));
#23056=CARTESIAN_POINT('Ctrl Pts',(-0.0124988168744899,-0.0332922465633352,
-0.0106285619925034));
#23057=CARTESIAN_POINT('Ctrl Pts',(-0.0126142570046326,-0.0332989589728471,
-0.0106327874828199));
#23058=CARTESIAN_POINT('Ctrl Pts',(-0.0127836855395962,-0.0333087273849002,
-0.0106581159980292));
#23059=CARTESIAN_POINT('Ctrl Pts',(-0.0128387476170901,-0.033311881019742,
-0.010669448583193));
#23060=CARTESIAN_POINT('Ctrl Pts',(-0.0129027652163431,-0.0333154316829873,
-0.0106863132112805));
#23061=CARTESIAN_POINT('Ctrl Pts',(-0.0129124324335934,-0.0333159646506537,
-0.0106889609052973));
#23062=CARTESIAN_POINT('Ctrl Pts',(-0.0129274300654441,-0.0333167857243618,
-0.0106932260395573));
#23063=CARTESIAN_POINT('Ctrl Pts',(-0.0129327785176059,-0.0333170773876581,
-0.0106947784164003));
#23064=CARTESIAN_POINT('Ctrl Pts',(-0.0129427654904171,-0.0333176196919689,
-0.0106977358323721));
#23065=CARTESIAN_POINT('Ctrl Pts',(-0.012947405803118,-0.0333178707116862,
-0.0106991337682948));
#23066=CARTESIAN_POINT('Ctrl Pts',(-0.0129581277551387,-0.0333184486020322,
-0.0107024190311331));
#23067=CARTESIAN_POINT('Ctrl Pts',(-0.0129642043768496,-0.0333187745511676,
-0.0107043221640999));
#23068=CARTESIAN_POINT('Ctrl Pts',(-0.0129840167495783,-0.0333198326717984,
-0.0107106621263353));
#23069=CARTESIAN_POINT('Ctrl Pts',(-0.0129977024153552,-0.033320556315193,
-0.0107152542026567));
#23070=CARTESIAN_POINT('Ctrl Pts',(-0.0130840725614564,-0.033325088623549,
-0.0107455897523201));
#23071=CARTESIAN_POINT('Ctrl Pts',(-0.0131548127864189,-0.0333286477435496,
-0.0107765616686534));
#23072=CARTESIAN_POINT('Ctrl Pts',(-0.0132840065245436,-0.0333353450740348,
-0.0108450791390976));
#23073=CARTESIAN_POINT('Ctrl Pts',(-0.0133428217329245,-0.0333384816962801,
-0.0108815282347096));
#23074=CARTESIAN_POINT('Ctrl Pts',(-0.013431351664073,-0.0333435735960127,
-0.0109449925399469));
#23075=CARTESIAN_POINT('Ctrl Pts',(-0.0134627981096062,-0.0333454630596884,
-0.0109694314546625));
#23076=CARTESIAN_POINT('Ctrl Pts',(-0.0135145943704972,-0.0333487489676268,
-0.0110130015095112));
#23077=CARTESIAN_POINT('Ctrl Pts',(-0.0135354345954656,-0.0333501226268487,
-0.011031518951365));
#23078=CARTESIAN_POINT('Ctrl Pts',(-0.0135643920696066,-0.0333521129825711,
-0.0110586878597246));
#23079=CARTESIAN_POINT('Ctrl Pts',(-0.0135729294094318,-0.0333527103608161,
-0.0110668846030151));
#23080=CARTESIAN_POINT('Ctrl Pts',(-0.0135875897039654,-0.0333537551825219,
-0.0110812877907902));
#23081=CARTESIAN_POINT('Ctrl Pts',(-0.0135937559755411,-0.0333542006490042,
-0.0110874494779754));
#23082=CARTESIAN_POINT('Ctrl Pts',(-0.0136063351284224,-0.0333551220227048,
-0.0111002341317816));
#23083=CARTESIAN_POINT('Ctrl Pts',(-0.0136127415179121,-0.0333555981874744,
-0.0111068629723535));
#23084=CARTESIAN_POINT('Ctrl Pts',(-0.0136289898413118,-0.0333568239492358,
-0.0111239798190084));
#23085=CARTESIAN_POINT('Ctrl Pts',(-0.0136387450853462,-0.0333575772364759,
-0.0111345485928338));
#23086=CARTESIAN_POINT('Ctrl Pts',(-0.0136776755201077,-0.0333606555628316,
-0.0111779269587674));
#23087=CARTESIAN_POINT('Ctrl Pts',(-0.0137055899193784,-0.0333630321607721,
-0.0112118361621427));
#23088=CARTESIAN_POINT('Ctrl Pts',(-0.0138013537393381,-0.0333718232991008,
-0.0113388406291071));
#23089=CARTESIAN_POINT('Ctrl Pts',(-0.0138601715899953,-0.0333785357074034,
-0.0114382626285861));
#23090=CARTESIAN_POINT('Ctrl Pts',(-0.0139304024462809,-0.0333883041179107,
-0.011594516204129));
#23091=CARTESIAN_POINT('Ctrl Pts',(-0.0139506170570479,-0.0333914577524209,
-0.0116469721736676));
#23092=CARTESIAN_POINT('Ctrl Pts',(-0.0139710154015459,-0.0333950084153505,
-0.0117099529283649));
#23093=CARTESIAN_POINT('Ctrl Pts',(-0.0139740107524153,-0.0333955413830057,
-0.0117195181383488));
#23094=CARTESIAN_POINT('Ctrl Pts',(-0.0139785251593245,-0.0333963624567005,
-0.0117344426300953));
#23095=CARTESIAN_POINT('Ctrl Pts',(-0.0139801087098747,-0.0333966541199944,
-0.0117397819354392));
#23096=CARTESIAN_POINT('Ctrl Pts',(-0.0139830162074801,-0.0333971964243033,
-0.0117497835549122));
#23097=CARTESIAN_POINT('Ctrl Pts',(-0.013984347099905,-0.0333974474440209,
-0.0117544435390592));
#23098=CARTESIAN_POINT('Ctrl Pts',(-0.0139873758422689,-0.033398025334371,
-0.0117652407576162));
#23099=CARTESIAN_POINT('Ctrl Pts',(-0.0139890576808882,-0.03339835128351,
-0.0117713823100489));
#23100=CARTESIAN_POINT('Ctrl Pts',(-0.0139944276440985,-0.0333994094041648,
-0.0117914792936379));
#23101=CARTESIAN_POINT('Ctrl Pts',(-0.0139979580720056,-0.0334001330475793,
-0.0118054764613262));
#23102=CARTESIAN_POINT('Ctrl Pts',(-0.0140190984339713,-0.0334046653624545,
-0.0118945447325097));
#23103=CARTESIAN_POINT('Ctrl Pts',(-0.0140312582910716,-0.0334082244880811,
-0.0119708047959815));
#23104=CARTESIAN_POINT('Ctrl Pts',(-0.0140412213047356,-0.033413716519899,
-0.012090310517274));
#23105=CARTESIAN_POINT('Ctrl Pts',(-0.0140430000004635,-0.0334156645237435,
-0.0121330785747856));
#23106=CARTESIAN_POINT('Ctrl Pts',(-0.014043,-0.033417632014157,-0.012175853303277));
#23107=CARTESIAN_POINT('Origin',(-0.0125,-0.0375520664398416,-0.0121758532865581));
#23108=CARTESIAN_POINT('',(-0.014043,-0.0339165738369763,-0.0121758532867271));
#23109=CARTESIAN_POINT('',(-0.014043,-0.0338009094848242,-0.0121758532862401));
#23110=CARTESIAN_POINT('',(-0.014043,-0.0375520664398416,-0.012175853286558));
#23111=CARTESIAN_POINT('Ctrl Pts',(-0.014043,-0.0338009094848242,-0.0121758532859222));
#23112=CARTESIAN_POINT('Ctrl Pts',(-0.0140429999999882,-0.0337993161421864,
-0.0121472447835339));
#23113=CARTESIAN_POINT('Ctrl Pts',(-0.0140422043596351,-0.0337977478260463,
-0.0121186389603028));
#23114=CARTESIAN_POINT('Ctrl Pts',(-0.0140401034932399,-0.0337957263984264,
-0.012080909112732));
#23115=CARTESIAN_POINT('Ctrl Pts',(-0.0140395117507698,-0.0337952395588485,
-0.0120717536068128));
#23116=CARTESIAN_POINT('Ctrl Pts',(-0.0140384442002407,-0.0337944746419083,
-0.0120572477009742));
#23117=CARTESIAN_POINT('Ctrl Pts',(-0.014038022063108,-0.0337941937084367,
-0.012051893707222));
#23118=CARTESIAN_POINT('Ctrl Pts',(-0.0140371635832908,-0.0337936608885854,
-0.0120416859828794));
#23119=CARTESIAN_POINT('Ctrl Pts',(-0.0140367321926341,-0.0337934087472843,
-0.0120368320093285));
#23120=CARTESIAN_POINT('Ctrl Pts',(-0.0140356448539427,-0.0337928084291541,
-0.0120252214066319));
#23121=CARTESIAN_POINT('Ctrl Pts',(-0.0140349672922442,-0.0337924614498812,
-0.0120184668330488));
#23122=CARTESIAN_POINT('Ctrl Pts',(-0.0140324774597902,-0.0337912730439428,
-0.011995193433061));
#23123=CARTESIAN_POINT('Ctrl Pts',(-0.0140304428741404,-0.0337904432043666,
-0.0119786990361259));
#23124=CARTESIAN_POINT('Ctrl Pts',(-0.0140247383311923,-0.0337884139433801,
-0.0119378899774222));
#23125=CARTESIAN_POINT('Ctrl Pts',(-0.0140207528468879,-0.0337872283690468,
-0.0119136236248547));
#23126=CARTESIAN_POINT('Ctrl Pts',(-0.0140002426252975,-0.0337819784027302,
-0.0118050401417757));
#23127=CARTESIAN_POINT('Ctrl Pts',(-0.0139772724781112,-0.0337781107988135,
-0.0117220935218472));
#23128=CARTESIAN_POINT('Ctrl Pts',(-0.0139165116455943,-0.0337700608211633,
-0.011557501856301));
#23129=CARTESIAN_POINT('Ctrl Pts',(-0.0138782597787381,-0.0337658833867196,
-0.0114763810169881));
#23130=CARTESIAN_POINT('Ctrl Pts',(-0.0138247317664289,-0.033760621247134,
-0.0113845143151584));
#23131=CARTESIAN_POINT('Ctrl Pts',(-0.0138160316133676,-0.0337597811589592,
-0.0113701285287535));
#23132=CARTESIAN_POINT('Ctrl Pts',(-0.0138018848947561,-0.0337584372151351,
-0.0113475773850191));
#23133=CARTESIAN_POINT('Ctrl Pts',(-0.0137965923750887,-0.0337579390498095,
-0.0113393167031883));
#23134=CARTESIAN_POINT('Ctrl Pts',(-0.0137865544843974,-0.0337570024904676,
-0.0113239734654));
#23135=CARTESIAN_POINT('Ctrl Pts',(-0.0137818284774537,-0.0337565648356068,
-0.011316878652754));
#23136=CARTESIAN_POINT('Ctrl Pts',(-0.0137711240412606,-0.0337555806628813,
-0.0113010939356291));
#23137=CARTESIAN_POINT('Ctrl Pts',(-0.013765114847874,-0.0337550329841646,
-0.0112924254940682));
#23138=CARTESIAN_POINT('Ctrl Pts',(-0.0137469589305725,-0.0337533920624747,
-0.0112668002152122));
#23139=CARTESIAN_POINT('Ctrl Pts',(-0.0137345570805766,-0.0337522890333457,
-0.0112500278071728));
#23140=CARTESIAN_POINT('Ctrl Pts',(-0.013674332877356,-0.0337470129602141,
-0.0111719423609822));
#23141=CARTESIAN_POINT('Ctrl Pts',(-0.0136222660851279,-0.0337426732782518,
-0.0111140571079612));
#23142=CARTESIAN_POINT('Ctrl Pts',(-0.0135079316199637,-0.0337336529532164,
-0.0110047901133805));
#23143=CARTESIAN_POINT('Ctrl Pts',(-0.0134455451123945,-0.0337289797791893,
-0.0109538633562121));
#23144=CARTESIAN_POINT('Ctrl Pts',(-0.013341928536635,-0.0337218379014151,
-0.0108819856786954));
#23145=CARTESIAN_POINT('Ctrl Pts',(-0.013303240966222,-0.0337192938699135,
-0.0108576189863246));
#23146=CARTESIAN_POINT('Ctrl Pts',(-0.0132550454566685,-0.0337163205427813,
-0.0108301747966004));
#23147=CARTESIAN_POINT('Ctrl Pts',(-0.0132465190733556,-0.0337158017197733,
-0.010825426123517));
#23148=CARTESIAN_POINT('Ctrl Pts',(-0.0132330693701639,-0.0337149952521195,
-0.0108181017783727));
#23149=CARTESIAN_POINT('Ctrl Pts',(-0.0132281763531113,-0.0337147043097953,
-0.0108154713327942));
#23150=CARTESIAN_POINT('Ctrl Pts',(-0.013219436461792,-0.0337141891326061,
-0.010810833505208));
#23151=CARTESIAN_POINT('Ctrl Pts',(-0.0132155952971133,-0.0337139642644757,
-0.0108088159069703));
#23152=CARTESIAN_POINT('Ctrl Pts',(-0.0132062916312206,-0.0337134232949145,
-0.0108039790516885));
#23153=CARTESIAN_POINT('Ctrl Pts',(-0.0132008207429022,-0.0337131082220881,
-0.0108011762068581));
#23154=CARTESIAN_POINT('Ctrl Pts',(-0.0131837748718316,-0.0337121354963773,
-0.0107925714782024));
#23155=CARTESIAN_POINT('Ctrl Pts',(-0.0131721432418526,-0.0337114844918601,
-0.0107868824013671));
#23156=CARTESIAN_POINT('Ctrl Pts',(-0.0131122926196203,-0.0337081927678809,
-0.0107585371619461));
#23157=CARTESIAN_POINT('Ctrl Pts',(-0.013062991426041,-0.0337056715322415,
-0.0107382410928924));
#23158=CARTESIAN_POINT('Ctrl Pts',(-0.0129225442086121,-0.0336987596843853,
-0.0106887589465888));
#23159=CARTESIAN_POINT('Ctrl Pts',(-0.0128295948403706,-0.0336944792739199,
-0.010665435800378));
#23160=CARTESIAN_POINT('Ctrl Pts',(-0.0126769219728509,-0.0336872558351469,
-0.0106419006425537));
#23161=CARTESIAN_POINT('Ctrl Pts',(-0.0126183004437683,-0.0336844409819132,
-0.010636270161355));
#23162=CARTESIAN_POINT('Ctrl Pts',(-0.0125437949286773,-0.0336807405292667,
-0.0106333948137545));
#23163=CARTESIAN_POINT('Ctrl Pts',(-0.0125280780996695,-0.0336799532024085,
-0.0106330286907548));
#23164=CARTESIAN_POINT('Ctrl Pts',(-0.0125028790765382,-0.0336786790296563,
-0.0106328268508412));
#23165=CARTESIAN_POINT('Ctrl Pts',(-0.0124933990256157,-0.0336781969945015,
-0.0106328382858915));
#23166=CARTESIAN_POINT('Ctrl Pts',(-0.0124753438588177,-0.0336772736084814,
-0.0106330264557832));
#23167=CARTESIAN_POINT('Ctrl Pts',(-0.012466768913629,-0.0336768327744806,
-0.0106331873324422));
#23168=CARTESIAN_POINT('Ctrl Pts',(-0.0124471215681905,-0.0336758173059761,
-0.0106337198287589));
#23169=CARTESIAN_POINT('Ctrl Pts',(-0.0124360510243703,-0.0336752411879286,
-0.0106341392241955));
#23170=CARTESIAN_POINT('Ctrl Pts',(-0.0124013558395995,-0.0336734229251345,
-0.0106358279478391));
#23171=CARTESIAN_POINT('Ctrl Pts',(-0.0123777560685275,-0.0336721675905996,
-0.0106375213809762));
#23172=CARTESIAN_POINT('Ctrl Pts',(-0.0123223978071859,-0.0336691783284451,
-0.0106427755658311));
#23173=CARTESIAN_POINT('Ctrl Pts',(-0.012290693300643,-0.0336674315300226,
-0.0106467815580481));
#23174=CARTESIAN_POINT('Ctrl Pts',(-0.0121666504603399,-0.033660466405645,
-0.0106663849836567));
#23175=CARTESIAN_POINT('Ctrl Pts',(-0.0120756920903544,-0.0336550565078558,
-0.010689388851595));
#23176=CARTESIAN_POINT('Ctrl Pts',(-0.0119187425037636,-0.0336455029100956,
-0.0107446699532416));
#23177=CARTESIAN_POINT('Ctrl Pts',(-0.0118518857586418,-0.0336413623995634,
-0.0107736778824404));
#23178=CARTESIAN_POINT('Ctrl Pts',(-0.0117780852797928,-0.0336368928693253,
-0.0108121096941789));
#23179=CARTESIAN_POINT('Ctrl Pts',(-0.0117688974356628,-0.033636338385576,
-0.0108170131557909));
#23180=CARTESIAN_POINT('Ctrl Pts',(-0.0117547569759684,-0.0336354888936514,
-0.0108247447252493));
#23181=CARTESIAN_POINT('Ctrl Pts',(-0.0117497693724786,-0.0336351900180373,
-0.0108275078126939));
#23182=CARTESIAN_POINT('Ctrl Pts',(-0.0117406097014453,-0.0336346427005868,
-0.0108326487479675));
#23183=CARTESIAN_POINT('Ctrl Pts',(-0.0117364333805626,-0.0336343937747531,
-0.0108350184434727));
#23184=CARTESIAN_POINT('Ctrl Pts',(-0.0117268808787237,-0.0336338257764111,
-0.0108404977555914));
#23185=CARTESIAN_POINT('Ctrl Pts',(-0.0117215123532047,-0.0336335075426844,
-0.0108436203654327));
#23186=CARTESIAN_POINT('Ctrl Pts',(-0.0117047199848925,-0.0336325147617991,
-0.0108535238358687));
#23187=CARTESIAN_POINT('Ctrl Pts',(-0.0116933644961017,-0.0336318472632097,
-0.0108604200253056));
#23188=CARTESIAN_POINT('Ctrl Pts',(-0.01163440278987,-0.0336283941404489,
-0.0108972781421191));
#23189=CARTESIAN_POINT('Ctrl Pts',(-0.0115883683270542,-0.0336257413791545,
-0.010929682483491));
#23190=CARTESIAN_POINT('Ctrl Pts',(-0.0114667999306948,-0.0336185718693533,
-0.0110256063226618));
#23191=CARTESIAN_POINT('Ctrl Pts',(-0.0113954298323821,-0.0336141583269674,
-0.0110939588575385));
#23192=CARTESIAN_POINT('Ctrl Pts',(-0.0112963589614724,-0.0336070240749296,
-0.0112089382003157));
#23193=CARTESIAN_POINT('Ctrl Pts',(-0.0112637572688373,-0.0336044686101761,
-0.0112509858663945));
#23194=CARTESIAN_POINT('Ctrl Pts',(-0.0112246463162661,-0.0336010667294697,
-0.0113072011642105));
#23195=CARTESIAN_POINT('Ctrl Pts',(-0.0112160880000167,-0.0336002992132186,
-0.0113199014869486));
#23196=CARTESIAN_POINT('Ctrl Pts',(-0.0112025881226012,-0.0335990494464454,
-0.0113405930649407));
#23197=CARTESIAN_POINT('Ctrl Pts',(-0.0111975279256079,-0.0335985716741744,
-0.011348505894139));
#23198=CARTESIAN_POINT('Ctrl Pts',(-0.0111879737939721,-0.033597651277201,
-0.0113637509633083));
#23199=CARTESIAN_POINT('Ctrl Pts',(-0.0111834682876219,-0.033597209106703,
-0.0113710755563534));
#23200=CARTESIAN_POINT('Ctrl Pts',(-0.0111732076750668,-0.0335961829393702,
-0.011388072983773));
#23201=CARTESIAN_POINT('Ctrl Pts',(-0.0111674967588407,-0.0335955973507975,
-0.011397771811267));
#23202=CARTESIAN_POINT('Ctrl Pts',(-0.0111496234025559,-0.0335937173847962,
-0.0114289000305843));
#23203=CARTESIAN_POINT('Ctrl Pts',(-0.0111378683530392,-0.0335924085121383,
-0.0114505578961369));
#23204=CARTESIAN_POINT('Ctrl Pts',(-0.0110785156272132,-0.0335853981118196,
-0.0115664474891109));
#23205=CARTESIAN_POINT('Ctrl Pts',(-0.0110401697666802,-0.0335793807025071,
-0.0116650860648329));
#23206=CARTESIAN_POINT('Ctrl Pts',(-0.0109895189172441,-0.0335683883686168,
-0.011849335361499));
#23207=CARTESIAN_POINT('Ctrl Pts',(-0.0109737405501886,-0.0335634594430176,
-0.0119335698749898));
#23208=CARTESIAN_POINT('Ctrl Pts',(-0.0109635742156463,-0.0335580475888531,
-0.0120328573633552));
#23209=CARTESIAN_POINT('Ctrl Pts',(-0.0109623191989988,-0.0335572834824804,
-0.0120470518599872));
#23210=CARTESIAN_POINT('Ctrl Pts',(-0.0109607916799848,-0.0335561951365938,
-0.0120675635152863));
#23211=CARTESIAN_POINT('Ctrl Pts',(-0.0109603611184368,-0.0335558627866068,
-0.0120738677773221));
#23212=CARTESIAN_POINT('Ctrl Pts',(-0.010959670238414,-0.0335552805549607,
-0.0120849880868));
#23213=CARTESIAN_POINT('Ctrl Pts',(-0.0109593937543555,-0.033555029793311,
-0.0120898029700394));
#23214=CARTESIAN_POINT('Ctrl Pts',(-0.0109588473426091,-0.0335544929317273,
-0.0121001673960661));
#23215=CARTESIAN_POINT('Ctrl Pts',(-0.0109585848083938,-0.0335542072400902,
-0.0121057171591305));
#23216=CARTESIAN_POINT('Ctrl Pts',(-0.0109579324790847,-0.0335534103551736,
-0.0121212883021568));
#23217=CARTESIAN_POINT('Ctrl Pts',(-0.0109576103939953,-0.0335529027961535,
-0.0121313124070385));
#23218=CARTESIAN_POINT('Ctrl Pts',(-0.0109561078014767,-0.0335495345987556,
-0.0121984710539084));
#23219=CARTESIAN_POINT('Ctrl Pts',(-0.0109580043126801,-0.0335468234182701,
-0.0122556353169623));
#23220=CARTESIAN_POINT('Ctrl Pts',(-0.0109736621619191,-0.033538615021032,
-0.0124316602842457));
#23221=CARTESIAN_POINT('Ctrl Pts',(-0.0109980610362408,-0.0335333044598007,
-0.012549115392993));
#23222=CARTESIAN_POINT('Ctrl Pts',(-0.0110482585049746,-0.0335257098401372,
-0.0127001253793906));
#23223=CARTESIAN_POINT('Ctrl Pts',(-0.0110621786177751,-0.0335237848857979,
-0.0127371766791065));
#23224=CARTESIAN_POINT('Ctrl Pts',(-0.0110828785354006,-0.0335211215997775,
-0.0127864333521761));
#23225=CARTESIAN_POINT('Ctrl Pts',(-0.0110884224630571,-0.0335204248252831,
-0.0127991430291343));
#23226=CARTESIAN_POINT('Ctrl Pts',(-0.0110978801888293,-0.0335192619159308,
-0.0128200516521546));
#23227=CARTESIAN_POINT('Ctrl Pts',(-0.0111016965060982,-0.0335187991489379,
-0.0128282939608061));
#23228=CARTESIAN_POINT('Ctrl Pts',(-0.0111093233170813,-0.0335178865973378,
-0.0128443916800384));
#23229=CARTESIAN_POINT('Ctrl Pts',(-0.0111131281551799,-0.0335174370223177,
-0.0128522493996618));
#23230=CARTESIAN_POINT('Ctrl Pts',(-0.0111223562120245,-0.0335163597694635,
-0.0128709018638421));
#23231=CARTESIAN_POINT('Ctrl Pts',(-0.0111278398653843,-0.0335157299835402,
-0.0128816659281876));
#23232=CARTESIAN_POINT('Ctrl Pts',(-0.0111471980251655,-0.0335135411948309,
-0.0129185863769873));
#23233=CARTESIAN_POINT('Ctrl Pts',(-0.0111616979969911,-0.0335119601906147,
-0.0129444059604938));
#23234=CARTESIAN_POINT('Ctrl Pts',(-0.0111992267583206,-0.0335080038670154,
-0.0130069462784028));
#23235=CARTESIAN_POINT('Ctrl Pts',(-0.0112230761605314,-0.0335056014448284,
-0.0130431431185843));
#23236=CARTESIAN_POINT('Ctrl Pts',(-0.0112861775452646,-0.0334995236535978,
-0.0131306584133039));
#23237=CARTESIAN_POINT('Ctrl Pts',(-0.011327187965282,-0.0334958054491696,
-0.0131806065012802));
#23238=CARTESIAN_POINT('Ctrl Pts',(-0.0113876125062547,-0.0334907088480056,
-0.013245443063642));
#23239=CARTESIAN_POINT('Ctrl Pts',(-0.0114044308269542,-0.0334893267526076,
-0.0132626635002469));
#23240=CARTESIAN_POINT('Ctrl Pts',(-0.0114632168773144,-0.0334846341095007,
-0.013320103218506));
#23241=CARTESIAN_POINT('Ctrl Pts',(-0.0115070543606992,-0.0334813641346384,
-0.013358345275774));
#23242=CARTESIAN_POINT('Ctrl Pts',(-0.0115610136486099,-0.0334776949471436,
-0.0134002951954203));
#23243=CARTESIAN_POINT('Ctrl Pts',(-0.0115691408846366,-0.033477151274234,
-0.0134064851058104));
#23244=CARTESIAN_POINT('Ctrl Pts',(-0.0115818638775508,-0.0334763148016256,
-0.0134159770986217));
#23245=CARTESIAN_POINT('Ctrl Pts',(-0.0115864171951332,-0.0334760183111638,
-0.0134193352804976));
#23246=CARTESIAN_POINT('Ctrl Pts',(-0.0115948731107472,-0.0334754731476334,
-0.0134255002047708));
#23247=CARTESIAN_POINT('Ctrl Pts',(-0.0115987703768681,-0.0334752240205868,
-0.0134283137741033));
#23248=CARTESIAN_POINT('Ctrl Pts',(-0.0116077829487013,-0.0334746527395366,
-0.0134347564069586));
#23249=CARTESIAN_POINT('Ctrl Pts',(-0.0116129072875935,-0.0334743314629325,
-0.0134383725360855));
#23250=CARTESIAN_POINT('Ctrl Pts',(-0.0116292245495253,-0.0334733191286818,
-0.0134497388606907));
#23251=CARTESIAN_POINT('Ctrl Pts',(-0.0116404983402653,-0.0334726355212428,
-0.0134573724093256));
#23252=CARTESIAN_POINT('Ctrl Pts',(-0.0117013853385578,-0.0334690191951031,
-0.0134974343621052));
#23253=CARTESIAN_POINT('Ctrl Pts',(-0.0117527390760291,-0.0334662335974016,
-0.0135271357213447));
#23254=CARTESIAN_POINT('Ctrl Pts',(-0.0118955823028583,-0.0334588454306064,
-0.0135991112142569));
#23255=CARTESIAN_POINT('Ctrl Pts',(-0.0119897014924633,-0.033454335838558,
-0.0136355037320265));
#23256=CARTESIAN_POINT('Ctrl Pts',(-0.0121334190071866,-0.0334472899210698,
-0.0136754596367959));
#23257=CARTESIAN_POINT('Ctrl Pts',(-0.0121807256702241,-0.0334449496763278,
-0.013686238728406));
#23258=CARTESIAN_POINT('Ctrl Pts',(-0.0122430792972829,-0.0334417997756893,
-0.0136973858494454));
#23259=CARTESIAN_POINT('Ctrl Pts',(-0.012257736323028,-0.0334410548115421,
-0.0136997882847579));
#23260=CARTESIAN_POINT('Ctrl Pts',(-0.0122816167292075,-0.0334398327984506,
-0.0137033493112696));
#23261=CARTESIAN_POINT('Ctrl Pts',(-0.0122908200834134,-0.0334393598608983,
-0.0137046368278112));
#23262=CARTESIAN_POINT('Ctrl Pts',(-0.0123085933590506,-0.0334384425120381,
-0.0137069597509572));
#23263=CARTESIAN_POINT('Ctrl Pts',(-0.0123171614571464,-0.0334379984809096,
-0.0137080065330458));
#23264=CARTESIAN_POINT('Ctrl Pts',(-0.0123371456877173,-0.0334369584764007,
-0.0137102780305097));
#23265=CARTESIAN_POINT('Ctrl Pts',(-0.0123485675025721,-0.0334363607718203,
-0.0137114473120011));
#23266=CARTESIAN_POINT('Ctrl Pts',(-0.0123858296028133,-0.0334343997161618,
-0.0137148421654574));
#23267=CARTESIAN_POINT('Ctrl Pts',(-0.012411712177496,-0.0334330200571125,
-0.0137165436510788));
#23268=CARTESIAN_POINT('Ctrl Pts',(-0.0125237778463481,-0.0334269691166154,
-0.0137210776039364));
#23269=CARTESIAN_POINT('Ctrl Pts',(-0.0126100616949541,-0.0334221009520264,
-0.0137173352890856));
#23270=CARTESIAN_POINT('Ctrl Pts',(-0.0127992737083723,-0.0334111566346289,
-0.0136931581157646));
#23271=CARTESIAN_POINT('Ctrl Pts',(-0.0129013654514121,-0.0334050681875574,
-0.0136694016889682));
#23272=CARTESIAN_POINT('Ctrl Pts',(-0.0130127642015683,-0.0333986984259702,
-0.013631221352361));
#23273=CARTESIAN_POINT('Ctrl Pts',(-0.0130251994520558,-0.0333979916904246,
-0.0136267801943549));
#23274=CARTESIAN_POINT('Ctrl Pts',(-0.0130433836875074,-0.0333969662000074,
-0.0136200214033853));
#23275=CARTESIAN_POINT('Ctrl Pts',(-0.0130491778632807,-0.0333966406420563,
-0.0136178279945866));
#23276=CARTESIAN_POINT('Ctrl Pts',(-0.0130594382125888,-0.033396066486081,
-0.0136138730823058));
#23277=CARTESIAN_POINT('Ctrl Pts',(-0.0130639095641964,-0.0333958170813107,
-0.0136121255629249));
#23278=CARTESIAN_POINT('Ctrl Pts',(-0.0130736842136804,-0.0333952736610276,
-0.0136082526938462));
#23279=CARTESIAN_POINT('Ctrl Pts',(-0.0130789839112385,-0.0333949801621741,
-0.0136061187414957));
#23280=CARTESIAN_POINT('Ctrl Pts',(-0.0130942414297293,-0.0333941381531118,
-0.0135998765151017));
#23281=CARTESIAN_POINT('Ctrl Pts',(-0.0131041684233866,-0.0333935939679268,
-0.0135956932637267));
#23282=CARTESIAN_POINT('Ctrl Pts',(-0.013191282834957,-0.0333888440155744,
-0.0135579040065656));
#23283=CARTESIAN_POINT('Ctrl Pts',(-0.0132656523958536,-0.033384962121768,
-0.0135181333250506));
#23284=CARTESIAN_POINT('Ctrl Pts',(-0.013435825044743,-0.0333756910891636,
-0.0134083612398965));
#23285=CARTESIAN_POINT('Ctrl Pts',(-0.0135275244517434,-0.033370332225433,
-0.0133330203761054));
#23286=CARTESIAN_POINT('Ctrl Pts',(-0.0136239922957768,-0.0333635114639151,
-0.0132331671162951));
#23287=CARTESIAN_POINT('Ctrl Pts',(-0.0136379720976605,-0.0333624902858058,
-0.0132181059769125));
#23288=CARTESIAN_POINT('Ctrl Pts',(-0.0136587149173031,-0.0333609218855837,
-0.0131948437363644));
#23289=CARTESIAN_POINT('Ctrl Pts',(-0.013665701103049,-0.0333603840753491,
-0.0131868442496253));
#23290=CARTESIAN_POINT('Ctrl Pts',(-0.0136781483644111,-0.0333594080830567,
-0.013172291037784));
#23291=CARTESIAN_POINT('Ctrl Pts',(-0.0136836387638517,-0.0333589711435588,
-0.0131657628952886));
#23292=CARTESIAN_POINT('Ctrl Pts',(-0.0136952932600395,-0.0333580295591694,
-0.0131516699898979));
#23293=CARTESIAN_POINT('Ctrl Pts',(-0.0137014402686912,-0.0333575242451902,
-0.0131440916306087));
#23294=CARTESIAN_POINT('Ctrl Pts',(-0.0137181078465028,-0.0333561297419265,
-0.0131231398295445));
#23295=CARTESIAN_POINT('Ctrl Pts',(-0.0137284795161363,-0.0333552346712883,
-0.0131096501420463));
#23296=CARTESIAN_POINT('Ctrl Pts',(-0.0138016805908148,-0.0333487143003003,
-0.013011112033157));
#23297=CARTESIAN_POINT('Ctrl Pts',(-0.0138558340513196,-0.0333427500414317,
-0.0129199884605444));
#23298=CARTESIAN_POINT('Ctrl Pts',(-0.0139416967924835,-0.0333310089665558,
-0.0127345099440163));
#23299=CARTESIAN_POINT('Ctrl Pts',(-0.0139744683273538,-0.0333252803615069,
-0.0126411837191641));
#23300=CARTESIAN_POINT('Ctrl Pts',(-0.0140010448289976,-0.0333192715551104,
-0.0125334345461984));
#23301=CARTESIAN_POINT('Ctrl Pts',(-0.0140038444429358,-0.0333186127660152,
-0.012521471349666));
#23302=CARTESIAN_POINT('Ctrl Pts',(-0.0140078237389314,-0.0333176370673577,
-0.0125035024901238));
#23303=CARTESIAN_POINT('Ctrl Pts',(-0.0140091110093342,-0.0333173145791908,
-0.0124975214265061));
#23304=CARTESIAN_POINT('Ctrl Pts',(-0.0140113681965968,-0.0333167365986814,
-0.0124867219553947));
#23305=CARTESIAN_POINT('Ctrl Pts',(-0.014012350729376,-0.0333164804067694,
-0.0124819062695477));
#23306=CARTESIAN_POINT('Ctrl Pts',(-0.014014320135465,-0.0333159573369494,
-0.0124720125107152));
#23307=CARTESIAN_POINT('Ctrl Pts',(-0.0140153045087452,-0.0333156905993573,
-0.0124669340417576));
#23308=CARTESIAN_POINT('Ctrl Pts',(-0.0140177971545341,-0.0333150008298448,
-0.0124537188587988));
#23309=CARTESIAN_POINT('Ctrl Pts',(-0.0140192655620973,-0.0333145800056606,
-0.01244557469135));
#23310=CARTESIAN_POINT('Ctrl Pts',(-0.0140254881224478,-0.0333127280474943,
-0.0124093984920448));
#23311=CARTESIAN_POINT('Ctrl Pts',(-0.0140295327235197,-0.0333113330052668,
-0.0123812485367736));
#23312=CARTESIAN_POINT('Ctrl Pts',(-0.0140390255558211,-0.0333073550934322,
-0.0122991105353976));
#23313=CARTESIAN_POINT('Ctrl Pts',(-0.014042407755512,-0.0333048456618236,
-0.012244925585549));
#23314=CARTESIAN_POINT('Ctrl Pts',(-0.0140429762849904,-0.0333021306885963,
-0.0121857322010147));
#23315=CARTESIAN_POINT('Ctrl Pts',(-0.0140430000000311,-0.0333019043280856,
-0.0121807923972907));
#23316=CARTESIAN_POINT('Ctrl Pts',(-0.014043,-0.033301678145883,-0.0121758532768531));
#23317=CARTESIAN_POINT('Ctrl Pts',(-0.014043,-0.033417632014157,-0.012175853303277));
#23318=CARTESIAN_POINT('Ctrl Pts',(-0.014042999999715,-0.0334188419092182,
-0.0122021573362673));
#23319=CARTESIAN_POINT('Ctrl Pts',(-0.0140423273793937,-0.0334200590347099,
-0.0122284638982962));
#23320=CARTESIAN_POINT('Ctrl Pts',(-0.0140389460965616,-0.0334231503636634,
-0.0122945082372041));
#23321=CARTESIAN_POINT('Ctrl Pts',(-0.0140353724136637,-0.033425039819269,
-0.0123341737634836));
#23322=CARTESIAN_POINT('Ctrl Pts',(-0.0140266957573011,-0.0334283257145249,
-0.0124012996251137));
#23323=CARTESIAN_POINT('Ctrl Pts',(-0.0140223741544198,-0.0334296993693816,
-0.0124288410353687));
#23324=CARTESIAN_POINT('Ctrl Pts',(-0.0140151584755546,-0.0334316897198655,
-0.0124678872954614));
#23325=CARTESIAN_POINT('Ctrl Pts',(-0.0140128740083621,-0.0334322870973805,
-0.0124794999449829));
#23326=CARTESIAN_POINT('Ctrl Pts',(-0.014008675324236,-0.0334333319182327,
-0.0124996182548541));
#23327=CARTESIAN_POINT('Ctrl Pts',(-0.0140068221732928,-0.0334337773846008,
-0.0125081361819942));
#23328=CARTESIAN_POINT('Ctrl Pts',(-0.0140028609645677,-0.033434698758464,
-0.0125256287913865));
#23329=CARTESIAN_POINT('Ctrl Pts',(-0.0140007444563308,-0.0334351749235147,
-0.0125346011847215));
#23330=CARTESIAN_POINT('Ctrl Pts',(-0.01399512033785,-0.0334364006868484,
-0.012557522029801));
#23331=CARTESIAN_POINT('Ctrl Pts',(-0.0139914979243137,-0.0334371539753981,
-0.0125714411744428));
#23332=CARTESIAN_POINT('Ctrl Pts',(-0.0139760309415478,-0.0334402323152038,
-0.012627637821355));
#23333=CARTESIAN_POINT('Ctrl Pts',(-0.0139625798505904,-0.0334426089258601,
-0.0126694485361724));
#23334=CARTESIAN_POINT('Ctrl Pts',(-0.0139074519912897,-0.033451400066983,
-0.0128186523112334));
#23335=CARTESIAN_POINT('Ctrl Pts',(-0.0138555717064292,-0.0334581124628146,
-0.0129218640318063));
#23336=CARTESIAN_POINT('Ctrl Pts',(-0.0137620362154178,-0.033467880857382,
-0.0130653860550227));
#23337=CARTESIAN_POINT('Ctrl Pts',(-0.0137288184927417,-0.0334710344884734,
-0.0131107384041683));
#23338=CARTESIAN_POINT('Ctrl Pts',(-0.0136868438010502,-0.0334745851481467,
-0.0131619320091844));
#23339=CARTESIAN_POINT('Ctrl Pts',(-0.0136804134221039,-0.033475118115687,
-0.0131696206731239));
#23340=CARTESIAN_POINT('Ctrl Pts',(-0.0136702941516215,-0.0334759391892443,
-0.0131814832448776));
#23341=CARTESIAN_POINT('Ctrl Pts',(-0.0136666569165708,-0.0334762308525137,
-0.0131857006291432));
#23342=CARTESIAN_POINT('Ctrl Pts',(-0.0136598118447903,-0.0334767731568024,
-0.0131935511653801));
#23343=CARTESIAN_POINT('Ctrl Pts',(-0.0136566097213111,-0.0334770241765241,
-0.013197188902726));
#23344=CARTESIAN_POINT('Ctrl Pts',(-0.0136491606889585,-0.0334776020669154,
-0.0132055713334287));
#23345=CARTESIAN_POINT('Ctrl Pts',(-0.0136449014955317,-0.0334779280160911,
-0.0132103048868706));
#23346=CARTESIAN_POINT('Ctrl Pts',(-0.013630892009917,-0.0334789861369936,
-0.0132256821354219));
#23347=CARTESIAN_POINT('Ctrl Pts',(-0.0136210213926637,-0.0334797097806135,
-0.0132362156847351));
#23348=CARTESIAN_POINT('Ctrl Pts',(-0.0135574948811643,-0.0334842421627514,
-0.013302130046507));
#23349=CARTESIAN_POINT('Ctrl Pts',(-0.0134998936434749,-0.0334878013464259,
-0.0133535670668619));
#23350=CARTESIAN_POINT('Ctrl Pts',(-0.0133838259435214,-0.033494498834056,
-0.013442533214749));
#23351=CARTESIAN_POINT('Ctrl Pts',(-0.0133262059647764,-0.033497635548298,
-0.0134808474604466));
#23352=CARTESIAN_POINT('Ctrl Pts',(-0.0132316572462242,-0.0335027274604619,
-0.0135349381301696));
#23353=CARTESIAN_POINT('Ctrl Pts',(-0.0131963507202493,-0.0335046168328217,
-0.0135533616709764));
#23354=CARTESIAN_POINT('Ctrl Pts',(-0.0131351809564327,-0.0335079025972543,
-0.0135823279884092));
#23355=CARTESIAN_POINT('Ctrl Pts',(-0.0131096716356768,-0.0335092762070825,
-0.0135935719861557));
#23356=CARTESIAN_POINT('Ctrl Pts',(-0.0130729178359096,-0.0335112665035286,
-0.0136085968847154));
#23357=CARTESIAN_POINT('Ctrl Pts',(-0.013061912006056,-0.0335118638735136,
-0.013612948952185));
#23358=CARTESIAN_POINT('Ctrl Pts',(-0.0130427147053381,-0.0335129086855603,
-0.0136202859560935));
#23359=CARTESIAN_POINT('Ctrl Pts',(-0.0130345459058136,-0.0335133541507502,
-0.0136233289024706));
#23360=CARTESIAN_POINT('Ctrl Pts',(-0.0130176861602339,-0.0335142755262911,
-0.0136294471167212));
#23361=CARTESIAN_POINT('Ctrl Pts',(-0.0130089925738914,-0.0335147516942412,
-0.0136325140357905));
#23362=CARTESIAN_POINT('Ctrl Pts',(-0.0129866664023287,-0.033515977473795,
-0.0136401659834561));
#23363=CARTESIAN_POINT('Ctrl Pts',(-0.0129729964467952,-0.0335167307758543,
-0.0136446385682866));
#23364=CARTESIAN_POINT('Ctrl Pts',(-0.0129173494210471,-0.0335198092544095,
-0.0136619879616927));
#23365=CARTESIAN_POINT('Ctrl Pts',(-0.012874897064272,-0.0335221859962418,
-0.0136732605412862));
#23366=CARTESIAN_POINT('Ctrl Pts',(-0.0127195607234908,-0.0335309771661923,
-0.0137074877957652));
#23367=CARTESIAN_POINT('Ctrl Pts',(-0.0126046823233424,-0.03353768943338,
-0.0137195980135792));
#23368=CARTESIAN_POINT('Ctrl Pts',(-0.0124333780789518,-0.033547457663513,
-0.0137184372899149));
#23369=CARTESIAN_POINT('Ctrl Pts',(-0.012377268351593,-0.0335506112593318,
-0.0137149900401518));
#23370=CARTESIAN_POINT('Ctrl Pts',(-0.0123115119429668,-0.0335541618854092,
-0.0137073302557702));
#23371=CARTESIAN_POINT('Ctrl Pts',(-0.0123015678167686,-0.0335546948517647,
-0.0137060735758977));
#23372=CARTESIAN_POINT('Ctrl Pts',(-0.012286118348364,-0.0335555159239032,
-0.013703968024865));
#23373=CARTESIAN_POINT('Ctrl Pts',(-0.0122806043327708,-0.0335558075869195,
-0.013703186111275));
#23374=CARTESIAN_POINT('Ctrl Pts',(-0.0122702999158708,-0.0335563498910004,
-0.0137016679408443));
#23375=CARTESIAN_POINT('Ctrl Pts',(-0.0122655087430625,-0.033556600910764,
-0.0137009389689751));
#23376=CARTESIAN_POINT('Ctrl Pts',(-0.0122544304169177,-0.0335571788015811,
-0.0136991999723327));
#23377=CARTESIAN_POINT('Ctrl Pts',(-0.0122481459999849,-0.033557504751136,
-0.0136981735914326));
#23378=CARTESIAN_POINT('Ctrl Pts',(-0.012227637051582,-0.0335585628745932,
-0.0136946935597877));
#23379=CARTESIAN_POINT('Ctrl Pts',(-0.0122134401913984,-0.0335592865203315,
-0.0136920791455995));
#23380=CARTESIAN_POINT('Ctrl Pts',(-0.0121236375502395,-0.0335638196053332,
-0.0136742351652825));
#23381=CARTESIAN_POINT('Ctrl Pts',(-0.012049219097992,-0.0335673793955917,
-0.0136535527859177));
#23382=CARTESIAN_POINT('Ctrl Pts',(-0.0119116147336543,-0.0335740783763959,
-0.0136039400287943));
#23383=CARTESIAN_POINT('Ctrl Pts',(-0.0118482257695319,-0.0335772159632486,
-0.0135761457803177));
#23384=CARTESIAN_POINT('Ctrl Pts',(-0.0117516281924312,-0.033582307991978,
-0.0135258058932876));
#23385=CARTESIAN_POINT('Ctrl Pts',(-0.0117170666046765,-0.0335841964967042,
-0.0135060590744796));
#23386=CARTESIAN_POINT('Ctrl Pts',(-0.0116596674613333,-0.0335874808975805,
-0.0134702514521083));
#23387=CARTESIAN_POINT('Ctrl Pts',(-0.0116364315437997,-0.0335888540380433,
-0.0134548664953536));
#23388=CARTESIAN_POINT('Ctrl Pts',(-0.0116039396891384,-0.0335908437712065,
-0.013432063836645));
#23389=CARTESIAN_POINT('Ctrl Pts',(-0.0115943323557847,-0.0335914410626901,
-0.0134251551456082));
#23390=CARTESIAN_POINT('Ctrl Pts',(-0.0115777875821499,-0.0335924857829406,
-0.0134129665554057));
#23391=CARTESIAN_POINT('Ctrl Pts',(-0.0115708135968848,-0.0335929312358514,
-0.0134077370504474));
#23392=CARTESIAN_POINT('Ctrl Pts',(-0.011556555650037,-0.0335938526288993,
-0.0133968556421665));
#23393=CARTESIAN_POINT('Ctrl Pts',(-0.0115492772959708,-0.0335943288270915,
-0.0133911969947188));
#23394=CARTESIAN_POINT('Ctrl Pts',(-0.011530772971779,-0.0335955547758169,
-0.013376542632161));
#23395=CARTESIAN_POINT('Ctrl Pts',(-0.0115196214679203,-0.033596308218779,
-0.0133674546677911));
#23396=CARTESIAN_POINT('Ctrl Pts',(-0.0114749355659099,-0.0335993881443212,
-0.0133299858017371));
#23397=CARTESIAN_POINT('Ctrl Pts',(-0.0114424956041238,-0.0336017662541618,
-0.0133003366754625));
#23398=CARTESIAN_POINT('Ctrl Pts',(-0.0113297703865931,-0.033610557725176,
-0.0131881123875606));
#23399=CARTESIAN_POINT('Ctrl Pts',(-0.0112575279296278,-0.0336172686512803,
-0.0130980051100665));
#23400=CARTESIAN_POINT('Ctrl Pts',(-0.0111659648444407,-0.0336270351665792,
-0.0129532549765209));
#23401=CARTESIAN_POINT('Ctrl Pts',(-0.0111385523345016,-0.0336301883940965,
-0.0129041832623619));
#23402=CARTESIAN_POINT('Ctrl Pts',(-0.0111094718289135,-0.0336337386693752,
-0.012844718636034));
#23403=CARTESIAN_POINT('Ctrl Pts',(-0.0111051564731134,-0.0336342716233584,
-0.0128356721982252));
#23404=CARTESIAN_POINT('Ctrl Pts',(-0.0110985808396488,-0.0336350926806802,
-0.0128215345940113));
#23405=CARTESIAN_POINT('Ctrl Pts',(-0.011096259536667,-0.0336353843410538,
-0.0128164723054101));
#23406=CARTESIAN_POINT('Ctrl Pts',(-0.0110919694629843,-0.0336359266429641,
-0.0128069812409461));
#23407=CARTESIAN_POINT('Ctrl Pts',(-0.0110899941459429,-0.0336361776631654,
-0.0128025557517783));
#23408=CARTESIAN_POINT('Ctrl Pts',(-0.011085471687265,-0.0336367555584293,
-0.0127922940368988));
#23409=CARTESIAN_POINT('Ctrl Pts',(-0.0110829397880767,-0.0336370815119439,
-0.0127864512760361));
#23410=CARTESIAN_POINT('Ctrl Pts',(-0.0110747867227164,-0.0336381396620814,
-0.0127673129036136));
#23411=CARTESIAN_POINT('Ctrl Pts',(-0.011069315795437,-0.0336388633299439,
-0.0127539537098811));
#23412=CARTESIAN_POINT('Ctrl Pts',(-0.0110357453120358,-0.0336434051251161,
-0.0126685826950959));
#23413=CARTESIAN_POINT('Ctrl Pts',(-0.0110129004208285,-0.0336469724342582,
-0.0125946147937823));
#23414=CARTESIAN_POINT('Ctrl Pts',(-0.0109802591867677,-0.0336536893025543,
-0.0124516204862864));
#23415=CARTESIAN_POINT('Ctrl Pts',(-0.0109694007204777,-0.0336568370952115,
-0.0123830374474221));
#23416=CARTESIAN_POINT('Ctrl Pts',(-0.0109578583589872,-0.033662867374927,
-0.0122545964123853));
#23417=CARTESIAN_POINT('Ctrl Pts',(-0.0109559680881269,-0.0336657191615092,
-0.0121949800949101));
#23418=CARTESIAN_POINT('Ctrl Pts',(-0.0109579320381111,-0.0336694409500641,
-0.0121200821823339));
#23419=CARTESIAN_POINT('Ctrl Pts',(-0.0109585622387561,-0.0336702092552543,
-0.0121047644549504));
#23420=CARTESIAN_POINT('Ctrl Pts',(-0.0109599480973457,-0.0336714613173229,
-0.0120800518813177));
#23421=CARTESIAN_POINT('Ctrl Pts',(-0.0109605617835608,-0.0336719405977302,
-0.0120706499372031));
#23422=CARTESIAN_POINT('Ctrl Pts',(-0.0109619032267775,-0.0336728646172739,
-0.0120526381640575));
#23423=CARTESIAN_POINT('Ctrl Pts',(-0.0109626172731864,-0.0336733089064685,
-0.0120440276538187));
#23424=CARTESIAN_POINT('Ctrl Pts',(-0.0109644173049838,-0.0336743312285039,
-0.0120243315010868));
#23425=CARTESIAN_POINT('Ctrl Pts',(-0.0109655510803624,-0.0336749107517826,
-0.0120132507990589));
#23426=CARTESIAN_POINT('Ctrl Pts',(-0.0109689077681384,-0.033676472640218,
-0.0119836172109057));
#23427=CARTESIAN_POINT('Ctrl Pts',(-0.0109713478369917,-0.0336774617790287,
-0.0119650912064516));
#23428=CARTESIAN_POINT('Ctrl Pts',(-0.0109802070646319,-0.0336806516392054,
-0.0119061217256684));
#23429=CARTESIAN_POINT('Ctrl Pts',(-0.0109878995051436,-0.0336828908783642,
-0.0118658897870954));
#23430=CARTESIAN_POINT('Ctrl Pts',(-0.0110217486329495,-0.0336912025163248,
-0.0117204829739705));
#23431=CARTESIAN_POINT('Ctrl Pts',(-0.0110573619899019,-0.0336975190679095,
-0.011617837821735));
#23432=CARTESIAN_POINT('Ctrl Pts',(-0.0111191447161997,-0.033705797005906,
-0.0114863212448241));
#23433=CARTESIAN_POINT('Ctrl Pts',(-0.0111360622430286,-0.033707880701205,
-0.0114534338591265));
#23434=CARTESIAN_POINT('Ctrl Pts',(-0.0111650056310049,-0.0337111391680469,
-0.0114018170668279));
#23435=CARTESIAN_POINT('Ctrl Pts',(-0.0111762829698282,-0.0337123441092489,
-0.0113826853612786));
#23436=CARTESIAN_POINT('Ctrl Pts',(-0.0111919706851298,-0.0337139297716866,
-0.01135733871569));
#23437=CARTESIAN_POINT('Ctrl Pts',(-0.011196019296504,-0.0337143313642452,
-0.0113509041239544));
#23438=CARTESIAN_POINT('Ctrl Pts',(-0.0112028318730518,-0.033714994229264,
-0.0113402521433342));
#23439=CARTESIAN_POINT('Ctrl Pts',(-0.0112055692184076,-0.0337152572033376,
-0.0113360179612292));
#23440=CARTESIAN_POINT('Ctrl Pts',(-0.0112108000905011,-0.0337157532663478,
-0.0113280130731278));
#23441=CARTESIAN_POINT('Ctrl Pts',(-0.0112132895094078,-0.0337159866332001,
-0.0113242397893671));
#23442=CARTESIAN_POINT('Ctrl Pts',(-0.0112199471104154,-0.0337166037288225,
-0.0113142445091727));
#23443=CARTESIAN_POINT('Ctrl Pts',(-0.0112241441189503,-0.0337169855559622,
-0.0113080417513844));
#23444=CARTESIAN_POINT('Ctrl Pts',(-0.011239550772152,-0.0337183622793037,
-0.0112856256413522));
#23445=CARTESIAN_POINT('Ctrl Pts',(-0.0112510260667238,-0.0337193406966561,
-0.0112695963154988));
#23446=CARTESIAN_POINT('Ctrl Pts',(-0.0113224235834729,-0.033725179398347,
-0.0111737974155291));
#23447=CARTESIAN_POINT('Ctrl Pts',(-0.011389664513514,-0.0337296656966443,
-0.0110997673076007));
#23448=CARTESIAN_POINT('Ctrl Pts',(-0.0115345618938466,-0.0337386231585147,
-0.0109683946848047));
#23449=CARTESIAN_POINT('Ctrl Pts',(-0.0116113687685034,-0.0337430724518835,
-0.0109108003156418));
#23450=CARTESIAN_POINT('Ctrl Pts',(-0.0117074261725664,-0.0337486513555158,
-0.0108518586884018));
#23451=CARTESIAN_POINT('Ctrl Pts',(-0.0117219836650929,-0.0337494966413229,
-0.0108432522502181));
#23452=CARTESIAN_POINT('Ctrl Pts',(-0.0117451627903961,-0.0337508435852963,
-0.0108300579543876));
#23453=CARTESIAN_POINT('Ctrl Pts',(-0.0117536917629376,-0.0337513394191275,
-0.0108253095817266));
#23454=CARTESIAN_POINT('Ctrl Pts',(-0.0117697934074394,-0.0337522761326918,
-0.0108165443434453));
#23455=CARTESIAN_POINT('Ctrl Pts',(-0.0117773556368542,-0.0337527163268646,
-0.0108125090192861));
#23456=CARTESIAN_POINT('Ctrl Pts',(-0.0117944535217119,-0.0337537123320167,
-0.0108035675436729));
#23457=CARTESIAN_POINT('Ctrl Pts',(-0.0118040074254927,-0.0337542693933093,
-0.0107986974052046));
#23458=CARTESIAN_POINT('Ctrl Pts',(-0.0118329753618903,-0.0337559602952649,
-0.0107843093200875));
#23459=CARTESIAN_POINT('Ctrl Pts',(-0.0118525388697481,-0.033757104784583,
-0.0107750997396421));
#23460=CARTESIAN_POINT('Ctrl Pts',(-0.0119675842690624,-0.0337638519033324,
-0.0107238668266645));
#23461=CARTESIAN_POINT('Ctrl Pts',(-0.0120669245023405,-0.0337697712544364,
-0.0106912082172402));
#23462=CARTESIAN_POINT('Ctrl Pts',(-0.0122353051240417,-0.033779684491913,
-0.0106542013779307));
#23463=CARTESIAN_POINT('Ctrl Pts',(-0.0123027242863996,-0.0337836159000032,
-0.0106440011856401));
#23464=CARTESIAN_POINT('Ctrl Pts',(-0.0123923464125038,-0.0337886405261163,
-0.0106364585944451));
#23465=CARTESIAN_POINT('Ctrl Pts',(-0.0124141314467661,-0.0337898459711493,
-0.0106350898446689));
#23466=CARTESIAN_POINT('Ctrl Pts',(-0.0124511545656918,-0.0337918596321266,
-0.0106335514239226));
#23467=CARTESIAN_POINT('Ctrl Pts',(-0.0124663791902328,-0.0337926776652764,
-0.0106331444393136));
#23468=CARTESIAN_POINT('Ctrl Pts',(-0.0124881822396982,-0.0337938324114437,
-0.0106328845348419));
#23469=CARTESIAN_POINT('Ctrl Pts',(-0.0124947571425421,-0.0337941784545337,
-0.0106328481848931));
#23470=CARTESIAN_POINT('Ctrl Pts',(-0.0125061905878966,-0.0337947761740979,
-0.0106328580562863));
#23471=CARTESIAN_POINT('Ctrl Pts',(-0.0125110489899436,-0.0337950288887853,
-0.0106328851967611));
#23472=CARTESIAN_POINT('Ctrl Pts',(-0.0125214216370628,-0.0337955656459904,
-0.0106329921379444));
#23473=CARTESIAN_POINT('Ctrl Pts',(-0.0125269356490412,-0.0337958493240467,
-0.0106330785515137));
#23474=CARTESIAN_POINT('Ctrl Pts',(-0.0125419646913128,-0.0337966182824319,
-0.0106333946809437));
#23475=CARTESIAN_POINT('Ctrl Pts',(-0.0125514783926477,-0.0337971004190363,
-0.0106336828779773));
#23476=CARTESIAN_POINT('Ctrl Pts',(-0.0126017531627813,-0.033799626570421,
-0.0106356716065254));
#23477=CARTESIAN_POINT('Ctrl Pts',(-0.0126424404025149,-0.0338015957707894,
-0.010638900283556));
#23478=CARTESIAN_POINT('Ctrl Pts',(-0.0127661891140722,-0.0338074794338633,
-0.010653677495936));
#23479=CARTESIAN_POINT('Ctrl Pts',(-0.0128484785538294,-0.033811251827044,
-0.0106703833519706));
#23480=CARTESIAN_POINT('Ctrl Pts',(-0.0130051857784739,-0.033818746274944,
-0.0107157417095733));
#23481=CARTESIAN_POINT('Ctrl Pts',(-0.0130795463175328,-0.0338224497980643,
-0.010743630209548));
#23482=CARTESIAN_POINT('Ctrl Pts',(-0.0131705446041,-0.0338273786683246,
-0.0107860102765897));
#23483=CARTESIAN_POINT('Ctrl Pts',(-0.0131894749911651,-0.033828426377807,
-0.0107953034536584));
#23484=CARTESIAN_POINT('Ctrl Pts',(-0.0132176433641564,-0.0338300219940254,
-0.0108098555642873));
#23485=CARTESIAN_POINT('Ctrl Pts',(-0.0132270275509547,-0.0338305598023805,
-0.0108148269428763));
#23486=CARTESIAN_POINT('Ctrl Pts',(-0.0132438849536706,-0.033831537538864,
-0.0108239814327754));
#23487=CARTESIAN_POINT('Ctrl Pts',(-0.0132513761267323,-0.0338319762423345,
-0.010828130672073));
#23488=CARTESIAN_POINT('Ctrl Pts',(-0.0132673953666124,-0.0338329236224645,
-0.0108371785426421));
#23489=CARTESIAN_POINT('Ctrl Pts',(-0.0132759118848646,-0.033833432996384,
-0.0108420967647028));
#23490=CARTESIAN_POINT('Ctrl Pts',(-0.0132988510462349,-0.0338348207641835,
-0.0108556380148122));
#23491=CARTESIAN_POINT('Ctrl Pts',(-0.0133131805051868,-0.0338357047748763,
-0.0108644156046177));
#23492=CARTESIAN_POINT('Ctrl Pts',(-0.0134117859614017,-0.0338419097792291,
-0.0109270544155038));
#23493=CARTESIAN_POINT('Ctrl Pts',(-0.0134907816943701,-0.0338475313241312,
-0.0109887566480671));
#23494=CARTESIAN_POINT('Ctrl Pts',(-0.0136194032055111,-0.0338577131435112,
-0.0111110570263196));
#23495=CARTESIAN_POINT('Ctrl Pts',(-0.0136714618823321,-0.0338622066619729,
-0.0111686133915369));
#23496=CARTESIAN_POINT('Ctrl Pts',(-0.0137333073952456,-0.0338678574080462,
-0.0112483037142908));
#23497=CARTESIAN_POINT('Ctrl Pts',(-0.0137472171817328,-0.0338691516903793,
-0.0112670932872624));
#23498=CARTESIAN_POINT('Ctrl Pts',(-0.0137699340005241,-0.033871296376397,
-0.0112992841885698));
#23499=CARTESIAN_POINT('Ctrl Pts',(-0.0137789686231406,-0.0338721582173478,
-0.0113125196026057));
#23500=CARTESIAN_POINT('Ctrl Pts',(-0.0137914911886668,-0.0338733629044542,
-0.011331492868959));
#23501=CARTESIAN_POINT('Ctrl Pts',(-0.0137951501211502,-0.0338737161772758,
-0.0113371160379705));
#23502=CARTESIAN_POINT('Ctrl Pts',(-0.0138014056211775,-0.0338743221276717,
-0.0113468682465799));
#23503=CARTESIAN_POINT('Ctrl Pts',(-0.0138040194736659,-0.0338745759284721,
-0.0113509860232788));
#23504=CARTESIAN_POINT('Ctrl Pts',(-0.013809510697429,-0.0338751103286701,
-0.0113597280549905));
#23505=CARTESIAN_POINT('Ctrl Pts',(-0.0138123831523895,-0.0338753906142976,
-0.0113643552130005));
#23506=CARTESIAN_POINT('Ctrl Pts',(-0.0138201750183855,-0.0338761532393882,
-0.0113770564977198));
#23507=CARTESIAN_POINT('Ctrl Pts',(-0.013825044888757,-0.0338766324508055,
-0.0113851609062188));
#23508=CARTESIAN_POINT('Ctrl Pts',(-0.0138492075520212,-0.0338790259337489,
-0.011426222491462));
#23509=CARTESIAN_POINT('Ctrl Pts',(-0.013867347903725,-0.0338808749196336,
-0.011459845278926));
#23510=CARTESIAN_POINT('Ctrl Pts',(-0.0139220774965238,-0.033886742484643,
-0.0115709689639838));
#23511=CARTESIAN_POINT('Ctrl Pts',(-0.0139534663360998,-0.0338905970346306,
-0.0116508518520702));
#23512=CARTESIAN_POINT('Ctrl Pts',(-0.0140032783571748,-0.0338985654211833,
-0.0118170778931771));
#23513=CARTESIAN_POINT('Ctrl Pts',(-0.0140212604602887,-0.0339026720376336,
-0.0119032179818425));
#23514=CARTESIAN_POINT('Ctrl Pts',(-0.014033824569558,-0.0339078493565943,
-0.0120070029145103));
#23515=CARTESIAN_POINT('Ctrl Pts',(-0.0140355632349712,-0.0339086849332264,
-0.0120236239127629));
#23516=CARTESIAN_POINT('Ctrl Pts',(-0.0140378855705759,-0.0339100199072247,
-0.0120499508257753));
#23517=CARTESIAN_POINT('Ctrl Pts',(-0.0140386480739004,-0.0339105136584508,
-0.0120596398757809));
#23518=CARTESIAN_POINT('Ctrl Pts',(-0.014039911085653,-0.0339114486147741,
-0.0120778919923943));
#23519=CARTESIAN_POINT('Ctrl Pts',(-0.0140404318250625,-0.0339118891627012,
-0.0120864533131702));
#23520=CARTESIAN_POINT('Ctrl Pts',(-0.0140414463073588,-0.0339128889318733,
-0.0121057914610266));
#23521=CARTESIAN_POINT('Ctrl Pts',(-0.0140418984581002,-0.0339134494426792,
-0.0121165699432197));
#23522=CARTESIAN_POINT('Ctrl Pts',(-0.014042745840595,-0.0339148590888116,
-0.0121435149562545));
#23523=CARTESIAN_POINT('Ctrl Pts',(-0.0140430000000035,-0.0339157125708919,
-0.0121596840009703));
#23524=CARTESIAN_POINT('Ctrl Pts',(-0.014043,-0.0339165738369763,-0.0121758532868962));
#23525=CARTESIAN_POINT('Origin',(-0.0125,-0.0375520664398416,-0.0121758532865581));
#23526=CARTESIAN_POINT('',(-0.014043,-0.0344186209509151,-0.012175853286558));
#23527=CARTESIAN_POINT('',(-0.014043,-0.0343031952477557,-0.0121758532813813));
#23528=CARTESIAN_POINT('',(-0.014043,-0.0375520664398416,-0.012175853286558));
#23529=CARTESIAN_POINT('Ctrl Pts',(-0.014043,-0.0343031952477557,-0.0121758532762046));
#23530=CARTESIAN_POINT('Ctrl Pts',(-0.0140429999999155,-0.0343025001782861,
-0.0121632591726524));
#23531=CARTESIAN_POINT('Ctrl Pts',(-0.0140428458087414,-0.0343018010815279,
-0.0121506642448564));
#23532=CARTESIAN_POINT('Ctrl Pts',(-0.014040120579621,-0.0342955917809417,
-0.0120394004326745));
#23533=CARTESIAN_POINT('Ctrl Pts',(-0.0140282417712872,-0.0342898578569338,
-0.0119411935070349));
#23534=CARTESIAN_POINT('Ctrl Pts',(-0.0139949955681177,-0.0342809983564059,
-0.011789843232452));
#23535=CARTESIAN_POINT('Ctrl Pts',(-0.0139799239403911,-0.0342778221547362,
-0.0117355787661732));
#23536=CARTESIAN_POINT('Ctrl Pts',(-0.0139576695576264,-0.034274058406594,
-0.0116696665560275));
#23537=CARTESIAN_POINT('Ctrl Pts',(-0.013953256529049,-0.03427334709226,
-0.011657132716861));
#23538=CARTESIAN_POINT('Ctrl Pts',(-0.0139465438191688,-0.0342723162749851,
-0.0116388257687814));
#23539=CARTESIAN_POINT('Ctrl Pts',(-0.0139443704074148,-0.0342719898716033,
-0.0116330073559015));
#23540=CARTESIAN_POINT('Ctrl Pts',(-0.0139404544759888,-0.0342714148059591,
-0.0116227140995119));
#23541=CARTESIAN_POINT('Ctrl Pts',(-0.0139387261284921,-0.0342711653269669,
-0.0116182340736097));
#23542=CARTESIAN_POINT('Ctrl Pts',(-0.0139348999118669,-0.0342706224223885,
-0.0116084524157116));
#23543=CARTESIAN_POINT('Ctrl Pts',(-0.0139327935552788,-0.0342703295055538,
-0.0116031542946884));
#23544=CARTESIAN_POINT('Ctrl Pts',(-0.013926757549759,-0.0342695063942333,
-0.0115882136773387));
#23545=CARTESIAN_POINT('Ctrl Pts',(-0.0139227595288143,-0.0342689801383092,
-0.0115785989433625));
#23546=CARTESIAN_POINT('Ctrl Pts',(-0.0138901791117773,-0.0342648331201147,
-0.0115024312836866));
#23547=CARTESIAN_POINT('Ctrl Pts',(-0.0138570370162666,-0.034261452496981,
-0.0114379184286584));
#23548=CARTESIAN_POINT('Ctrl Pts',(-0.0137708047440976,-0.034253803946893,
-0.0112956707371701));
#23549=CARTESIAN_POINT('Ctrl Pts',(-0.0137149017722829,-0.0342495768176398,
-0.011219987504965));
#23550=CARTESIAN_POINT('Ctrl Pts',(-0.013631191248228,-0.0342436222914258,
-0.0111259585078482));
#23551=CARTESIAN_POINT('Ctrl Pts',(-0.0136091792952162,-0.0342420871570714,
-0.0111027298897534));
#23552=CARTESIAN_POINT('Ctrl Pts',(-0.0135696450220958,-0.0342393658079462,
-0.0110635271549066));
#23553=CARTESIAN_POINT('Ctrl Pts',(-0.0135524469812946,-0.0342381929600111,
-0.0110472412306433));
#23554=CARTESIAN_POINT('Ctrl Pts',(-0.0135266609059339,-0.0342364463305617,
-0.0110239248097739));
#23555=CARTESIAN_POINT('Ctrl Pts',(-0.0135183606171101,-0.0342358858573487,
-0.0110165804642149));
#23556=CARTESIAN_POINT('Ctrl Pts',(-0.0135034977590349,-0.0342348849638155,
-0.0110037121635231));
#23557=CARTESIAN_POINT('Ctrl Pts',(-0.0134969668436084,-0.0342344460680893,
-0.0109981522746276));
#23558=CARTESIAN_POINT('Ctrl Pts',(-0.013483122355339,-0.0342335174184684,
-0.0109865638938266));
#23559=CARTESIAN_POINT('Ctrl Pts',(-0.0134757989300945,-0.0342330271846811,
-0.0109805477742034));
#23560=CARTESIAN_POINT('Ctrl Pts',(-0.0134561905046735,-0.0342317170125173,
-0.0109647399525555));
#23561=CARTESIAN_POINT('Ctrl Pts',(-0.0134438108191034,-0.0342308923214378,
-0.0109550679237343));
#23562=CARTESIAN_POINT('Ctrl Pts',(-0.0133845203030087,-0.0342269531238785,
-0.0109101862460423));
#23563=CARTESIAN_POINT('Ctrl Pts',(-0.0133357789788223,-0.0342237427947477,
-0.0108774844912127));
#23564=CARTESIAN_POINT('Ctrl Pts',(-0.0132028632044925,-0.0342150854732618,
-0.0107988988580127));
#23565=CARTESIAN_POINT('Ctrl Pts',(-0.0131160715130319,-0.0342095165175969,
-0.0107579414345621));
#23566=CARTESIAN_POINT('Ctrl Pts',(-0.0129759041915379,-0.034201005896186,
-0.0107071089824328));
#23567=CARTESIAN_POINT('Ctrl Pts',(-0.0129248420221395,-0.0341980026431484,
-0.0106915336481659));
#23568=CARTESIAN_POINT('Ctrl Pts',(-0.0128605010395783,-0.0341944181106357,
-0.0106755013799547));
#23569=CARTESIAN_POINT('Ctrl Pts',(-0.0128478906298712,-0.0341937249746895,
-0.0106725273157621));
#23570=CARTESIAN_POINT('Ctrl Pts',(-0.0128292422996723,-0.0341927153295564,
-0.0106683764836284));
#23571=CARTESIAN_POINT('Ctrl Pts',(-0.0128232327044016,-0.0341923923028462,
-0.0106670764890774));
#23572=CARTESIAN_POINT('Ctrl Pts',(-0.0128129690918423,-0.0341918447957871,
-0.0106649204044006));
#23573=CARTESIAN_POINT('Ctrl Pts',(-0.0128087190292513,-0.0341916193048559,
-0.0106640462918413));
#23574=CARTESIAN_POINT('Ctrl Pts',(-0.0127990202809435,-0.0341911075549493,
-0.0106620941512873));
#23575=CARTESIAN_POINT('Ctrl Pts',(-0.0127935694186492,-0.0341908219498469,
-0.0106610276047234));
#23576=CARTESIAN_POINT('Ctrl Pts',(-0.01277852983684,-0.0341900391665776,
-0.0106581691029102));
#23577=CARTESIAN_POINT('Ctrl Pts',(-0.0127689295492263,-0.0341895453411792,
-0.0106564385774857));
#23578=CARTESIAN_POINT('Ctrl Pts',(-0.012714358969439,-0.0341867682217497,
-0.0106471352430246));
#23579=CARTESIAN_POINT('Ctrl Pts',(-0.0126690833101511,-0.0341845788641603,
-0.0106414673787615));
#23580=CARTESIAN_POINT('Ctrl Pts',(-0.0125434049372057,-0.0341786597351835,
-0.0106313659900271));
#23581=CARTESIAN_POINT('Ctrl Pts',(-0.0124628061911458,-0.0341750358121085,
-0.0106312036349826));
#23582=CARTESIAN_POINT('Ctrl Pts',(-0.0123050045562738,-0.0341677598296407,
-0.0106432490600485));
#23583=CARTESIAN_POINT('Ctrl Pts',(-0.0122280131332436,-0.0341641222036786,
-0.0106550243931813));
#23584=CARTESIAN_POINT('Ctrl Pts',(-0.0121319177140237,-0.0341592772142508,
-0.0106772540591647));
#23585=CARTESIAN_POINT('Ctrl Pts',(-0.012111690785222,-0.0341582403689585,
-0.0106823673927283));
#23586=CARTESIAN_POINT('Ctrl Pts',(-0.012081402302508,-0.0341566593984008,
-0.0106906811641245));
#23587=CARTESIAN_POINT('Ctrl Pts',(-0.0120712593558486,-0.0341561251314964,
-0.0106935774288066));
#23588=CARTESIAN_POINT('Ctrl Pts',(-0.0120529743466897,-0.0341551529170905,
-0.0106990019950824));
#23589=CARTESIAN_POINT('Ctrl Pts',(-0.0120448219774238,-0.0341547161680707,
-0.010701494227259));
#23590=CARTESIAN_POINT('Ctrl Pts',(-0.0120273333812615,-0.0341537720022813,
-0.0107069994799274));
#23591=CARTESIAN_POINT('Ctrl Pts',(-0.012018004432477,-0.0341532638825246,
-0.010710034230663));
#23592=CARTESIAN_POINT('Ctrl Pts',(-0.0119927710666613,-0.0341518770894466,
-0.0107185096929943));
#23593=CARTESIAN_POINT('Ctrl Pts',(-0.011976925905318,-0.0341509927790022,
-0.0107241215614215));
#23594=CARTESIAN_POINT('Ctrl Pts',(-0.011873853308883,-0.034145150004962,
-0.0107625332350306));
#23595=CARTESIAN_POINT('Ctrl Pts',(-0.0117896707683111,-0.034139933704283,
-0.0108029144086997));
#23596=CARTESIAN_POINT('Ctrl Pts',(-0.0116195660128787,-0.0341285959118747,
-0.0109043629369295));
#23597=CARTESIAN_POINT('Ctrl Pts',(-0.0115351884367015,-0.0341224712879432,
-0.0109671383273606));
#23598=CARTESIAN_POINT('Ctrl Pts',(-0.0114444985879512,-0.0341157494274545,
-0.0110502011985624));
#23599=CARTESIAN_POINT('Ctrl Pts',(-0.0114313814725755,-0.0341147739626844,
-0.0110626460495307));
#23600=CARTESIAN_POINT('Ctrl Pts',(-0.0114134820691962,-0.0341134421749624,
-0.0110802361096432));
#23601=CARTESIAN_POINT('Ctrl Pts',(-0.0114085120577957,-0.0341130723119575,
-0.0110851873028349));
#23602=CARTESIAN_POINT('Ctrl Pts',(-0.0114001199648845,-0.0341124479396526,
-0.0110936624379642));
#23603=CARTESIAN_POINT('Ctrl Pts',(-0.0113966806506289,-0.0341121921031992,
-0.0110971691158545));
#23604=CARTESIAN_POINT('Ctrl Pts',(-0.0113895795570858,-0.034111664086293,
-0.0111044787913426));
#23605=CARTESIAN_POINT('Ctrl Pts',(-0.0113859204782858,-0.0341113921050778,
-0.0111082842302582));
#23606=CARTESIAN_POINT('Ctrl Pts',(-0.0113762430693028,-0.0341106727974637,
-0.0111184526689691));
#23607=CARTESIAN_POINT('Ctrl Pts',(-0.0113702591797555,-0.0341102280436273,
-0.0111248483430431));
#23608=CARTESIAN_POINT('Ctrl Pts',(-0.0113438122980292,-0.0341082606183883,
-0.0111536020519938));
#23609=CARTESIAN_POINT('Ctrl Pts',(-0.0113239551060861,-0.0341067786152503,
-0.0111765103943231));
#23610=CARTESIAN_POINT('Ctrl Pts',(-0.0112469980073477,-0.0341009473641577,
-0.0112707657352405));
#23611=CARTESIAN_POINT('Ctrl Pts',(-0.0111956085801621,-0.0340968387689115,
-0.0113465386881616));
#23612=CARTESIAN_POINT('Ctrl Pts',(-0.0111069104476058,-0.0340884633623077,
-0.0115061707450445));
#23613=CARTESIAN_POINT('Ctrl Pts',(-0.0110697609084799,-0.0340842097093618,
-0.0115896903431503));
#23614=CARTESIAN_POINT('Ctrl Pts',(-0.011034779142933,-0.0340788625490606,
-0.0116918514858917));
#23615=CARTESIAN_POINT('Ctrl Pts',(-0.0110296085039665,-0.0340780245885084,
-0.0117077948247062));
#23616=CARTESIAN_POINT('Ctrl Pts',(-0.0110218560302274,-0.0340766879942518,
-0.0117330965129598));
#23617=CARTESIAN_POINT('Ctrl Pts',(-0.0110191009637645,-0.034076195065444,
-0.011742400642326));
#23618=CARTESIAN_POINT('Ctrl Pts',(-0.0110140874660354,-0.0340752630514139,
-0.0117599376549591));
#23619=CARTESIAN_POINT('Ctrl Pts',(-0.0110118092392667,-0.0340748246351806,
-0.0117681645241889));
#23620=CARTESIAN_POINT('Ctrl Pts',(-0.0110068294485792,-0.0340738316198713,
-0.0117867450807002));
#23621=CARTESIAN_POINT('Ctrl Pts',(-0.0110041671026767,-0.034073275767296,
-0.0117971087460061));
#23622=CARTESIAN_POINT('Ctrl Pts',(-0.0109964463349754,-0.0340715850131807,
-0.0118285152010133));
#23623=CARTESIAN_POINT('Ctrl Pts',(-0.0109917227785662,-0.0340704394205825,
-0.0118496369038934));
#23624=CARTESIAN_POINT('Ctrl Pts',(-0.0109671718474253,-0.0340637851152729,
-0.0119713885849393));
#23625=CARTESIAN_POINT('Ctrl Pts',(-0.0109569757564983,-0.0340579714105121,
-0.012073683851691));
#23626=CARTESIAN_POINT('Ctrl Pts',(-0.0109570221828998,-0.034046703314225,
-0.0122696877500179));
#23627=CARTESIAN_POINT('Ctrl Pts',(-0.0109655372081662,-0.0340412926146118,
-0.0123629673414816));
#23628=CARTESIAN_POINT('Ctrl Pts',(-0.0109847321391462,-0.0340355405047427,
-0.0124673536575062));
#23629=CARTESIAN_POINT('Ctrl Pts',(-0.0109871739779461,-0.0340348613835662,
-0.0124797720309346));
#23630=CARTESIAN_POINT('Ctrl Pts',(-0.0109910408991057,-0.0340338608848952,
-0.0124982349931949));
#23631=CARTESIAN_POINT('Ctrl Pts',(-0.0109923500721701,-0.0340335335474189,
-0.0125043030249268));
#23632=CARTESIAN_POINT('Ctrl Pts',(-0.010994669976286,-0.034032972777018,
-0.0125147495982409));
#23633=CARTESIAN_POINT('Ctrl Pts',(-0.0109956632707457,-0.0340327383782787,
-0.0125191318853797));
#23634=CARTESIAN_POINT('Ctrl Pts',(-0.0109978086250615,-0.0340322440592089,
-0.012528408751749));
#23635=CARTESIAN_POINT('Ctrl Pts',(-0.0109989654948077,-0.0340319844292006,
-0.0125333021616155));
#23636=CARTESIAN_POINT('Ctrl Pts',(-0.011001932652963,-0.0340313353815449,
-0.0125455843965908));
#23637=CARTESIAN_POINT('Ctrl Pts',(-0.0110037737244983,-0.0340309476997052,
-0.0125529657460045));
#23638=CARTESIAN_POINT('Ctrl Pts',(-0.0110112515671131,-0.0340294295694962,
-0.0125820293341924));
#23639=CARTESIAN_POINT('Ctrl Pts',(-0.0110173059019867,-0.0340283210758478,
-0.0126036022626613));
#23640=CARTESIAN_POINT('Ctrl Pts',(-0.0110347453129404,-0.0340254072208504,
-0.0126609141907877));
#23641=CARTESIAN_POINT('Ctrl Pts',(-0.0110469673856446,-0.0340236364636228,
-0.0126963836774273));
#23642=CARTESIAN_POINT('Ctrl Pts',(-0.0111011427833561,-0.0340166364647975,
-0.0128367691975007));
#23643=CARTESIAN_POINT('Ctrl Pts',(-0.0111532656534442,-0.0340116126488013,
-0.0129373773537217));
#23644=CARTESIAN_POINT('Ctrl Pts',(-0.0112416655960233,-0.0340040648823587,
-0.0130700578661278));
#23645=CARTESIAN_POINT('Ctrl Pts',(-0.0112691559250478,-0.0340018188346173,
-0.0131075343881972));
#23646=CARTESIAN_POINT('Ctrl Pts',(-0.0113074673874814,-0.0339987799213331,
-0.0131551024233376));
#23647=CARTESIAN_POINT('Ctrl Pts',(-0.0113168025875147,-0.0339980460281833,
-0.0131663616248628));
#23648=CARTESIAN_POINT('Ctrl Pts',(-0.0113322971197394,-0.0339968376225824,
-0.0131845179682216));
#23649=CARTESIAN_POINT('Ctrl Pts',(-0.0113383609892643,-0.0339963670458924,
-0.0131914955761731));
#23650=CARTESIAN_POINT('Ctrl Pts',(-0.0113502199331881,-0.0339954510291983,
-0.0132048963517449));
#23651=CARTESIAN_POINT('Ctrl Pts',(-0.0113560070553403,-0.0339950059318243,
-0.0132113261111845));
#23652=CARTESIAN_POINT('Ctrl Pts',(-0.01136968279182,-0.0339939583872156,
-0.0132262658976273));
#23653=CARTESIAN_POINT('Ctrl Pts',(-0.0113776138723128,-0.0339933541328016,
-0.0132347361955889));
#23654=CARTESIAN_POINT('Ctrl Pts',(-0.0114040767878785,-0.0339913481755186,
-0.0132623669024121));
#23655=CARTESIAN_POINT('Ctrl Pts',(-0.0114230088841539,-0.0339899291129235,
-0.0132811358483241));
#23656=CARTESIAN_POINT('Ctrl Pts',(-0.0114697181287215,-0.0339864645574422,
-0.0133251026197715));
#23657=CARTESIAN_POINT('Ctrl Pts',(-0.0114979453942418,-0.0339843999464167,
-0.0133497958032575));
#23658=CARTESIAN_POINT('Ctrl Pts',(-0.011637651110176,-0.0339743343944601,
-0.0134632976154327));
#23659=CARTESIAN_POINT('Ctrl Pts',(-0.0117601616082825,-0.0339658753144117,
-0.0135373937570606));
#23660=CARTESIAN_POINT('Ctrl Pts',(-0.0119093496999108,-0.0339569652999109,
-0.0136014675862712));
#23661=CARTESIAN_POINT('Ctrl Pts',(-0.0119277598477927,-0.0339558895009686,
-0.0136089566285915));
#23662=CARTESIAN_POINT('Ctrl Pts',(-0.0119533035028888,-0.0339544343401563,
-0.013618776733013));
#23663=CARTESIAN_POINT('Ctrl Pts',(-0.011960316297486,-0.0339540386794832,
-0.013621414298075));
#23664=CARTESIAN_POINT('Ctrl Pts',(-0.011971578654342,-0.0339534097221458,
-0.0136255567734038));
#23665=CARTESIAN_POINT('Ctrl Pts',(-0.0119758159973781,-0.0339531745402035,
-0.0136270942902337));
#23666=CARTESIAN_POINT('Ctrl Pts',(-0.0119847782164407,-0.0339526802831967,
-0.0136303018508139));
#23667=CARTESIAN_POINT('Ctrl Pts',(-0.0119895046014784,-0.0339524214839101,
-0.0136319674858335));
#23668=CARTESIAN_POINT('Ctrl Pts',(-0.0120013490607268,-0.0339517773686502,
-0.0136360768577345));
#23669=CARTESIAN_POINT('Ctrl Pts',(-0.0120084771505703,-0.0339513937330016,
-0.0136384916321495));
#23670=CARTESIAN_POINT('Ctrl Pts',(-0.0120362812142936,-0.033949911808473,
-0.0136476845653664));
#23671=CARTESIAN_POINT('Ctrl Pts',(-0.0120570828194464,-0.0339488341641262,
-0.0136540775205268));
#23672=CARTESIAN_POINT('Ctrl Pts',(-0.0121125738806857,-0.0339460245121221,
-0.0136698549496255));
#23673=CARTESIAN_POINT('Ctrl Pts',(-0.0121474686241941,-0.0339443241260699,
-0.0136784716199955));
#23674=CARTESIAN_POINT('Ctrl Pts',(-0.0122472492148597,-0.0339395714174577,
-0.0136994429950605));
#23675=CARTESIAN_POINT('Ctrl Pts',(-0.012312670921864,-0.0339365821794981,
-0.0137088623568889));
#23676=CARTESIAN_POINT('Ctrl Pts',(-0.0124695198751476,-0.0339293672839225,
-0.0137212519344233));
#23677=CARTESIAN_POINT('Ctrl Pts',(-0.0125609950934298,-0.0339251121722748,
-0.013720347791863));
#23678=CARTESIAN_POINT('Ctrl Pts',(-0.012668527312152,-0.0339197637057954,
-0.0137097139447504));
#23679=CARTESIAN_POINT('Ctrl Pts',(-0.0126851797925043,-0.0339189260030248,
-0.0137077927078329));
#23680=CARTESIAN_POINT('Ctrl Pts',(-0.0127115127304582,-0.0339175850251615,
-0.0137043189870211));
#23681=CARTESIAN_POINT('Ctrl Pts',(-0.0127212156050764,-0.0339170873970374,
-0.0137029448630254));
#23682=CARTESIAN_POINT('Ctrl Pts',(-0.0127393343318218,-0.0339161513139628,
-0.0137002025791944));
#23683=CARTESIAN_POINT('Ctrl Pts',(-0.0127477532388353,-0.0339157135910384,
-0.0136988569034629));
#23684=CARTESIAN_POINT('Ctrl Pts',(-0.0127665763240518,-0.0339147285598326,
-0.0136956880238568));
#23685=CARTESIAN_POINT('Ctrl Pts',(-0.0127769737358373,-0.0339141800816312,
-0.0136938276300223));
#23686=CARTESIAN_POINT('Ctrl Pts',(-0.0128079189208646,-0.0339125343235155,
-0.0136879621363756));
#23687=CARTESIAN_POINT('Ctrl Pts',(-0.0128284045828412,-0.0339114271713619,
-0.0136836455823627));
#23688=CARTESIAN_POINT('Ctrl Pts',(-0.0129251292450522,-0.0339061138457267,
-0.0136611999642417));
#23689=CARTESIAN_POINT('Ctrl Pts',(-0.0129999935089968,-0.033901738289074,
-0.0136376992090498));
#23690=CARTESIAN_POINT('Ctrl Pts',(-0.0131486557125619,-0.0338926037356183,
-0.0135782721193122));
#23691=CARTESIAN_POINT('Ctrl Pts',(-0.0132220365602471,-0.0338878509325728,
-0.0135419411007113));
#23692=CARTESIAN_POINT('Ctrl Pts',(-0.013329778709678,-0.0338807514782663,
-0.0134774809683645));
#23693=CARTESIAN_POINT('Ctrl Pts',(-0.01336639292423,-0.0338783171863884,
-0.0134534022032823));
#23694=CARTESIAN_POINT('Ctrl Pts',(-0.0134097757816292,-0.0338754515491987,
-0.0134221479554379));
#23695=CARTESIAN_POINT('Ctrl Pts',(-0.0134175630498147,-0.0338749379522715,
-0.0134164259097671));
#23696=CARTESIAN_POINT('Ctrl Pts',(-0.0134297243011914,-0.0338741378081026,
-0.0134073127223922));
#23697=CARTESIAN_POINT('Ctrl Pts',(-0.0134341345492815,-0.0338738480435428,
-0.0134039706523065));
#23698=CARTESIAN_POINT('Ctrl Pts',(-0.0134423585012808,-0.0338733086268853,
-0.0133976686402707));
#23699=CARTESIAN_POINT('Ctrl Pts',(-0.0134461762972185,-0.0338730586071664,
-0.0133947145249577));
#23700=CARTESIAN_POINT('Ctrl Pts',(-0.0134550759381883,-0.0338724766146771,
-0.0133877611906282));
#23701=CARTESIAN_POINT('Ctrl Pts',(-0.0134601465741876,-0.033872145642017,
-0.0133837478906604));
#23702=CARTESIAN_POINT('Ctrl Pts',(-0.0134766598247441,-0.0338710692824627,
-0.0133705083152189));
#23703=CARTESIAN_POINT('Ctrl Pts',(-0.0134879961645058,-0.0338703327408832,
-0.0133611501520987));
#23704=CARTESIAN_POINT('Ctrl Pts',(-0.0135150749094679,-0.0338685744948397,
-0.0133381381409284));
#23705=CARTESIAN_POINT('Ctrl Pts',(-0.0135306780669897,-0.0338675622911256,
-0.0133243244194481));
#23706=CARTESIAN_POINT('Ctrl Pts',(-0.0135921505298278,-0.0338635563248979,
-0.0132676397082127));
#23707=CARTESIAN_POINT('Ctrl Pts',(-0.0136356661331904,-0.0338606769791345,
-0.0132223014160844));
#23708=CARTESIAN_POINT('Ctrl Pts',(-0.013748768832314,-0.0338526845189636,
-0.0130890698215807));
#23709=CARTESIAN_POINT('Ctrl Pts',(-0.0138117230367726,-0.0338475881631072,
-0.0129960779024097));
#23710=CARTESIAN_POINT('Ctrl Pts',(-0.0138738817199854,-0.0338410609070436,
-0.0128785193145112));
#23711=CARTESIAN_POINT('Ctrl Pts',(-0.0138833227899311,-0.0338400172924914,
-0.012859745480525));
#23712=CARTESIAN_POINT('Ctrl Pts',(-0.0138969955099977,-0.0338384212191129,
-0.0128311146042731));
#23713=CARTESIAN_POINT('Ctrl Pts',(-0.0139015127879805,-0.0338378786935256,
-0.012821396272776));
#23714=CARTESIAN_POINT('Ctrl Pts',(-0.0139094463617619,-0.0338368976195423,
-0.0128038523704722));
#23715=CARTESIAN_POINT('Ctrl Pts',(-0.0139128996525081,-0.0338364603723145,
-0.0127960439541196));
#23716=CARTESIAN_POINT('Ctrl Pts',(-0.0139201344036976,-0.0338355219611277,
-0.0127793110037617));
#23717=CARTESIAN_POINT('Ctrl Pts',(-0.01392389692116,-0.033835020171144,
-0.0127703787218071));
#23718=CARTESIAN_POINT('Ctrl Pts',(-0.0139339156993355,-0.0338336454730962,
-0.0127459532225766));
#23719=CARTESIAN_POINT('Ctrl Pts',(-0.0139400047342329,-0.0338327669578527,
-0.0127303931909371));
#23720=CARTESIAN_POINT('Ctrl Pts',(-0.0139770304278779,-0.0338271390945943,
-0.0126310523803796));
#23721=CARTESIAN_POINT('Ctrl Pts',(-0.0140008924353247,-0.0338221541627022,
-0.012544828933463));
#23722=CARTESIAN_POINT('Ctrl Pts',(-0.0140332301460074,-0.0338120131433148,
-0.012370346730091));
#23723=CARTESIAN_POINT('Ctrl Pts',(-0.0140418372477321,-0.0338068806733685,
-0.0122824390536171));
#23724=CARTESIAN_POINT('Ctrl Pts',(-0.014042963335665,-0.0338015947159046,
-0.0121881359786935));
#23725=CARTESIAN_POINT('Ctrl Pts',(-0.0140430000000025,-0.0338012515219821,
-0.0121819945706754));
#23726=CARTESIAN_POINT('Ctrl Pts',(-0.014043,-0.0338009094848242,-0.0121758532859222));
#23727=CARTESIAN_POINT('Ctrl Pts',(-0.014043,-0.0339165738369763,-0.0121758532868962));
#23728=CARTESIAN_POINT('Ctrl Pts',(-0.0140429999999987,-0.0339168819553875,
-0.0121816378577507));
#23729=CARTESIAN_POINT('Ctrl Pts',(-0.0140429674712373,-0.033917191068193,
-0.0121874224595749));
#23730=CARTESIAN_POINT('Ctrl Pts',(-0.0140418661808551,-0.0339224402550407,
-0.0122853381697386));
#23731=CARTESIAN_POINT('Ctrl Pts',(-0.0140325801638651,-0.0339276333236809,
-0.0123771794184772));
#23732=CARTESIAN_POINT('Ctrl Pts',(-0.0140005714140538,-0.0339373450165894,
-0.0125433955946321));
#23733=CARTESIAN_POINT('Ctrl Pts',(-0.0139803192175374,-0.0339418181117581,
-0.0126179590145431));
#23734=CARTESIAN_POINT('Ctrl Pts',(-0.0139467928300904,-0.0339474463079475,
-0.0127126804242815));
#23735=CARTESIAN_POINT('Ctrl Pts',(-0.0139385137036548,-0.0339487375513169,
-0.0127344866971223));
#23736=CARTESIAN_POINT('Ctrl Pts',(-0.0139237275806061,-0.033950877777093,
-0.0127709202301066));
#23737=CARTESIAN_POINT('Ctrl Pts',(-0.0139174816935648,-0.0339517381395521,
-0.0127856488087573));
#23738=CARTESIAN_POINT('Ctrl Pts',(-0.0139082946000599,-0.0339529411465164,
-0.01280640880767));
#23739=CARTESIAN_POINT('Ctrl Pts',(-0.0139055415684377,-0.033953294179785,
-0.0128125218411621));
#23740=CARTESIAN_POINT('Ctrl Pts',(-0.0139007173125061,-0.0339538998557613,
-0.0128230501587434));
#23741=CARTESIAN_POINT('Ctrl Pts',(-0.0138986648578924,-0.0339541536188767,
-0.0128274738806194));
#23742=CARTESIAN_POINT('Ctrl Pts',(-0.0138942749599308,-0.0339546880892563,
-0.0128368192612915));
#23743=CARTESIAN_POINT('Ctrl Pts',(-0.0138919323914168,-0.0339549684811363,
-0.0128417383390659));
#23744=CARTESIAN_POINT('Ctrl Pts',(-0.0138854492956723,-0.0339557317070355,
-0.0128551682535083));
#23745=CARTESIAN_POINT('Ctrl Pts',(-0.0138812563780146,-0.0339562114047318,
-0.0128636536950639));
#23746=CARTESIAN_POINT('Ctrl Pts',(-0.0138596882441195,-0.0339586126064289,
-0.0129063095507802));
#23747=CARTESIAN_POINT('Ctrl Pts',(-0.013841120852835,-0.0339604683146547,
-0.0129398649008883));
#23748=CARTESIAN_POINT('Ctrl Pts',(-0.0137771292331624,-0.0339663367787027,
-0.0130459755702796));
#23749=CARTESIAN_POINT('Ctrl Pts',(-0.0137269155223952,-0.0339701867653888,
-0.0131154551184635));
#23750=CARTESIAN_POINT('Ctrl Pts',(-0.0136140448127748,-0.0339781479683432,
-0.0132470487015677));
#23751=CARTESIAN_POINT('Ctrl Pts',(-0.0135513143481563,-0.0339822520805361,
-0.0133086778101584));
#23752=CARTESIAN_POINT('Ctrl Pts',(-0.0134708167675302,-0.0339874264744039,
-0.0133752877386101));
#23753=CARTESIAN_POINT('Ctrl Pts',(-0.0134577714770716,-0.0339882619674114,
-0.0133857301278624));
#23754=CARTESIAN_POINT('Ctrl Pts',(-0.0134368746619523,-0.0339895968383089,
-0.0134019076566646));
#23755=CARTESIAN_POINT('Ctrl Pts',(-0.0134291339232105,-0.0339900905715831,
-0.01340778412786));
#23756=CARTESIAN_POINT('Ctrl Pts',(-0.0134144580375437,-0.0339910255129273,
-0.0134187084934615));
#23757=CARTESIAN_POINT('Ctrl Pts',(-0.0134075352859757,-0.0339914660640731,
-0.0134237724620258));
#23758=CARTESIAN_POINT('Ctrl Pts',(-0.0133918105008916,-0.0339924658665136,
-0.0134350750385165));
#23759=CARTESIAN_POINT('Ctrl Pts',(-0.0133829845956837,-0.033993026407715,
-0.0134412795332876));
#23760=CARTESIAN_POINT('Ctrl Pts',(-0.0133565991031334,-0.0339947006558988,
-0.0134594177420068));
#23761=CARTESIAN_POINT('Ctrl Pts',(-0.0133388579822405,-0.0339958244594125,
-0.0134710818222768));
#23762=CARTESIAN_POINT('Ctrl Pts',(-0.0132295442832735,-0.0340027394800111,
-0.0135397631460481));
#23763=CARTESIAN_POINT('Ctrl Pts',(-0.0131324528691232,-0.034008872529904,
-0.0135874063062154));
#23764=CARTESIAN_POINT('Ctrl Pts',(-0.012969652526776,-0.0340188463127523,
-0.0136471022663717));
#23765=CARTESIAN_POINT('Ctrl Pts',(-0.0129067222950847,-0.0340226252486277,
-0.0136657273388944));
#23766=CARTESIAN_POINT('Ctrl Pts',(-0.0128219608150001,-0.0340274779539682,
-0.0136850407778995));
#23767=CARTESIAN_POINT('Ctrl Pts',(-0.0128010282009019,-0.0340286573498574,
-0.0136893551027976));
#23768=CARTESIAN_POINT('Ctrl Pts',(-0.0127652697494482,-0.0340306323340263,
-0.0136959538398902));
#23769=CARTESIAN_POINT('Ctrl Pts',(-0.0127504881781399,-0.0340314372853405,
-0.0136984594200026));
#23770=CARTESIAN_POINT('Ctrl Pts',(-0.0127292147095755,-0.0340325770535712,
-0.0137017472240129));
#23771=CARTESIAN_POINT('Ctrl Pts',(-0.012722751113083,-0.034032920883753,
-0.0137027041751847));
#23772=CARTESIAN_POINT('Ctrl Pts',(-0.0127114763373589,-0.0340335161068744,
-0.0137043003125492));
#23773=CARTESIAN_POINT('Ctrl Pts',(-0.0127066679255429,-0.0340337685120117,
-0.0137049579014638));
#23774=CARTESIAN_POINT('Ctrl Pts',(-0.0126963667331323,-0.034034306096683,
-0.0137063171921365));
#23775=CARTESIAN_POINT('Ctrl Pts',(-0.0126908732145924,-0.03403459089536,
-0.0137070120235859));
#23776=CARTESIAN_POINT('Ctrl Pts',(-0.0126758286714037,-0.0340353659628247,
-0.0137088326616785));
#23777=CARTESIAN_POINT('Ctrl Pts',(-0.01266627052738,-0.034035853004221,
-0.0137098987900806));
#23778=CARTESIAN_POINT('Ctrl Pts',(-0.0126144778912107,-0.0340384660171013,
-0.0137151860436606));
#23779=CARTESIAN_POINT('Ctrl Pts',(-0.0125720897816036,-0.0340405108877644,
-0.0137177528066572));
#23780=CARTESIAN_POINT('Ctrl Pts',(-0.0124470069403706,-0.0340464052221194,
-0.0137201565645436));
#23781=CARTESIAN_POINT('Ctrl Pts',(-0.0123643700750698,-0.0340501257252152,
-0.0137151019765015));
#23782=CARTESIAN_POINT('Ctrl Pts',(-0.0122045639817979,-0.0340575430202072,
-0.013692352199915));
#23783=CARTESIAN_POINT('Ctrl Pts',(-0.01212756464644,-0.0340612226693292,
-0.0136753004213883));
#23784=CARTESIAN_POINT('Ctrl Pts',(-0.0120320943646422,-0.0340661217417427,
-0.0136463481344442));
#23785=CARTESIAN_POINT('Ctrl Pts',(-0.012012107731748,-0.0340671661508977,
-0.013639838212183));
#23786=CARTESIAN_POINT('Ctrl Pts',(-0.0119822453669242,-0.0340687577323076,
-0.013629432190861));
#23787=CARTESIAN_POINT('Ctrl Pts',(-0.0119722662719568,-0.0340692948845896,
-0.0136258390092792));
#23788=CARTESIAN_POINT('Ctrl Pts',(-0.0119542992869944,-0.0340702719232579,
-0.0136191595774042));
#23789=CARTESIAN_POINT('Ctrl Pts',(-0.0119462984888226,-0.0340707105931873,
-0.0136161091492304));
#23790=CARTESIAN_POINT('Ctrl Pts',(-0.0119291546369109,-0.0340716584595555,
-0.0136094088253486));
#23791=CARTESIAN_POINT('Ctrl Pts',(-0.0119200203267481,-0.0340721683596231,
-0.013605737716826));
#23792=CARTESIAN_POINT('Ctrl Pts',(-0.0118953508102537,-0.0340735589724287,
-0.0135955476849608));
#23793=CARTESIAN_POINT('Ctrl Pts',(-0.0118798865356904,-0.0340744453405359,
-0.0135888614565525));
#23794=CARTESIAN_POINT('Ctrl Pts',(-0.0117830585293732,-0.0340800898728459,
-0.0135451006373227));
#23795=CARTESIAN_POINT('Ctrl Pts',(-0.0117049480160294,-0.0340850837187335,
-0.0135012708639027));
#23796=CARTESIAN_POINT('Ctrl Pts',(-0.0115600854845306,-0.0340951046315003,
-0.0134025523475392));
#23797=CARTESIAN_POINT('Ctrl Pts',(-0.0114932556694099,-0.0341001028324449,
-0.013348327577726));
#23798=CARTESIAN_POINT('Ctrl Pts',(-0.0114135372186772,-0.0341063064698478,
-0.0132717789779167));
#23799=CARTESIAN_POINT('Ctrl Pts',(-0.0113961976756812,-0.0341076716363909,
-0.0132543128512691));
#23800=CARTESIAN_POINT('Ctrl Pts',(-0.0113678443336097,-0.0341099199323959,
-0.0132243519613536));
#23801=CARTESIAN_POINT('Ctrl Pts',(-0.0113566018868824,-0.034110815869021,
-0.0132120804445538));
#23802=CARTESIAN_POINT('Ctrl Pts',(-0.0113410418169122,-0.0341120592011703,
-0.0131945344416672));
#23803=CARTESIAN_POINT('Ctrl Pts',(-0.0113365575880127,-0.0341124179146666,
-0.0131894099565694));
#23804=CARTESIAN_POINT('Ctrl Pts',(-0.0113289097754156,-0.034113030125752,
-0.0131805525573911));
#23805=CARTESIAN_POINT('Ctrl Pts',(-0.0113257297810704,-0.0341132848106381,
-0.0131768340028047));
#23806=CARTESIAN_POINT('Ctrl Pts',(-0.0113190777067926,-0.0341138177497968,
-0.0131689800115793));
#23807=CARTESIAN_POINT('Ctrl Pts',(-0.0113156095912245,-0.0341140957258592,
-0.0131648414138303));
#23808=CARTESIAN_POINT('Ctrl Pts',(-0.0113062650182166,-0.0341148453117391,
-0.0131535706236289));
#23809=CARTESIAN_POINT('Ctrl Pts',(-0.0113004307062702,-0.0341153139708604,
-0.0131464036023412));
#23810=CARTESIAN_POINT('Ctrl Pts',(-0.0112726333011313,-0.0341175524042072,
-0.0131116229387454));
#23811=CARTESIAN_POINT('Ctrl Pts',(-0.0112515559114053,-0.0341192666688254,
-0.0130833121254884));
#23812=CARTESIAN_POINT('Ctrl Pts',(-0.0111815198250803,-0.034125117201908,
-0.0129821757173299));
#23813=CARTESIAN_POINT('Ctrl Pts',(-0.011137812967947,-0.0341290632318393,
-0.0129059176817033));
#23814=CARTESIAN_POINT('Ctrl Pts',(-0.0110665693752285,-0.0341368196305555,
-0.0127526783502748));
#23815=CARTESIAN_POINT('Ctrl Pts',(-0.011038191181993,-0.0341406071633157,
-0.0126764167811611));
#23816=CARTESIAN_POINT('Ctrl Pts',(-0.0110101121022922,-0.0341456409612672,
-0.0125777709467302));
#23817=CARTESIAN_POINT('Ctrl Pts',(-0.0110046999714092,-0.0341467001635747,
-0.0125571425758574));
#23818=CARTESIAN_POINT('Ctrl Pts',(-0.0109972248765825,-0.0341483098244435,
-0.0125260385130953));
#23819=CARTESIAN_POINT('Ctrl Pts',(-0.0109948401621653,-0.0341488499092875,
-0.0125156423676058));
#23820=CARTESIAN_POINT('Ctrl Pts',(-0.0109907515084667,-0.0341498260794714,
-0.0124969296714958));
#23821=CARTESIAN_POINT('Ctrl Pts',(-0.0109890080441714,-0.0341502608711658,
-0.0124886221465086));
#23822=CARTESIAN_POINT('Ctrl Pts',(-0.0109854049022679,-0.0341512010374324,
-0.0124707197057026));
#23823=CARTESIAN_POINT('Ctrl Pts',(-0.0109835676686091,-0.0341517071119637,
-0.0124611206937532));
#23824=CARTESIAN_POINT('Ctrl Pts',(-0.010978868711545,-0.034153077070768,
-0.0124352407394915));
#23825=CARTESIAN_POINT('Ctrl Pts',(-0.0109761772794249,-0.0341539463330875,
-0.0124189305067325));
#23826=CARTESIAN_POINT('Ctrl Pts',(-0.0109625220912687,-0.0341588796863046,
-0.0123270084003832));
#23827=CARTESIAN_POINT('Ctrl Pts',(-0.0109569254141913,-0.0341631120817109,
-0.012250716307284));
#23828=CARTESIAN_POINT('Ctrl Pts',(-0.0109570599964251,-0.0341708617876835,
-0.0121142608933694));
#23829=CARTESIAN_POINT('Ctrl Pts',(-0.0109606271248052,-0.0341743301422374,
-0.0120542462511054));
#23830=CARTESIAN_POINT('Ctrl Pts',(-0.0109762855719327,-0.0341819839972782,
-0.0119218736270641));
#23831=CARTESIAN_POINT('Ctrl Pts',(-0.0109900545224996,-0.0341861514704352,
-0.0118498503352225));
#23832=CARTESIAN_POINT('Ctrl Pts',(-0.0110115743999154,-0.0341906470959918,
-0.0117689782013035));
#23833=CARTESIAN_POINT('Ctrl Pts',(-0.0110143628699955,-0.0341912032825339,
-0.0117589115261202));
#23834=CARTESIAN_POINT('Ctrl Pts',(-0.0110188371096052,-0.0341920555827564,
-0.0117433741014541));
#23835=CARTESIAN_POINT('Ctrl Pts',(-0.0110204514078073,-0.034192355583777,
-0.011737883288903));
#23836=CARTESIAN_POINT('Ctrl Pts',(-0.0110234824791191,-0.0341929051354327,
-0.0117277815556296));
#23837=CARTESIAN_POINT('Ctrl Pts',(-0.0110248903332141,-0.0341931551716302,
-0.0117231682556579));
#23838=CARTESIAN_POINT('Ctrl Pts',(-0.0110281707749667,-0.0341937260555698,
-0.0117125966219053));
#23839=CARTESIAN_POINT('Ctrl Pts',(-0.011030057923812,-0.034194046052353,
-0.0117066429922562));
#23840=CARTESIAN_POINT('Ctrl Pts',(-0.0110361036969079,-0.0341950457294547,
-0.0116879641251366));
#23841=CARTESIAN_POINT('Ctrl Pts',(-0.0110403919102006,-0.0341957182474183,
-0.0116752811468108));
#23842=CARTESIAN_POINT('Ctrl Pts',(-0.0110637921214595,-0.0341992111765697,
-0.0116089306680731));
#23843=CARTESIAN_POINT('Ctrl Pts',(-0.0110857018862287,-0.034201895485191,
-0.0115562919490737));
#23844=CARTESIAN_POINT('Ctrl Pts',(-0.0111536770251621,-0.0342091294323706,
-0.0114155001548916));
#23845=CARTESIAN_POINT('Ctrl Pts',(-0.0112054208378183,-0.0342135776605898,
-0.0113304022107571));
#23846=CARTESIAN_POINT('Ctrl Pts',(-0.0112959237898262,-0.0342206841362531,
-0.0112095652720746));
#23847=CARTESIAN_POINT('Ctrl Pts',(-0.0113289095904308,-0.0342231669787839,
-0.0111698420270301));
#23848=CARTESIAN_POINT('Ctrl Pts',(-0.0113741618885419,-0.0342264896218121,
-0.0111205944995771));
#23849=CARTESIAN_POINT('Ctrl Pts',(-0.011384668643336,-0.0342272556095621,
-0.0111094956990838));
#23850=CARTESIAN_POINT('Ctrl Pts',(-0.0114019093675456,-0.0342285048183376,
-0.0110918170591769));
#23851=CARTESIAN_POINT('Ctrl Pts',(-0.0114085418524266,-0.0342289836011937,
-0.0110851394440199));
#23852=CARTESIAN_POINT('Ctrl Pts',(-0.0114213816155277,-0.034229907293543,
-0.0110724467050304));
#23853=CARTESIAN_POINT('Ctrl Pts',(-0.011427579173089,-0.034230351760627,
-0.0110664222299238));
#23854=CARTESIAN_POINT('Ctrl Pts',(-0.0114420327825883,-0.0342313853077307,
-0.0110526065523283));
#23855=CARTESIAN_POINT('Ctrl Pts',(-0.0114503247823202,-0.0342319760226555,
-0.0110448538227376));
#23856=CARTESIAN_POINT('Ctrl Pts',(-0.01147716705339,-0.0342338815517711,
-0.011020306704095));
#23857=CARTESIAN_POINT('Ctrl Pts',(-0.0114960399330842,-0.0342352113660145,
-0.0110038723882454));
#23858=CARTESIAN_POINT('Ctrl Pts',(-0.0115867473111157,-0.0342415588360713,
-0.0109286845707943));
#23859=CARTESIAN_POINT('Ctrl Pts',(-0.0116633789458999,-0.0342468118296892,
-0.0108760373479941));
#23860=CARTESIAN_POINT('Ctrl Pts',(-0.0118302512465144,-0.0342578068989465,
-0.0107822921191419));
#23861=CARTESIAN_POINT('Ctrl Pts',(-0.0119206760742138,-0.0342635322458617,
-0.0107423393303115));
#23862=CARTESIAN_POINT('Ctrl Pts',(-0.0120259792068886,-0.0342695394874135,
-0.010707417147708));
#23863=CARTESIAN_POINT('Ctrl Pts',(-0.012037704699816,-0.0342701993351495,
-0.0107036836360494));
#23864=CARTESIAN_POINT('Ctrl Pts',(-0.0120553421645006,-0.0342711770218776,
-0.0106982992081205));
#23865=CARTESIAN_POINT('Ctrl Pts',(-0.0120612211157337,-0.0342715004505767,
-0.0106965427246439));
#23866=CARTESIAN_POINT('Ctrl Pts',(-0.0120718459873247,-0.0342720803496296,
-0.0106934371903639));
#23867=CARTESIAN_POINT('Ctrl Pts',(-0.0120765881985979,-0.0342723375211186,
-0.010692075746158));
#23868=CARTESIAN_POINT('Ctrl Pts',(-0.0120863423381146,-0.0342728629797478,
-0.0106893259966914));
#23869=CARTESIAN_POINT('Ctrl Pts',(-0.0120913548806263,-0.0342731311213061,
-0.0106879402471858));
#23870=CARTESIAN_POINT('Ctrl Pts',(-0.0121044195150341,-0.0342738253265849,
-0.0106843994462253));
#23871=CARTESIAN_POINT('Ctrl Pts',(-0.0121124823328493,-0.0342742491457788,
-0.0106822842250389));
#23872=CARTESIAN_POINT('Ctrl Pts',(-0.0121484985631459,-0.0342761234157088,
-0.010673146921336));
#23873=CARTESIAN_POINT('Ctrl Pts',(-0.0121766298190491,-0.0342775367744566,
-0.0106668431475499));
#23874=CARTESIAN_POINT('Ctrl Pts',(-0.0122593065354476,-0.0342815862738689,
-0.0106507350859149));
#23875=CARTESIAN_POINT('Ctrl Pts',(-0.0123142248016605,-0.03428414596265,
-0.0106430756999138));
#23876=CARTESIAN_POINT('Ctrl Pts',(-0.0124925214292395,-0.0342923481943397,
-0.0106279347851452));
#23877=CARTESIAN_POINT('Ctrl Pts',(-0.0126164021547135,-0.0342979222621967,
-0.0106323002044008));
#23878=CARTESIAN_POINT('Ctrl Pts',(-0.0127564829825984,-0.034304894310201,
-0.0106542097215534));
#23879=CARTESIAN_POINT('Ctrl Pts',(-0.0127744778656844,-0.0343058018431939,
-0.010657352537306));
#23880=CARTESIAN_POINT('Ctrl Pts',(-0.0128032320490911,-0.0343072729945317,
-0.0106629022783815));
#23881=CARTESIAN_POINT('Ctrl Pts',(-0.012814028966042,-0.0343078301740489,
-0.0106651063755651));
#23882=CARTESIAN_POINT('Ctrl Pts',(-0.0128332315208545,-0.0343088300182377,
-0.010669241153507));
#23883=CARTESIAN_POINT('Ctrl Pts',(-0.0128416463865858,-0.0343092712258645,
-0.0106711270295678));
#23884=CARTESIAN_POINT('Ctrl Pts',(-0.0128592788420057,-0.0343102023283021,
-0.0106752342123483));
#23885=CARTESIAN_POINT('Ctrl Pts',(-0.0128684926289635,-0.0343106926803488,
-0.0106774701348917));
#23886=CARTESIAN_POINT('Ctrl Pts',(-0.0128928155464958,-0.0343119974403325,
-0.0106836105223035));
#23887=CARTESIAN_POINT('Ctrl Pts',(-0.0129078867897223,-0.0343128164998596,
-0.0106876594606027));
#23888=CARTESIAN_POINT('Ctrl Pts',(-0.0129841371338026,-0.0343170155297221,
-0.0107093896420596));
#23889=CARTESIAN_POINT('Ctrl Pts',(-0.0130442347208517,-0.0343205102854798,
-0.0107306157847064));
#23890=CARTESIAN_POINT('Ctrl Pts',(-0.0131637612941513,-0.0343278159899963,
-0.0107813464492047));
#23891=CARTESIAN_POINT('Ctrl Pts',(-0.013222949450712,-0.0343316265907891,
-0.0108110926124364));
#23892=CARTESIAN_POINT('Ctrl Pts',(-0.0132999518711651,-0.0343367588370512,
-0.0108562099697055));
#23893=CARTESIAN_POINT('Ctrl Pts',(-0.0133195975824376,-0.034338084110897,
-0.0108683207611632));
#23894=CARTESIAN_POINT('Ctrl Pts',(-0.0133886065513542,-0.034342781360564,
-0.010913028651199));
#23895=CARTESIAN_POINT('Ctrl Pts',(-0.013436362987608,-0.0343461120321917,
-0.0109480205363585));
#23896=CARTESIAN_POINT('Ctrl Pts',(-0.0134899171378269,-0.0343498398806495,
-0.0109922070016261));
#23897=CARTESIAN_POINT('Ctrl Pts',(-0.0134977733931625,-0.034350386505033,
-0.0109988219638662));
#23898=CARTESIAN_POINT('Ctrl Pts',(-0.0135098744994844,-0.0343512272905925,
-0.0110092193233459));
#23899=CARTESIAN_POINT('Ctrl Pts',(-0.0135141653446655,-0.034351525182294,
-0.011012947458667));
#23900=CARTESIAN_POINT('Ctrl Pts',(-0.0135220624227746,-0.034352072831153,
-0.0110198858508781));
#23901=CARTESIAN_POINT('Ctrl Pts',(-0.0135256742153983,-0.034352323047202,
-0.0110230893415534));
#23902=CARTESIAN_POINT('Ctrl Pts',(-0.013533964311583,-0.0343528968425861,
-0.0110305120764382));
#23903=CARTESIAN_POINT('Ctrl Pts',(-0.0135386318644841,-0.0343532195365757,
-0.0110347430648929));
#23904=CARTESIAN_POINT('Ctrl Pts',(-0.013553352486738,-0.0343542365682551,
-0.0110482519930885));
#23905=CARTESIAN_POINT('Ctrl Pts',(-0.0135633083998079,-0.034354923384867,
-0.0110576353250008));
#23906=CARTESIAN_POINT('Ctrl Pts',(-0.013616011049628,-0.0343585619753758,
-0.0111086473952346));
#23907=CARTESIAN_POINT('Ctrl Pts',(-0.0136564443444972,-0.034361364809422,
-0.0111526002560622));
#23908=CARTESIAN_POINT('Ctrl Pts',(-0.0137587137663943,-0.0343688224020463,
-0.0112776006168463));
#23909=CARTESIAN_POINT('Ctrl Pts',(-0.0138152329854705,-0.0343733834884902,
-0.0113626002734257));
#23910=CARTESIAN_POINT('Ctrl Pts',(-0.0138850475166336,-0.0343804288090042,
-0.0114941560716249));
#23911=CARTESIAN_POINT('Ctrl Pts',(-0.0139052095747807,-0.0343827046221997,
-0.0115367498061741));
#23912=CARTESIAN_POINT('Ctrl Pts',(-0.0139290773392635,-0.0343857801539392,
-0.0115937846297097));
#23913=CARTESIAN_POINT('Ctrl Pts',(-0.0139345685567039,-0.0343865191528315,
-0.0116074528995361));
#23914=CARTESIAN_POINT('Ctrl Pts',(-0.0139432035754576,-0.0343877351642379,
-0.0116298690416399));
#23915=CARTESIAN_POINT('Ctrl Pts',(-0.0139464655601267,-0.0343882081750974,
-0.0116385705543616));
#23916=CARTESIAN_POINT('Ctrl Pts',(-0.0139526236571518,-0.0343891283853403,
-0.011655460227402));
#23917=CARTESIAN_POINT('Ctrl Pts',(-0.0139555296322574,-0.0343895752324933,
-0.0116636444318603));
#23918=CARTESIAN_POINT('Ctrl Pts',(-0.0139621662630897,-0.0343906260883323,
-0.0116828480551826));
#23919=CARTESIAN_POINT('Ctrl Pts',(-0.013965841657881,-0.0343912319070737,
-0.0116938858985679));
#23920=CARTESIAN_POINT('Ctrl Pts',(-0.0139775273935811,-0.0343932396398711,
-0.0117303507889806));
#23921=CARTESIAN_POINT('Ctrl Pts',(-0.013985003317691,-0.0343946588963027,
-0.011755942937559));
#23922=CARTESIAN_POINT('Ctrl Pts',(-0.0140013808732151,-0.0343981218848936,
-0.0118179319184796));
#23923=CARTESIAN_POINT('Ctrl Pts',(-0.0140096268551409,-0.0344001846568486,
-0.0118544832622702));
#23924=CARTESIAN_POINT('Ctrl Pts',(-0.0140341595026928,-0.0344076234534603,
-0.0119852290946746));
#23925=CARTESIAN_POINT('Ctrl Pts',(-0.014043,-0.0344131679976405,-0.0120804906866184));
#23926=CARTESIAN_POINT('Ctrl Pts',(-0.014043,-0.0344186209509151,-0.012175853286558));
#23927=CARTESIAN_POINT('Origin',(-0.0125,-0.0375520664398416,-0.0121758532865581));
#23928=CARTESIAN_POINT('',(-0.014043,-0.0349189332996453,-0.0121758532870635));
#23929=CARTESIAN_POINT('',(-0.014043,-0.0348029487958341,-0.0121758532497851));
#23930=CARTESIAN_POINT('',(-0.014043,-0.0375520664398416,-0.012175853286558));
#23931=CARTESIAN_POINT('Ctrl Pts',(-0.014043,-0.0348029487975611,-0.0121758532497038));
#23932=CARTESIAN_POINT('Ctrl Pts',(-0.0140429999991421,-0.0348012580629849,
-0.0121399335435184));
#23933=CARTESIAN_POINT('Ctrl Pts',(-0.014041745734116,-0.0347995408373542,
-0.0121040125839542));
#23934=CARTESIAN_POINT('Ctrl Pts',(-0.01403751176791,-0.0347965809558476,
-0.012043499716227));
#23935=CARTESIAN_POINT('Ctrl Pts',(-0.0140351945091131,-0.0347953584651334,
-0.0120188894748785));
#23936=CARTESIAN_POINT('Ctrl Pts',(-0.014030961674456,-0.0347935516956769,
-0.011983155759407));
#23937=CARTESIAN_POINT('Ctrl Pts',(-0.0140295135721886,-0.0347929821110866,
-0.0119719802638061));
#23938=CARTESIAN_POINT('Ctrl Pts',(-0.0140267445567563,-0.034791970918662,
-0.0119523045466312));
#23939=CARTESIAN_POINT('Ctrl Pts',(-0.0140254747189967,-0.0347915309495704,
-0.0119437975638588));
#23940=CARTESIAN_POINT('Ctrl Pts',(-0.0140226705680918,-0.0347906060983903,
-0.0119260304715128));
#23941=CARTESIAN_POINT('Ctrl Pts',(-0.0140211227541889,-0.0347901208019042,
-0.0119167728756742));
#23942=CARTESIAN_POINT('Ctrl Pts',(-0.0140168326182398,-0.0347888380831219,
-0.0118924782121651));
#23943=CARTESIAN_POINT('Ctrl Pts',(-0.0140139512013873,-0.0347880362541413,
-0.0118774670241026));
#23944=CARTESIAN_POINT('Ctrl Pts',(-0.0140001148026942,-0.0347844303922262,
-0.0118107538762324));
#23945=CARTESIAN_POINT('Ctrl Pts',(-0.0139867318031865,-0.0347815496634318,
-0.0117595965603673));
#23946=CARTESIAN_POINT('Ctrl Pts',(-0.0139408670432501,-0.034773090139021,
-0.0116150351352174));
#23947=CARTESIAN_POINT('Ctrl Pts',(-0.0139020029980949,-0.0347673494112467,
-0.0115239332417468));
#23948=CARTESIAN_POINT('Ctrl Pts',(-0.0138277053165867,-0.0347584755960986,
-0.0113876734085803));
#23949=CARTESIAN_POINT('Ctrl Pts',(-0.013798013594988,-0.0347552923452348,
-0.0113396770781155));
#23950=CARTESIAN_POINT('Ctrl Pts',(-0.0137581520650528,-0.0347515213179414,
-0.0112825004569037));
#23951=CARTESIAN_POINT('Ctrl Pts',(-0.0137504046323687,-0.0347508092782744,
-0.0112716883814002));
#23952=CARTESIAN_POINT('Ctrl Pts',(-0.0137388340669561,-0.0347497776175363,
-0.0112559740766092));
#23953=CARTESIAN_POINT('Ctrl Pts',(-0.0137351197652447,-0.0347494510805446,
-0.0112509928784568));
#23954=CARTESIAN_POINT('Ctrl Pts',(-0.0137284816915407,-0.0347488758708944,
-0.0112422019635401));
#23955=CARTESIAN_POINT('Ctrl Pts',(-0.0137255701010103,-0.0347486263799291,
-0.011238383293038));
#23956=CARTESIAN_POINT('Ctrl Pts',(-0.0137191637439839,-0.034748083555758,
-0.0112300619513505));
#23957=CARTESIAN_POINT('Ctrl Pts',(-0.0137156618268175,-0.0347477907300632,
-0.0112255650096444));
#23958=CARTESIAN_POINT('Ctrl Pts',(-0.0137056972964128,-0.0347469681255311,
-0.011212914413566));
#23959=CARTESIAN_POINT('Ctrl Pts',(-0.013699176909141,-0.034746442277628,
-0.0112048064311313));
#23960=CARTESIAN_POINT('Ctrl Pts',(-0.013648176290168,-0.0347424187219958,
-0.0111426853287046));
#23961=CARTESIAN_POINT('Ctrl Pts',(-0.0136001458317616,-0.0347391448638842,
-0.0110916826586344));
#23962=CARTESIAN_POINT('Ctrl Pts',(-0.0134785476955321,-0.0347315126789831,
-0.0109789943837103));
#23963=CARTESIAN_POINT('Ctrl Pts',(-0.01340237143499,-0.0347272062335571,
-0.0109205635125968));
#23964=CARTESIAN_POINT('Ctrl Pts',(-0.0132939182019669,-0.0347211501204998,
-0.010852378079092));
#23965=CARTESIAN_POINT('Ctrl Pts',(-0.0132660355449561,-0.0347196007418359,
-0.0108360465380061));
#23966=CARTESIAN_POINT('Ctrl Pts',(-0.013216707639586,-0.0347168564646891,
-0.0108091973977016));
#23967=CARTESIAN_POINT('Ctrl Pts',(-0.0131954925442745,-0.0347156752600287,
-0.0107982799842638));
#23968=CARTESIAN_POINT('Ctrl Pts',(-0.0131640355302172,-0.0347139184946066,
-0.0107830039234968));
#23969=CARTESIAN_POINT('Ctrl Pts',(-0.0131539855139859,-0.0347133564706586,
-0.0107782569669066));
#23970=CARTESIAN_POINT('Ctrl Pts',(-0.013136087158528,-0.0347123538342471,
-0.0107700383061924));
#23971=CARTESIAN_POINT('Ctrl Pts',(-0.0131282594335889,-0.0347119147657585,
-0.0107665226963752));
#23972=CARTESIAN_POINT('Ctrl Pts',(-0.0131117400723384,-0.0347109868114844,
-0.0107592684497054));
#23973=CARTESIAN_POINT('Ctrl Pts',(-0.0131030425782815,-0.0347104974573156,
-0.0107555441091177));
#23974=CARTESIAN_POINT('Ctrl Pts',(-0.013079883891889,-0.0347091921786198,
-0.0107458784308514));
#23975=CARTESIAN_POINT('Ctrl Pts',(-0.0130653659692476,-0.0347083715638186,
-0.0107400765934362));
#23976=CARTESIAN_POINT('Ctrl Pts',(-0.0129971769284857,-0.0347045052814919,
-0.0107140205999448));
#23977=CARTESIAN_POINT('Ctrl Pts',(-0.012942496253295,-0.0347013682441913,
-0.0106965508671733));
#23978=CARTESIAN_POINT('Ctrl Pts',(-0.0127936343780978,-0.0346927557600194,
-0.0106579847228088));
#23979=CARTESIAN_POINT('Ctrl Pts',(-0.0126982363183118,-0.0346871497843407,
-0.0106426063059972));
#23980=CARTESIAN_POINT('Ctrl Pts',(-0.0125481484477505,-0.0346785606464023,
-0.010632659369271));
#23981=CARTESIAN_POINT('Ctrl Pts',(-0.0124941049071916,-0.0346755183130572,
-0.0106319193779547));
#23982=CARTESIAN_POINT('Ctrl Pts',(-0.0124271083915702,-0.0346718931775235,
-0.0106345208644435));
#23983=CARTESIAN_POINT('Ctrl Pts',(-0.0124140931256991,-0.0346711958684321,
-0.0106351914635125));
#23984=CARTESIAN_POINT('Ctrl Pts',(-0.0123949373131373,-0.0346701813572464,
-0.0106364219588273));
#23985=CARTESIAN_POINT('Ctrl Pts',(-0.0123887894361534,-0.03466985755058,
-0.0106368538732956));
#23986=CARTESIAN_POINT('Ctrl Pts',(-0.0123783161241449,-0.0346693091732236,
-0.0106376527548753));
#23987=CARTESIAN_POINT('Ctrl Pts',(-0.0123739894365506,-0.0346690835831548,
-0.0106380011542992));
#23988=CARTESIAN_POINT('Ctrl Pts',(-0.0123641395461644,-0.0346685722226116,
-0.0106388361502355));
#23989=CARTESIAN_POINT('Ctrl Pts',(-0.0123586174510793,-0.0346682870993795,
-0.0106393342606434));
#23990=CARTESIAN_POINT('Ctrl Pts',(-0.0123434305523197,-0.0346675069527838,
-0.01064078673296));
#23991=CARTESIAN_POINT('Ctrl Pts',(-0.0123337717363325,-0.0346670152453671,
-0.0106418026063482));
#23992=CARTESIAN_POINT('Ctrl Pts',(-0.0122796699143721,-0.0346642829411992,
-0.0106480097948837));
#23993=CARTESIAN_POINT('Ctrl Pts',(-0.0122354561737832,-0.0346621327194156,
-0.0106550415726527));
#23994=CARTESIAN_POINT('Ctrl Pts',(-0.0121121622172345,-0.0346562196910767,
-0.0106801912180253));
#23995=CARTESIAN_POINT('Ctrl Pts',(-0.0120341153318108,-0.034652568891892,
-0.0107026338102876));
#23996=CARTESIAN_POINT('Ctrl Pts',(-0.0118851068061876,-0.0346452533972879,
-0.0107585149605496));
#23997=CARTESIAN_POINT('Ctrl Pts',(-0.0118142125622679,-0.0346416038930214,
-0.0107914271992862));
#23998=CARTESIAN_POINT('Ctrl Pts',(-0.0117278848647284,-0.034636744087275,
-0.0108397680112178));
#23999=CARTESIAN_POINT('Ctrl Pts',(-0.0117098625537106,-0.0346357055856312,
-0.0108503464368677));
#24000=CARTESIAN_POINT('Ctrl Pts',(-0.011683068762984,-0.0346341225896791,
-0.010866814035145));
#24001=CARTESIAN_POINT('Ctrl Pts',(-0.0116741334895471,-0.0346335879927251,
-0.0108724328219833));
#24002=CARTESIAN_POINT('Ctrl Pts',(-0.0116580867218919,-0.0346326154279782,
-0.0108827547938788));
#24003=CARTESIAN_POINT('Ctrl Pts',(-0.0116509551818055,-0.0346321786627748,
-0.0108874261165389));
#24004=CARTESIAN_POINT('Ctrl Pts',(-0.0116357054653001,-0.0346312347449588,
-0.0108975966232083));
#24005=CARTESIAN_POINT('Ctrl Pts',(-0.0116276002921786,-0.0346307268925758,
-0.0109031145529893));
#24006=CARTESIAN_POINT('Ctrl Pts',(-0.0116057627621163,-0.0346293415456556,
-0.010918287957471));
#24007=CARTESIAN_POINT('Ctrl Pts',(-0.0115921347630105,-0.0346284584335719,
-0.0109280906986019));
#24008=CARTESIAN_POINT('Ctrl Pts',(-0.0115071365015549,-0.0346228303094849,
-0.0109913604379074));
#24009=CARTESIAN_POINT('Ctrl Pts',(-0.0114403638143025,-0.0346178508380652,
-0.0110507006533252));
#24010=CARTESIAN_POINT('Ctrl Pts',(-0.0113198272228724,-0.0346078258708291,
-0.0111781163137375));
#24011=CARTESIAN_POINT('Ctrl Pts',(-0.0112659160124668,-0.0346028078556228,
-0.0112456254768164));
#24012=CARTESIAN_POINT('Ctrl Pts',(-0.0112042216707944,-0.0345965842034982,
-0.0113377517207346));
#24013=CARTESIAN_POINT('Ctrl Pts',(-0.0111910073972785,-0.0345952176661557,
-0.0113585441729841));
#24014=CARTESIAN_POINT('Ctrl Pts',(-0.0111697097040237,-0.0345929681388785,
-0.0113938982932357));
#24015=CARTESIAN_POINT('Ctrl Pts',(-0.0111613541210226,-0.034592072289641,
-0.0114082901699963));
#24016=CARTESIAN_POINT('Ctrl Pts',(-0.0111499180136471,-0.0345908299782384,
-0.0114287430142325));
#24017=CARTESIAN_POINT('Ctrl Pts',(-0.0111466424789714,-0.0345904721865331,
-0.0114346930120205));
#24018=CARTESIAN_POINT('Ctrl Pts',(-0.0111410841852982,-0.0345898618858341,
-0.0114449493529299));
#24019=CARTESIAN_POINT('Ctrl Pts',(-0.0111387823650064,-0.0345896081919407,
-0.0114492452049711));
#24020=CARTESIAN_POINT('Ctrl Pts',(-0.0111339875844909,-0.0345890778025186,
-0.0114582963856109));
#24021=CARTESIAN_POINT('Ctrl Pts',(-0.0111314990500196,-0.0345888013776382,
-0.0114630538918928));
#24022=CARTESIAN_POINT('Ctrl Pts',(-0.0111248289077022,-0.0345880570649138,
-0.0114759693659859));
#24023=CARTESIAN_POINT('Ctrl Pts',(-0.0111206950246796,-0.034587592075028,
-0.0114841518855002));
#24024=CARTESIAN_POINT('Ctrl Pts',(-0.0111012792213883,-0.0345853878878853,
-0.011523449401265));
#24025=CARTESIAN_POINT('Ctrl Pts',(-0.0110869748538561,-0.0345837022660812,
-0.0115550385811138));
#24026=CARTESIAN_POINT('Ctrl Pts',(-0.01104008192827,-0.0345778522521503,
-0.0116686336922188));
#24027=CARTESIAN_POINT('Ctrl Pts',(-0.0110134721977819,-0.0345738843268449,
-0.0117529238063195));
#24028=CARTESIAN_POINT('Ctrl Pts',(-0.0109747091602888,-0.0345657346855752,
-0.0119262162696693));
#24029=CARTESIAN_POINT('Ctrl Pts',(-0.0109628173557519,-0.0345615629243733,
-0.0120149246320466));
#24030=CARTESIAN_POINT('Ctrl Pts',(-0.0109578902189873,-0.0345563116029354,
-0.0121208475924382));
#24031=CARTESIAN_POINT('Ctrl Pts',(-0.0109573850016952,-0.0345554761140637,
-0.0121375499888535));
#24032=CARTESIAN_POINT('Ctrl Pts',(-0.0109570154826123,-0.0345541425670264,
-0.0121639484849535));
#24033=CARTESIAN_POINT('Ctrl Pts',(-0.0109569711456687,-0.0345536501686099,
-0.01217364098189));
#24034=CARTESIAN_POINT('Ctrl Pts',(-0.0109570595178176,-0.0345527186021928,
-0.0121918709027938));
#24035=CARTESIAN_POINT('Ctrl Pts',(-0.0109571717679699,-0.0345522800959843,
-0.0122004080850345));
#24036=CARTESIAN_POINT('Ctrl Pts',(-0.0109575846833157,-0.0345512861226654,
-0.0122196577761233));
#24037=CARTESIAN_POINT('Ctrl Pts',(-0.0109579261096864,-0.0345507293921081,
-0.0122303688938816));
#24038=CARTESIAN_POINT('Ctrl Pts',(-0.0109592672037795,-0.0345490706659133,
-0.0122620676283123));
#24039=CARTESIAN_POINT('Ctrl Pts',(-0.0109605839821037,-0.0345479588055577,
-0.0122830387664267));
#24040=CARTESIAN_POINT('Ctrl Pts',(-0.0109716291063822,-0.0345408367033072,
-0.0124155976015113));
#24041=CARTESIAN_POINT('Ctrl Pts',(-0.010993054851541,-0.034534454179706,
-0.0125258591424952));
#24042=CARTESIAN_POINT('Ctrl Pts',(-0.0110448051221494,-0.0345244015989573,
-0.0126927638524296));
#24043=CARTESIAN_POINT('Ctrl Pts',(-0.0110670350297019,-0.0345207895977096,
-0.0127515274245164));
#24044=CARTESIAN_POINT('Ctrl Pts',(-0.0111013291370773,-0.0345161274986028,
-0.0128277757172094));
#24045=CARTESIAN_POINT('Ctrl Pts',(-0.0111102591466179,-0.0345149787699522,
-0.0128466017260878));
#24046=CARTESIAN_POINT('Ctrl Pts',(-0.0111261345057325,-0.0345130501332825,
-0.0128783905533677));
#24047=CARTESIAN_POINT('Ctrl Pts',(-0.0111328887549882,-0.034512261366232,
-0.0128914452669116));
#24048=CARTESIAN_POINT('Ctrl Pts',(-0.0111428818634372,-0.0345111410406802,
-0.0129101020017497));
#24049=CARTESIAN_POINT('Ctrl Pts',(-0.0111459708455386,-0.0345108008422562,
-0.012915782921158));
#24050=CARTESIAN_POINT('Ctrl Pts',(-0.0111514280551518,-0.0345102105969556,
-0.0129256706053631));
#24051=CARTESIAN_POINT('Ctrl Pts',(-0.0111537804470121,-0.0345099595712933,
-0.0129298859246751));
#24052=CARTESIAN_POINT('Ctrl Pts',(-0.0111588718750154,-0.0345094235687743,
-0.0129389096228454));
#24053=CARTESIAN_POINT('Ctrl Pts',(-0.0111616170232771,-0.0345091389843756,
-0.0129437143608758));
#24054=CARTESIAN_POINT('Ctrl Pts',(-0.0111692270630409,-0.0345083617834544,
-0.0129568691490597));
#24055=CARTESIAN_POINT('Ctrl Pts',(-0.0111741447184453,-0.0345078724419543,
-0.0129651885566677));
#24056=CARTESIAN_POINT('Ctrl Pts',(-0.0112017872861205,-0.0345051889368049,
-0.013010965363179));
#24057=CARTESIAN_POINT('Ctrl Pts',(-0.0112260230999787,-0.0345030813511353,
-0.013047490756475));
#24058=CARTESIAN_POINT('Ctrl Pts',(-0.0112998359588708,-0.0344971748629624,
-0.0131490629118939));
#24059=CARTESIAN_POINT('Ctrl Pts',(-0.0113530696020962,-0.0344934948411737,
-0.0132112674077798));
#24060=CARTESIAN_POINT('Ctrl Pts',(-0.0114664916952165,-0.0344861362843386,
-0.0133242648397486));
#24061=CARTESIAN_POINT('Ctrl Pts',(-0.0115261285457597,-0.0344824737558901,
-0.0133752536876955));
#24062=CARTESIAN_POINT('Ctrl Pts',(-0.0116062743455237,-0.0344775977020852,
-0.013433844410628));
#24063=CARTESIAN_POINT('Ctrl Pts',(-0.0116234227475888,-0.0344765573886726,
-0.0134458530824239));
#24064=CARTESIAN_POINT('Ctrl Pts',(-0.0116495830095334,-0.0344749721775005,
-0.0134633902784696));
#24065=CARTESIAN_POINT('Ctrl Pts',(-0.0116584163806167,-0.0344744372198324,
-0.0134691813839847));
#24066=CARTESIAN_POINT('Ctrl Pts',(-0.0116744860615738,-0.0344734642718251,
-0.0134794822313509));
#24067=CARTESIAN_POINT('Ctrl Pts',(-0.0116817016621884,-0.0344730274885644,
-0.0134840235792547));
#24068=CARTESIAN_POINT('Ctrl Pts',(-0.0116972911702999,-0.0344720838399689,
-0.0134936558395733));
#24069=CARTESIAN_POINT('Ctrl Pts',(-0.0117056766547608,-0.0344715762783654,
-0.0134987272228245));
#24070=CARTESIAN_POINT('Ctrl Pts',(-0.011728535198581,-0.0344701925037559,
-0.0135122559372665));
#24071=CARTESIAN_POINT('Ctrl Pts',(-0.0117430984048055,-0.0344693106944539,
-0.0135205576889706));
#24072=CARTESIAN_POINT('Ctrl Pts',(-0.0118355791730597,-0.034463708092659,
-0.013571297998802));
#24073=CARTESIAN_POINT('Ctrl Pts',(-0.0119168898298866,-0.0344587553480055,
-0.0136071812099891));
#24074=CARTESIAN_POINT('Ctrl Pts',(-0.0120828077546296,-0.0344487351974828,
-0.0136639080563882));
#24075=CARTESIAN_POINT('Ctrl Pts',(-0.0121670083159569,-0.0344436930623477,
-0.0136849832016467));
#24076=CARTESIAN_POINT('Ctrl Pts',(-0.0122769000602528,-0.0344374432036704,
-0.0137028388305269));
#24077=CARTESIAN_POINT('Ctrl Pts',(-0.0123013598632317,-0.0344360734899141,
-0.0137062129303402));
#24078=CARTESIAN_POINT('Ctrl Pts',(-0.0123424517868188,-0.0344338193407467,
-0.013710879460063));
#24079=CARTESIAN_POINT('Ctrl Pts',(-0.0123590425179456,-0.0344329219829101,
-0.0137124917688753));
#24080=CARTESIAN_POINT('Ctrl Pts',(-0.0123824308491513,-0.0344316779667341,
-0.0137143826762979));
#24081=CARTESIAN_POINT('Ctrl Pts',(-0.0123892086150432,-0.0344313199386283,
-0.0137148855996492));
#24082=CARTESIAN_POINT('Ctrl Pts',(-0.012400852788297,-0.0344307093644327,
-0.013715672298297));
#24083=CARTESIAN_POINT('Ctrl Pts',(-0.0124057175844363,-0.0344304556306669,
-0.0137159778227638));
#24084=CARTESIAN_POINT('Ctrl Pts',(-0.0124159419035796,-0.0344299252977918,
-0.0137165713143825));
#24085=CARTESIAN_POINT('Ctrl Pts',(-0.0124213015638884,-0.0344296489678495,
-0.0137168543776347));
#24086=CARTESIAN_POINT('Ctrl Pts',(-0.0124358106491749,-0.034428905190079,
-0.0137175447609512));
#24087=CARTESIAN_POINT('Ctrl Pts',(-0.0124449625339696,-0.0344284406330838,
-0.0137178986036904));
#24088=CARTESIAN_POINT('Ctrl Pts',(-0.0124886603330122,-0.0344262421684204,
-0.0137191985795725));
#24089=CARTESIAN_POINT('Ctrl Pts',(-0.0125232305406614,-0.0344245614994274,
-0.0137190655004037));
#24090=CARTESIAN_POINT('Ctrl Pts',(-0.0126460070657806,-0.0344187120481743,
-0.013714465577828));
#24091=CARTESIAN_POINT('Ctrl Pts',(-0.0127338029101666,-0.0344147407483755,
-0.0137035914232518));
#24092=CARTESIAN_POINT('Ctrl Pts',(-0.0129076304177375,-0.0344065857117213,
-0.0136667175489091));
#24093=CARTESIAN_POINT('Ctrl Pts',(-0.012993286343299,-0.0344024120093137,
-0.0136406075715908));
#24094=CARTESIAN_POINT('Ctrl Pts',(-0.0130916959270272,-0.034397158417778,
-0.0136009933410134));
#24095=CARTESIAN_POINT('Ctrl Pts',(-0.0131070949117104,-0.034396322868048,
-0.0135945019342409));
#24096=CARTESIAN_POINT('Ctrl Pts',(-0.0131312543787784,-0.0343949892459798,
-0.0135838521713802));
#24097=CARTESIAN_POINT('Ctrl Pts',(-0.0131400865170009,-0.0343944968345006,
-0.0135798590541857));
#24098=CARTESIAN_POINT('Ctrl Pts',(-0.0131566265255959,-0.0343935652570884,
-0.0135721926080917));
#24099=CARTESIAN_POINT('Ctrl Pts',(-0.0131643426920788,-0.034393126753125,
-0.0135685379883299));
#24100=CARTESIAN_POINT('Ctrl Pts',(-0.0131816743247193,-0.0343921328035431,
-0.0135601523686827));
#24101=CARTESIAN_POINT('Ctrl Pts',(-0.0131912715675292,-0.0343915760947242,
-0.0135553848903495));
#24102=CARTESIAN_POINT('Ctrl Pts',(-0.0132201729881524,-0.0343898800699295,
-0.0135406506478272));
#24103=CARTESIAN_POINT('Ctrl Pts',(-0.0132393164956937,-0.0343887299648524,
-0.0135303760897539));
#24104=CARTESIAN_POINT('Ctrl Pts',(-0.0133439590897324,-0.034382291844298,
-0.0134713338477309));
#24105=CARTESIAN_POINT('Ctrl Pts',(-0.0134248458984153,-0.0343767256154551,
-0.0134148819204856));
#24106=CARTESIAN_POINT('Ctrl Pts',(-0.0135550778538552,-0.0343669025282936,
-0.0133040941262781));
#24107=CARTESIAN_POINT('Ctrl Pts',(-0.0136069739435985,-0.0343627037007513,
-0.0132532232252696));
#24108=CARTESIAN_POINT('Ctrl Pts',(-0.013677372847466,-0.0343567640962357,
-0.0131737365056892));
#24109=CARTESIAN_POINT('Ctrl Pts',(-0.0136988222322934,-0.0343549168131173,
-0.0131478632159134));
#24110=CARTESIAN_POINT('Ctrl Pts',(-0.0137247641618978,-0.0343526552957386,
-0.0131144043359448));
#24111=CARTESIAN_POINT('Ctrl Pts',(-0.0137300586754671,-0.0343521922225408,
-0.013107454588873));
#24112=CARTESIAN_POINT('Ctrl Pts',(-0.0137384545114311,-0.0343514559544015,
-0.0130962375767377));
#24113=CARTESIAN_POINT('Ctrl Pts',(-0.0137415934031003,-0.034351180244284,
-0.0130919988216753));
#24114=CARTESIAN_POINT('Ctrl Pts',(-0.0137475817111962,-0.0343506535243498,
-0.0130838249142345));
#24115=CARTESIAN_POINT('Ctrl Pts',(-0.0137504343479523,-0.03435040230315,
-0.0130798923037048));
#24116=CARTESIAN_POINT('Ctrl Pts',(-0.0137573439934643,-0.0343497928862808,
-0.0130702714750008));
#24117=CARTESIAN_POINT('Ctrl Pts',(-0.0137613810865214,-0.0343494360404971,
-0.013064568973313));
#24118=CARTESIAN_POINT('Ctrl Pts',(-0.0137728329372339,-0.0343484209271794,
-0.0130481576846542));
#24119=CARTESIAN_POINT('Ctrl Pts',(-0.0137801511740157,-0.0343477687156927,
-0.0130373819519556));
#24120=CARTESIAN_POINT('Ctrl Pts',(-0.0138318843500512,-0.034343122660757,
-0.0129590925156564));
#24121=CARTESIAN_POINT('Ctrl Pts',(-0.0138710754892787,-0.0343394053229053,
-0.0128882676210948));
#24122=CARTESIAN_POINT('Ctrl Pts',(-0.0139500787897683,-0.0343306739126644,
-0.012714572418188));
#24123=CARTESIAN_POINT('Ctrl Pts',(-0.0139847782156196,-0.0343256821182595,
-0.0126098792706016));
#24124=CARTESIAN_POINT('Ctrl Pts',(-0.0140132724251587,-0.0343191116588909,
-0.0124782832610245));
#24125=CARTESIAN_POINT('Ctrl Pts',(-0.0140179130323191,-0.0343178916782183,
-0.0124540569241657));
#24126=CARTESIAN_POINT('Ctrl Pts',(-0.0140238234510058,-0.0343160879454099,
-0.0124186245096236));
#24127=CARTESIAN_POINT('Ctrl Pts',(-0.0140255543805702,-0.0343155188157125,
-0.0124074987048593));
#24128=CARTESIAN_POINT('Ctrl Pts',(-0.0140283923323993,-0.0343145081406761,
-0.0123878434683056));
#24129=CARTESIAN_POINT('Ctrl Pts',(-0.0140295501047151,-0.0343140682283638,
-0.0123793217904838));
#24130=CARTESIAN_POINT('Ctrl Pts',(-0.0140318229146649,-0.0343131432033015,
-0.0123614758534347));
#24131=CARTESIAN_POINT('Ctrl Pts',(-0.0140329241873776,-0.0343126576730004,
-0.0123521502228244));
#24132=CARTESIAN_POINT('Ctrl Pts',(-0.0140355963351681,-0.0343113736545842,
-0.0123276002306477));
#24133=CARTESIAN_POINT('Ctrl Pts',(-0.0140370259083655,-0.0343105707436344,
-0.012312361798405));
#24134=CARTESIAN_POINT('Ctrl Pts',(-0.0140414088711038,-0.0343076187357149,
-0.0122567584652518));
#24135=CARTESIAN_POINT('Ctrl Pts',(-0.0140430000002715,-0.0343054280631435,
-0.0122163101074072));
#24136=CARTESIAN_POINT('Ctrl Pts',(-0.014043,-0.0343031952477557,-0.0121758532762046));
#24137=CARTESIAN_POINT('Ctrl Pts',(-0.014043,-0.0344186209509151,-0.012175853286558));
#24138=CARTESIAN_POINT('Ctrl Pts',(-0.014043,-0.0344212507268401,-0.0122218434604753));
#24139=CARTESIAN_POINT('Ctrl Pts',(-0.0140409438983355,-0.0344238559182217,
-0.0122678573148423));
#24140=CARTESIAN_POINT('Ctrl Pts',(-0.0140349925434263,-0.0344275142554532,
-0.0123341798515428));
#24141=CARTESIAN_POINT('Ctrl Pts',(-0.014032753055036,-0.0344286252473827,
-0.0123545641161567));
#24142=CARTESIAN_POINT('Ctrl Pts',(-0.014029127197785,-0.0344301204238227,
-0.0123824369283828));
#24143=CARTESIAN_POINT('Ctrl Pts',(-0.0140280908529206,-0.0344305220049617,
-0.0123899680641488));
#24144=CARTESIAN_POINT('Ctrl Pts',(-0.0140263465288212,-0.0344311586276199,
-0.0124019857676221));
#24145=CARTESIAN_POINT('Ctrl Pts',(-0.0140256743384956,-0.0344313956230572,
-0.0124064773073147));
#24146=CARTESIAN_POINT('Ctrl Pts',(-0.0140242176896289,-0.0344318920770031,
-0.012415925392678));
#24147=CARTESIAN_POINT('Ctrl Pts',(-0.0140234288656404,-0.0344321512710044,
-0.0124208811903783));
#24148=CARTESIAN_POINT('Ctrl Pts',(-0.014021402918539,-0.0344327938360067,
-0.0124332211438851));
#24149=CARTESIAN_POINT('Ctrl Pts',(-0.0140201361843025,-0.0344331755607431,
-0.0124406004113445));
#24150=CARTESIAN_POINT('Ctrl Pts',(-0.0140150577362094,-0.0344346331018128,
-0.0124689456686067));
#24151=CARTESIAN_POINT('Ctrl Pts',(-0.0140108654191812,-0.0344356891821672,
-0.0124898419133742));
#24152=CARTESIAN_POINT('Ctrl Pts',(-0.0139986874897082,-0.0344384250248136,
-0.0125446308192381));
#24153=CARTESIAN_POINT('Ctrl Pts',(-0.0139899851396795,-0.0344400752532725,
-0.0125783524600527));
#24154=CARTESIAN_POINT('Ctrl Pts',(-0.0139614688427985,-0.0344447874594057,
-0.012675183064974));
#24155=CARTESIAN_POINT('Ctrl Pts',(-0.0139387301644725,-0.0344477820149067,
-0.0127373489605207));
#24156=CARTESIAN_POINT('Ctrl Pts',(-0.0138746491574022,-0.034455067885897,
-0.0128828236496189));
#24157=CARTESIAN_POINT('Ctrl Pts',(-0.0138296375007157,-0.0344593888479459,
-0.0129642244645762));
#24158=CARTESIAN_POINT('Ctrl Pts',(-0.0137681720549098,-0.0344648141028137,
-0.013054983881949));
#24159=CARTESIAN_POINT('Ctrl Pts',(-0.0137585300794762,-0.0344656532479546,
-0.0130687323241851));
#24160=CARTESIAN_POINT('Ctrl Pts',(-0.0137428898990631,-0.0344669973190432,
-0.0130902768021956));
#24161=CARTESIAN_POINT('Ctrl Pts',(-0.0137370380960509,-0.0344674965869797,
-0.0130981777469375));
#24162=CARTESIAN_POINT('Ctrl Pts',(-0.0137259487763708,-0.0344684362777711,
-0.0131128548529574));
#24163=CARTESIAN_POINT('Ctrl Pts',(-0.0137207295603245,-0.0344688759688194,
-0.0131196444045108));
#24164=CARTESIAN_POINT('Ctrl Pts',(-0.0137089099485386,-0.0344698661564612,
-0.0131347581766962));
#24165=CARTESIAN_POINT('Ctrl Pts',(-0.0137022796029769,-0.0344704178421874,
-0.0131430583323764));
#24166=CARTESIAN_POINT('Ctrl Pts',(-0.0136822220287321,-0.0344720759439644,
-0.0131676423327415));
#24167=CARTESIAN_POINT('Ctrl Pts',(-0.0136685462341116,-0.0344731924098364,
-0.013183719387019));
#24168=CARTESIAN_POINT('Ctrl Pts',(-0.013601830900007,-0.0344785752545321,
-0.0132589651751012));
#24169=CARTESIAN_POINT('Ctrl Pts',(-0.0135446091033189,-0.0344830159552006,
-0.0133142520737316));
#24170=CARTESIAN_POINT('Ctrl Pts',(-0.0134185518572565,-0.0344923550363818,
-0.0134185082873221));
#24171=CARTESIAN_POINT('Ctrl Pts',(-0.0133494350079558,-0.0344972493751752,
-0.0134667402443044));
#24172=CARTESIAN_POINT('Ctrl Pts',(-0.0132418511657536,-0.0345042684666625,
-0.0135294172345303));
#24173=CARTESIAN_POINT('Ctrl Pts',(-0.0132061847201313,-0.0345065049803165,
-0.0135483627201609));
#24174=CARTESIAN_POINT('Ctrl Pts',(-0.0131611701940534,-0.0345091814720202,
-0.0135700537865768));
#24175=CARTESIAN_POINT('Ctrl Pts',(-0.0131524877115586,-0.0345096911585609,
-0.013574138255789));
#24176=CARTESIAN_POINT('Ctrl Pts',(-0.0131387902837861,-0.0345104843077879,
-0.0135804265195531));
#24177=CARTESIAN_POINT('Ctrl Pts',(-0.0131338008787443,-0.0345107709621863,
-0.0135826849898683));
#24178=CARTESIAN_POINT('Ctrl Pts',(-0.013124353670445,-0.0345113093241089,
-0.0135869008390902));
#24179=CARTESIAN_POINT('Ctrl Pts',(-0.0131198985359548,-0.0345115613494253,
-0.0135888637276754));
#24180=CARTESIAN_POINT('Ctrl Pts',(-0.0131093386806568,-0.0345121544506331,
-0.0135934567415438));
#24181=CARTESIAN_POINT('Ctrl Pts',(-0.0131032260643617,-0.0345124944268501,
-0.0135960685877475));
#24182=CARTESIAN_POINT('Ctrl Pts',(-0.0130826620287619,-0.0345136275953856,
-0.0136046986297439));
#24183=CARTESIAN_POINT('Ctrl Pts',(-0.0130681355260242,-0.0345144106331394,
-0.0136105365666277));
#24184=CARTESIAN_POINT('Ctrl Pts',(-0.0130323805919522,-0.0345163013261759,
-0.0136242775637009));
#24185=CARTESIAN_POINT('Ctrl Pts',(-0.0130110618042765,-0.0345173974993715,
-0.0136319363528153));
#24186=CARTESIAN_POINT('Ctrl Pts',(-0.0129203948004886,-0.0345219585292715,
-0.0136622717458253));
#24187=CARTESIAN_POINT('Ctrl Pts',(-0.0128496497782722,-0.0345252747761337,
-0.0136804854118785));
#24188=CARTESIAN_POINT('Ctrl Pts',(-0.012681684620417,-0.0345330813399018,
-0.0137112369833737));
#24189=CARTESIAN_POINT('Ctrl Pts',(-0.0125840398651382,-0.0345375805294642,
-0.0137196627070563));
#24190=CARTESIAN_POINT('Ctrl Pts',(-0.0124644990598134,-0.0345434431340746,
-0.0137185983581558));
#24191=CARTESIAN_POINT('Ctrl Pts',(-0.012442743171024,-0.0345445235251208,
-0.0137179441623546));
#24192=CARTESIAN_POINT('Ctrl Pts',(-0.0124102721184903,-0.0345461590552488,
-0.0137162796858622));
#24193=CARTESIAN_POINT('Ctrl Pts',(-0.0123995414261918,-0.0345467033036156,
-0.0137156171164198));
#24194=CARTESIAN_POINT('Ctrl Pts',(-0.0123802671483107,-0.0345476879542266,
-0.0137142246835322));
#24195=CARTESIAN_POINT('Ctrl Pts',(-0.0123717210068596,-0.0345481270513804,
-0.0137135356356726));
#24196=CARTESIAN_POINT('Ctrl Pts',(-0.0123534764071276,-0.0345490699698217,
-0.0137119114773233));
#24197=CARTESIAN_POINT('Ctrl Pts',(-0.0123437802057966,-0.0345495744283035,
-0.013710955660578));
#24198=CARTESIAN_POINT('Ctrl Pts',(-0.012317367260995,-0.0345509579434118,
-0.0137080991329777));
#24199=CARTESIAN_POINT('Ctrl Pts',(-0.0123006718484562,-0.0345518426943833,
-0.0137060167774706));
#24200=CARTESIAN_POINT('Ctrl Pts',(-0.0121929255386265,-0.0345576205837428,
-0.0136907847209407));
#24201=CARTESIAN_POINT('Ctrl Pts',(-0.0121031840000439,-0.03456276464901,
-0.0136697892702447));
#24202=CARTESIAN_POINT('Ctrl Pts',(-0.0119278500652107,-0.0345733294245694,
-0.0136118493040906));
#24203=CARTESIAN_POINT('Ctrl Pts',(-0.0118426414073102,-0.0345787284675585,
-0.0135748959628348));
#24204=CARTESIAN_POINT('Ctrl Pts',(-0.011736278603535,-0.0345854665044419,
-0.0135168933738501));
#24205=CARTESIAN_POINT('Ctrl Pts',(-0.0117116738317919,-0.0345870239106572,
-0.0135025789304071));
#24206=CARTESIAN_POINT('Ctrl Pts',(-0.0116801682658603,-0.0345890025386721,
-0.0134830636198682));
#24207=CARTESIAN_POINT('Ctrl Pts',(-0.011672896614481,-0.0345894581002025,
-0.0134784748448617));
#24208=CARTESIAN_POINT('Ctrl Pts',(-0.0116612403164175,-0.0345901860513018,
-0.0134709821767271));
#24209=CARTESIAN_POINT('Ctrl Pts',(-0.0116568315909705,-0.0345904608443533,
-0.0134681162956237));
#24210=CARTESIAN_POINT('Ctrl Pts',(-0.0116482954647415,-0.0345909917094007,
-0.0134625051255732));
#24211=CARTESIAN_POINT('Ctrl Pts',(-0.011644166533352,-0.0345912479316971,
-0.013459762414175));
#24212=CARTESIAN_POINT('Ctrl Pts',(-0.011634093270176,-0.0345918718315033,
-0.0134530008972992));
#24213=CARTESIAN_POINT('Ctrl Pts',(-0.0116281635339138,-0.0345922380702319,
-0.0134489603773653));
#24214=CARTESIAN_POINT('Ctrl Pts',(-0.0116065999958337,-0.0345935669625945,
-0.0134340456745451));
#24215=CARTESIAN_POINT('Ctrl Pts',(-0.0115911391205138,-0.0345945140808452,
-0.0134229232989986));
#24216=CARTESIAN_POINT('Ctrl Pts',(-0.0115521392417426,-0.0345968992515924,
-0.0133937565659356));
#24217=CARTESIAN_POINT('Ctrl Pts',(-0.0115289068157599,-0.0345983163853198,
-0.0133753142510458));
#24218=CARTESIAN_POINT('Ctrl Pts',(-0.0114514862346744,-0.0346030787644519,
-0.0133101315167793));
#24219=CARTESIAN_POINT('Ctrl Pts',(-0.0114000225827501,-0.0346063175145695,
-0.0132602972377898));
#24220=CARTESIAN_POINT('Ctrl Pts',(-0.0112883237706678,-0.0346139721258716,
-0.0131359705705696));
#24221=CARTESIAN_POINT('Ctrl Pts',(-0.0112311951148977,-0.0346184113773414,
-0.0130590951188015));
#24222=CARTESIAN_POINT('Ctrl Pts',(-0.0111728350093234,-0.0346239717535003,
-0.0129631038363583));
#24223=CARTESIAN_POINT('Ctrl Pts',(-0.0111643558936737,-0.034624809994748,
-0.0129486308316105));
#24224=CARTESIAN_POINT('Ctrl Pts',(-0.0111512856205181,-0.0346261529418966,
-0.0129254632569788));
#24225=CARTESIAN_POINT('Ctrl Pts',(-0.0111465386009794,-0.0346266520062032,
-0.0129168578889023));
#24226=CARTESIAN_POINT('Ctrl Pts',(-0.0111378093737311,-0.0346275915178356,
-0.012900669844358));
#24227=CARTESIAN_POINT('Ctrl Pts',(-0.0111338074505789,-0.0346280312360786,
-0.0128930981950225));
#24228=CARTESIAN_POINT('Ctrl Pts',(-0.0111249804694063,-0.0346290217558974,
-0.0128760555893368));
#24229=CARTESIAN_POINT('Ctrl Pts',(-0.0111201898570151,-0.0346295737501186,
-0.0128665673634514));
#24230=CARTESIAN_POINT('Ctrl Pts',(-0.0111061675002692,-0.0346312337242514,
-0.0128380667285328));
#24231=CARTESIAN_POINT('Ctrl Pts',(-0.0110972282144649,-0.0346323517877049,
-0.0128189138885718));
#24232=CARTESIAN_POINT('Ctrl Pts',(-0.0110564691595448,-0.0346377492536229,
-0.0127266884485972));
#24233=CARTESIAN_POINT('Ctrl Pts',(-0.0110299528350907,-0.0346422040800077,
-0.0126514153285098));
#24234=CARTESIAN_POINT('Ctrl Pts',(-0.0109875065077053,-0.0346515861904159,
-0.0124926748650385));
#24235=CARTESIAN_POINT('Ctrl Pts',(-0.01097240774431,-0.0346565098378627,
-0.0124092508181465));
#24236=CARTESIAN_POINT('Ctrl Pts',(-0.0109603913409666,-0.0346635128933569,
-0.0122855251281353));
#24237=CARTESIAN_POINT('Ctrl Pts',(-0.010958080395888,-0.0346657093357846,
-0.0122459042652407));
#24238=CARTESIAN_POINT('Ctrl Pts',(-0.0109571111242769,-0.034668345670086,
-0.0121966884258337));
#24239=CARTESIAN_POINT('Ctrl Pts',(-0.0109570117242127,-0.0346688528747534,
-0.0121871393696784));
#24240=CARTESIAN_POINT('Ctrl Pts',(-0.010956994824899,-0.0346696430421348,
-0.0121721230666707));
#24241=CARTESIAN_POINT('Ctrl Pts',(-0.0109570177247147,-0.0346699291585376,
-0.0121666562813285));
#24242=CARTESIAN_POINT('Ctrl Pts',(-0.0109571159709193,-0.0346704671196264,
-0.0121563186645673));
#24243=CARTESIAN_POINT('Ctrl Pts',(-0.010957185328934,-0.0346707192749122,
-0.0121514479661761));
#24244=CARTESIAN_POINT('Ctrl Pts',(-0.0109574042410045,-0.0346713134964511,
-0.0121399120923173));
#24245=CARTESIAN_POINT('Ctrl Pts',(-0.0109575739297537,-0.0346716544506249,
-0.0121332473469337));
#24246=CARTESIAN_POINT('Ctrl Pts',(-0.0109582904115228,-0.0346727944660679,
-0.0121108203325944));
#24247=CARTESIAN_POINT('Ctrl Pts',(-0.0109590356851479,-0.0346735832046999,
-0.0120950649399482));
#24248=CARTESIAN_POINT('Ctrl Pts',(-0.0109614536953316,-0.0346754904615439,
-0.0120564896014039));
#24249=CARTESIAN_POINT('Ctrl Pts',(-0.0109633926884691,-0.03467659723158,
-0.0120336897343118));
#24250=CARTESIAN_POINT('Ctrl Pts',(-0.0109737857491623,-0.0346812339026118,
-0.0119370044324663));
#24251=CARTESIAN_POINT('Ctrl Pts',(-0.0109870682727495,-0.0346846102113984,
-0.0118637354869106));
#24252=CARTESIAN_POINT('Ctrl Pts',(-0.0110294743414793,-0.0346923988376801,
-0.0116987662729677));
#24253=CARTESIAN_POINT('Ctrl Pts',(-0.0110619818392575,-0.0346968199988048,
-0.011608262439399));
#24254=CARTESIAN_POINT('Ctrl Pts',(-0.0111119193099963,-0.0347025934885319,
-0.0115016460443384));
#24255=CARTESIAN_POINT('Ctrl Pts',(-0.0111215742441188,-0.034703674693506,
-0.0114821200642037));
#24256=CARTESIAN_POINT('Ctrl Pts',(-0.0111366086924991,-0.0347053112167356,
-0.0114532684840331));
#24257=CARTESIAN_POINT('Ctrl Pts',(-0.0111416779145405,-0.0347058556241761,
-0.0114437837825054));
#24258=CARTESIAN_POINT('Ctrl Pts',(-0.0111509661488267,-0.0347068404469925,
-0.0114268338048159));
#24259=CARTESIAN_POINT('Ctrl Pts',(-0.0111551490551011,-0.0347072795552926,
-0.0114193491902687));
#24260=CARTESIAN_POINT('Ctrl Pts',(-0.0111642169170902,-0.0347082223703798,
-0.0114034366618691));
#24261=CARTESIAN_POINT('Ctrl Pts',(-0.0111691197225938,-0.0347087267129308,
-0.0113950193938277));
#24262=CARTESIAN_POINT('Ctrl Pts',(-0.011182701766812,-0.034710109577188,
-0.0113722009507238));
#24263=CARTESIAN_POINT('Ctrl Pts',(-0.0111915370541682,-0.0347109937842608,
-0.0113578946071711));
#24264=CARTESIAN_POINT('Ctrl Pts',(-0.0112499986394791,-0.0347167496779284,
-0.0112666037139836));
#24265=CARTESIAN_POINT('Ctrl Pts',(-0.0113061556332917,-0.0347218699466105,
-0.011194033775052));
#24266=CARTESIAN_POINT('Ctrl Pts',(-0.0114309511580672,-0.0347323707039697,
-0.0110594091082525));
#24267=CARTESIAN_POINT('Ctrl Pts',(-0.0114994045822469,-0.0347377292348476,
-0.01099766722472));
#24268=CARTESIAN_POINT('Ctrl Pts',(-0.0115964408072155,-0.034744488767067,
-0.010924736496737));
#24269=CARTESIAN_POINT('Ctrl Pts',(-0.011620431400459,-0.0347460985075692,
-0.0109077556060341));
#24270=CARTESIAN_POINT('Ctrl Pts',(-0.0116521282506485,-0.034748132193312,
-0.010886652745782));
#24271=CARTESIAN_POINT('Ctrl Pts',(-0.0116594035212191,-0.0347485928061274,
-0.0108818972964116));
#24272=CARTESIAN_POINT('Ctrl Pts',(-0.0116711615260432,-0.0347493268534591,
-0.0108743527491169));
#24273=CARTESIAN_POINT('Ctrl Pts',(-0.01167561897002,-0.034749602761412,
-0.0108715248064854));
#24274=CARTESIAN_POINT('Ctrl Pts',(-0.0116842805814157,-0.0347501341877967,
-0.0108660917472102));
#24275=CARTESIAN_POINT('Ctrl Pts',(-0.0116884828674735,-0.0347503898732507,
-0.0108634839011457));
#24276=CARTESIAN_POINT('Ctrl Pts',(-0.011698761429683,-0.0347510102205853,
-0.0108571734990464));
#24277=CARTESIAN_POINT('Ctrl Pts',(-0.0117048510011,-0.0347513734828541,
-0.0108534926315561));
#24278=CARTESIAN_POINT('Ctrl Pts',(-0.0117269779680434,-0.0347526788612845,
-0.0108403260104871));
#24279=CARTESIAN_POINT('Ctrl Pts',(-0.0117431619490734,-0.034753606152339,
-0.0108310884782717));
#24280=CARTESIAN_POINT('Ctrl Pts',(-0.0117847432090315,-0.0347559295268815,
-0.0108083431553214));
#24281=CARTESIAN_POINT('Ctrl Pts',(-0.0118103586684988,-0.0347573060424203,
-0.0107952479045287));
#24282=CARTESIAN_POINT('Ctrl Pts',(-0.0119493823579586,-0.034764563769676,
-0.0107290111082644));
#24283=CARTESIAN_POINT('Ctrl Pts',(-0.0120685763625761,-0.0347700819971045,
-0.0106891089616857));
#24284=CARTESIAN_POINT('Ctrl Pts',(-0.0122378970252888,-0.0347782528460791,
-0.0106545334591239));
#24285=CARTESIAN_POINT('Ctrl Pts',(-0.0122849180065759,-0.0347805502851189,
-0.0106471769961609));
#24286=CARTESIAN_POINT('Ctrl Pts',(-0.0123468933462481,-0.0347836511966907,
-0.0106403970701265));
#24287=CARTESIAN_POINT('Ctrl Pts',(-0.0123616074013197,-0.0347843926393942,
-0.0106390010134324));
#24288=CARTESIAN_POINT('Ctrl Pts',(-0.012385612520354,-0.0347856116538727,
-0.0106370709562861));
#24289=CARTESIAN_POINT('Ctrl Pts',(-0.0123948925285678,-0.0347860851851846,
-0.0106364092408305));
#24290=CARTESIAN_POINT('Ctrl Pts',(-0.0124128416008519,-0.0347870056835294,
-0.0106352924259929));
#24291=CARTESIAN_POINT('Ctrl Pts',(-0.0124215096514107,-0.0347874522899658,
-0.0106348264818894));
#24292=CARTESIAN_POINT('Ctrl Pts',(-0.0124417753208816,-0.0347885014552659,
-0.0106339085438657));
#24293=CARTESIAN_POINT('Ctrl Pts',(-0.0124533749188357,-0.034789105807075,
-0.010633514220517));
#24294=CARTESIAN_POINT('Ctrl Pts',(-0.0124914671727522,-0.0347911034375968,
-0.0106326493962043));
#24295=CARTESIAN_POINT('Ctrl Pts',(-0.0125179665803499,-0.0347925138192516,
-0.0106327304330261));
#24296=CARTESIAN_POINT('Ctrl Pts',(-0.0126295277406936,-0.0347985404059354,
-0.0106359455470927));
#24297=CARTESIAN_POINT('Ctrl Pts',(-0.0127142470947548,-0.0348033462275276,
-0.0106454323101142));
#24298=CARTESIAN_POINT('Ctrl Pts',(-0.0129006082005719,-0.0348142427166544,
-0.0106820820321214));
#24299=CARTESIAN_POINT('Ctrl Pts',(-0.0130011488008545,-0.0348203490665612,
-0.010712742995192));
#24300=CARTESIAN_POINT('Ctrl Pts',(-0.0131098159395933,-0.0348267247793116,
-0.0107584107980874));
#24301=CARTESIAN_POINT('Ctrl Pts',(-0.0131217610027258,-0.0348274221141635,
-0.0107636096936498));
#24302=CARTESIAN_POINT('Ctrl Pts',(-0.0131392927328714,-0.0348284388279881,
-0.0107715056629536));
#24303=CARTESIAN_POINT('Ctrl Pts',(-0.0131449309932392,-0.0348287647621707,
-0.0107740860224269));
#24304=CARTESIAN_POINT('Ctrl Pts',(-0.0131549318099693,-0.034829340815958,
-0.0107787360271017));
#24305=CARTESIAN_POINT('Ctrl Pts',(-0.01315930040594,-0.0348295917318798,
-0.0107807922523895));
#24306=CARTESIAN_POINT('Ctrl Pts',(-0.0131687873096692,-0.034830135021877,
-0.0107853120977104));
#24307=CARTESIAN_POINT('Ctrl Pts',(-0.0131739017150181,-0.0348304269145063,
-0.0107877834958212));
#24308=CARTESIAN_POINT('Ctrl Pts',(-0.0131884712285375,-0.0348312559053572,
-0.01079492332561));
#24309=CARTESIAN_POINT('Ctrl Pts',(-0.0131978924551705,-0.0348317889037202,
-0.0107996605957608));
#24310=CARTESIAN_POINT('Ctrl Pts',(-0.0132771326879101,-0.0348362519471852,
-0.0108405279466831));
#24311=CARTESIAN_POINT('Ctrl Pts',(-0.0133441528350246,-0.0348398985544469,
-0.0108818526568864));
#24312=CARTESIAN_POINT('Ctrl Pts',(-0.0135092295622997,-0.0348492609955216,
-0.0110019464219508));
#24313=CARTESIAN_POINT('Ctrl Pts',(-0.0136013257636308,-0.0348549164922762,
-0.0110878821278987));
#24314=CARTESIAN_POINT('Ctrl Pts',(-0.013693601149457,-0.0348619787007947,
-0.0111978496251147));
#24315=CARTESIAN_POINT('Ctrl Pts',(-0.0137049608330007,-0.0348628758751834,
-0.0112118801423067));
#24316=CARTESIAN_POINT('Ctrl Pts',(-0.0137228893480208,-0.0348643394227479,
-0.0112348361059553));
#24317=CARTESIAN_POINT('Ctrl Pts',(-0.0137296129122642,-0.0348648996281477,
-0.0112436388426649));
#24318=CARTESIAN_POINT('Ctrl Pts',(-0.0137413918132987,-0.0348659018439433,
-0.0112594093680791));
#24319=CARTESIAN_POINT('Ctrl Pts',(-0.0137464847513141,-0.0348663423497975,
-0.0112663485583684));
#24320=CARTESIAN_POINT('Ctrl Pts',(-0.0137571041425502,-0.0348672763137529,
-0.0112810743519968));
#24321=CARTESIAN_POINT('Ctrl Pts',(-0.0137626168971439,-0.0348677702764735,
-0.011288870348456));
#24322=CARTESIAN_POINT('Ctrl Pts',(-0.0137771251407206,-0.0348690951303613,
-0.0113097968826123));
#24323=CARTESIAN_POINT('Ctrl Pts',(-0.0137859902563478,-0.0348699309309308,
-0.0113230160484024));
#24324=CARTESIAN_POINT('Ctrl Pts',(-0.0138321383068054,-0.0348744261404011,
-0.0113941854307183));
#24325=CARTESIAN_POINT('Ctrl Pts',(-0.0138657082887652,-0.0348782212023065,
-0.0114544407312063));
#24326=CARTESIAN_POINT('Ctrl Pts',(-0.0139354997108496,-0.0348874499541373,
-0.0116021655012082));
#24327=CARTESIAN_POINT('Ctrl Pts',(-0.0139679273055855,-0.0348929562700478,
-0.0116911211347877));
#24328=CARTESIAN_POINT('Ctrl Pts',(-0.0140044249149756,-0.0349010831195163,
-0.0118295522751019));
#24329=CARTESIAN_POINT('Ctrl Pts',(-0.0140146018867452,-0.0349038007813811,
-0.0118771885495423));
#24330=CARTESIAN_POINT('Ctrl Pts',(-0.0140241282398028,-0.0349069469760492,
-0.0119350600933263));
#24331=CARTESIAN_POINT('Ctrl Pts',(-0.0140256512231199,-0.0349074768703016,
-0.0119449060873067));
#24332=CARTESIAN_POINT('Ctrl Pts',(-0.0140278833574914,-0.034908297470321,
-0.0119603237581672));
#24333=CARTESIAN_POINT('Ctrl Pts',(-0.014028657610351,-0.0349085916387056,
-0.011965885565256));
#24334=CARTESIAN_POINT('Ctrl Pts',(-0.014029978069052,-0.0349091107582605,
-0.0119757656751512));
#24335=CARTESIAN_POINT('Ctrl Pts',(-0.0140305363729834,-0.0349093363724382,
-0.0119800821051503));
#24336=CARTESIAN_POINT('Ctrl Pts',(-0.0140318364186023,-0.0349098770088289,
-0.0119904787904951));
#24337=CARTESIAN_POINT('Ctrl Pts',(-0.0140325602275405,-0.0349101910230965,
-0.0119965611545858));
#24338=CARTESIAN_POINT('Ctrl Pts',(-0.014034679258444,-0.034911152879147,
-0.0120153192144296));
#24339=CARTESIAN_POINT('Ctrl Pts',(-0.0140359536117413,-0.0349117943095468,
-0.0120280083099307));
#24340=CARTESIAN_POINT('Ctrl Pts',(-0.0140410215997774,-0.0349146720774839,
-0.0120856506686283));
#24341=CARTESIAN_POINT('Ctrl Pts',(-0.0140430000000296,-0.0349168242222948,
-0.0121307411443307));
#24342=CARTESIAN_POINT('Ctrl Pts',(-0.014043,-0.0349189332996453,-0.012175853287569));
#24343=CARTESIAN_POINT('Origin',(-0.0125,-0.0375520664398416,-0.0121758532865581));
#24344=CARTESIAN_POINT('',(-0.014043,-0.0354167228394876,-0.0121758532865582));
#24345=CARTESIAN_POINT('',(-0.014043,-0.0353007220219321,-0.0121758532865564));
#24346=CARTESIAN_POINT('',(-0.014043,-0.0375520664398416,-0.012175853286558));
#24347=CARTESIAN_POINT('Ctrl Pts',(-0.014043,-0.0353007220219321,-0.0121758532865547));
#24348=CARTESIAN_POINT('Ctrl Pts',(-0.0140429999999998,-0.0352954039244155,
-0.0120668252355584));
#24349=CARTESIAN_POINT('Ctrl Pts',(-0.0140314443207502,-0.0352905409360675,
-0.0119580939458071));
#24350=CARTESIAN_POINT('Ctrl Pts',(-0.013992016855839,-0.0352819214273844,
-0.0117747332594792));
#24351=CARTESIAN_POINT('Ctrl Pts',(-0.0139696823889352,-0.0352782525208751,
-0.0116993622952759));
#24352=CARTESIAN_POINT('Ctrl Pts',(-0.0139342467037295,-0.0352733685094644,
-0.0116064462491928));
#24353=CARTESIAN_POINT('Ctrl Pts',(-0.0139263830231519,-0.0352723273106245,
-0.011587024449181));
#24354=CARTESIAN_POINT('Ctrl Pts',(-0.0139139625982418,-0.0352707410170081,
-0.0115580584905924));
#24355=CARTESIAN_POINT('Ctrl Pts',(-0.0139096990796995,-0.035270205883243,
-0.0115483908282159));
#24356=CARTESIAN_POINT('Ctrl Pts',(-0.0139018164013339,-0.0352692327480824,
-0.0115310025523506));
#24357=CARTESIAN_POINT('Ctrl Pts',(-0.0138982318747997,-0.0352687959559578,
-0.0115232666540929));
#24358=CARTESIAN_POINT('Ctrl Pts',(-0.0138903910347189,-0.0352678524384189,
-0.0115067062526937));
#24359=CARTESIAN_POINT('Ctrl Pts',(-0.0138861144327696,-0.0352673450184413,
-0.0114978918159259));
#24360=CARTESIAN_POINT('Ctrl Pts',(-0.0138742990390152,-0.0352659620091812,
-0.011474118477497));
#24361=CARTESIAN_POINT('Ctrl Pts',(-0.0138666002714438,-0.0352650808339306,
-0.0114592409373305));
#24362=CARTESIAN_POINT('Ctrl Pts',(-0.013814677765236,-0.035259262822918,
-0.011362783696945));
#24363=CARTESIAN_POINT('Ctrl Pts',(-0.0137634199271336,-0.0352540703848136,
-0.0112852212326224));
#24364=CARTESIAN_POINT('Ctrl Pts',(-0.013653473927396,-0.0352439889131749,
-0.0111476032717579));
#24365=CARTESIAN_POINT('Ctrl Pts',(-0.0135962395857289,-0.0352391429977949,
-0.0110867897838852));
#24366=CARTESIAN_POINT('Ctrl Pts',(-0.0135163933747742,-0.0352331068429438,
-0.0110146553940041));
#24367=CARTESIAN_POINT('Ctrl Pts',(-0.0134980338822266,-0.0352317634746433,
-0.0109988382010494));
#24368=CARTESIAN_POINT('Ctrl Pts',(-0.013466604489085,-0.035229547708235,
-0.0109730253575504));
#24369=CARTESIAN_POINT('Ctrl Pts',(-0.0134537337931488,-0.0352286629071687,
-0.0109627946896621));
#24370=CARTESIAN_POINT('Ctrl Pts',(-0.0134353434495738,-0.0352274330920666,
-0.0109486502374509));
#24371=CARTESIAN_POINT('Ctrl Pts',(-0.013429958218279,-0.0352270770411098,
-0.0109445643651442));
#24372=CARTESIAN_POINT('Ctrl Pts',(-0.0134206484985942,-0.0352264687515745,
-0.0109375968334244));
#24373=CARTESIAN_POINT('Ctrl Pts',(-0.0134167369357639,-0.0352262153485278,
-0.0109346981412629));
#24374=CARTESIAN_POINT('Ctrl Pts',(-0.01340847136182,-0.0352256845293894,
-0.0109286332721922));
#24375=CARTESIAN_POINT('Ctrl Pts',(-0.0134041144373421,-0.0352254073949649,
-0.0109254713187599));
#24376=CARTESIAN_POINT('Ctrl Pts',(-0.0133922405522074,-0.0352246590822618,
-0.0109169485893466));
#24377=CARTESIAN_POINT('Ctrl Pts',(-0.0133846917712237,-0.035224190855451,
-0.0109116322941855));
#24378=CARTESIAN_POINT('Ctrl Pts',(-0.0133479044577275,-0.0352219428535436,
-0.0108862153831996));
#24379=CARTESIAN_POINT('Ctrl Pts',(-0.0133180243757956,-0.0352202192728915,
-0.0108670582879946));
#24380=CARTESIAN_POINT('Ctrl Pts',(-0.0132122357564922,-0.0352143702231927,
-0.0108042735573172));
#24381=CARTESIAN_POINT('Ctrl Pts',(-0.0131332944278842,-0.0352104329567915,
-0.0107660835988117));
#24382=CARTESIAN_POINT('Ctrl Pts',(-0.0129683167857677,-0.0352023251367187,
-0.0107029417246487));
#24383=CARTESIAN_POINT('Ctrl Pts',(-0.012882500628084,-0.0351981634880242,
-0.010678362021703));
#24384=CARTESIAN_POINT('Ctrl Pts',(-0.012778655598113,-0.0351929239911381,
-0.010658131625068));
#24385=CARTESIAN_POINT('Ctrl Pts',(-0.0127622106391915,-0.0351920888212098,
-0.0106552042352081));
#24386=CARTESIAN_POINT('Ctrl Pts',(-0.0127361543326203,-0.0351907556674694,
-0.0106510011464575));
#24387=CARTESIAN_POINT('Ctrl Pts',(-0.0127265726986002,-0.0351902633375946,
-0.01064954803379));
#24388=CARTESIAN_POINT('Ctrl Pts',(-0.0127085249136169,-0.0351893318289823,
-0.0106469846659262));
#24389=CARTESIAN_POINT('Ctrl Pts',(-0.0127000619727321,-0.0351888933111071,
-0.0106458542336471));
#24390=CARTESIAN_POINT('Ctrl Pts',(-0.0126809545641554,-0.0351878992136181,
-0.0106434632142573));
#24391=CARTESIAN_POINT('Ctrl Pts',(-0.0126703055404811,-0.0351873423692668,
-0.0106422431982268));
#24392=CARTESIAN_POINT('Ctrl Pts',(-0.0126387363420048,-0.035185682980067,
-0.010638959300821));
#24393=CARTESIAN_POINT('Ctrl Pts',(-0.0126177863232004,-0.0351845705588175,
-0.0106372119316136));
#24394=CARTESIAN_POINT('Ctrl Pts',(-0.0124852085743953,-0.0351774578972247,
-0.01062887758477));
#24395=CARTESIAN_POINT('Ctrl Pts',(-0.0123731930680936,-0.0351710867988278,
-0.010634014935825));
#24396=CARTESIAN_POINT('Ctrl Pts',(-0.0122005870972706,-0.0351610376918551,
-0.0106608757977568));
#24397=CARTESIAN_POINT('Ctrl Pts',(-0.0121390862371291,-0.0351574179871451,
-0.0106743384554941));
#24398=CARTESIAN_POINT('Ctrl Pts',(-0.0120585119157,-0.0351527471264743,
-0.0106972146149091));
#24399=CARTESIAN_POINT('Ctrl Pts',(-0.0120385638115219,-0.0351515970117509,
-0.0107033177982365));
#24400=CARTESIAN_POINT('Ctrl Pts',(-0.0120047685959642,-0.0351496663071883,
-0.010714411792339));
#24401=CARTESIAN_POINT('Ctrl Pts',(-0.0119908581818634,-0.035148876834957,
-0.0107191995786856));
#24402=CARTESIAN_POINT('Ctrl Pts',(-0.0119709322680835,-0.0351477556995824,
-0.0107263781483005));
#24403=CARTESIAN_POINT('Ctrl Pts',(-0.0119648603949052,-0.0351474153798778,
-0.0107286088540636));
#24404=CARTESIAN_POINT('Ctrl Pts',(-0.0119542818187599,-0.0351468249986837,
-0.0107325709263451));
#24405=CARTESIAN_POINT('Ctrl Pts',(-0.0119497689460431,-0.035146573956988,
-0.010734285357502));
#24406=CARTESIAN_POINT('Ctrl Pts',(-0.0119401016879257,-0.0351460380040336,
-0.0107380099412361));
#24407=CARTESIAN_POINT('Ctrl Pts',(-0.0119349500096747,-0.0351457534843036,
-0.0107400266550166));
#24408=CARTESIAN_POINT('Ctrl Pts',(-0.0119208348724951,-0.0351449766368309,
-0.0107456400048453));
#24409=CARTESIAN_POINT('Ctrl Pts',(-0.011911894021667,-0.035144487579214,
-0.0107492932130306));
#24410=CARTESIAN_POINT('Ctrl Pts',(-0.0118626904962162,-0.0351418098454449,
-0.0107699388598854));
#24411=CARTESIAN_POINT('Ctrl Pts',(-0.011823126447455,-0.0351397073037646,
-0.0107885531898061));
#24412=CARTESIAN_POINT('Ctrl Pts',(-0.0117119147232486,-0.0351338015823805,
-0.0108467689940691));
#24413=CARTESIAN_POINT('Ctrl Pts',(-0.0116425566594987,-0.0351301181076973,
-0.0108904212873636));
#24414=CARTESIAN_POINT('Ctrl Pts',(-0.0115141668459892,-0.0351227544551838,
-0.0109862621410874));
#24415=CARTESIAN_POINT('Ctrl Pts',(-0.011455017796256,-0.0351190903796698,
-0.0110378705478477));
#24416=CARTESIAN_POINT('Ctrl Pts',(-0.011385365521147,-0.0351142123956274,
-0.0111086713064869));
#24417=CARTESIAN_POINT('Ctrl Pts',(-0.0113709874800098,-0.0351131718672164,
-0.0111238941253043));
#24418=CARTESIAN_POINT('Ctrl Pts',(-0.011349828628903,-0.0351115863931175,
-0.0111472297408439));
#24419=CARTESIAN_POINT('Ctrl Pts',(-0.0113428138672507,-0.0351110513925958,
-0.011155127648273));
#24420=CARTESIAN_POINT('Ctrl Pts',(-0.0113302849055304,-0.035110078398942,
-0.0111695291404365));
#24421=CARTESIAN_POINT('Ctrl Pts',(-0.0113247424344345,-0.0351096416134206,
-0.0111760076284687));
#24422=CARTESIAN_POINT('Ctrl Pts',(-0.0113129457698155,-0.0351086979963888,
-0.0111900301400834));
#24423=CARTESIAN_POINT('Ctrl Pts',(-0.0113067092040792,-0.0351081904690234,
-0.011197588449242));
#24424=CARTESIAN_POINT('Ctrl Pts',(-0.0112900021719658,-0.0351068068798073,
-0.0112182337664188));
#24425=CARTESIAN_POINT('Ctrl Pts',(-0.0112796724576945,-0.0351059252241669,
-0.011231432538834));
#24426=CARTESIAN_POINT('Ctrl Pts',(-0.0112142025544493,-0.0351001625459669,
-0.0113179544302265));
#24427=CARTESIAN_POINT('Ctrl Pts',(-0.0111654876927915,-0.0350950321715532,
-0.01139589293744));
#24428=CARTESIAN_POINT('Ctrl Pts',(-0.0110937374019318,-0.0350859598421296,
-0.0115373048732213));
#24429=CARTESIAN_POINT('Ctrl Pts',(-0.0110673942372996,-0.0350820868188733,
-0.0115988270375849));
#24430=CARTESIAN_POINT('Ctrl Pts',(-0.0110334265828864,-0.0350762875489232,
-0.0116949743341376));
#24431=CARTESIAN_POINT('Ctrl Pts',(-0.0110228620762184,-0.0350743124266521,
-0.0117284765310563));
#24432=CARTESIAN_POINT('Ctrl Pts',(-0.011007709068249,-0.035071203459733,
-0.0117829467605495));
#24433=CARTESIAN_POINT('Ctrl Pts',(-0.011002398593164,-0.0350700423918871,
-0.0118037002549353));
#24434=CARTESIAN_POINT('Ctrl Pts',(-0.0109958182990081,-0.0350685055922548,
-0.0118318439993315));
#24435=CARTESIAN_POINT('Ctrl Pts',(-0.0109941678664211,-0.0350681104843747,
-0.0118391418830467));
#24436=CARTESIAN_POINT('Ctrl Pts',(-0.0109915026899573,-0.0350674561582841,
-0.0118513384381392));
#24437=CARTESIAN_POINT('Ctrl Pts',(-0.0109904585788777,-0.0350671953104402,
-0.0118562305071027));
#24438=CARTESIAN_POINT('Ctrl Pts',(-0.0109883911160468,-0.0350666695781939,
-0.0118661535323106));
#24439=CARTESIAN_POINT('Ctrl Pts',(-0.01098736905088,-0.0350664047657853,
-0.0118711846647692));
#24440=CARTESIAN_POINT('Ctrl Pts',(-0.0109847998184951,-0.0350657259018598,
-0.0118841634403861));
#24441=CARTESIAN_POINT('Ctrl Pts',(-0.010983290044503,-0.0350653139284998,
-0.0118921184230557));
#24442=CARTESIAN_POINT('Ctrl Pts',(-0.010977497935617,-0.0350636777271097,
-0.0119240050983901));
#24443=CARTESIAN_POINT('Ctrl Pts',(-0.0109737186508502,-0.0350624792140348,
-0.0119480256991938));
#24444=CARTESIAN_POINT('Ctrl Pts',(-0.0109578393397728,-0.0350566554285851,
-0.012067240766773));
#24445=CARTESIAN_POINT('Ctrl Pts',(-0.0109540690501827,-0.0350523409907202,
-0.0121633367238258));
#24446=CARTESIAN_POINT('Ctrl Pts',(-0.0109643183224831,-0.0350436425809516,
-0.0123528815474466));
#24447=CARTESIAN_POINT('Ctrl Pts',(-0.0109779249888903,-0.03503927645826,
-0.012445931836608));
#24448=CARTESIAN_POINT('Ctrl Pts',(-0.0110038376878683,-0.0350337974195278,
-0.0125535176383299));
#24449=CARTESIAN_POINT('Ctrl Pts',(-0.0110080441755761,-0.0350329563818056,
-0.0125698073661045));
#24450=CARTESIAN_POINT('Ctrl Pts',(-0.0110150990930963,-0.0350316159939692,
-0.0125953919798349));
#24451=CARTESIAN_POINT('Ctrl Pts',(-0.0110177705011337,-0.0350311224051761,
-0.0126047345352977));
#24452=CARTESIAN_POINT('Ctrl Pts',(-0.0110229537242415,-0.0350301898307496,
-0.0126222344479279));
#24453=CARTESIAN_POINT('Ctrl Pts',(-0.0110254453359723,-0.0350297515230363,
-0.0126303974327609));
#24454=CARTESIAN_POINT('Ctrl Pts',(-0.0110312070057516,-0.0350287596830806,
-0.0126487276895015));
#24455=CARTESIAN_POINT('Ctrl Pts',(-0.0110345151401086,-0.0350282049095644,
-0.0126588824560726));
#24456=CARTESIAN_POINT('Ctrl Pts',(-0.011044811823034,-0.0350265207837027,
-0.0126894097408411));
#24457=CARTESIAN_POINT('Ctrl Pts',(-0.0110521215511163,-0.0350253808629573,
-0.012709670480015));
#24458=CARTESIAN_POINT('Ctrl Pts',(-0.0110978815623562,-0.0350185527313626,
-0.0128286433225629));
#24459=CARTESIAN_POINT('Ctrl Pts',(-0.0111459859520115,-0.0350125365676485,
-0.0129233228953379));
#24460=CARTESIAN_POINT('Ctrl Pts',(-0.0112397372329089,-0.0350025907139899,
-0.0130686469408664));
#24461=CARTESIAN_POINT('Ctrl Pts',(-0.0112797108605154,-0.034998723634024,
-0.0131225516702715));
#24462=CARTESIAN_POINT('Ctrl Pts',(-0.0113370428704942,-0.0349937727506698,
-0.0131901742023993));
#24463=CARTESIAN_POINT('Ctrl Pts',(-0.0113513663993812,-0.0349925793479096,
-0.0132063663307641));
#24464=CARTESIAN_POINT('Ctrl Pts',(-0.0113762711407729,-0.0349905842334855,
-0.0132333553820207));
#24465=CARTESIAN_POINT('Ctrl Pts',(-0.0113866791912224,-0.0349897728961346,
-0.0132443073291911));
#24466=CARTESIAN_POINT('Ctrl Pts',(-0.0114018193870056,-0.0349886266938911,
-0.0132597772134039));
#24467=CARTESIAN_POINT('Ctrl Pts',(-0.0114064217201269,-0.0349882826494873,
-0.0132644203661504));
#24468=CARTESIAN_POINT('Ctrl Pts',(-0.0114144798494721,-0.0349876880765889,
-0.0132724472823926));
#24469=CARTESIAN_POINT('Ctrl Pts',(-0.0114179222583034,-0.0349874365242794,
-0.01327584426474));
#24470=CARTESIAN_POINT('Ctrl Pts',(-0.0114253089867612,-0.034986902011804,
-0.0132830652825972));
#24471=CARTESIAN_POINT('Ctrl Pts',(-0.0114292578018425,-0.034986619415297,
-0.0132868844854979));
#24472=CARTESIAN_POINT('Ctrl Pts',(-0.0114400816704452,-0.0349858530587617,
-0.0132972417760865));
#24473=CARTESIAN_POINT('Ctrl Pts',(-0.0114469968651873,-0.0349853724250091,
-0.0133037377737417));
#24474=CARTESIAN_POINT('Ctrl Pts',(-0.0114839047410759,-0.0349828515031324,
-0.0133377729699757));
#24475=CARTESIAN_POINT('Ctrl Pts',(-0.0115149209544446,-0.0349808857910871,
-0.0133641826541099));
#24476=CARTESIAN_POINT('Ctrl Pts',(-0.0116129575030509,-0.0349749998726223,
-0.0134411791733277));
#24477=CARTESIAN_POINT('Ctrl Pts',(-0.0116830898665416,-0.0349712227064863,
-0.01348755183374));
#24478=CARTESIAN_POINT('Ctrl Pts',(-0.0118328091226443,-0.0349633739712203,
-0.0135698614872455));
#24479=CARTESIAN_POINT('Ctrl Pts',(-0.0119123648486291,-0.0349593075518563,
-0.0136052186328943));
#24480=CARTESIAN_POINT('Ctrl Pts',(-0.0120101869478757,-0.0349541793007366,
-0.0136391403398384));
#24481=CARTESIAN_POINT('Ctrl Pts',(-0.0120259934568373,-0.0349533472806077,
-0.0136443367206617));
#24482=CARTESIAN_POINT('Ctrl Pts',(-0.0120511214400963,-0.0349520180101334,
-0.0136521495603865));
#24483=CARTESIAN_POINT('Ctrl Pts',(-0.0120603890306984,-0.0349515263564394,
-0.0136549357182527));
#24484=CARTESIAN_POINT('Ctrl Pts',(-0.012077883232411,-0.0349505954142842,
-0.0136600161366901));
#24485=CARTESIAN_POINT('Ctrl Pts',(-0.0120861039010516,-0.0349501567774791,
-0.0136623296390623));
#24486=CARTESIAN_POINT('Ctrl Pts',(-0.0121047052241171,-0.0349491614382916,
-0.0136673982516778));
#24487=CARTESIAN_POINT('Ctrl Pts',(-0.0121150962177201,-0.034948603458306,
-0.0136701134423976));
#24488=CARTESIAN_POINT('Ctrl Pts',(-0.0121460073498791,-0.0349469374493509,
-0.0136778467765611));
#24489=CARTESIAN_POINT('Ctrl Pts',(-0.012166602548647,-0.0349458194270115,
-0.0136825521018522));
#24490=CARTESIAN_POINT('Ctrl Pts',(-0.0122947255159789,-0.0349388126536597,
-0.0137090684689962));
#24491=CARTESIAN_POINT('Ctrl Pts',(-0.0124042139206035,-0.034932568645501,
-0.0137197783838096));
#24492=CARTESIAN_POINT('Ctrl Pts',(-0.0125782423052445,-0.034922557396283,
-0.0137182112837191));
#24493=CARTESIAN_POINT('Ctrl Pts',(-0.0126424939810499,-0.0349188507740264,
-0.0137136068998331));
#24494=CARTESIAN_POINT('Ctrl Pts',(-0.0127272114952592,-0.0349140812326848,
-0.0137021790571953));
#24495=CARTESIAN_POINT('Ctrl Pts',(-0.0127480912002074,-0.0349129156397414,
-0.0136989246082645));
#24496=CARTESIAN_POINT('Ctrl Pts',(-0.0127835237595683,-0.0349109618661706,
-0.0136926538278739));
#24497=CARTESIAN_POINT('Ctrl Pts',(-0.0127981116420341,-0.0349101645404439,
-0.0136898543054446));
#24498=CARTESIAN_POINT('Ctrl Pts',(-0.0128190160397944,-0.0349090343917211,
-0.0136855287254055));
#24499=CARTESIAN_POINT('Ctrl Pts',(-0.0128253664859997,-0.0349086927259179,
-0.0136841728206991));
#24500=CARTESIAN_POINT('Ctrl Pts',(-0.0128364259129553,-0.0349081008337498,
-0.0136817383882204));
#24501=CARTESIAN_POINT('Ctrl Pts',(-0.0128411386736466,-0.0349078496114162,
-0.0136806777752841));
#24502=CARTESIAN_POINT('Ctrl Pts',(-0.0128512241017425,-0.0349073141969859,
-0.0136783582209965));
#24503=CARTESIAN_POINT('Ctrl Pts',(-0.0128565950578364,-0.0349070303861969,
-0.0136770925793525));
#24504=CARTESIAN_POINT('Ctrl Pts',(-0.0128712864437572,-0.0349062574096767,
-0.0136735473275669));
#24505=CARTESIAN_POINT('Ctrl Pts',(-0.012880592725105,-0.0349057714606663,
-0.0136712095151038));
#24506=CARTESIAN_POINT('Ctrl Pts',(-0.0129310147463276,-0.034903155717133,
-0.0136580418819085));
#24507=CARTESIAN_POINT('Ctrl Pts',(-0.0129716942854991,-0.0349011073682053,
-0.013645602173136));
#24508=CARTESIAN_POINT('Ctrl Pts',(-0.0130897874220151,-0.0348952097961284,
-0.0136040801035105));
#24509=CARTESIAN_POINT('Ctrl Pts',(-0.0131654377561261,-0.0348914892833095,
-0.0135704409539774));
#24510=CARTESIAN_POINT('Ctrl Pts',(-0.0133072120882321,-0.0348840708646198,
-0.0134932231306809));
#24511=CARTESIAN_POINT('Ctrl Pts',(-0.0133734004358846,-0.0348803900787379,
-0.0134503040488251));
#24512=CARTESIAN_POINT('Ctrl Pts',(-0.0134527021743808,-0.0348754912438697,
-0.0133897923203613));
#24513=CARTESIAN_POINT('Ctrl Pts',(-0.0134691238115638,-0.0348744483983488,
-0.0133767231361152));
#24514=CARTESIAN_POINT('Ctrl Pts',(-0.0134934098695993,-0.0348728600915784,
-0.013356572394316));
#24515=CARTESIAN_POINT('Ctrl Pts',(-0.0135014766692104,-0.0348723246302969,
-0.0133497379717983));
#24516=CARTESIAN_POINT('Ctrl Pts',(-0.0135159210123895,-0.0348713511465354,
-0.0133372430562134));
#24517=CARTESIAN_POINT('Ctrl Pts',(-0.0135223231194179,-0.0348709143374003,
-0.0133316115381396));
#24518=CARTESIAN_POINT('Ctrl Pts',(-0.0135359767387985,-0.0348699710615018,
-0.0133193991245462));
#24519=CARTESIAN_POINT('Ctrl Pts',(-0.013543212911812,-0.0348694639033336,
-0.0133128017029724));
#24520=CARTESIAN_POINT('Ctrl Pts',(-0.0135626401476217,-0.0348680823095054,
-0.0132947477319779));
#24521=CARTESIAN_POINT('Ctrl Pts',(-0.0135747082449835,-0.0348672023069664,
-0.0132831612932567));
#24522=CARTESIAN_POINT('Ctrl Pts',(-0.0136545150602694,-0.0348612326709022,
-0.0132040059324208));
#24523=CARTESIAN_POINT('Ctrl Pts',(-0.0137160212583936,-0.0348558698931575,
-0.0131304685845076));
#24524=CARTESIAN_POINT('Ctrl Pts',(-0.0138110048715943,-0.0348462834566206,
-0.0129927089973075));
#24525=CARTESIAN_POINT('Ctrl Pts',(-0.0138475318622819,-0.0348421281719534,
-0.0129309328142644));
#24526=CARTESIAN_POINT('Ctrl Pts',(-0.0138928827958914,-0.0348364036879076,
-0.0128403847166573));
#24527=CARTESIAN_POINT('Ctrl Pts',(-0.0139053702691509,-0.0348347505952777,
-0.0128135515545336));
#24528=CARTESIAN_POINT('Ctrl Pts',(-0.0139245957692367,-0.034832090178242,
-0.0127689273191175));
#24529=CARTESIAN_POINT('Ctrl Pts',(-0.0139317901106737,-0.0348310637794803,
-0.0127513418240695));
#24530=CARTESIAN_POINT('Ctrl Pts',(-0.0139412429097299,-0.0348296752538405,
-0.0127269603568708));
#24531=CARTESIAN_POINT('Ctrl Pts',(-0.013943781350078,-0.0348292980797765,
-0.0127202754985326));
#24532=CARTESIAN_POINT('Ctrl Pts',(-0.0139479936249754,-0.0348286650946708,
-0.0127089459912977));
#24533=CARTESIAN_POINT('Ctrl Pts',(-0.0139496917931445,-0.0348284078696832,
-0.0127043105478727));
#24534=CARTESIAN_POINT('Ctrl Pts',(-0.0139531438102045,-0.0348278808408587,
-0.0126947457982177));
#24535=CARTESIAN_POINT('Ctrl Pts',(-0.0139548948755508,-0.0348276111967017,
-0.0126898156144382));
#24536=CARTESIAN_POINT('Ctrl Pts',(-0.0139594391953792,-0.0348269050366806,
-0.0126768115897947));
#24537=CARTESIAN_POINT('Ctrl Pts',(-0.0139621905670056,-0.0348264709284387,
-0.0126687231869728));
#24538=CARTESIAN_POINT('Ctrl Pts',(-0.0139737160628962,-0.0348246219355165,
-0.0126338947237922));
#24539=CARTESIAN_POINT('Ctrl Pts',(-0.0139818253670753,-0.0348232419263447,
-0.0126069388390049));
#24540=CARTESIAN_POINT('Ctrl Pts',(-0.0140135310494007,-0.0348174170145163,
-0.0124900451124282));
#24541=CARTESIAN_POINT('Ctrl Pts',(-0.0140297109697846,-0.0348132365962009,
-0.0123982932890866));
#24542=CARTESIAN_POINT('Ctrl Pts',(-0.0140411772148268,-0.0348069865052287,
-0.0122624549177015));
#24543=CARTESIAN_POINT('Ctrl Pts',(-0.0140430000010343,-0.0348049870032333,
-0.0122191549896209));
#24544=CARTESIAN_POINT('Ctrl Pts',(-0.014043,-0.0348029487975611,-0.0121758532497038));
#24545=CARTESIAN_POINT('',(-0.0140429998634136,-0.0354166912456805,-0.0121752040518626));
#24546=CARTESIAN_POINT('Ctrl Pts',(-0.014043,-0.0349189332996453,-0.012175853287569));
#24547=CARTESIAN_POINT('Ctrl Pts',(-0.0140429999999959,-0.0349192278748801,
-0.0121821541091974));
#24548=CARTESIAN_POINT('Ctrl Pts',(-0.0140429614060005,-0.0349195216032071,
-0.0121884553538268));
#24549=CARTESIAN_POINT('Ctrl Pts',(-0.014041484780039,-0.0349251257502518,
-0.0123089768072391));
#24550=CARTESIAN_POINT('Ctrl Pts',(-0.014027406816373,-0.0349302046700773,
-0.0124226862737504));
#24551=CARTESIAN_POINT('Ctrl Pts',(-0.0139904944307964,-0.0349377505488585,
-0.0125774624844816));
#24552=CARTESIAN_POINT('Ctrl Pts',(-0.0139781827078049,-0.0349399234980106,
-0.0126206442839973));
#24553=CARTESIAN_POINT('Ctrl Pts',(-0.0139594304292141,-0.0349428784164322,
-0.0126769738016862));
#24554=CARTESIAN_POINT('Ctrl Pts',(-0.0139546604213203,-0.0349436056922872,
-0.0126906561506721));
#24555=CARTESIAN_POINT('Ctrl Pts',(-0.0139465337035157,-0.0349448073080629,
-0.0127129516471389));
#24556=CARTESIAN_POINT('Ctrl Pts',(-0.0139432909845762,-0.0349452778305313,
-0.0127216055502295));
#24557=CARTESIAN_POINT('Ctrl Pts',(-0.0139368426242571,-0.0349461967441564,
-0.0127383549112451));
#24558=CARTESIAN_POINT('Ctrl Pts',(-0.0139336458089462,-0.0349466448238317,
-0.0127464534048471));
#24559=CARTESIAN_POINT('Ctrl Pts',(-0.0139259663413774,-0.034947704170217,
-0.0127654358001774));
#24560=CARTESIAN_POINT('Ctrl Pts',(-0.0139214273891821,-0.034948317332994,
-0.0127762962180796));
#24561=CARTESIAN_POINT('Ctrl Pts',(-0.0139058782018645,-0.0349503762370247,
-0.0128123363557482));
#24562=CARTESIAN_POINT('Ctrl Pts',(-0.0138943200499805,-0.0349518405603365,
-0.0128372727324749));
#24563=CARTESIAN_POINT('Ctrl Pts',(-0.0138361285420905,-0.0349589184051529,
-0.0129545071121626));
#24564=CARTESIAN_POINT('Ctrl Pts',(-0.0137809659904748,-0.0349648241834418,
-0.0130422608974412));
#24565=CARTESIAN_POINT('Ctrl Pts',(-0.0136661962118816,-0.0349755709059691,
-0.0131896560518137));
#24566=CARTESIAN_POINT('Ctrl Pts',(-0.0136096804700388,-0.0349803719604161,
-0.0132512234284747));
#24567=CARTESIAN_POINT('Ctrl Pts',(-0.0135379507941278,-0.0349856741910349,
-0.0133176555160852));
#24568=CARTESIAN_POINT('Ctrl Pts',(-0.0135273060148863,-0.0349864424581803,
-0.013327242257742));
#24569=CARTESIAN_POINT('Ctrl Pts',(-0.0135117531071228,-0.0349875364436436,
-0.0133408618483028));
#24570=CARTESIAN_POINT('Ctrl Pts',(-0.0135069514517016,-0.0349878703568017,
-0.0133450145566205));
#24571=CARTESIAN_POINT('Ctrl Pts',(-0.0134984409179205,-0.0349884552476121,
-0.0133522835638559));
#24572=CARTESIAN_POINT('Ctrl Pts',(-0.0134947427932698,-0.0349887071138764,
-0.0133554122046813));
#24573=CARTESIAN_POINT('Ctrl Pts',(-0.0134867521285533,-0.0349892463678287,
-0.0133621080588484));
#24574=CARTESIAN_POINT('Ctrl Pts',(-0.0134824549228922,-0.0349895333432447,
-0.0133656694380615));
#24575=CARTESIAN_POINT('Ctrl Pts',(-0.0134703436270403,-0.034990334012746,
-0.0133755965191546));
#24576=CARTESIAN_POINT('Ctrl Pts',(-0.0134624862230763,-0.0349908440360555,
-0.0133819091970804));
#24577=CARTESIAN_POINT('Ctrl Pts',(-0.0134091896442855,-0.0349942448185815,
-0.0134238753260312));
#24578=CARTESIAN_POINT('Ctrl Pts',(-0.0133618371648448,-0.0349969829915576,
-0.0134570335008771));
#24579=CARTESIAN_POINT('Ctrl Pts',(-0.0132315907913201,-0.0350040962160063,
-0.0135377402091237));
#24580=CARTESIAN_POINT('Ctrl Pts',(-0.0131459584125612,-0.0350083691588784,
-0.0135803814538955));
#24581=CARTESIAN_POINT('Ctrl Pts',(-0.0130018016638577,-0.0350155952728165,
-0.0136361747908962));
#24582=CARTESIAN_POINT('Ctrl Pts',(-0.0129454938790591,-0.0350184221681892,
-0.0136543248269263));
#24583=CARTESIAN_POINT('Ctrl Pts',(-0.0128730171721841,-0.0350221383638682,
-0.0136731695911866));
#24584=CARTESIAN_POINT('Ctrl Pts',(-0.0128576878572948,-0.0350229284737961,
-0.01367690535106));
#24585=CARTESIAN_POINT('Ctrl Pts',(-0.0128330231942587,-0.0350242073967137,
-0.0136825168686683));
#24586=CARTESIAN_POINT('Ctrl Pts',(-0.0128237228934832,-0.0350246913664161,
-0.0136845424793624));
#24587=CARTESIAN_POINT('Ctrl Pts',(-0.0128059709390309,-0.0350256186493354,
-0.0136882371636811));
#24588=CARTESIAN_POINT('Ctrl Pts',(-0.0127975228641939,-0.0350260614431616,
-0.0136899217620818));
#24589=CARTESIAN_POINT('Ctrl Pts',(-0.0127781253379242,-0.0350270817398846,
-0.0136936211344696));
#24590=CARTESIAN_POINT('Ctrl Pts',(-0.0127671673870795,-0.035027660743206,
-0.0136955883036771));
#24591=CARTESIAN_POINT('Ctrl Pts',(-0.0127327164854055,-0.035029489647266,
-0.0137013888087877));
#24592=CARTESIAN_POINT('Ctrl Pts',(-0.0127091563228732,-0.0350307529073,
-0.0137047970852208));
#24593=CARTESIAN_POINT('Ctrl Pts',(-0.0126535838033979,-0.0350337629107386,
-0.0137115278581568));
#24594=CARTESIAN_POINT('Ctrl Pts',(-0.0126215284635323,-0.0350355227270624,
-0.0137143964324962));
#24595=CARTESIAN_POINT('Ctrl Pts',(-0.0124947106963579,-0.0350425710299601,
-0.0137217571884371));
#24596=CARTESIAN_POINT('Ctrl Pts',(-0.0123997140466747,-0.0350480559704158,
-0.0137185090355401));
#24597=CARTESIAN_POINT('Ctrl Pts',(-0.0122351309786807,-0.0350575769048951,
-0.0136976099306512));
#24598=CARTESIAN_POINT('Ctrl Pts',(-0.0121653303295028,-0.0350616147864906,
-0.0136837978905335));
#24599=CARTESIAN_POINT('Ctrl Pts',(-0.0120866529293196,-0.0350659933987778,
-0.01366249449768));
#24600=CARTESIAN_POINT('Ctrl Pts',(-0.0120766081790851,-0.0350665490356654,
-0.0136596650229496));
#24601=CARTESIAN_POINT('Ctrl Pts',(-0.0120611021319024,-0.0350674006743878,
-0.0136551268884433));
#24602=CARTESIAN_POINT('Ctrl Pts',(-0.0120556205113603,-0.0350677005544777,
-0.0136534894393385));
#24603=CARTESIAN_POINT('Ctrl Pts',(-0.012045533926267,-0.0350682499957669,
-0.0136504152064394));
#24604=CARTESIAN_POINT('Ctrl Pts',(-0.0120409265519993,-0.0350685000410071,
-0.0136489873055105));
#24605=CARTESIAN_POINT('Ctrl Pts',(-0.0120303661320681,-0.0350690710863216,
-0.0136456601013735));
#24606=CARTESIAN_POINT('Ctrl Pts',(-0.0120244178638815,-0.0350693912335158,
-0.0136437462244846));
#24607=CARTESIAN_POINT('Ctrl Pts',(-0.0120057471240004,-0.035070391873913,
-0.0136376134410386));
#24608=CARTESIAN_POINT('Ctrl Pts',(-0.0119930675950396,-0.0350710651850754,
-0.0136332647639384));
#24609=CARTESIAN_POINT('Ctrl Pts',(-0.0119266660968784,-0.0350745660782618,
-0.0136095196918036));
#24610=CARTESIAN_POINT('Ctrl Pts',(-0.0118739907908064,-0.0350772568707838,
-0.0135873151821283));
#24611=CARTESIAN_POINT('Ctrl Pts',(-0.0116959210881877,-0.0350864258207977,
-0.0135003170642539));
#24612=CARTESIAN_POINT('Ctrl Pts',(-0.0115782757134133,-0.0350926835113507,
-0.0134213137138952));
#24613=CARTESIAN_POINT('Ctrl Pts',(-0.01145758237785,-0.035100626472104,
-0.0133136762919159));
#24614=CARTESIAN_POINT('Ctrl Pts',(-0.0114424441622214,-0.0351016528845517,
-0.0132996198503045));
#24615=CARTESIAN_POINT('Ctrl Pts',(-0.0114199215459087,-0.0351032290829109,
-0.0132778484672597));
#24616=CARTESIAN_POINT('Ctrl Pts',(-0.01141232723575,-0.0351037693533707,
-0.0132703535358799));
#24617=CARTESIAN_POINT('Ctrl Pts',(-0.0113987764453279,-0.0351047497196259,
-0.013256699750894));
#24618=CARTESIAN_POINT('Ctrl Pts',(-0.0113927923334941,-0.0351051885599997,
-0.0132505688657363));
#24619=CARTESIAN_POINT('Ctrl Pts',(-0.0113800740682142,-0.035106134168763,
-0.0132373196875376));
#24620=CARTESIAN_POINT('Ctrl Pts',(-0.0113733560675464,-0.0351066416109347,
-0.0132301864675762));
#24621=CARTESIAN_POINT('Ctrl Pts',(-0.0113551126602553,-0.0351080419031602,
-0.0132104420193764));
#24622=CARTESIAN_POINT('Ctrl Pts',(-0.0113437282836082,-0.035108940681098,
-0.0131977028610675));
#24623=CARTESIAN_POINT('Ctrl Pts',(-0.0112615186880988,-0.0351156199649834,
-0.013102576870036));
#24624=CARTESIAN_POINT('Ctrl Pts',(-0.0111993705232442,-0.0351217599111498,
-0.0130131158575664));
#24625=CARTESIAN_POINT('Ctrl Pts',(-0.0111013513515596,-0.0351334747941228,
-0.0128344092911922));
#24626=CARTESIAN_POINT('Ctrl Pts',(-0.011063386164316,-0.0351389916492257,
-0.0127468673381362));
#24627=CARTESIAN_POINT('Ctrl Pts',(-0.0110294001501643,-0.035144904557628,
-0.0126431631692948));
#24628=CARTESIAN_POINT('Ctrl Pts',(-0.0110252474810955,-0.0351456499822229,
-0.0126298879540799));
#24629=CARTESIAN_POINT('Ctrl Pts',(-0.0110194827658824,-0.0351467176415384,
-0.0126105452276401));
#24630=CARTESIAN_POINT('Ctrl Pts',(-0.0110177274486277,-0.0351470475529177,
-0.0126045215152663));
#24631=CARTESIAN_POINT('Ctrl Pts',(-0.0110146844059113,-0.0351476279859805,
-0.0125938365025539));
#24632=CARTESIAN_POINT('Ctrl Pts',(-0.0110133817824504,-0.0351478793500546,
-0.0125891796227748));
#24633=CARTESIAN_POINT('Ctrl Pts',(-0.0110106101979945,-0.035148420513058,
-0.0125790885809712));
#24634=CARTESIAN_POINT('Ctrl Pts',(-0.0110091490643315,-0.0351487098659902,
-0.0125736524501426));
#24635=CARTESIAN_POINT('Ctrl Pts',(-0.0110050978289862,-0.0351495241837776,
-0.0125582439917753));
#24636=CARTESIAN_POINT('Ctrl Pts',(-0.0110025777692413,-0.0351500452738054,
-0.0125482533752353));
#24637=CARTESIAN_POINT('Ctrl Pts',(-0.0109848017237453,-0.0351538369924973,
-0.0124746816727093));
#24638=CARTESIAN_POINT('Ctrl Pts',(-0.0109734993320685,-0.0351569117924867,
-0.0124102068762238));
#24639=CARTESIAN_POINT('Ctrl Pts',(-0.0109550633142776,-0.0351646666328646,
-0.0122432461221478));
#24640=CARTESIAN_POINT('Ctrl Pts',(-0.0109540000424025,-0.0351692610412371,
-0.0121404227228415));
#24641=CARTESIAN_POINT('Ctrl Pts',(-0.0109672701340439,-0.0351763072216525,
-0.0119922088521544));
#24642=CARTESIAN_POINT('Ctrl Pts',(-0.0109734595736708,-0.0351785425438435,
-0.0119463756987252));
#24643=CARTESIAN_POINT('Ctrl Pts',(-0.0109843050854499,-0.0351815706909719,
-0.0118864881278773));
#24644=CARTESIAN_POINT('Ctrl Pts',(-0.0109871183260745,-0.0351823052110926,
-0.011872122664027));
#24645=CARTESIAN_POINT('Ctrl Pts',(-0.0109920469091079,-0.0351835157210243,
-0.0118487256859834));
#24646=CARTESIAN_POINT('Ctrl Pts',(-0.0109940400868623,-0.0351839877799489,
-0.0118396692201924));
#24647=CARTESIAN_POINT('Ctrl Pts',(-0.0109980596333535,-0.0351849074789414,
-0.0118221589264326));
#24648=CARTESIAN_POINT('Ctrl Pts',(-0.011000076052585,-0.035185354782227,
-0.0118137031613598));
#24649=CARTESIAN_POINT('Ctrl Pts',(-0.0110049701676435,-0.0351864088082339,
-0.0117939222265011));
#24650=CARTESIAN_POINT('Ctrl Pts',(-0.0110079052477468,-0.0351870173730948,
-0.011782611917395));
#24651=CARTESIAN_POINT('Ctrl Pts',(-0.011018037372148,-0.0351890441199869,
-0.0117453154597867));
#24652=CARTESIAN_POINT('Ctrl Pts',(-0.0110257868167337,-0.0351904800997411,
-0.0117194856524783));
#24653=CARTESIAN_POINT('Ctrl Pts',(-0.0110460925637809,-0.035193992795591,
-0.0116577320933375));
#24654=CARTESIAN_POINT('Ctrl Pts',(-0.011059308314014,-0.035196089284498,
-0.0116220450534919));
#24655=CARTESIAN_POINT('Ctrl Pts',(-0.0111198453258141,-0.0352049649548892,
-0.0114754563411682));
#24656=CARTESIAN_POINT('Ctrl Pts',(-0.0111787567257122,-0.0352120470701014,
-0.0113698164392069));
#24657=CARTESIAN_POINT('Ctrl Pts',(-0.0112710303650416,-0.0352208989449371,
-0.0112421232346664));
#24658=CARTESIAN_POINT('Ctrl Pts',(-0.0112937761695284,-0.0352229423963625,
-0.0112129188984447));
#24659=CARTESIAN_POINT('Ctrl Pts',(-0.0113235723120526,-0.0352254249107107,
-0.0111773770868772));
#24660=CARTESIAN_POINT('Ctrl Pts',(-0.0113296584923796,-0.0352259224642264,
-0.011170250188713));
#24661=CARTESIAN_POINT('Ctrl Pts',(-0.0113393717949308,-0.0352267010280163,
-0.0111590835815567));
#24662=CARTESIAN_POINT('Ctrl Pts',(-0.0113429558569228,-0.0352269850458421,
-0.0111550069140975));
#24663=CARTESIAN_POINT('Ctrl Pts',(-0.0113498048887272,-0.0352275214898538,
-0.0111472989367761));
#24664=CARTESIAN_POINT('Ctrl Pts',(-0.0113530656527687,-0.0352277741982832,
-0.0111436641334304));
#24665=CARTESIAN_POINT('Ctrl Pts',(-0.0113608726695489,-0.0352283730004217,
-0.0111350442537846));
#24666=CARTESIAN_POINT('Ctrl Pts',(-0.0113654345124865,-0.0352287179314594,
-0.0111300733501051));
#24667=CARTESIAN_POINT('Ctrl Pts',(-0.011381097972403,-0.0352298861196759,
-0.0111132284791137));
#24668=CARTESIAN_POINT('Ctrl Pts',(-0.0113923548849554,-0.0352306983474067,
-0.0111014997286535));
#24669=CARTESIAN_POINT('Ctrl Pts',(-0.0114205685227779,-0.0352326743002262,
-0.0110730184298032));
#24670=CARTESIAN_POINT('Ctrl Pts',(-0.0114377323623434,-0.0352338251371262,
-0.0110564764084946));
#24671=CARTESIAN_POINT('Ctrl Pts',(-0.0115145281002074,-0.0352387906107325,
-0.010985820762947));
#24672=CARTESIAN_POINT('Ctrl Pts',(-0.0115779624968361,-0.0352424291992976,
-0.0109360224433093));
#24673=CARTESIAN_POINT('Ctrl Pts',(-0.0117251191616811,-0.0352505241307344,
-0.0108380667512559));
#24674=CARTESIAN_POINT('Ctrl Pts',(-0.0118100502824741,-0.0352549921551669,
-0.0107923504942044));
#24675=CARTESIAN_POINT('Ctrl Pts',(-0.0119141253550243,-0.0352605857024441,
-0.0107483095134318));
#24676=CARTESIAN_POINT('Ctrl Pts',(-0.0119296771278133,-0.0352614239192091,
-0.0107420255013818));
#24677=CARTESIAN_POINT('Ctrl Pts',(-0.0119544985938413,-0.0352627668352553,
-0.0107324635960763));
#24678=CARTESIAN_POINT('Ctrl Pts',(-0.0119637027052372,-0.0352632658933655,
-0.0107290185383925));
#24679=CARTESIAN_POINT('Ctrl Pts',(-0.0119809879928628,-0.0352642053984294,
-0.0107227363328822));
#24680=CARTESIAN_POINT('Ctrl Pts',(-0.0119890611271197,-0.03526464511637,
-0.0107198780776865));
#24681=CARTESIAN_POINT('Ctrl Pts',(-0.0120072063384381,-0.0352656356422503,
-0.0107136233511478));
#24682=CARTESIAN_POINT('Ctrl Pts',(-0.0120172904929665,-0.0352661876429202,
-0.0107102634731803));
#24683=CARTESIAN_POINT('Ctrl Pts',(-0.0120475281325399,-0.0352678476598518,
-0.0107005347046513));
#24684=CARTESIAN_POINT('Ctrl Pts',(-0.0120677780318011,-0.0352689657604726,
-0.010694475610447));
#24685=CARTESIAN_POINT('Ctrl Pts',(-0.0121649566631374,-0.0352743635739593,
-0.010667560366849));
#24686=CARTESIAN_POINT('Ctrl Pts',(-0.0122432914515529,-0.0352788187375334,
-0.0106522721270687));
#24687=CARTESIAN_POINT('Ctrl Pts',(-0.0124065346341412,-0.0352882018671932,
-0.0106333622253194));
#24688=CARTESIAN_POINT('Ctrl Pts',(-0.0124912793349515,-0.0352931262060502,
-0.0106305577064839));
#24689=CARTESIAN_POINT('Ctrl Pts',(-0.0126154323267523,-0.0353001288900669,
-0.0106366662222009));
#24690=CARTESIAN_POINT('Ctrl Pts',(-0.0126549517083395,-0.0353023243949546,
-0.0106401411136288));
#24691=CARTESIAN_POINT('Ctrl Pts',(-0.0127037679935924,-0.0353049597878984,
-0.0106463374253121));
#24692=CARTESIAN_POINT('Ctrl Pts',(-0.0127132289046396,-0.0353054669332946,
-0.0106476276460621));
#24693=CARTESIAN_POINT('Ctrl Pts',(-0.0127280867004815,-0.0353062570289947,
-0.0106497945264506));
#24694=CARTESIAN_POINT('Ctrl Pts',(-0.012733491793894,-0.0353065431320929,
-0.0106506121691469));
#24695=CARTESIAN_POINT('Ctrl Pts',(-0.0127437050289793,-0.0353070810823052,
-0.0106522127160859));
#24696=CARTESIAN_POINT('Ctrl Pts',(-0.0127485139094776,-0.0353073332398516,
-0.0106529896793348));
#24697=CARTESIAN_POINT('Ctrl Pts',(-0.0127598957869477,-0.0353079274855676,
-0.010654883980213));
#24698=CARTESIAN_POINT('Ctrl Pts',(-0.0127664654294669,-0.035308268461373,
-0.0106560211810382));
#24699=CARTESIAN_POINT('Ctrl Pts',(-0.0127885528853254,-0.035309408632534,
-0.0106599921262914));
#24700=CARTESIAN_POINT('Ctrl Pts',(-0.0128040350168475,-0.0353101975013507,
-0.0106630213164853));
#24701=CARTESIAN_POINT('Ctrl Pts',(-0.0128418563300488,-0.0353121051373797,
-0.0106710254189021));
#24702=CARTESIAN_POINT('Ctrl Pts',(-0.0128641368900721,-0.0353132121502159,
-0.0106762609847965));
#24703=CARTESIAN_POINT('Ctrl Pts',(-0.0129583190584852,-0.0353178505673233,
-0.0107006152743959));
#24704=CARTESIAN_POINT('Ctrl Pts',(-0.0130289072199716,-0.035321228262489,
-0.0107244257399117));
#24705=CARTESIAN_POINT('Ctrl Pts',(-0.013185720711164,-0.0353290055307256,
-0.0107902881063701));
#24706=CARTESIAN_POINT('Ctrl Pts',(-0.0132702936924813,-0.0353334137029007,
-0.0108354618222048));
#24707=CARTESIAN_POINT('Ctrl Pts',(-0.0133684374919634,-0.035339179324623,
-0.010900256788681));
#24708=CARTESIAN_POINT('Ctrl Pts',(-0.0133864817561702,-0.0353402679167725,
-0.0109127301181926));
#24709=CARTESIAN_POINT('Ctrl Pts',(-0.0134129913189206,-0.0353419134508962,
-0.0109319030709441));
#24710=CARTESIAN_POINT('Ctrl Pts',(-0.0134216625192168,-0.0353424592987653,
-0.0109383140021867));
#24711=CARTESIAN_POINT('Ctrl Pts',(-0.0134371083636149,-0.0353434456833796,
-0.0109499860526849));
#24712=CARTESIAN_POINT('Ctrl Pts',(-0.0134439077311533,-0.0353438848950614,
-0.0109552138019583));
#24713=CARTESIAN_POINT('Ctrl Pts',(-0.013458320403366,-0.0353448267868719,
-0.0109664875374962));
#24714=CARTESIAN_POINT('Ctrl Pts',(-0.0134659208347509,-0.0353453300899173,
-0.0109725493159497));
#24715=CARTESIAN_POINT('Ctrl Pts',(-0.0134864388355817,-0.0353467071232581,
-0.0109892332519152));
#24716=CARTESIAN_POINT('Ctrl Pts',(-0.0134992415538547,-0.0353475864587699,
-0.0109999940389266));
#24717=CARTESIAN_POINT('Ctrl Pts',(-0.0135785132529602,-0.0353531606049416,
-0.0110688522031373));
#24718=CARTESIAN_POINT('Ctrl Pts',(-0.0136400596206086,-0.0353580851422487,
-0.011132348395693));
#24719=CARTESIAN_POINT('Ctrl Pts',(-0.0137504600378492,-0.0353680644443494,
-0.0112677396009183));
#24720=CARTESIAN_POINT('Ctrl Pts',(-0.0137993595571494,-0.0353730947626295,
-0.0113392018376263));
#24721=CARTESIAN_POINT('Ctrl Pts',(-0.0138603335630965,-0.0353800376867678,
-0.0114466626058166));
#24722=CARTESIAN_POINT('Ctrl Pts',(-0.0138774801042879,-0.0353820875318691,
-0.0114795951385183));
#24723=CARTESIAN_POINT('Ctrl Pts',(-0.0138974519739828,-0.0353845765205087,
-0.011521586553736));
#24724=CARTESIAN_POINT('Ctrl Pts',(-0.0139014034144621,-0.0353850745115089,
-0.0115300936905956));
#24725=CARTESIAN_POINT('Ctrl Pts',(-0.0139075194814681,-0.0353858536018432,
-0.0115435816741634));
#24726=CARTESIAN_POINT('Ctrl Pts',(-0.0139097357492781,-0.035386137715287,
-0.0115485386912028));
#24727=CARTESIAN_POINT('Ctrl Pts',(-0.0139138951485842,-0.0353866742301261,
-0.0115579751850743));
#24728=CARTESIAN_POINT('Ctrl Pts',(-0.0139158432281681,-0.0353869269150386,
-0.0115624522815244));
#24729=CARTESIAN_POINT('Ctrl Pts',(-0.0139204310632585,-0.0353875255113124,
-0.0115731343940845));
#24730=CARTESIAN_POINT('Ctrl Pts',(-0.0139230514831374,-0.035387870262338,
-0.0115793476718229));
#24731=CARTESIAN_POINT('Ctrl Pts',(-0.0139318409212051,-0.0353890371443356,
-0.0116005758981555));
#24732=CARTESIAN_POINT('Ctrl Pts',(-0.0139378138853745,-0.0353898482794882,
-0.0116156713807252));
#24733=CARTESIAN_POINT('Ctrl Pts',(-0.0139519499788152,-0.0353918210174683,
-0.0116531141961429));
#24734=CARTESIAN_POINT('Ctrl Pts',(-0.013959836780341,-0.0353929697871273,
-0.0116755618057165));
#24735=CARTESIAN_POINT('Ctrl Pts',(-0.0140173505844951,-0.0354018108256075,
-0.0118522202099648));
#24736=CARTESIAN_POINT('Ctrl Pts',(-0.0140429316914556,-0.0354088077580484,
-0.0120131835640155));
#24737=CARTESIAN_POINT('Ctrl Pts',(-0.0140429998634136,-0.0354166912456806,
-0.0121752040518639));
#24738=CARTESIAN_POINT('Ctrl Pts',(-0.0140429998634136,-0.0354166912456805,
-0.0121752040518624));
#24739=CARTESIAN_POINT('Ctrl Pts',(-0.0140429999558722,-0.035416701937705,
-0.0121754237930612));
#24740=CARTESIAN_POINT('Ctrl Pts',(-0.014043,-0.0354167121449367,-0.012175633545861));
#24741=CARTESIAN_POINT('Ctrl Pts',(-0.014043,-0.0354167228394876,-0.0121758532865585));
#24742=CARTESIAN_POINT('Origin',(-0.0125,-0.0375520664398416,-0.0121758532865581));
#24743=CARTESIAN_POINT('',(-0.014043,-0.0359172995678105,-0.0121758532865606));
#24744=CARTESIAN_POINT('',(-0.014043,-0.035802018678757,-0.0121758532865075));
#24745=CARTESIAN_POINT('',(-0.014043,-0.0375520664398416,-0.012175853286558));
#24746=CARTESIAN_POINT('',(-0.0140429999599998,-0.0353007391609988,-0.0121762046275615));
#24747=CARTESIAN_POINT('Ctrl Pts',(-0.014043,-0.035802018678757,-0.012175853286457));
#24748=CARTESIAN_POINT('Ctrl Pts',(-0.0140429999999942,-0.0357969039511853,
-0.0120869245163723));
#24749=CARTESIAN_POINT('Ctrl Pts',(-0.0140353120831769,-0.0357917698082273,
-0.0119981559031497));
#24750=CARTESIAN_POINT('Ctrl Pts',(-0.0140175842681859,-0.0357861805132807,
-0.0118965909125327));
#24751=CARTESIAN_POINT('Ctrl Pts',(-0.0140149576625064,-0.0357854213234747,
-0.0118826762184364));
#24752=CARTESIAN_POINT('Ctrl Pts',(-0.0140108854541471,-0.0357843386179533,
-0.0118626219404954));
#24753=CARTESIAN_POINT('Ctrl Pts',(-0.0140095932455082,-0.0357840071050992,
-0.0118564523354713));
#24754=CARTESIAN_POINT('Ctrl Pts',(-0.0140072460029681,-0.0357834257958607,
-0.0118455780520453));
#24755=CARTESIAN_POINT('Ctrl Pts',(-0.0140062066735373,-0.0357831751292779,
-0.0118408701486142));
#24756=CARTESIAN_POINT('Ctrl Pts',(-0.0140039198885508,-0.0357826378450967,
-0.0118307374355294));
#24757=CARTESIAN_POINT('Ctrl Pts',(-0.0140026651343067,-0.0357823516428319,
-0.0118253144472818));
#24758=CARTESIAN_POINT('Ctrl Pts',(-0.0139990564962871,-0.0357815518511041,
-0.0118100935887655));
#24759=CARTESIAN_POINT('Ctrl Pts',(-0.0139966359028222,-0.035781041938553,
-0.0118003116508037));
#24760=CARTESIAN_POINT('Ctrl Pts',(-0.0139794992746883,-0.0357776015109178,
-0.0117338589862703));
#24761=CARTESIAN_POINT('Ctrl Pts',(-0.0139616623912841,-0.0357748279314554,
-0.0116780366703213));
#24762=CARTESIAN_POINT('Ctrl Pts',(-0.0139062743513583,-0.0357676511346147,
-0.0115336058452449));
#24763=CARTESIAN_POINT('Ctrl Pts',(-0.0138635433588903,-0.0357633483770738,
-0.0114472660511692));
#24764=CARTESIAN_POINT('Ctrl Pts',(-0.0137826698329396,-0.0357561417055771,
-0.0113162287481834));
#24765=CARTESIAN_POINT('Ctrl Pts',(-0.0137495414647113,-0.0357533721258981,
-0.0112687471686669));
#24766=CARTESIAN_POINT('Ctrl Pts',(-0.0137041572123496,-0.0357497232978149,
-0.0112109181841473));
#24767=CARTESIAN_POINT('Ctrl Pts',(-0.0136943001222839,-0.0357489387544438,
-0.0111987445213389));
#24768=CARTESIAN_POINT('Ctrl Pts',(-0.0136781904338011,-0.0357476680119432,
-0.0111794568098598));
#24769=CARTESIAN_POINT('Ctrl Pts',(-0.0136720545768633,-0.0357471865762327,
-0.0111722464408795));
#24770=CARTESIAN_POINT('Ctrl Pts',(-0.0136602328312253,-0.0357462636257307,
-0.0111586107477681));
#24771=CARTESIAN_POINT('Ctrl Pts',(-0.0136545589341768,-0.0357458226191196,
-0.0111521754715607));
#24772=CARTESIAN_POINT('Ctrl Pts',(-0.013641420283427,-0.0357448057215296,
-0.0111375219362815));
#24773=CARTESIAN_POINT('Ctrl Pts',(-0.0136339199665133,-0.0357442283325195,
-0.0111293363219425));
#24774=CARTESIAN_POINT('Ctrl Pts',(-0.0136100729922263,-0.0357424018719868,
-0.0111038678190353));
#24775=CARTESIAN_POINT('Ctrl Pts',(-0.0135934151578517,-0.0357411394408294,
-0.0110868821675252));
#24776=CARTESIAN_POINT('Ctrl Pts',(-0.0135533121968993,-0.0357381300090292,
-0.0110478381235019));
#24777=CARTESIAN_POINT('Ctrl Pts',(-0.0135295568871957,-0.0357363699005796,
-0.0110261153977616));
#24778=CARTESIAN_POINT('Ctrl Pts',(-0.0134330285084361,-0.0357293110005793,
-0.0109432380339284));
#24779=CARTESIAN_POINT('Ctrl Pts',(-0.0133553543197461,-0.0357238147747226,
-0.0108881232248371));
#24780=CARTESIAN_POINT('Ctrl Pts',(-0.0132117020613102,-0.0357142892220465,
-0.010804954074116));
#24781=CARTESIAN_POINT('Ctrl Pts',(-0.0131479053382555,-0.035710257547409,
-0.0107736746321215));
#24782=CARTESIAN_POINT('Ctrl Pts',(-0.0130725396235192,-0.0357058862499264,
-0.0107429695942542));
#24783=CARTESIAN_POINT('Ctrl Pts',(-0.0130628624889502,-0.0357053321656911,
-0.0107391406756869));
#24784=CARTESIAN_POINT('Ctrl Pts',(-0.0130478259484627,-0.0357044831574408,
-0.01073336646848));
#24785=CARTESIAN_POINT('Ctrl Pts',(-0.0130424934253114,-0.0357041843724694,
-0.0107313525507736));
#24786=CARTESIAN_POINT('Ctrl Pts',(-0.0130326481964725,-0.0357036371428417,
-0.0107276965417633));
#24787=CARTESIAN_POINT('Ctrl Pts',(-0.0130281389472009,-0.0357033882152627,
-0.010726045950438));
#24788=CARTESIAN_POINT('Ctrl Pts',(-0.0130177780869906,-0.0357028201148599,
-0.0107223081558072));
#24789=CARTESIAN_POINT('Ctrl Pts',(-0.0130119215159286,-0.0357025017821357,
-0.0107202352189984));
#24790=CARTESIAN_POINT('Ctrl Pts',(-0.0129934923365365,-0.035701508350312,
-0.0107138371836837));
#24791=CARTESIAN_POINT('Ctrl Pts',(-0.012980875950078,-0.035700840313235,
-0.0107096390749429));
#24792=CARTESIAN_POINT('Ctrl Pts',(-0.0129145144581758,-0.0356973817815611,
-0.010688505998918));
#24793=CARTESIAN_POINT('Ctrl Pts',(-0.0128599213965291,-0.0356947246143362,
-0.0106743600863118));
#24794=CARTESIAN_POINT('Ctrl Pts',(-0.0127079168213646,-0.0356875463643613,
-0.0106437432627425));
#24795=CARTESIAN_POINT('Ctrl Pts',(-0.0126095157178928,-0.0356831282475872,
-0.0106335831483342));
#24796=CARTESIAN_POINT('Ctrl Pts',(-0.0124577272187848,-0.0356759918334553,
-0.0106325190068169));
#24797=CARTESIAN_POINT('Ctrl Pts',(-0.0124046574529035,-0.035673439853699,
-0.0106348870995712));
#24798=CARTESIAN_POINT('Ctrl Pts',(-0.0123366432010291,-0.0356700450042746,
-0.0106414491754506));
#24799=CARTESIAN_POINT('Ctrl Pts',(-0.0123214912351247,-0.0356692808543534,
-0.0106431380423654));
#24800=CARTESIAN_POINT('Ctrl Pts',(-0.0122970638029911,-0.0356680352380575,
-0.0106462278957082));
#24801=CARTESIAN_POINT('Ctrl Pts',(-0.012287771554196,-0.0356675581945331,
-0.0106474894496113));
#24802=CARTESIAN_POINT('Ctrl Pts',(-0.0122699770666586,-0.0356666382926994,
-0.0106500707098385));
#24803=CARTESIAN_POINT('Ctrl Pts',(-0.0122614732176514,-0.0356661958777746,
-0.0106513769858636));
#24804=CARTESIAN_POINT('Ctrl Pts',(-0.0122418396092341,-0.0356651677907679,
-0.0106545612025663));
#24805=CARTESIAN_POINT('Ctrl Pts',(-0.0122307187373199,-0.0356645805074265,
-0.010656490267197));
#24806=CARTESIAN_POINT('Ctrl Pts',(-0.0121952144602948,-0.0356626893136001,
-0.0106630510010518));
#24807=CARTESIAN_POINT('Ctrl Pts',(-0.0121709220996311,-0.0356613706630401,
-0.0106681488662015));
#24808=CARTESIAN_POINT('Ctrl Pts',(-0.0120493794043543,-0.035654646179712,
-0.0106967324722927));
#24809=CARTESIAN_POINT('Ctrl Pts',(-0.0119544652589708,-0.0356489609153181,
-0.0107290484677886));
#24810=CARTESIAN_POINT('Ctrl Pts',(-0.0117803691321364,-0.0356379703138455,
-0.0108079056507223));
#24811=CARTESIAN_POINT('Ctrl Pts',(-0.0117008662078673,-0.0356327038727902,
-0.0108527747752512));
#24812=CARTESIAN_POINT('Ctrl Pts',(-0.0116153408069296,-0.0356270786123029,
-0.0109115796960468));
#24813=CARTESIAN_POINT('Ctrl Pts',(-0.0116049867755636,-0.0356263985281629,
-0.0109188883119078));
#24814=CARTESIAN_POINT('Ctrl Pts',(-0.0115896934242431,-0.0356253968597755,
-0.0109299682506319));
#24815=CARTESIAN_POINT('Ctrl Pts',(-0.0115846851647509,-0.03562506929708,
-0.0109336430227286));
#24816=CARTESIAN_POINT('Ctrl Pts',(-0.0115760916967042,-0.0356245082482817,
-0.0109400286038204));
#24817=CARTESIAN_POINT('Ctrl Pts',(-0.0115724959260372,-0.0356242737941744,
-0.0109427249910546));
#24818=CARTESIAN_POINT('Ctrl Pts',(-0.011564903393968,-0.0356237794848083,
-0.0109484704582584));
#24819=CARTESIAN_POINT('Ctrl Pts',(-0.0115609096511328,-0.0356235199187744,
-0.0109515234341272));
#24820=CARTESIAN_POINT('Ctrl Pts',(-0.0115509148455304,-0.0356228712518423,
-0.0109592415391782));
#24821=CARTESIAN_POINT('Ctrl Pts',(-0.0115449331246344,-0.0356224838824401,
-0.0109639316544165));
#24822=CARTESIAN_POINT('Ctrl Pts',(-0.0115214987256851,-0.03562096858775,
-0.0109825872341537));
#24823=CARTESIAN_POINT('Ctrl Pts',(-0.011504314973799,-0.0356198625128401,
-0.0109968876210711));
#24824=CARTESIAN_POINT('Ctrl Pts',(-0.0114592437712256,-0.0356169568934583,
-0.0110360846639483));
#24825=CARTESIAN_POINT('Ctrl Pts',(-0.0114319393593185,-0.0356151917118042,
-0.0110616303313854));
#24826=CARTESIAN_POINT('Ctrl Pts',(-0.0113262129776787,-0.0356082136566246,
-0.0111680081443195));
#24827=CARTESIAN_POINT('Ctrl Pts',(-0.0112558188348658,-0.0356032060506992,
-0.0112563197107745));
#24828=CARTESIAN_POINT('Ctrl Pts',(-0.0111705938449963,-0.035595657845881,
-0.0113911688753597));
#24829=CARTESIAN_POINT('Ctrl Pts',(-0.0111473514117971,-0.0355933904449234,
-0.0114319503066239));
#24830=CARTESIAN_POINT('Ctrl Pts',(-0.0111193267175715,-0.0355903265330415,
-0.0114867918859883));
#24831=CARTESIAN_POINT('Ctrl Pts',(-0.0111128363343671,-0.035589590268226,
-0.0114999529444264));
#24832=CARTESIAN_POINT('Ctrl Pts',(-0.0111025602892601,-0.0355883789456883,
-0.0115215621395346));
#24833=CARTESIAN_POINT('Ctrl Pts',(-0.011098661128386,-0.0355879078610364,
-0.011529955452356));
#24834=CARTESIAN_POINT('Ctrl Pts',(-0.011091265594989,-0.0355869915607104,
-0.0115462572753471));
#24835=CARTESIAN_POINT('Ctrl Pts',(-0.0110877597246949,-0.0355865466957615,
-0.0115541611103725));
#24836=CARTESIAN_POINT('Ctrl Pts',(-0.0110797155400832,-0.0355855007956478,
-0.0115727155914201));
#24837=CARTESIAN_POINT('Ctrl Pts',(-0.0110752303385841,-0.0355848979699681,
-0.0115833885800852));
#24838=CARTESIAN_POINT('Ctrl Pts',(-0.0110608758472488,-0.0355829018932249,
-0.0116186524590689));
#24839=CARTESIAN_POINT('Ctrl Pts',(-0.0110515202176966,-0.035581491517141,
-0.0116434462127955));
#24840=CARTESIAN_POINT('Ctrl Pts',(-0.0110305784778562,-0.0355780527125094,
-0.011703590075391));
#24841=CARTESIAN_POINT('Ctrl Pts',(-0.0110196235604196,-0.035576005540787,
-0.0117391411899085));
#24842=CARTESIAN_POINT('Ctrl Pts',(-0.0109926936782248,-0.0355702105554153,
-0.011839256749101));
#24843=CARTESIAN_POINT('Ctrl Pts',(-0.0109795921172323,-0.0355663966691419,
-0.0119045075947239));
#24844=CARTESIAN_POINT('Ctrl Pts',(-0.0109594743588605,-0.0355577051302924,
-0.0120542479737002));
#24845=CARTESIAN_POINT('Ctrl Pts',(-0.0109551236424415,-0.0355528331275439,
-0.0121388908996066));
#24846=CARTESIAN_POINT('Ctrl Pts',(-0.0109581753140536,-0.035547470599006,
-0.0122377352119439));
#24847=CARTESIAN_POINT('Ctrl Pts',(-0.0109588137371642,-0.0355467051249706,
-0.0122519956968508));
#24848=CARTESIAN_POINT('Ctrl Pts',(-0.0109600204030318,-0.035545615202657,
-0.0122725581161415));
#24849=CARTESIAN_POINT('Ctrl Pts',(-0.0109604296369369,-0.0355452826126924,
-0.0122788682518567));
#24850=CARTESIAN_POINT('Ctrl Pts',(-0.010961219392323,-0.0355447001101853,
-0.0122899870060016));
#24851=CARTESIAN_POINT('Ctrl Pts',(-0.0109615836874813,-0.0355444493149205,
-0.0122947966175866));
#24852=CARTESIAN_POINT('Ctrl Pts',(-0.0109624159173361,-0.0355439125552217,
-0.0123051398915939));
#24853=CARTESIAN_POINT('Ctrl Pts',(-0.0109628911751381,-0.0355436269971503,
-0.0123106727952155));
#24854=CARTESIAN_POINT('Ctrl Pts',(-0.0109643073634688,-0.0355428308784808,
-0.012326177769754));
#24855=CARTESIAN_POINT('Ctrl Pts',(-0.0109653155522594,-0.0355423239408678,
-0.0123361435858477));
#24856=CARTESIAN_POINT('Ctrl Pts',(-0.0109726862327671,-0.0355389742721936,
-0.0124025388817137));
#24857=CARTESIAN_POINT('Ctrl Pts',(-0.0109820632692576,-0.0355362791101029,
-0.0124585951352789));
#24858=CARTESIAN_POINT('Ctrl Pts',(-0.0110203320101982,-0.0355281658738612,
-0.0126289687648708));
#24859=CARTESIAN_POINT('Ctrl Pts',(-0.0110592340137502,-0.0355229309491022,
-0.0127405879390835));
#24860=CARTESIAN_POINT('Ctrl Pts',(-0.0111284041509055,-0.0355153537855548,
-0.0128838626344016));
#24861=CARTESIAN_POINT('Ctrl Pts',(-0.0111478308226674,-0.0355133490449166,
-0.0129202930553938));
#24862=CARTESIAN_POINT('Ctrl Pts',(-0.0111758023790196,-0.0355105923519372,
-0.0129680321832902));
#24863=CARTESIAN_POINT('Ctrl Pts',(-0.0111830767039385,-0.0355098859813953,
-0.01298006703893));
#24864=CARTESIAN_POINT('Ctrl Pts',(-0.0111953405075296,-0.0355087113334865,
-0.0129997439717324));
#24865=CARTESIAN_POINT('Ctrl Pts',(-0.0112002351783702,-0.0355082465677578,
-0.0130074443255663));
#24866=CARTESIAN_POINT('Ctrl Pts',(-0.0112099335575592,-0.0355073332891935,
-0.0130224071154273));
#24867=CARTESIAN_POINT('Ctrl Pts',(-0.0112147310176271,-0.0355068850215266,
-0.0130296732030951));
#24868=CARTESIAN_POINT('Ctrl Pts',(-0.0112262558779372,-0.0355058161847234,
-0.0130468111597219));
#24869=CARTESIAN_POINT('Ctrl Pts',(-0.0112330368650322,-0.0355051935931092,
-0.0130566461731665));
#24870=CARTESIAN_POINT('Ctrl Pts',(-0.0112565252736293,-0.0355030576417126,
-0.0130898807772476));
#24871=CARTESIAN_POINT('Ctrl Pts',(-0.0112737714947859,-0.0355015236816646,
-0.0131128907204594));
#24872=CARTESIAN_POINT('Ctrl Pts',(-0.0113175172855969,-0.0354977125856331,
-0.0131679792242129));
#24873=CARTESIAN_POINT('Ctrl Pts',(-0.0113446898662361,-0.0354954108714996,
-0.013199492551242));
#24874=CARTESIAN_POINT('Ctrl Pts',(-0.0114188087639352,-0.0354893111225179,
-0.0132787367259381));
#24875=CARTESIAN_POINT('Ctrl Pts',(-0.0114676452390555,-0.0354854589165813,
-0.0133245783195241));
#24876=CARTESIAN_POINT('Ctrl Pts',(-0.0115329903724915,-0.035480591339684,
-0.0133783739068904));
#24877=CARTESIAN_POINT('Ctrl Pts',(-0.0115468742989383,-0.035479572469939,
-0.013389407928267));
#24878=CARTESIAN_POINT('Ctrl Pts',(-0.0116123473635524,-0.0354748470711335,
-0.0134396247242715));
#24879=CARTESIAN_POINT('Ctrl Pts',(-0.0116661860400421,-0.0354711834050243,
-0.0134757768415772));
#24880=CARTESIAN_POINT('Ctrl Pts',(-0.011731094231683,-0.0354671468820992,
-0.0135136650672111));
#24881=CARTESIAN_POINT('Ctrl Pts',(-0.0117400987833732,-0.0354665950421411,
-0.0135188002674091));
#24882=CARTESIAN_POINT('Ctrl Pts',(-0.0117541263285647,-0.0354657487326962,
-0.0135266137586506));
#24883=CARTESIAN_POINT('Ctrl Pts',(-0.0117591133854929,-0.0354654504392737,
-0.0135293555633174));
#24884=CARTESIAN_POINT('Ctrl Pts',(-0.011768337141258,-0.0354649036533949,
-0.0135343603824996));
#24885=CARTESIAN_POINT('Ctrl Pts',(-0.0117725692703024,-0.0354646546842331,
-0.0135366312268464));
#24886=CARTESIAN_POINT('Ctrl Pts',(-0.0117823110393535,-0.0354640859098827,
-0.0135417999569554));
#24887=CARTESIAN_POINT('Ctrl Pts',(-0.0117878276699755,-0.0354637669526756,
-0.0135446842934925));
#24888=CARTESIAN_POINT('Ctrl Pts',(-0.0118052405366685,-0.0354627695423985,
-0.0135536547394338));
#24889=CARTESIAN_POINT('Ctrl Pts',(-0.0118171987489832,-0.0354620982320017,
-0.0135596198961374));
#24890=CARTESIAN_POINT('Ctrl Pts',(-0.0118805234644829,-0.0354586069941102,
-0.0135901875755987));
#24891=CARTESIAN_POINT('Ctrl Pts',(-0.0119331495835205,-0.0354559231943394,
-0.0136120894594758));
#24892=CARTESIAN_POINT('Ctrl Pts',(-0.0120805363248874,-0.0354486917767345,
-0.0136640614326879));
#24893=CARTESIAN_POINT('Ctrl Pts',(-0.012177170877928,-0.0354442456487917,
-0.0136879693251362));
#24894=CARTESIAN_POINT('Ctrl Pts',(-0.0123266286244941,-0.0354371353458193,
-0.0137099553001116));
#24895=CARTESIAN_POINT('Ctrl Pts',(-0.0123781659979896,-0.0354346458527557,
-0.0137149057378052));
#24896=CARTESIAN_POINT('Ctrl Pts',(-0.0124450920885785,-0.0354313173935996,
-0.013717951488272));
#24897=CARTESIAN_POINT('Ctrl Pts',(-0.0124603412969363,-0.0354305527272303,
-0.0137184189767821));
#24898=CARTESIAN_POINT('Ctrl Pts',(-0.0124849732334615,-0.0354293064703981,
-0.0137188086252244));
#24899=CARTESIAN_POINT('Ctrl Pts',(-0.0124943528870484,-0.0354288293111643,
-0.0137188714607378));
#24900=CARTESIAN_POINT('Ctrl Pts',(-0.0125123353986931,-0.0354279093235751,
-0.0137188279623061));
#24901=CARTESIAN_POINT('Ctrl Pts',(-0.0125209379551196,-0.0354274669402418,
-0.0137187352036501));
#24902=CARTESIAN_POINT('Ctrl Pts',(-0.0125408192668135,-0.0354264391310958,
-0.0137183545263135));
#24903=CARTESIAN_POINT('Ctrl Pts',(-0.0125520964428259,-0.0354258520969612,
-0.0137180148340955));
#24904=CARTESIAN_POINT('Ctrl Pts',(-0.0125881398599833,-0.0354239625815609,
-0.0137165333354301));
#24905=CARTESIAN_POINT('Ctrl Pts',(-0.0126128818459542,-0.03542264539729,
-0.0137149183405773));
#24906=CARTESIAN_POINT('Ctrl Pts',(-0.012729021647587,-0.0354163657331576,
-0.0137045219568074));
#24907=CARTESIAN_POINT('Ctrl Pts',(-0.0128195454793205,-0.0354111728501523,
-0.0136881910773662));
#24908=CARTESIAN_POINT('Ctrl Pts',(-0.0130047128766322,-0.0354001462547104,
-0.0136374127751207));
#24909=CARTESIAN_POINT('Ctrl Pts',(-0.0130985494428649,-0.0353943240570536,
-0.0136015573800375));
#24910=CARTESIAN_POINT('Ctrl Pts',(-0.0132003161283345,-0.0353881695729477,
-0.0135508398608999));
#24911=CARTESIAN_POINT('Ctrl Pts',(-0.0132123035581187,-0.0353874475750909,
-0.0135446682574568));
#24912=CARTESIAN_POINT('Ctrl Pts',(-0.0132296667885471,-0.0353864078475456,
-0.0135354390991178));
#24913=CARTESIAN_POINT('Ctrl Pts',(-0.0132351072423483,-0.0353860829464431,
-0.013532505249609));
#24914=CARTESIAN_POINT('Ctrl Pts',(-0.0132447481074795,-0.0353855089708859,
-0.0135272312400917));
#24915=CARTESIAN_POINT('Ctrl Pts',(-0.0132489554029518,-0.0353852591022197,
-0.0135249040354987));
#24916=CARTESIAN_POINT('Ctrl Pts',(-0.0132580813174181,-0.0353847184987099,
-0.0135198003149205));
#24917=CARTESIAN_POINT('Ctrl Pts',(-0.0132629956168666,-0.0353844282362377,
-0.0135170164345293));
#24918=CARTESIAN_POINT('Ctrl Pts',(-0.0132769685716638,-0.0353836050470774,
-0.0135089992955165));
#24919=CARTESIAN_POINT('Ctrl Pts',(-0.0132859896018094,-0.0353830761505662,
-0.0135037007174639));
#24920=CARTESIAN_POINT('Ctrl Pts',(-0.0133590446671285,-0.0353788082271515,
-0.0134597858181012));
#24921=CARTESIAN_POINT('Ctrl Pts',(-0.0134202549907116,-0.0353753257478028,
-0.0134166488323846));
#24922=CARTESIAN_POINT('Ctrl Pts',(-0.0135767124135399,-0.035366033529131,
-0.0132884160783385));
#24923=CARTESIAN_POINT('Ctrl Pts',(-0.0136649187121481,-0.0353603083418362,
-0.0131956907410332));
#24924=CARTESIAN_POINT('Ctrl Pts',(-0.0137532075334448,-0.0353530188981106,
-0.013076276204333));
#24925=CARTESIAN_POINT('Ctrl Pts',(-0.0137653530709777,-0.0353519752543415,
-0.0130591268032346));
#24926=CARTESIAN_POINT('Ctrl Pts',(-0.0137831582557623,-0.0353503791444993,
-0.0130328648051373));
#24927=CARTESIAN_POINT('Ctrl Pts',(-0.0137890795647408,-0.0353498366123341,
-0.0130239321275609));
#24928=CARTESIAN_POINT('Ctrl Pts',(-0.0137995501911555,-0.0353488555306339,
-0.0130077734733189));
#24929=CARTESIAN_POINT('Ctrl Pts',(-0.0138041335205856,-0.035348418282341,
-0.0130005699973533));
#24930=CARTESIAN_POINT('Ctrl Pts',(-0.0138137916906811,-0.0353474798734455,
-0.0129851087056279));
#24931=CARTESIAN_POINT('Ctrl Pts',(-0.0138188489630555,-0.0353469780868683,
-0.0129768403942403));
#24932=CARTESIAN_POINT('Ctrl Pts',(-0.013832411201842,-0.035345603410027,
-0.012954190326563));
#24933=CARTESIAN_POINT('Ctrl Pts',(-0.0138407608375782,-0.035344724912894,
-0.0129397174795719));
#24934=CARTESIAN_POINT('Ctrl Pts',(-0.0138922347644605,-0.0353390977301337,
-0.0128470501612627));
#24935=CARTESIAN_POINT('Ctrl Pts',(-0.0139287317140502,-0.0353341135310749,
-0.0127653824252391));
#24936=CARTESIAN_POINT('Ctrl Pts',(-0.0139873036985356,-0.035323889821245,
-0.0125963407799078));
#24937=CARTESIAN_POINT('Ctrl Pts',(-0.0140092129194892,-0.0353186705221667,
-0.0125092579559972));
#24938=CARTESIAN_POINT('Ctrl Pts',(-0.0140287593860278,-0.0353117780849695,
-0.0123876721089134));
#24939=CARTESIAN_POINT('Ctrl Pts',(-0.0140330001986164,-0.0353099337113886,
-0.0123544118673696));
#24940=CARTESIAN_POINT('Ctrl Pts',(-0.0140370069540922,-0.0353076566286295,
-0.0123120175797208));
#24941=CARTESIAN_POINT('Ctrl Pts',(-0.0140377800268162,-0.0353071759668753,
-0.0123029897823005));
#24942=CARTESIAN_POINT('Ctrl Pts',(-0.0140388827043345,-0.0353064184909591,
-0.0122886256116348));
#24943=CARTESIAN_POINT('Ctrl Pts',(-0.0140392641630286,-0.0353061389109068,
-0.0122832935635803));
#24944=CARTESIAN_POINT('Ctrl Pts',(-0.0140399228468762,-0.0353056212513196,
-0.0122733615447578));
#24945=CARTESIAN_POINT('Ctrl Pts',(-0.0140402071831392,-0.0353053827895653,
-0.0122687622094284));
#24946=CARTESIAN_POINT('Ctrl Pts',(-0.0140407476026397,-0.0353048964943224,
-0.0122593350075553));
#24947=CARTESIAN_POINT('Ctrl Pts',(-0.0140410016089317,-0.0353046487738411,
-0.0122545070548441));
#24948=CARTESIAN_POINT('Ctrl Pts',(-0.0140417001238575,-0.0353039043255891,
-0.0122399241972072));
#24949=CARTESIAN_POINT('Ctrl Pts',(-0.0140420747354765,-0.035303411297403,
-0.012230166018556));
#24950=CARTESIAN_POINT('Ctrl Pts',(-0.0140427821474273,-0.0353021853411504,
-0.0122056756323501));
#24951=CARTESIAN_POINT('Ctrl Pts',(-0.014042996604584,-0.0353014580834576,
-0.012190940756967));
#24952=CARTESIAN_POINT('Ctrl Pts',(-0.0140429999599998,-0.0353007391609988,
-0.0121762046275615));
#24953=CARTESIAN_POINT('Ctrl Pts',(-0.0140429999576932,-0.0353007396482844,
-0.0121762146156828));
#24954=CARTESIAN_POINT('Ctrl Pts',(-0.0140429999866775,-0.0353007336098254,
-0.0121760908428857));
#24955=CARTESIAN_POINT('Ctrl Pts',(-0.014043,-0.0353007280592019,-0.0121759770585901));
#24956=CARTESIAN_POINT('Ctrl Pts',(-0.014043,-0.0353007220219321,-0.0121758532865547));
#24957=CARTESIAN_POINT('Ctrl Pts',(-0.014043,-0.0354167228394876,-0.0121758532865585));
#24958=CARTESIAN_POINT('Ctrl Pts',(-0.014043,-0.035417538263066,-0.0121926077765226));
#24959=CARTESIAN_POINT('Ctrl Pts',(-0.0140427271104671,-0.0354183611678139,
-0.0122093607612358));
#24960=CARTESIAN_POINT('Ctrl Pts',(-0.0140417685719733,-0.0354198211756583,
-0.012238777109034));
#24961=CARTESIAN_POINT('Ctrl Pts',(-0.0140411995180436,-0.0354204547183743,
-0.0122514427736288));
#24962=CARTESIAN_POINT('Ctrl Pts',(-0.0140399887678596,-0.035421520736642,
-0.0122725782331701));
#24963=CARTESIAN_POINT('Ctrl Pts',(-0.0140394330952479,-0.0354219505219931,
-0.0122810524402915));
#24964=CARTESIAN_POINT('Ctrl Pts',(-0.0140382045355412,-0.0354227988691123,
-0.0122976843243592));
#24965=CARTESIAN_POINT('Ctrl Pts',(-0.0140375366342218,-0.0354232172607349,
-0.0123058420935309));
#24966=CARTESIAN_POINT('Ctrl Pts',(-0.0140359793582494,-0.0354241107987572,
-0.0123231666507131));
#24967=CARTESIAN_POINT('Ctrl Pts',(-0.0140350727566955,-0.0354245864744903,
-0.0123323315372455));
#24968=CARTESIAN_POINT('Ctrl Pts',(-0.0140325448714191,-0.0354258094854592,
-0.0123557444887567));
#24969=CARTESIAN_POINT('Ctrl Pts',(-0.014030806934916,-0.0354265604788053,
-0.0123699788561657));
#24970=CARTESIAN_POINT('Ctrl Pts',(-0.0140229833542211,-0.0354296204633904,
-0.0124273928316668));
#24971=CARTESIAN_POINT('Ctrl Pts',(-0.014015267400232,-0.0354319802695828,
-0.0124703267818655));
#24972=CARTESIAN_POINT('Ctrl Pts',(-0.0139822027321551,-0.0354403440093628,
-0.0126180535266602));
#24973=CARTESIAN_POINT('Ctrl Pts',(-0.0139477065189253,-0.0354466011298809,
-0.0127204701704748));
#24974=CARTESIAN_POINT('Ctrl Pts',(-0.0138763762887735,-0.0354564035862904,
-0.0128761901813467));
#24975=CARTESIAN_POINT('Ctrl Pts',(-0.0138463810887516,-0.0354599911032783,
-0.0129322545595041));
#24976=CARTESIAN_POINT('Ctrl Pts',(-0.0138076263626106,-0.0354639511183184,
-0.012995040352923));
#24977=CARTESIAN_POINT('Ctrl Pts',(-0.0138021532101693,-0.0354644967010965,
-0.0130037126841737));
#24978=CARTESIAN_POINT('Ctrl Pts',(-0.0137935479553903,-0.0354653328691484,
-0.0130170513939889));
#24979=CARTESIAN_POINT('Ctrl Pts',(-0.0137904762307793,-0.0354656272164334,
-0.0130217561584067));
#24980=CARTESIAN_POINT('Ctrl Pts',(-0.0137847122174207,-0.0354661717675542,
-0.0130304800577772));
#24981=CARTESIAN_POINT('Ctrl Pts',(-0.0137820267200105,-0.0354664223849583,
-0.0130345033254885));
#24982=CARTESIAN_POINT('Ctrl Pts',(-0.0137758058959943,-0.0354669959460088,
-0.0130437287809533));
#24983=CARTESIAN_POINT('Ctrl Pts',(-0.0137722576408999,-0.0354673180164202,
-0.0130489220443681));
#24984=CARTESIAN_POINT('Ctrl Pts',(-0.0137607121587926,-0.0354683502437189,
-0.0130656002768523));
#24985=CARTESIAN_POINT('Ctrl Pts',(-0.0137525902033759,-0.0354690524408411,
-0.0130769984815103));
#24986=CARTESIAN_POINT('Ctrl Pts',(-0.0136885109390342,-0.0354744236599395,
-0.0131643855469434));
#24987=CARTESIAN_POINT('Ctrl Pts',(-0.0136258378970183,-0.0354787124484996,
-0.013235214955224));
#24988=CARTESIAN_POINT('Ctrl Pts',(-0.0134868969734785,-0.0354874302268959,
-0.013365880687416));
#24989=CARTESIAN_POINT('Ctrl Pts',(-0.0134106907122304,-0.0354918474751161,
-0.0134251616558607));
#24990=CARTESIAN_POINT('Ctrl Pts',(-0.0133082669836429,-0.035497770110377,
-0.0134904578721875));
#24991=CARTESIAN_POINT('Ctrl Pts',(-0.0132867470097625,-0.0354990126198941,
-0.0135034487772144));
#24992=CARTESIAN_POINT('Ctrl Pts',(-0.0132550445462775,-0.0355008450225241,
-0.013521544943571));
#24993=CARTESIAN_POINT('Ctrl Pts',(-0.013245107186957,-0.0355014196621042,
-0.0135270725780204));
#24994=CARTESIAN_POINT('Ctrl Pts',(-0.0132275083114406,-0.0355024381831614,
-0.0135366087404738));
#24995=CARTESIAN_POINT('Ctrl Pts',(-0.0132198724372623,-0.0355028803783177,
-0.0135406636831382));
#24996=CARTESIAN_POINT('Ctrl Pts',(-0.0132038619605968,-0.0355038082845106,
-0.0135489941199081));
#24997=CARTESIAN_POINT('Ctrl Pts',(-0.0131954815653213,-0.0355042943957357,
-0.0135532576552256));
#24998=CARTESIAN_POINT('Ctrl Pts',(-0.013173416306837,-0.0355055756006282,
-0.0135642306707867));
#24999=CARTESIAN_POINT('Ctrl Pts',(-0.0131596703157171,-0.0355063750508658,
-0.0135708143381179));
#25000=CARTESIAN_POINT('Ctrl Pts',(-0.0130993785241876,-0.0355098880897902,
-0.0135986007525472));
#25001=CARTESIAN_POINT('Ctrl Pts',(-0.0130518961096092,-0.0355126730668131,
-0.0136176836676285));
#25002=CARTESIAN_POINT('Ctrl Pts',(-0.0129106772181637,-0.0355209940506767,
-0.0136664398268578));
#25003=CARTESIAN_POINT('Ctrl Pts',(-0.0128149509892039,-0.035526696481029,
-0.0136895597022195));
#25004=CARTESIAN_POINT('Ctrl Pts',(-0.0126598867444597,-0.0355356611436972,
-0.0137116573244957));
#25005=CARTESIAN_POINT('Ctrl Pts',(-0.0126016597900705,-0.0355389627120218,
-0.0137166077098071));
#25006=CARTESIAN_POINT('Ctrl Pts',(-0.0125297516509561,-0.0355428570120161,
-0.0137186258642752));
#25007=CARTESIAN_POINT('Ctrl Pts',(-0.0125162100491415,-0.0355435823238261,
-0.0137188275721978));
#25008=CARTESIAN_POINT('Ctrl Pts',(-0.0124963930115429,-0.0355446302373783,
-0.0137188618263989));
#25009=CARTESIAN_POINT('Ctrl Pts',(-0.0124901188003424,-0.035544960030483,
-0.0137188344040641));
#25010=CARTESIAN_POINT('Ctrl Pts',(-0.012479019540911,-0.0355455397215488,
-0.013718718188697));
#25011=CARTESIAN_POINT('Ctrl Pts',(-0.0124741945214161,-0.0355457904663236,
-0.0137186450304713));
#25012=CARTESIAN_POINT('Ctrl Pts',(-0.0124636688862054,-0.0355463346864205,
-0.0137184360436819));
#25013=CARTESIAN_POINT('Ctrl Pts',(-0.0124579686271335,-0.0355466276652384,
-0.0137182912522884));
#25014=CARTESIAN_POINT('Ctrl Pts',(-0.0124419238167432,-0.0355474477251486,
-0.0137177946883889));
#25015=CARTESIAN_POINT('Ctrl Pts',(-0.0124315816373423,-0.035547970932797,
-0.0137173704186023));
#25016=CARTESIAN_POINT('Ctrl Pts',(-0.0123588578895035,-0.0355516168853343,
-0.013713653705422));
#25017=CARTESIAN_POINT('Ctrl Pts',(-0.0122967164334764,-0.0355545619364441,
-0.0137066793692749));
#25018=CARTESIAN_POINT('Ctrl Pts',(-0.0122155560241945,-0.0355583716479132,
-0.0136925394000703));
#25019=CARTESIAN_POINT('Ctrl Pts',(-0.0121960157883835,-0.0355592859007906,
-0.0136887441476266));
#25020=CARTESIAN_POINT('Ctrl Pts',(-0.0121113871561957,-0.0355632507623223,
-0.0136706010892576));
#25021=CARTESIAN_POINT('Ctrl Pts',(-0.0120471940633684,-0.0355662751546393,
-0.0136524227997781));
#25022=CARTESIAN_POINT('Ctrl Pts',(-0.0119449645359015,-0.0355713323502744,
-0.0136161773507942));
#25023=CARTESIAN_POINT('Ctrl Pts',(-0.0119061364059356,-0.0355733118418777,
-0.0136006071292289));
#25024=CARTESIAN_POINT('Ctrl Pts',(-0.0118416398519728,-0.0355767388122657,
-0.0135716488398111));
#25025=CARTESIAN_POINT('Ctrl Pts',(-0.0118156281260667,-0.035578160656025,
-0.0135590807864966));
#25026=CARTESIAN_POINT('Ctrl Pts',(-0.0117793336648419,-0.0355802087655277,
-0.0135402700007129));
#25027=CARTESIAN_POINT('Ctrl Pts',(-0.0117687468842372,-0.0355808140967,
-0.0135346254553647));
#25028=CARTESIAN_POINT('Ctrl Pts',(-0.0117505594061091,-0.0355818682492176,
-0.0135246543330535));
#25029=CARTESIAN_POINT('Ctrl Pts',(-0.0117429276040978,-0.0355823149901962,
-0.0135203854914519));
#25030=CARTESIAN_POINT('Ctrl Pts',(-0.0117273726661433,-0.0355832347480198,
-0.0135115104244732));
#25031=CARTESIAN_POINT('Ctrl Pts',(-0.0117194534695483,-0.0355837079773526,
-0.0135068980251071));
#25032=CARTESIAN_POINT('Ctrl Pts',(-0.0116994321632487,-0.0355849172845839,
-0.0134949968413004));
#25033=CARTESIAN_POINT('Ctrl Pts',(-0.0116873883797606,-0.0355856568624891,
-0.0134876119975843));
#25034=CARTESIAN_POINT('Ctrl Pts',(-0.0116403393984216,-0.0355885948941978,
-0.0134578665250885));
#25035=CARTESIAN_POINT('Ctrl Pts',(-0.0116061439513489,-0.0355908390715005,
-0.0134342630841133));
#25036=CARTESIAN_POINT('Ctrl Pts',(-0.0114790364240769,-0.0355996040285156,
-0.0133387301642425));
#25037=CARTESIAN_POINT('Ctrl Pts',(-0.0113935022152167,-0.0356064499641351,
-0.013257660257279));
#25038=CARTESIAN_POINT('Ctrl Pts',(-0.0112932882785753,-0.0356153425541661,
-0.0131382328369357));
#25039=CARTESIAN_POINT('Ctrl Pts',(-0.0112696796450308,-0.0356175132074002,
-0.0131078617142498));
#25040=CARTESIAN_POINT('Ctrl Pts',(-0.0112339166844679,-0.0356208896384625,
-0.0130581242507803));
#25041=CARTESIAN_POINT('Ctrl Pts',(-0.0112210154245895,-0.0356221280695043,
-0.0130393158384932));
#25042=CARTESIAN_POINT('Ctrl Pts',(-0.01120433420036,-0.0356237500805105,
-0.0130138020142348));
#25043=CARTESIAN_POINT('Ctrl Pts',(-0.0112001811113789,-0.035624155722908,
-0.0130073451964266));
#25044=CARTESIAN_POINT('Ctrl Pts',(-0.011193372102047,-0.0356248234552689,
-0.0129965835199921));
#25045=CARTESIAN_POINT('Ctrl Pts',(-0.0111906888870229,-0.0356250872966508,
-0.0129922961755423));
#25046=CARTESIAN_POINT('Ctrl Pts',(-0.0111856539079778,-0.0356255836202184,
-0.0129841624318032));
#25047=CARTESIAN_POINT('Ctrl Pts',(-0.0111832978414756,-0.0356258163942267,
-0.0129803187927589));
#25048=CARTESIAN_POINT('Ctrl Pts',(-0.0111771081509562,-0.0356264294688649,
-0.012970121015926));
#25049=CARTESIAN_POINT('Ctrl Pts',(-0.0111733034174747,-0.0356268079148198,
-0.0129637493789283));
#25050=CARTESIAN_POINT('Ctrl Pts',(-0.0111598008641189,-0.0356281576818971,
-0.0129407620350326));
#25051=CARTESIAN_POINT('Ctrl Pts',(-0.0111503676755422,-0.0356291133641934,
-0.0129239921566899));
#25052=CARTESIAN_POINT('Ctrl Pts',(-0.0110937802677852,-0.0356349547750304,
-0.0128188382703318));
#25053=CARTESIAN_POINT('Ctrl Pts',(-0.011055008709352,-0.0356394595560296,
-0.0127262055578693));
#25054=CARTESIAN_POINT('Ctrl Pts',(-0.0109972071381422,-0.0356484442081871,
-0.0125387272801521));
#25055=CARTESIAN_POINT('Ctrl Pts',(-0.010977548926401,-0.0356529017668573,
-0.0124445615224224));
#25056=CARTESIAN_POINT('Ctrl Pts',(-0.0109648666206234,-0.0356584903818084,
-0.0123323800309566));
#25057=CARTESIAN_POINT('Ctrl Pts',(-0.010963243024204,-0.0356593358806267,
-0.0123155425240403));
#25058=CARTESIAN_POINT('Ctrl Pts',(-0.0109611194310561,-0.0356606831066016,
-0.0122889501884429));
#25059=CARTESIAN_POINT('Ctrl Pts',(-0.0109604346580237,-0.0356611790062028,
-0.0122792112409949));
#25060=CARTESIAN_POINT('Ctrl Pts',(-0.0109593223034823,-0.0356621158097155,
-0.0122609104097332));
#25061=CARTESIAN_POINT('Ctrl Pts',(-0.0109588735602583,-0.0356625560275748,
-0.0122523501591947));
#25062=CARTESIAN_POINT('Ctrl Pts',(-0.0109580240645614,-0.035663552040944,
-0.0122330739255528));
#25063=CARTESIAN_POINT('Ctrl Pts',(-0.0109576636510691,-0.035664109086248,
-0.0122223566835455));
#25064=CARTESIAN_POINT('Ctrl Pts',(-0.0109569136485729,-0.0356657997806266,
-0.0121900249013261));
#25065=CARTESIAN_POINT('Ctrl Pts',(-0.0109568665669177,-0.0356669440732218,
-0.0121684057175958));
#25066=CARTESIAN_POINT('Ctrl Pts',(-0.0109592410085505,-0.0356736985751078,
-0.0120423518205215));
#25067=CARTESIAN_POINT('Ctrl Pts',(-0.0109718087919673,-0.035679626460196,
-0.0119383944508523));
#25068=CARTESIAN_POINT('Ctrl Pts',(-0.0110097316105512,-0.0356895421858127,
-0.011770175775862));
#25069=CARTESIAN_POINT('Ctrl Pts',(-0.0110290581599853,-0.0356934675244374,
-0.0117048916354903));
#25070=CARTESIAN_POINT('Ctrl Pts',(-0.0110601871920318,-0.0356984853357591,
-0.0116206383538668));
#25071=CARTESIAN_POINT('Ctrl Pts',(-0.011068177974536,-0.035699689769178,
-0.0116003445464052));
#25072=CARTESIAN_POINT('Ctrl Pts',(-0.0110824716121913,-0.0357017019349492,
-0.0115661862422581));
#25073=CARTESIAN_POINT('Ctrl Pts',(-0.0110885542779068,-0.0357025194664206,
-0.0115522334961816));
#25074=CARTESIAN_POINT('Ctrl Pts',(-0.0110975583502747,-0.0357036736439031,
-0.0115323864046457));
#25075=CARTESIAN_POINT('Ctrl Pts',(-0.0111003123642749,-0.0357040196075081,
-0.011526417581899));
#25076=CARTESIAN_POINT('Ctrl Pts',(-0.0111051679466173,-0.0357046172303319,
-0.0115160683642111));
#25077=CARTESIAN_POINT('Ctrl Pts',(-0.0111072521887665,-0.0357048699269926,
-0.0115116800128579));
#25078=CARTESIAN_POINT('Ctrl Pts',(-0.011111746590513,-0.0357054066688588,
-0.0115023312881098));
#25079=CARTESIAN_POINT('Ctrl Pts',(-0.0111141626440735,-0.0357056903493329,
-0.0114973739308591));
#25080=CARTESIAN_POINT('Ctrl Pts',(-0.0111208218361023,-0.0357064594261836,
-0.0114838943122178));
#25081=CARTESIAN_POINT('Ctrl Pts',(-0.0111251174143067,-0.0357069416761742,
-0.0114753980673129));
#25082=CARTESIAN_POINT('Ctrl Pts',(-0.0111482697008385,-0.035709471740201,
-0.0114306387248139));
#25083=CARTESIAN_POINT('Ctrl Pts',(-0.0111684844176995,-0.0357114444378021,
-0.0113950932149696));
#25084=CARTESIAN_POINT('Ctrl Pts',(-0.0112343653579111,-0.0357173289109132,
-0.0112892659824057));
#25085=CARTESIAN_POINT('Ctrl Pts',(-0.0112843632695977,-0.0357210991646329,
-0.0112218634153045));
#25086=CARTESIAN_POINT('Ctrl Pts',(-0.0113918466557909,-0.0357285905173704,
-0.0110992235615449));
#25087=CARTESIAN_POINT('Ctrl Pts',(-0.0114486195185337,-0.0357322931406509,
-0.0110437168676197));
#25088=CARTESIAN_POINT('Ctrl Pts',(-0.0115255665755736,-0.0357372208744698,
-0.0109792861058802));
#25089=CARTESIAN_POINT('Ctrl Pts',(-0.0115420067217226,-0.0357382684137658,
-0.0109660837459334));
#25090=CARTESIAN_POINT('Ctrl Pts',(-0.0115671252196121,-0.0357398637809694,
-0.0109467453222488));
#25091=CARTESIAN_POINT('Ctrl Pts',(-0.0115756051946543,-0.0357404015124628,
-0.0109403550144667));
#25092=CARTESIAN_POINT('Ctrl Pts',(-0.0115910412616539,-0.0357413791122815,
-0.0109289706433845));
#25093=CARTESIAN_POINT('Ctrl Pts',(-0.0115979742973058,-0.0357418177561619,
-0.0109239459650628));
#25094=CARTESIAN_POINT('Ctrl Pts',(-0.0116129585651714,-0.0357427650096174,
-0.0109132752942515));
#25095=CARTESIAN_POINT('Ctrl Pts',(-0.0116210226409081,-0.0357432743163894,
-0.0109076480626554));
#25096=CARTESIAN_POINT('Ctrl Pts',(-0.0116430094375146,-0.0357446619019811,
-0.0108926157944065));
#25097=CARTESIAN_POINT('Ctrl Pts',(-0.011657032607279,-0.035745545796952,
-0.0108833606443831));
#25098=CARTESIAN_POINT('Ctrl Pts',(-0.0117484809983781,-0.0357513044388423,
-0.0108251269832672));
#25099=CARTESIAN_POINT('Ctrl Pts',(-0.0118299762477806,-0.0357564277451144,
-0.010782904518244));
#25100=CARTESIAN_POINT('Ctrl Pts',(-0.0119926333580017,-0.0357664852478599,
-0.0107162238407659));
#25101=CARTESIAN_POINT('Ctrl Pts',(-0.0120730268582602,-0.0357713809695852,
-0.010690715827138));
#25102=CARTESIAN_POINT('Ctrl Pts',(-0.0121788509745417,-0.035777472936617,
-0.0106664474247667));
#25103=CARTESIAN_POINT('Ctrl Pts',(-0.0122027282525893,-0.03577882431594,
-0.0106615638936586));
#25104=CARTESIAN_POINT('Ctrl Pts',(-0.0122429724663214,-0.0357810524983995,
-0.0106543215560742));
#25105=CARTESIAN_POINT('Ctrl Pts',(-0.0122592793707944,-0.0357819418388727,
-0.0106516565860661));
#25106=CARTESIAN_POINT('Ctrl Pts',(-0.0122823438622849,-0.035783177681601,
-0.0106482666596645));
#25107=CARTESIAN_POINT('Ctrl Pts',(-0.0122890677373651,-0.0357835353283668,
-0.010647323705256));
#25108=CARTESIAN_POINT('Ctrl Pts',(-0.012300643912423,-0.0357841462860588,
-0.0106457781072292));
#25109=CARTESIAN_POINT('Ctrl Pts',(-0.0123054932135286,-0.0357844007720166,
-0.0106451540945236));
#25110=CARTESIAN_POINT('Ctrl Pts',(-0.0123157120487281,-0.0357849339146059,
-0.0106438884723644));
#25111=CARTESIAN_POINT('Ctrl Pts',(-0.0123210820699328,-0.035785212286465,
-0.010643252028253));
#25112=CARTESIAN_POINT('Ctrl Pts',(-0.0123356752054156,-0.0357859641576637,
-0.0106416002253992));
#25113=CARTESIAN_POINT('Ctrl Pts',(-0.0123449044475783,-0.0357864346750686,
-0.0106406397927773));
#25114=CARTESIAN_POINT('Ctrl Pts',(-0.0123897463113916,-0.0357886989309618,
-0.0106363818771694));
#25115=CARTESIAN_POINT('Ctrl Pts',(-0.0124254598653898,-0.0357904355883029,
-0.0106342397785467));
#25116=CARTESIAN_POINT('Ctrl Pts',(-0.0125485986406493,-0.0357962896463038,
-0.0106311437973323));
#25117=CARTESIAN_POINT('Ctrl Pts',(-0.0126360124487232,-0.0358002211655603,
-0.0106363756144821));
#25118=CARTESIAN_POINT('Ctrl Pts',(-0.0127963420740552,-0.0358076581588916,
-0.0106597410437196));
#25119=CARTESIAN_POINT('Ctrl Pts',(-0.0128692853572265,-0.0358111313058451,
-0.0106758392841192));
#25120=CARTESIAN_POINT('Ctrl Pts',(-0.0129652689056642,-0.0358160115089282,
-0.010704450157234));
#25121=CARTESIAN_POINT('Ctrl Pts',(-0.0129895778562697,-0.035817274444655,
-0.010712358922853));
#25122=CARTESIAN_POINT('Ctrl Pts',(-0.0130244713756424,-0.0358191315425556,
-0.0107246779749105));
#25123=CARTESIAN_POINT('Ctrl Pts',(-0.013035221477153,-0.0358197098504035,
-0.0107286083279273));
#25124=CARTESIAN_POINT('Ctrl Pts',(-0.0130540235151206,-0.0358207325892026,
-0.0107357206938683));
#25125=CARTESIAN_POINT('Ctrl Pts',(-0.0130620943239165,-0.0358211752876358,
-0.0107388515792498));
#25126=CARTESIAN_POINT('Ctrl Pts',(-0.013078845384833,-0.0358221019787196,
-0.0107455124802516));
#25127=CARTESIAN_POINT('Ctrl Pts',(-0.0130875206639524,-0.0358225863471656,
-0.0107490539783336));
#25128=CARTESIAN_POINT('Ctrl Pts',(-0.0131100806439124,-0.0358238577821161,
-0.0107585042479233));
#25129=CARTESIAN_POINT('Ctrl Pts',(-0.0131239116442288,-0.035824649084183,
-0.0107645379682441));
#25130=CARTESIAN_POINT('Ctrl Pts',(-0.0131837227946175,-0.0358281236661638,
-0.0107916813906519));
#25131=CARTESIAN_POINT('Ctrl Pts',(-0.0132287337563207,-0.0358308768061549,
-0.0108148407845955));
#25132=CARTESIAN_POINT('Ctrl Pts',(-0.0133580888275027,-0.035839193754723,
-0.0108896560860379));
#25133=CARTESIAN_POINT('Ctrl Pts',(-0.0134386966940992,-0.0358449296268151,
-0.0109472502910151));
#25134=CARTESIAN_POINT('Ctrl Pts',(-0.0135574242818815,-0.0358539404575158,
-0.0110506261666084));
#25135=CARTESIAN_POINT('Ctrl Pts',(-0.0135993906310767,-0.0358572543292559,
-0.0110915915455285));
#25136=CARTESIAN_POINT('Ctrl Pts',(-0.0136480799681388,-0.0358611613542917,
-0.0111448608462335));
#25137=CARTESIAN_POINT('Ctrl Pts',(-0.0136571000404844,-0.0358618879504305,
-0.0111549945567507));
#25138=CARTESIAN_POINT('Ctrl Pts',(-0.0136700982185564,-0.0358629373931393,
-0.0111699911751856));
#25139=CARTESIAN_POINT('Ctrl Pts',(-0.0136741819175222,-0.0358632674573547,
-0.0111747612551081));
#25140=CARTESIAN_POINT('Ctrl Pts',(-0.0136813536579705,-0.0358638475325092,
-0.0111832426671715));
#25141=CARTESIAN_POINT('Ctrl Pts',(-0.0136844535431825,-0.0358640983920467,
-0.0111869437290948));
#25142=CARTESIAN_POINT('Ctrl Pts',(-0.0136911777512973,-0.0358646428065021,
-0.0111950489766623));
#25143=CARTESIAN_POINT('Ctrl Pts',(-0.0136947950605076,-0.0358649358653873,
-0.0111994587480089));
#25144=CARTESIAN_POINT('Ctrl Pts',(-0.0137049057401215,-0.0358657558476487,
-0.0112119247516473));
#25145=CARTESIAN_POINT('Ctrl Pts',(-0.0137113427571681,-0.0358662789044783,
-0.011220026524731));
#25146=CARTESIAN_POINT('Ctrl Pts',(-0.0137558875444062,-0.0358699104599345,
-0.0112772644152026));
#25147=CARTESIAN_POINT('Ctrl Pts',(-0.0137910797333647,-0.0358728430552178,
-0.0113286047588747));
#25148=CARTESIAN_POINT('Ctrl Pts',(-0.0138590239319443,-0.0358789514660897,
-0.0114418348156645));
#25149=CARTESIAN_POINT('Ctrl Pts',(-0.0138908587964206,-0.0358821075324161,
-0.0115041083911386));
#25150=CARTESIAN_POINT('Ctrl Pts',(-0.0139466453468204,-0.0358886443007121,
-0.0116343504305186));
#25151=CARTESIAN_POINT('Ctrl Pts',(-0.0139702790972508,-0.0358920218825581,
-0.0117022647089915));
#25152=CARTESIAN_POINT('Ctrl Pts',(-0.0139943697395063,-0.0358965446035975,
-0.0117909984710678));
#25153=CARTESIAN_POINT('Ctrl Pts',(-0.0139992627618673,-0.0358975459972766,
-0.0118105242962637));
#25154=CARTESIAN_POINT('Ctrl Pts',(-0.014006109641926,-0.0358990850461903,
-0.0118403066050354));
#25155=CARTESIAN_POINT('Ctrl Pts',(-0.0140083437815026,-0.0358996136832455,
-0.011850496776193));
#25156=CARTESIAN_POINT('Ctrl Pts',(-0.0140120526384652,-0.0359005397057748,
-0.0118682731650658));
#25157=CARTESIAN_POINT('Ctrl Pts',(-0.0140135740262824,-0.0359009355747758,
-0.0118758493254116));
#25158=CARTESIAN_POINT('Ctrl Pts',(-0.0140168739668857,-0.0359018317763048,
-0.0118929466232066));
#25159=CARTESIAN_POINT('Ctrl Pts',(-0.0140186198956436,-0.0359023331364207,
-0.0119024736633533));
#25160=CARTESIAN_POINT('Ctrl Pts',(-0.0140231048398058,-0.0359036986921826,
-0.0119283167217085));
#25161=CARTESIAN_POINT('Ctrl Pts',(-0.0140256712723982,-0.0359045683313978,
-0.0119446610640595));
#25162=CARTESIAN_POINT('Ctrl Pts',(-0.0140379803374731,-0.0359092602595188,
-0.0120322171326661));
#25163=CARTESIAN_POINT('Ctrl Pts',(-0.014043,-0.0359132300652073,-0.0121039945751363));
#25164=CARTESIAN_POINT('Ctrl Pts',(-0.014043,-0.0359172995678105,-0.0121758532865631));
#25165=CARTESIAN_POINT('Origin',(-0.0125,-0.0375520664398416,-0.0121758532865581));
#25166=CARTESIAN_POINT('',(-0.0140437065963746,-0.0364192084819633,-0.0121758951269253));
#25167=CARTESIAN_POINT('',(-0.014043,-0.0363035228772662,-0.012175853286558));
#25168=CARTESIAN_POINT('',(-0.014043,-0.0375520664398416,-0.012175853286558));
#25169=CARTESIAN_POINT('',(-0.0118291591918074,-0.0365787743898683,-0.0135653933579797));
#25170=CARTESIAN_POINT('Ctrl Pts',(-0.0140437065963746,-0.0364192084819633,
-0.0121758951269253));
#25171=CARTESIAN_POINT('Ctrl Pts',(-0.0140437112943485,-0.036419761179091,
-0.0121864484221882));
#25172=CARTESIAN_POINT('Ctrl Pts',(-0.0140436034281201,-0.0364203105081606,
-0.0121969992050036));
#25173=CARTESIAN_POINT('Ctrl Pts',(-0.0140433816474543,-0.036420856696369,
-0.0122075457453187));
#25174=CARTESIAN_POINT('Ctrl Pts',(-0.0140366019703916,-0.0364375532810555,
-0.0125299459744092));
#25175=CARTESIAN_POINT('Ctrl Pts',(-0.0139230960548442,-0.0364513147894128,
-0.012850374408135));
#25176=CARTESIAN_POINT('Ctrl Pts',(-0.0137289094917718,-0.0364686314224829,
-0.0131077331936447));
#25177=CARTESIAN_POINT('Ctrl Pts',(-0.0136165391819018,-0.0364786520716628,
-0.0132566594943009));
#25178=CARTESIAN_POINT('Ctrl Pts',(-0.0134773604198345,-0.0364896481824746,
-0.0133847691368121));
#25179=CARTESIAN_POINT('Ctrl Pts',(-0.0133205998717288,-0.036499396683921,
-0.0134832463847913));
#25180=CARTESIAN_POINT('Ctrl Pts',(-0.0133159948840397,-0.0364996830552669,
-0.0134861392460379));
#25181=CARTESIAN_POINT('Ctrl Pts',(-0.0133113740270396,-0.0364999685740012,
-0.0134890066645617));
#25182=CARTESIAN_POINT('Ctrl Pts',(-0.0133067374026243,-0.0365002532689413,
-0.0134918483279206));
#25183=CARTESIAN_POINT('Ctrl Pts',(-0.0130296930677077,-0.0365172641616254,
-0.013661641406849));
#25184=CARTESIAN_POINT('Ctrl Pts',(-0.0126940553902617,-0.0365313339299439,
-0.0137398854281534));
#25185=CARTESIAN_POINT('Ctrl Pts',(-0.0123670284176581,-0.0365486100887429,
-0.0137121595855382));
#25186=CARTESIAN_POINT('Ctrl Pts',(-0.0121807148347873,-0.0365584526501025,
-0.0136963636374712));
#25187=CARTESIAN_POINT('Ctrl Pts',(-0.0119971991141735,-0.0365691508384448,
-0.0136465196655769));
#25188=CARTESIAN_POINT('Ctrl Pts',(-0.0118291591918087,-0.0365787743898699,
-0.0135653933579771));
#25189=CARTESIAN_POINT('',(-0.0110424215937398,-0.0365780008767028,-0.0116655070342102));
#25190=CARTESIAN_POINT('Origin',(-0.01249999999999,-0.0365787743898623,
-0.0121758532865681));
#25191=CARTESIAN_POINT('Ctrl Pts',(-0.0110436695558073,-0.0365772219729834,
-0.0116659997415889));
#25192=CARTESIAN_POINT('Ctrl Pts',(-0.0110413413253198,-0.0365768613442727,
-0.0116726500296443));
#25193=CARTESIAN_POINT('Ctrl Pts',(-0.0110390586313932,-0.0365765033099709,
-0.0116793163109309));
#25194=CARTESIAN_POINT('Ctrl Pts',(-0.0110331441531789,-0.0365755630462582,
-0.0116969826275963));
#25195=CARTESIAN_POINT('Ctrl Pts',(-0.0110295903814817,-0.0365749849430677,
-0.0117080084925528));
#25196=CARTESIAN_POINT('Ctrl Pts',(-0.0110018695876898,-0.0365703579284431,
-0.0117974520234474));
#25197=CARTESIAN_POINT('Ctrl Pts',(-0.0109838665983412,-0.0365665919497779,
-0.0118776513718294));
#25198=CARTESIAN_POINT('Ctrl Pts',(-0.0109610197781968,-0.0365591623540998,
-0.0120385331394252));
#25199=CARTESIAN_POINT('Ctrl Pts',(-0.0109559550810136,-0.0365555071961878,
-0.0121189184109854));
#25200=CARTESIAN_POINT('Ctrl Pts',(-0.0109576515052428,-0.03655022296515,
-0.0122304092373323));
#25201=CARTESIAN_POINT('Ctrl Pts',(-0.0109590634848909,-0.0365487288644723,
-0.0122614672222852));
#25202=CARTESIAN_POINT('Ctrl Pts',(-0.0109631698988874,-0.0365460697877951,
-0.012315649868047));
#25203=CARTESIAN_POINT('Ctrl Pts',(-0.0109654513753443,-0.036544917066,
-0.0123387958887093));
#25204=CARTESIAN_POINT('Ctrl Pts',(-0.0109695920243148,-0.0365431907320122,
-0.0123728898705308));
#25205=CARTESIAN_POINT('Ctrl Pts',(-0.0109710476816302,-0.03654262967808,
-0.0123838840232355));
#25206=CARTESIAN_POINT('Ctrl Pts',(-0.0109738529018824,-0.0365416231574254,
-0.0124034478349961));
#25207=CARTESIAN_POINT('Ctrl Pts',(-0.0109751564699005,-0.0365411791495177,
-0.0124120236662987));
#25208=CARTESIAN_POINT('Ctrl Pts',(-0.010978068081404,-0.0365402346714895,
-0.0124301483828666));
#25209=CARTESIAN_POINT('Ctrl Pts',(-0.010979693837407,-0.0365397336622288,
-0.0124396940096787));
#25210=CARTESIAN_POINT('Ctrl Pts',(-0.0109842970108224,-0.0365383817039533,
-0.0124652649548254));
#25211=CARTESIAN_POINT('Ctrl Pts',(-0.0109874386312575,-0.036537525648099,
-0.0124812591541087));
#25212=CARTESIAN_POINT('Ctrl Pts',(-0.0110048757141424,-0.0365330878068891,
-0.0125631503139248));
#25213=CARTESIAN_POINT('Ctrl Pts',(-0.0110232247437051,-0.0365293801249451,
-0.0126281018280259));
#25214=CARTESIAN_POINT('Ctrl Pts',(-0.0110792690894689,-0.0365199418545631,
-0.0127861167056582));
#25215=CARTESIAN_POINT('Ctrl Pts',(-0.0111219029326016,-0.0365141171036886,
-0.0128770987029434));
#25216=CARTESIAN_POINT('Ctrl Pts',(-0.0111864714025118,-0.0365070199561684,
-0.012985904180547));
#25217=CARTESIAN_POINT('Ctrl Pts',(-0.011200460812554,-0.0365055618840411,
-0.0130081620321976));
#25218=CARTESIAN_POINT('Ctrl Pts',(-0.0112246982922675,-0.0365031760519759,
-0.0130446229127339));
#25219=CARTESIAN_POINT('Ctrl Pts',(-0.0112346315146955,-0.0365022341795758,
-0.0130590281018188));
#25220=CARTESIAN_POINT('Ctrl Pts',(-0.0112488954723028,-0.0365009342774367,
-0.0130789788889831));
#25221=CARTESIAN_POINT('Ctrl Pts',(-0.0112530220518657,-0.0365005641265106,
-0.0130846681155898));
#25222=CARTESIAN_POINT('Ctrl Pts',(-0.0112601502576373,-0.0364999350416149,
-0.0130943556590413));
#25223=CARTESIAN_POINT('Ctrl Pts',(-0.011263132681514,-0.0364996748537728,
-0.0130983679097475));
#25224=CARTESIAN_POINT('Ctrl Pts',(-0.0112693765992203,-0.0364991364985014,
-0.0131066831295149));
#25225=CARTESIAN_POINT('Ctrl Pts',(-0.0112726412832027,-0.0364988585582687,
-0.0131109836160336));
#25226=CARTESIAN_POINT('Ctrl Pts',(-0.0112815235986745,-0.036498111607591,
-0.0131225574195308));
#25227=CARTESIAN_POINT('Ctrl Pts',(-0.0112871838259889,-0.0364976454637784,
-0.0131297979347385));
#25228=CARTESIAN_POINT('Ctrl Pts',(-0.0113143539787749,-0.0364954518495148,
-0.0131639210106748));
#25229=CARTESIAN_POINT('Ctrl Pts',(-0.0113366962779269,-0.036493776475585,
-0.0131901308971525));
#25230=CARTESIAN_POINT('Ctrl Pts',(-0.0114191879601148,-0.0364879423349833,
-0.0132805869397727));
#25231=CARTESIAN_POINT('Ctrl Pts',(-0.0114839332225997,-0.0364839774412235,
-0.0133404137763914));
#25232=CARTESIAN_POINT('Ctrl Pts',(-0.0116236752279367,-0.0364758436404758,
-0.0134489660993623));
#25233=CARTESIAN_POINT('Ctrl Pts',(-0.0116985037441817,-0.0364716849115544,
-0.0134973535182993));
#25234=CARTESIAN_POINT('Ctrl Pts',(-0.0117918364787748,-0.0364664504687041,
-0.0135468501986224));
#25235=CARTESIAN_POINT('Ctrl Pts',(-0.0118067216300561,-0.0364656147820267,
-0.0135544370454084));
#25236=CARTESIAN_POINT('Ctrl Pts',(-0.0118304430635244,-0.0364642803300907,
-0.0135660463239072));
#25237=CARTESIAN_POINT('Ctrl Pts',(-0.011839199355654,-0.0364637871813342,
-0.0135702297332574));
#25238=CARTESIAN_POINT('Ctrl Pts',(-0.0118557496459913,-0.0364628537850768,
-0.0135779459006358));
#25239=CARTESIAN_POINT('Ctrl Pts',(-0.0118635347276592,-0.0364624141931766,
-0.0135814969719489));
#25240=CARTESIAN_POINT('Ctrl Pts',(-0.0118811676824705,-0.0364614171746888,
-0.0135893635131932));
#25241=CARTESIAN_POINT('Ctrl Pts',(-0.0118910318671119,-0.036460858477707,
-0.0135936411420864));
#25242=CARTESIAN_POINT('Ctrl Pts',(-0.0119210661205281,-0.0364591541865196,
-0.0136062943118299));
#25243=CARTESIAN_POINT('Ctrl Pts',(-0.011941369454711,-0.0364579977204633,
-0.0136143447921375));
#25244=CARTESIAN_POINT('Ctrl Pts',(-0.0120527574339059,-0.0364516274201177,
-0.0136557974226373));
#25245=CARTESIAN_POINT('Ctrl Pts',(-0.0121466548019251,-0.0364461451595593,
-0.0136809788599299));
#25246=CARTESIAN_POINT('Ctrl Pts',(-0.0123415290797136,-0.0364347883212946,
-0.0137139913812855));
#25247=CARTESIAN_POINT('Ctrl Pts',(-0.0124421895407285,-0.0364289365899841,
-0.0137210530108708));
#25248=CARTESIAN_POINT('Ctrl Pts',(-0.0125550736832121,-0.0364228218462438,
-0.0137179187985579));
#25249=CARTESIAN_POINT('Ctrl Pts',(-0.012567318580438,-0.0364221647166439,
-0.013717432794944));
#25250=CARTESIAN_POINT('Ctrl Pts',(-0.0125856534854465,-0.036421191296847,
-0.0137164861921277));
#25251=CARTESIAN_POINT('Ctrl Pts',(-0.0125917484028276,-0.0364208694574206,
-0.0137161352420211));
#25252=CARTESIAN_POINT('Ctrl Pts',(-0.0126027345821641,-0.036420292685185,
-0.0137154372068821));
#25253=CARTESIAN_POINT('Ctrl Pts',(-0.0126076265510193,-0.0364200370559862,
-0.0137151029638449));
#25254=CARTESIAN_POINT('Ctrl Pts',(-0.0126176258330754,-0.0364195171130362,
-0.0137143718610214));
#25255=CARTESIAN_POINT('Ctrl Pts',(-0.0126227329326062,-0.0364192529242134,
-0.0137139728753217));
#25256=CARTESIAN_POINT('Ctrl Pts',(-0.0126359960318198,-0.0364185701728793,
-0.0137128702325989));
#25257=CARTESIAN_POINT('Ctrl Pts',(-0.0126441486869814,-0.0364181537836636,
-0.0137121270820833));
#25258=CARTESIAN_POINT('Ctrl Pts',(-0.0126801668027033,-0.0364163272435666,
-0.0137085546243455));
#25259=CARTESIAN_POINT('Ctrl Pts',(-0.0127079595924972,-0.0364149523757724,
-0.0137050316462605));
#25260=CARTESIAN_POINT('Ctrl Pts',(-0.0127881091964472,-0.0364110489374761,
-0.0136926461434163));
#25261=CARTESIAN_POINT('Ctrl Pts',(-0.012840125523996,-0.0364085914089047,
-0.0136818356039508));
#25262=CARTESIAN_POINT('Ctrl Pts',(-0.0130152296410503,-0.0364002894449418,
-0.0136359060510962));
#25263=CARTESIAN_POINT('Ctrl Pts',(-0.0131344473943982,-0.0363945393897937,
-0.0135881883457398));
#25264=CARTESIAN_POINT('Ctrl Pts',(-0.0132618881358502,-0.0363873732161357,
-0.0135177505513322));
#25265=CARTESIAN_POINT('Ctrl Pts',(-0.0132772186293565,-0.0363864939817884,
-0.0135089297925464));
#25266=CARTESIAN_POINT('Ctrl Pts',(-0.0133017351985128,-0.0363850581900037,
-0.0134942569389985));
#25267=CARTESIAN_POINT('Ctrl Pts',(-0.0133110170662623,-0.0363845075691182,
-0.0134885675851075));
#25268=CARTESIAN_POINT('Ctrl Pts',(-0.0133274176793357,-0.0363835217115884,
-0.0134782744319408));
#25269=CARTESIAN_POINT('Ctrl Pts',(-0.0133345602036579,-0.0363830879287251,
-0.0134737092564782));
#25270=CARTESIAN_POINT('Ctrl Pts',(-0.0133495578165482,-0.0363821675132236,
-0.0134639484723184));
#25271=CARTESIAN_POINT('Ctrl Pts',(-0.0133574036588562,-0.0363816803791029,
-0.0134587393499677));
#25272=CARTESIAN_POINT('Ctrl Pts',(-0.0133782216519824,-0.0363803724984877,
-0.0134446412950377));
#25273=CARTESIAN_POINT('Ctrl Pts',(-0.0133911061947453,-0.0363795469151349,
-0.0134356254902591));
#25274=CARTESIAN_POINT('Ctrl Pts',(-0.0134589528571959,-0.0363751116892407,
-0.0133865889232085));
#25275=CARTESIAN_POINT('Ctrl Pts',(-0.0135113565166372,-0.0363713689783282,
-0.0133431696584503));
#25276=CARTESIAN_POINT('Ctrl Pts',(-0.0136300417414365,-0.0363621389831824,
-0.0132308250161338));
#25277=CARTESIAN_POINT('Ctrl Pts',(-0.0136931189529005,-0.0363565699079917,
-0.0131589226767223));
#25278=CARTESIAN_POINT('Ctrl Pts',(-0.0137784575429079,-0.0363483039904904,
-0.0130412365326283));
#25279=CARTESIAN_POINT('Ctrl Pts',(-0.0138057910623317,-0.0363455122864103,
-0.012999414091956));
#25280=CARTESIAN_POINT('Ctrl Pts',(-0.0138360674834308,-0.036342300838994,
-0.0129477801386804));
#25281=CARTESIAN_POINT('Ctrl Pts',(-0.0138410022080424,-0.0363417731941031,
-0.0129391752851103));
#25282=CARTESIAN_POINT('Ctrl Pts',(-0.013848569380809,-0.0363409581287575,
-0.0129256802362088));
#25283=CARTESIAN_POINT('Ctrl Pts',(-0.0138512589063317,-0.0363406672233578,
-0.0129208225471677));
#25284=CARTESIAN_POINT('Ctrl Pts',(-0.0138559859010768,-0.0363401539126488,
-0.0129121750558806));
#25285=CARTESIAN_POINT('Ctrl Pts',(-0.0138580337537298,-0.0363399308538065,
-0.0129083912281472));
#25286=CARTESIAN_POINT('Ctrl Pts',(-0.0138629145975095,-0.0363393974964837,
-0.0128992820548153));
#25287=CARTESIAN_POINT('Ctrl Pts',(-0.0138657322196297,-0.036339088170409,
-0.0128939486071689));
#25288=CARTESIAN_POINT('Ctrl Pts',(-0.0138742494954952,-0.0363381482922685,
-0.012877594871444));
#25289=CARTESIAN_POINT('Ctrl Pts',(-0.0138798476981278,-0.0363375237742507,
-0.0128665220032575));
#25290=CARTESIAN_POINT('Ctrl Pts',(-0.0139225301212537,-0.0363326990408032,
-0.0127795081289901));
#25291=CARTESIAN_POINT('Ctrl Pts',(-0.0139534560740148,-0.0363288136101808,
-0.0127006957296058));
#25292=CARTESIAN_POINT('Ctrl Pts',(-0.0140114615447175,-0.0363195886396248,
-0.0125075858141706));
#25293=CARTESIAN_POINT('Ctrl Pts',(-0.014032270353752,-0.0363142705475785,
-0.0123919727712827));
#25294=CARTESIAN_POINT('Ctrl Pts',(-0.0140410174835801,-0.036307579139371,
-0.0122562906716157));
#25295=CARTESIAN_POINT('Ctrl Pts',(-0.0140418858837587,-0.0363066405351284,
-0.0122374401385291));
#25296=CARTESIAN_POINT('Ctrl Pts',(-0.0140426307508922,-0.0363052870875798,
-0.0122105502030893));
#25297=CARTESIAN_POINT('Ctrl Pts',(-0.0140427904568757,-0.0363048810602615,
-0.0122025199818726));
#25298=CARTESIAN_POINT('Ctrl Pts',(-0.0140429624864267,-0.0363041575108634,
-0.0121882772977707));
#25299=CARTESIAN_POINT('Ctrl Pts',(-0.014043,-0.0363038407833747,-0.0121820652889604));
#25300=CARTESIAN_POINT('Ctrl Pts',(-0.014043,-0.0363035228772662,-0.012175853286558));
#25301=CARTESIAN_POINT('Origin',(0.006,-0.0412787743898723,-0.0121758532865581));
#25302=CARTESIAN_POINT('',(0.00473550001147424,-0.0374057743898623,-0.0121760236343295));
#25303=CARTESIAN_POINT('',(0.00473550000005949,-0.0373433241596449,-0.0121758410210368));
#25304=CARTESIAN_POINT('',(0.0047355,-0.0412787743898723,-0.0121758532865581));
#25305=CARTESIAN_POINT('',(0.00648836437725255,-0.0369998285136293,-0.013342241080151));
#25306=CARTESIAN_POINT('Ctrl Pts',(0.00473550025703334,-0.0373432743898623,
-0.0121750470376861));
#25307=CARTESIAN_POINT('Ctrl Pts',(0.00473568325203442,-0.0373252099538459,
-0.0118880424416283));
#25308=CARTESIAN_POINT('Ctrl Pts',(0.00483793644636973,-0.0373071455178294,
-0.0116004870680416));
#25309=CARTESIAN_POINT('Ctrl Pts',(0.00501920341792046,-0.0372890810818129,
-0.0113777315448538));
#25310=CARTESIAN_POINT('Ctrl Pts',(0.00512512778104792,-0.0372785250281429,
-0.0112475631157962));
#25311=CARTESIAN_POINT('Ctrl Pts',(0.00525693102794947,-0.0372679689744728,
-0.0111393205108283));
#25312=CARTESIAN_POINT('Ctrl Pts',(0.00540338669147187,-0.0372574129208027,
-0.0110609484430458));
#25313=CARTESIAN_POINT('Ctrl Pts',(0.00564541444099014,-0.0372399683382436,
-0.0109314333752479));
#25314=CARTESIAN_POINT('Ctrl Pts',(0.00593538390252328,-0.0372225237556846,
-0.0108827068727731));
#25315=CARTESIAN_POINT('Ctrl Pts',(0.00620981161123333,-0.0372050791731255,
-0.0109288812187909));
#25316=CARTESIAN_POINT('Ctrl Pts',(0.00638562427830956,-0.037193903265998,
-0.0109584629070323));
#25317=CARTESIAN_POINT('Ctrl Pts',(0.0065544278780534,-0.0371827273588706,
-0.0110258476768364));
#25318=CARTESIAN_POINT('Ctrl Pts',(0.0067008437840681,-0.0371715514517431,
-0.0111233428398959));
#25319=CARTESIAN_POINT('Ctrl Pts',(0.00692938580140116,-0.0371541068691841,
-0.011275523991878));
#25320=CARTESIAN_POINT('Ctrl Pts',(0.00710929857406147,-0.037136662286625,
-0.0115081326048137));
#25321=CARTESIAN_POINT('Ctrl Pts',(0.00719821248300049,-0.0371192177040659,
-0.01177181480376));
#25322=CARTESIAN_POINT('Ctrl Pts',(0.00725517535874009,-0.0371080417969385,
-0.0119407433382553));
#25323=CARTESIAN_POINT('Ctrl Pts',(0.00727550551639853,-0.0370968658898111,
-0.0121213293802333));
#25324=CARTESIAN_POINT('Ctrl Pts',(0.0072587419762938,-0.0370856899826836,
-0.0122963891198857));
#25325=CARTESIAN_POINT('Ctrl Pts',(0.00723164584045649,-0.0370676255466671,
-0.0125793509797095));
#25326=CARTESIAN_POINT('Ctrl Pts',(0.00710450570407131,-0.0370495611106507,
-0.0128555001058568));
#25327=CARTESIAN_POINT('Ctrl Pts',(0.00690294869731533,-0.0370314966746343,
-0.0130610899215979));
#25328=CARTESIAN_POINT('Ctrl Pts',(0.00678516773925136,-0.0370209406209642,
-0.0131812274740249));
#25329=CARTESIAN_POINT('Ctrl Pts',(0.00664306435621841,-0.0370103845672941,
-0.0132774684896714));
#25330=CARTESIAN_POINT('Ctrl Pts',(0.00648836437725186,-0.036999828513624,
-0.0133422410801462));
#25331=CARTESIAN_POINT('',(0.00629997434768202,-0.0370498280494119,-0.0134042879004366));
#25332=CARTESIAN_POINT('Ctrl Pts',(0.00648836437725163,-0.0369998285136324,
-0.0133422410801463));
#25333=CARTESIAN_POINT('Ctrl Pts',(0.00642782011983403,-0.0370199281538104,
-0.0133675908469498));
#25334=CARTESIAN_POINT('Ctrl Pts',(0.00636459046969111,-0.0370367243067544,
-0.0133884784301787));
#25335=CARTESIAN_POINT('Ctrl Pts',(0.00629996344159552,-0.0370494722341879,
-0.0134042596459141));
#25336=CARTESIAN_POINT('Ctrl Pts',(0.0062999658725511,-0.0370498392335843,
-0.013404259015438));
#25337=CARTESIAN_POINT('Ctrl Pts',(0.00657769650495509,-0.0370678301487587,
-0.0133364248152246));
#25338=CARTESIAN_POINT('Ctrl Pts',(0.00683220741234104,-0.0370858210639329,
-0.0131699966762561));
#25339=CARTESIAN_POINT('Ctrl Pts',(0.00711803563641934,-0.0371154591215677,
-0.0127949611817838));
#25340=CARTESIAN_POINT('Ctrl Pts',(0.0071968245232809,-0.0371271062640282,
-0.0126231472652464));
#25341=CARTESIAN_POINT('Ctrl Pts',(0.00729359082809241,-0.0371561129842236,
-0.012177703957702));
#25342=CARTESIAN_POINT('Ctrl Pts',(0.00726184701836556,-0.0371734725619587,
-0.0118867675894431));
#25343=CARTESIAN_POINT('Ctrl Pts',(0.00705957405455359,-0.0372031403991936,
-0.0114582842983591));
#25344=CARTESIAN_POINT('Ctrl Pts',(0.00693355052798508,-0.0372154486586936,
-0.0113012882727189));
#25345=CARTESIAN_POINT('Ctrl Pts',(0.00656697755162586,-0.0372451164959285,
-0.0110131261916979));
#25346=CARTESIAN_POINT('Ctrl Pts',(0.00629140300613193,-0.0372624760736636,
-0.0109145405765421));
#25347=CARTESIAN_POINT('Ctrl Pts',(0.00581761467049966,-0.0372921439108985,
-0.0109092292197413));
#25348=CARTESIAN_POINT('Ctrl Pts',(0.00562134440445418,-0.0373044521703985,
-0.0109539728290903));
#25349=CARTESIAN_POINT('Ctrl Pts',(0.00519265839058833,-0.0373347811246729,
-0.0111622673120118));
#25350=CARTESIAN_POINT('Ctrl Pts',(0.00497856419804905,-0.0373528018194475,
-0.0113769651953921));
#25351=CARTESIAN_POINT('Ctrl Pts',(0.00477692330866625,-0.0373824696566824,
-0.0118049823559411));
#25352=CARTESIAN_POINT('Ctrl Pts',(0.00473549949759476,-0.0373941167991429,
-0.0119907730648006));
#25353=CARTESIAN_POINT('Ctrl Pts',(0.00473550000000466,-0.0374057639416033,
-0.0121758567190455));
#25354=CARTESIAN_POINT('Origin',(0.006,-0.0412787743898723,-0.0121758532865581));
#25355=CARTESIAN_POINT('',(0.00473550017865996,-0.037905744212147,-0.0121763258579932));
#25356=CARTESIAN_POINT('',(0.00473550000001974,-0.0378432065283682,-0.0121758603510965));
#25357=CARTESIAN_POINT('',(0.0047355,-0.0412787743898723,-0.0121758532865581));
#25358=CARTESIAN_POINT('Ctrl Pts',(0.00473550000001974,-0.0378432065283682,
-0.0121758603510965));
#25359=CARTESIAN_POINT('Ctrl Pts',(0.00473549837272941,-0.0378248823123293,
-0.0118845874474744));
#25360=CARTESIAN_POINT('Ctrl Pts',(0.00484035109591382,-0.0378065586722709,
-0.0115938253847216));
#25361=CARTESIAN_POINT('Ctrl Pts',(0.00505105497354914,-0.0377857311838847,
-0.011339169850239));
#25362=CARTESIAN_POINT('Ctrl Pts',(0.00507778670136795,-0.0377832298915577,
-0.0113097962795975));
#25363=CARTESIAN_POINT('Ctrl Pts',(0.00530742653977762,-0.0377627394571817,
-0.011080133980301));
#25364=CARTESIAN_POINT('Ctrl Pts',(0.00558084995454937,-0.037744747444154,
-0.0109491016718024));
#25365=CARTESIAN_POINT('Ctrl Pts',(0.00590979445143813,-0.0377239227486984,
-0.0109137688503134));
#25366=CARTESIAN_POINT('Ctrl Pts',(0.00595486118160276,-0.0377210841223431,
-0.0109113574437742));
#25367=CARTESIAN_POINT('Ctrl Pts',(0.00628617625603332,-0.0377001962616308,
-0.0109113268906981));
#25368=CARTESIAN_POINT('Ctrl Pts',(0.00657310567735865,-0.0376821544149174,
-0.0110127817202872));
#25369=CARTESIAN_POINT('Ctrl Pts',(0.00683015446989156,-0.0376613110970863,
-0.0112210002627126));
#25370=CARTESIAN_POINT('Ctrl Pts',(0.00686291103859084,-0.037658534889714,
-0.0112504997221244));
#25371=CARTESIAN_POINT('Ctrl Pts',(0.00709653430797494,-0.0376376773949044,
-0.0114840596727804));
#25372=CARTESIAN_POINT('Ctrl Pts',(0.00722770261872788,-0.0376195658123854,
-0.0117587590126114));
#25373=CARTESIAN_POINT('Ctrl Pts',(0.00726219389305527,-0.0375987847351207,
-0.012087753553734));
#25374=CARTESIAN_POINT('Ctrl Pts',(0.00726449212525363,-0.0375960237122921,
-0.0121317099105978));
#25375=CARTESIAN_POINT('Ctrl Pts',(0.00726455115590598,-0.0375752932001571,
-0.0124617697191545));
#25376=CARTESIAN_POINT('Ctrl Pts',(0.00716322204369515,-0.0375574337462205,
-0.0127485930585501));
#25377=CARTESIAN_POINT('Ctrl Pts',(0.00695507757776487,-0.0375367589298144,
-0.0130057581485678));
#25378=CARTESIAN_POINT('Ctrl Pts',(0.00692547434391714,-0.0375339946126188,
-0.0130386431468708));
#25379=CARTESIAN_POINT('Ctrl Pts',(0.00669183782908888,-0.0375132881525957,
-0.0132723457410711));
#25380=CARTESIAN_POINT('Ctrl Pts',(0.0064171989090472,-0.0374952700466619,
-0.0134035071006325));
#25381=CARTESIAN_POINT('Ctrl Pts',(0.00608817313528417,-0.037474443859945,
-0.0134380452873456));
#25382=CARTESIAN_POINT('Ctrl Pts',(0.00604412422547741,-0.0374716683136219,
-0.0134403492751711));
#25383=CARTESIAN_POINT('Ctrl Pts',(0.005714859243909,-0.0374508977033079,
-0.0134403792481463));
#25384=CARTESIAN_POINT('Ctrl Pts',(0.00542886542456276,-0.0374328769759303,
-0.0133396240874224));
#25385=CARTESIAN_POINT('Ctrl Pts',(0.00517133362640543,-0.0374119654032364,
-0.0131320479206591));
#25386=CARTESIAN_POINT('Ctrl Pts',(0.00513774826390097,-0.0374091118927495,
-0.013101872008473));
#25387=CARTESIAN_POINT('Ctrl Pts',(0.00490049177048049,-0.0373878470509977,
-0.0128646348103454));
#25388=CARTESIAN_POINT('Ctrl Pts',(0.00476861571028705,-0.037369395015102,
-0.0125852190580139));
#25389=CARTESIAN_POINT('Ctrl Pts',(0.00473737972636936,-0.037348379083743,
-0.012255451925681));
#25390=CARTESIAN_POINT('Ctrl Pts',(0.00473549961401352,-0.0373458519661643,
-0.0122156399924958));
#25391=CARTESIAN_POINT('Ctrl Pts',(0.00473550000005949,-0.0373433241596449,
-0.0121758410210368));
#25392=CARTESIAN_POINT('Ctrl Pts',(0.00473550001147425,-0.0374057743898623,
-0.0121760236343295));
#25393=CARTESIAN_POINT('Ctrl Pts',(0.0047355392500951,-0.0374241027916517,
-0.0124672938705479));
#25394=CARTESIAN_POINT('Ctrl Pts',(0.00484043094080772,-0.0374424311934411,
-0.0127580388597337));
#25395=CARTESIAN_POINT('Ctrl Pts',(0.0050258589565221,-0.0374607595952306,
-0.0129820849390078));
#25396=CARTESIAN_POINT('Ctrl Pts',(0.00505117584857121,-0.0374632620119649,
-0.0130126744396351));
#25397=CARTESIAN_POINT('Ctrl Pts',(0.00507792113320851,-0.0374657644286992,
-0.0130420540382709));
#25398=CARTESIAN_POINT('Ctrl Pts',(0.00510596839668437,-0.0374682668454335,
-0.0130700947205528));
#25399=CARTESIAN_POINT('Ctrl Pts',(0.00530760914168099,-0.0374862575194625,
-0.0132716881512416));
#25400=CARTESIAN_POINT('Ctrl Pts',(0.00558105531573703,-0.0375042481934915,
-0.0134026753626389));
#25401=CARTESIAN_POINT('Ctrl Pts',(0.00586516527539268,-0.0375222388675206,
-0.0134331439637844));
#25402=CARTESIAN_POINT('Ctrl Pts',(0.00591001703228126,-0.0375250790120153,
-0.0134379539686605));
#25403=CARTESIAN_POINT('Ctrl Pts',(0.0059550942114837,-0.03752791915651,
-0.0134403577815941));
#25404=CARTESIAN_POINT('Ctrl Pts',(0.00600012639762061,-0.0375307593010047,
-0.0134403532802408));
#25405=CARTESIAN_POINT('Ctrl Pts',(0.00628643439849026,-0.0375488165210115,
-0.0134403246613003));
#25406=CARTESIAN_POINT('Ctrl Pts',(0.00657335761958725,-0.0375668737410184,
-0.0133388044586746));
#25407=CARTESIAN_POINT('Ctrl Pts',(0.00679614752363937,-0.0375849309610252,
-0.0131582530883714));
#25408=CARTESIAN_POINT('Ctrl Pts',(0.0068303681704066,-0.0375877045595421,
-0.0131305203026657));
#25409=CARTESIAN_POINT('Ctrl Pts',(0.00686311541701947,-0.0375904781580589,
-0.0131010160491334));
#25410=CARTESIAN_POINT('Ctrl Pts',(0.00689421035965139,-0.0375932517565758,
-0.01306991597043));
#25411=CARTESIAN_POINT('Ctrl Pts',(0.00709661267960903,-0.0376113055854924,
-0.012867480218901));
#25412=CARTESIAN_POINT('Ctrl Pts',(0.0072277038809594,-0.0376293594144089,
-0.0125928676077469));
#25413=CARTESIAN_POINT('Ctrl Pts',(0.00725760438561427,-0.0376474132433254,
-0.0123077299686658));
#25414=CARTESIAN_POINT('Ctrl Pts',(0.00726220359784015,-0.0376501902329326,
-0.012263870892344));
#25415=CARTESIAN_POINT('Ctrl Pts',(0.0072645028681267,-0.0376529672225398,
-0.0122198006318683));
#25416=CARTESIAN_POINT('Ctrl Pts',(0.00726449999731215,-0.037655744212147,
-0.0121757708390885));
#25417=CARTESIAN_POINT('Ctrl Pts',(0.0072644813335063,-0.0376737980410633,
-0.0118895233342346));
#25418=CARTESIAN_POINT('Ctrl Pts',(0.00716301179804758,-0.0376918518699797,
-0.0116026446414172));
#25419=CARTESIAN_POINT('Ctrl Pts',(0.00698252940739209,-0.037709905698896,
-0.0113798657152922));
#25420=CARTESIAN_POINT('Ctrl Pts',(0.00695476810947077,-0.0377126826885034,
-0.0113455984822603));
#25421=CARTESIAN_POINT('Ctrl Pts',(0.00692523078390005,-0.0377154596781108,
-0.0113128080448829));
#25422=CARTESIAN_POINT('Ctrl Pts',(0.006894093763348,-0.0377182366677182,
-0.0112816740023303));
#25423=CARTESIAN_POINT('Ctrl Pts',(0.0066916270241954,-0.0377362938877251,
-0.0110792266274528));
#25424=CARTESIAN_POINT('Ctrl Pts',(0.00641695897599585,-0.0377543511077321,
-0.0109481173224277));
#25425=CARTESIAN_POINT('Ctrl Pts',(0.00613176203582361,-0.037772408327739,
-0.0109182368840269));
#25426=CARTESIAN_POINT('Ctrl Pts',(0.00608795563539476,-0.0377751819262558,
-0.010913647232929));
#25427=CARTESIAN_POINT('Ctrl Pts',(0.00604393856281892,-0.0377779555247726,
-0.0109113519482759));
#25428=CARTESIAN_POINT('Ctrl Pts',(0.00599996150268144,-0.0377807291232894,
-0.0109113532871441));
#25429=CARTESIAN_POINT('Ctrl Pts',(0.00571470862671654,-0.0377987197973184,
-0.0109113619715813));
#25430=CARTESIAN_POINT('Ctrl Pts',(0.0054287293523573,-0.0378167104713474,
-0.0110121498534471));
#25431=CARTESIAN_POINT('Ctrl Pts',(0.00520635007387457,-0.0378347011453764,
-0.0111914346536782));
#25432=CARTESIAN_POINT('Ctrl Pts',(0.00517124359134334,-0.0378375412898711,
-0.0112197379144423));
#25433=CARTESIAN_POINT('Ctrl Pts',(0.00513768018197624,-0.0378403814343658,
-0.011249899223349));
#25434=CARTESIAN_POINT('Ctrl Pts',(0.00510585179227583,-0.0378432215788605,
-0.0112817284448141));
#25435=CARTESIAN_POINT('Ctrl Pts',(0.00490045255438429,-0.0378615499806493,
-0.0114871330503616));
#25436=CARTESIAN_POINT('Ctrl Pts',(0.00476859134920546,-0.0378798783824381,
-0.0117665590362431));
#25437=CARTESIAN_POINT('Ctrl Pts',(0.00474112757943725,-0.0378982067842269,
-0.0120566875249212));
#25438=CARTESIAN_POINT('Ctrl Pts',(0.00473737789095569,-0.0379007092009618,
-0.0120962994012715));
#25439=CARTESIAN_POINT('Ctrl Pts',(0.00473550017150005,-0.0379032116176968,
-0.0121360800717304));
#25440=CARTESIAN_POINT('Ctrl Pts',(0.00473550000001176,-0.0379057140344317,
-0.0121758478337256));
#25441=CARTESIAN_POINT('Origin',(0.006,-0.0412787743898723,-0.0121758532865581));
#25442=CARTESIAN_POINT('',(0.00473550020721395,-0.0384058072487128,-0.0121753454415193));
#25443=CARTESIAN_POINT('',(0.0047355000350514,-0.0383440997603813,-0.0121756391001055));
#25444=CARTESIAN_POINT('',(0.0047355,-0.0412787743898723,-0.0121758532865581));
#25445=CARTESIAN_POINT('Ctrl Pts',(0.00473550006772914,-0.0383440997603812,
-0.0121754394182212));
#25446=CARTESIAN_POINT('Ctrl Pts',(0.00473550974249037,-0.0383423607576411,
-0.0121458799331841));
#25447=CARTESIAN_POINT('Ctrl Pts',(0.0047365559087295,-0.0383405947365542,
-0.0121163319997317));
#25448=CARTESIAN_POINT('Ctrl Pts',(0.0047392614796249,-0.0383382365720843,
-0.0120779882914245));
#25449=CARTESIAN_POINT('Ctrl Pts',(0.00473998013712677,-0.038337687364268,
-0.0120691335163025));
#25450=CARTESIAN_POINT('Ctrl Pts',(0.00474148006416988,-0.0383366639294188,
-0.0120527902944031));
#25451=CARTESIAN_POINT('Ctrl Pts',(0.0047422350368259,-0.0383361910629747,
-0.0120452997736119));
#25452=CARTESIAN_POINT('Ctrl Pts',(0.00474401518407334,-0.0383351586666519,
-0.0120290899894216));
#25453=CARTESIAN_POINT('Ctrl Pts',(0.0047450643631106,-0.038334597825695,
-0.0120203738351233));
#25454=CARTESIAN_POINT('Ctrl Pts',(0.00474813704008429,-0.0383330738420285,
-0.0119969092018068));
#25455=CARTESIAN_POINT('Ctrl Pts',(0.00475033031362653,-0.038332102409206,
-0.0119821847900106));
#25456=CARTESIAN_POINT('Ctrl Pts',(0.00476526810161275,-0.0383261241576951,
-0.0118927647516049));
#25457=CARTESIAN_POINT('Ctrl Pts',(0.00478444511683913,-0.0383208866749639,
-0.0118193046409008));
#25458=CARTESIAN_POINT('Ctrl Pts',(0.00483464073841951,-0.0383107214526994,
-0.0116797009722359));
#25459=CARTESIAN_POINT('Ctrl Pts',(0.00486504012193256,-0.0383058093371502,
-0.0116136272923258));
#25460=CARTESIAN_POINT('Ctrl Pts',(0.00491177218601365,-0.0382996515186367,
-0.0115314933720116));
#25461=CARTESIAN_POINT('Ctrl Pts',(0.00492309079993836,-0.0382982414926402,
-0.0115127498675848));
#25462=CARTESIAN_POINT('Ctrl Pts',(0.00494291424779926,-0.038295901457145,
-0.0114817700391427));
#25463=CARTESIAN_POINT('Ctrl Pts',(0.00495115857748836,-0.0382949624196954,
-0.0114693736037016));
#25464=CARTESIAN_POINT('Ctrl Pts',(0.00496724732943143,-0.0382931920156278,
-0.0114460846667635));
#25465=CARTESIAN_POINT('Ctrl Pts',(0.00497504996397839,-0.0382923592752213,
-0.011435165928765));
#25466=CARTESIAN_POINT('Ctrl Pts',(0.0049961039371682,-0.0382901774441414,
-0.0114066736782037));
#25467=CARTESIAN_POINT('Ctrl Pts',(0.00500964307591435,-0.0382888393892673,
-0.0113893179574066));
#25468=CARTESIAN_POINT('Ctrl Pts',(0.00508173465858396,-0.0382820198826257,
-0.0113017192787193));
#25469=CARTESIAN_POINT('Ctrl Pts',(0.00514732679862287,-0.0382768286806568,
-0.0112376254943765));
#25470=CARTESIAN_POINT('Ctrl Pts',(0.00526278284619604,-0.0382683952347556,
-0.0111470034271226));
#25471=CARTESIAN_POINT('Ctrl Pts',(0.00530849448079938,-0.0382651956540521,
-0.0111157400209426));
#25472=CARTESIAN_POINT('Ctrl Pts',(0.00536956440240138,-0.0382609043601922,
-0.0110796069977995));
#25473=CARTESIAN_POINT('Ctrl Pts',(0.00538317380505029,-0.0382599469161624,
-0.0110718920716276));
#25474=CARTESIAN_POINT('Ctrl Pts',(0.00540477383212506,-0.0382584200137224,
-0.0110601714948468));
#25475=CARTESIAN_POINT('Ctrl Pts',(0.00541267020758086,-0.0382578603180602,
-0.0110559944761936));
#25476=CARTESIAN_POINT('Ctrl Pts',(0.00542827956076714,-0.038256749689617,
-0.0110479479516441));
#25477=CARTESIAN_POINT('Ctrl Pts',(0.00543598913283541,-0.0382561990914316,
-0.0110440730811823));
#25478=CARTESIAN_POINT('Ctrl Pts',(0.0054564351153719,-0.038254734657851,
-0.0110340576016111));
#25479=CARTESIAN_POINT('Ctrl Pts',(0.00546923565599044,-0.0382538135520933,
-0.0110280513251737));
#25480=CARTESIAN_POINT('Ctrl Pts',(0.00555449518481482,-0.0382476629121317,
-0.0109897769218209));
#25481=CARTESIAN_POINT('Ctrl Pts',(0.00562974789262337,-0.0382421731018808,
-0.0109641752842107));
#25482=CARTESIAN_POINT('Ctrl Pts',(0.00576761905774788,-0.0382324667285227,
-0.0109313229128065));
#25483=CARTESIAN_POINT('Ctrl Pts',(0.0058293348778137,-0.0382282386702702,
-0.0109213686212666));
#25484=CARTESIAN_POINT('Ctrl Pts',(0.00591736723567329,-0.0382224340613599,
-0.0109137898627642));
#25485=CARTESIAN_POINT('Ctrl Pts',(0.00594325847525168,-0.0382207532952864,
-0.010912360977878));
#25486=CARTESIAN_POINT('Ctrl Pts',(0.00598479543743047,-0.0382180978577547,
-0.0109113481838971));
#25487=CARTESIAN_POINT('Ctrl Pts',(0.00600042020489185,-0.0382171082066521,
-0.010911256832504));
#25488=CARTESIAN_POINT('Ctrl Pts',(0.00603068216275742,-0.0382152081904866,
-0.0109116408092541));
#25489=CARTESIAN_POINT('Ctrl Pts',(0.00604531721747602,-0.0382142969023267,
-0.0109120807751475));
#25490=CARTESIAN_POINT('Ctrl Pts',(0.00608030479958005,-0.0382121347055097,
-0.0109137411783001));
#25491=CARTESIAN_POINT('Ctrl Pts',(0.00610064221660877,-0.0382108912020008,
-0.0109151998652492));
#25492=CARTESIAN_POINT('Ctrl Pts',(0.00622350986786219,-0.0382034428226632,
-0.0109270050015834));
#25493=CARTESIAN_POINT('Ctrl Pts',(0.00632449174572357,-0.0381976321744983,
-0.0109493602552273));
#25494=CARTESIAN_POINT('Ctrl Pts',(0.00647115471914298,-0.0381886661499864,
-0.0110012336919901));
#25495=CARTESIAN_POINT('Ctrl Pts',(0.00651951942254762,-0.038185606567173,
-0.0110218097854021));
#25496=CARTESIAN_POINT('Ctrl Pts',(0.00657804445378298,-0.0381816149945491,
-0.0110511343181702));
#25497=CARTESIAN_POINT('Ctrl Pts',(0.00658953871713479,-0.0381808164229959,
-0.011057116400786));
#25498=CARTESIAN_POINT('Ctrl Pts',(0.00660833675089142,-0.0381794827906792,
-0.0110672697986541));
#25499=CARTESIAN_POINT('Ctrl Pts',(0.00661569478902127,-0.0381789536344057,
-0.0110713394226018));
#25500=CARTESIAN_POINT('Ctrl Pts',(0.00663110056833495,-0.0381778296042569,
-0.0110800619162578));
#25501=CARTESIAN_POINT('Ctrl Pts',(0.0066391384222595,-0.0381772338804882,
-0.0110847305989748));
#25502=CARTESIAN_POINT('Ctrl Pts',(0.00666213560290017,-0.0381755041835899,
-0.0110984295021851));
#25503=CARTESIAN_POINT('Ctrl Pts',(0.00667695964437776,-0.038174358022301,
-0.0111076814185698));
#25504=CARTESIAN_POINT('Ctrl Pts',(0.0067575427830394,-0.0381679729112217,
-0.0111603257992692));
#25505=CARTESIAN_POINT('Ctrl Pts',(0.00681932475879082,-0.0381625114775893,
-0.0112094821687601));
#25506=CARTESIAN_POINT('Ctrl Pts',(0.00692183586976768,-0.0381527912051747,
-0.0113079840958977));
#25507=CARTESIAN_POINT('Ctrl Pts',(0.00696418053016676,-0.0381485170987116,
-0.0113552827441237));
#25508=CARTESIAN_POINT('Ctrl Pts',(0.00701662100396916,-0.0381428976974481,
-0.0114235524685112));
#25509=CARTESIAN_POINT('Ctrl Pts',(0.00702995305424856,-0.0381414345659435,
-0.0114419107834808));
#25510=CARTESIAN_POINT('Ctrl Pts',(0.00705128360070422,-0.0381390328086286,
-0.0114730099104666));
#25511=CARTESIAN_POINT('Ctrl Pts',(0.00705956124976711,-0.038138084062126,
-0.011485551896358));
#25512=CARTESIAN_POINT('Ctrl Pts',(0.00707567633395429,-0.038136201534902,
-0.0115109419770585));
#25513=CARTESIAN_POINT('Ctrl Pts',(0.00708351187440794,-0.0381352679290252,
-0.011523788356514));
#25514=CARTESIAN_POINT('Ctrl Pts',(0.00710263741586795,-0.03813293968717,
-0.0115564417823842));
#25515=CARTESIAN_POINT('Ctrl Pts',(0.00711362477632549,-0.0381315557282313,
-0.0115764203587779));
#25516=CARTESIAN_POINT('Ctrl Pts',(0.00715127971672568,-0.0381266224545275,
-0.0116495022831765));
#25517=CARTESIAN_POINT('Ctrl Pts',(0.0071747378912722,-0.0381231760691956,
-0.0117041731249888));
#25518=CARTESIAN_POINT('Ctrl Pts',(0.00721098982627317,-0.0381168355051107,
-0.0118083570121928));
#25519=CARTESIAN_POINT('Ctrl Pts',(0.00722479651110265,-0.0381139377163221,
-0.0118573832955558));
#25520=CARTESIAN_POINT('Ctrl Pts',(0.00724436401760256,-0.0381085898082324,
-0.0119473484721064));
#25521=CARTESIAN_POINT('Ctrl Pts',(0.00725114472730231,-0.0381061622998086,
-0.0119879902752478));
#25522=CARTESIAN_POINT('Ctrl Pts',(0.00725736262231289,-0.0381028927799663,
-0.0120411263227455));
#25523=CARTESIAN_POINT('Ctrl Pts',(0.00725861585636101,-0.0381021318306581,
-0.0120533860711974));
#25524=CARTESIAN_POINT('Ctrl Pts',(0.00726041354233924,-0.038100842347413,
-0.0120739368713227));
#25525=CARTESIAN_POINT('Ctrl Pts',(0.00726105581173342,-0.0381003188980919,
-0.0120822184105377));
#25526=CARTESIAN_POINT('Ctrl Pts',(0.00726226173103871,-0.0380991831231867,
-0.0121000445148492));
#25527=CARTESIAN_POINT('Ctrl Pts',(0.00726279877888703,-0.0380985695742431,
-0.0121095895847459));
#25528=CARTESIAN_POINT('Ctrl Pts',(0.00726407406333585,-0.0380967294633223,
-0.0121379949103421));
#25529=CARTESIAN_POINT('Ctrl Pts',(0.00726449827568978,-0.0380954883598766,
-0.0121568658637334));
#25530=CARTESIAN_POINT('Ctrl Pts',(0.00726450241961066,-0.0380924622964117,
-0.0122023563976265));
#25531=CARTESIAN_POINT('Ctrl Pts',(0.00726366435025537,-0.0380906639756224,
-0.012228966828908));
#25532=CARTESIAN_POINT('Ctrl Pts',(0.00725534795666524,-0.0380816772887418,
-0.0123606897285524));
#25533=CARTESIAN_POINT('Ctrl Pts',(0.0072355882239628,-0.0380743637674893,
-0.0124646279259903));
#25534=CARTESIAN_POINT('Ctrl Pts',(0.00719490893095668,-0.0380656643001295,
-0.0125904277038998));
#25535=CARTESIAN_POINT('Ctrl Pts',(0.00718584853738683,-0.0380639234751518,
-0.0126156745212516));
#25536=CARTESIAN_POINT('Ctrl Pts',(0.00717018845937666,-0.0380611981985746,
-0.0126552993258125));
#25537=CARTESIAN_POINT('Ctrl Pts',(0.00716411065595122,-0.0380601973130519,
-0.0126698734801178));
#25538=CARTESIAN_POINT('Ctrl Pts',(0.00715190090495607,-0.0380582898184641,
-0.0126976740887945));
#25539=CARTESIAN_POINT('Ctrl Pts',(0.00714581012024887,-0.0380573820285958,
-0.0127109157505791));
#25540=CARTESIAN_POINT('Ctrl Pts',(0.00713085035341409,-0.0380552503813735,
-0.0127420114142857));
#25541=CARTESIAN_POINT('Ctrl Pts',(0.00712178531407539,-0.0380540333452085,
-0.0127597670833557));
#25542=CARTESIAN_POINT('Ctrl Pts',(0.0070840275256758,-0.0380492375398036,
-0.0128295953985292));
#25543=CARTESIAN_POINT('Ctrl Pts',(0.00705209723552133,-0.0380457700394852,
-0.012879832606127));
#25544=CARTESIAN_POINT('Ctrl Pts',(0.00696865375690912,-0.0380376844199474,
-0.0129926849066957));
#25545=CARTESIAN_POINT('Ctrl Pts',(0.00691443349667901,-0.0380331248422485,
-0.0130529583829421));
#25546=CARTESIAN_POINT('Ctrl Pts',(0.00683812656162111,-0.0380269613655469,
-0.0131229637345937));
#25547=CARTESIAN_POINT('Ctrl Pts',(0.00682101083459093,-0.038025592243267,
-0.0131378384270219));
#25548=CARTESIAN_POINT('Ctrl Pts',(0.00679561599377313,-0.0380235642963763,
-0.0131587367196268));
#25549=CARTESIAN_POINT('Ctrl Pts',(0.0067876481868241,-0.0380229284805302,
-0.0131651333129319));
#25550=CARTESIAN_POINT('Ctrl Pts',(0.00677380894466891,-0.0380218232281778,
-0.0131759703513498));
#25551=CARTESIAN_POINT('Ctrl Pts',(0.00676797479343403,-0.038021356932129,
-0.0131804572558482));
#25552=CARTESIAN_POINT('Ctrl Pts',(0.0067535870498199,-0.0380202061219728,
-0.0131913239486484));
#25553=CARTESIAN_POINT('Ctrl Pts',(0.00674499161463305,-0.0380195180268725,
-0.0131976466039016));
#25554=CARTESIAN_POINT('Ctrl Pts',(0.0067154723950112,-0.0380171557553199,
-0.0132187899779236));
#25555=CARTESIAN_POINT('Ctrl Pts',(0.00669417936215945,-0.03801545329348,
-0.0132330819832831));
#25556=CARTESIAN_POINT('Ctrl Pts',(0.00663635987492588,-0.0380108629301987,
-0.0132693908165886));
#25557=CARTESIAN_POINT('Ctrl Pts',(0.00659912921382913,-0.0380079410605348,
-0.013290224005341));
#25558=CARTESIAN_POINT('Ctrl Pts',(0.00648213702032248,-0.037998983091039,
-0.0133481293932859));
#25559=CARTESIAN_POINT('Ctrl Pts',(0.00639949154536015,-0.0379929775869118,
-0.0133788072659486));
#25560=CARTESIAN_POINT('Ctrl Pts',(0.00629260407273725,-0.0379857782761919,
-0.0134062377196916));
#25561=CARTESIAN_POINT('Ctrl Pts',(0.00627074040808769,-0.0379843326697674,
-0.0134112328759312));
#25562=CARTESIAN_POINT('Ctrl Pts',(0.006235533100476,-0.0379820464431884,
-0.0134182969456217));
#25563=CARTESIAN_POINT('Ctrl Pts',(0.0062222699173018,-0.0379811945105474,
-0.0134207380979277));
#25564=CARTESIAN_POINT('Ctrl Pts',(0.00619435538463652,-0.0379794201362291,
-0.0134254155348955));
#25565=CARTESIAN_POINT('Ctrl Pts',(0.00617969859685401,-0.0379784991908188,
-0.0134276073642931));
#25566=CARTESIAN_POINT('Ctrl Pts',(0.00614369541127588,-0.0379762612079752,
-0.0134323459822949));
#25567=CARTESIAN_POINT('Ctrl Pts',(0.00612231574497327,-0.0379749530432353,
-0.0134346071167305));
#25568=CARTESIAN_POINT('Ctrl Pts',(0.00602535041493018,-0.0379690988733585,
-0.013442368215006));
#25569=CARTESIAN_POINT('Ctrl Pts',(0.00594942007337511,-0.0379647422498225,
-0.013441612294665));
#25570=CARTESIAN_POINT('Ctrl Pts',(0.00580057708008604,-0.0379561647576001,
-0.0134267077843195));
#25571=CARTESIAN_POINT('Ctrl Pts',(0.00572793841787632,-0.0379519561222335,
-0.0134129412246025));
#25572=CARTESIAN_POINT('Ctrl Pts',(0.00564277182284718,-0.0379465904651118,
-0.0133889338560403));
#25573=CARTESIAN_POINT('Ctrl Pts',(0.00562869131434428,-0.0379456885315878,
-0.0133846982959242));
#25574=CARTESIAN_POINT('Ctrl Pts',(0.00560636246622745,-0.0379442297987636,
-0.0133775546476917));
#25575=CARTESIAN_POINT('Ctrl Pts',(0.00559806448833046,-0.0379436813524884,
-0.0133748047051537));
#25576=CARTESIAN_POINT('Ctrl Pts',(0.00558146889480631,-0.0379425704680611,
-0.0133691132997638));
#25577=CARTESIAN_POINT('Ctrl Pts',(0.00557317217116028,-0.0379420080029346,
-0.0133661707815615));
#25578=CARTESIAN_POINT('Ctrl Pts',(0.00555082134023114,-0.0379404747815161,
-0.0133579801140248));
#25579=CARTESIAN_POINT('Ctrl Pts',(0.00553682920953142,-0.0379394955745321,
-0.0133525682385566));
#25580=CARTESIAN_POINT('Ctrl Pts',(0.00547690766188492,-0.0379352277019553,
-0.013328157504644));
#25581=CARTESIAN_POINT('Ctrl Pts',(0.00543202702965478,-0.0379318420215861,
-0.0133067098344694));
#25582=CARTESIAN_POINT('Ctrl Pts',(0.00529989308609221,-0.0379214964607171,
-0.013233711800486));
#25583=CARTESIAN_POINT('Ctrl Pts',(0.00521744341414155,-0.0379145436881024,
-0.0131742651574567));
#25584=CARTESIAN_POINT('Ctrl Pts',(0.00512778334700654,-0.0379066208031836,
-0.013091617761053));
#25585=CARTESIAN_POINT('Ctrl Pts',(0.00511294791782444,-0.0379052942548962,
-0.0130772550537105));
#25586=CARTESIAN_POINT('Ctrl Pts',(0.00508827772630164,-0.0379030597615259,
-0.0130521717353925));
#25587=CARTESIAN_POINT('Ctrl Pts',(0.00507826445866174,-0.0379021442860712,
-0.0130416333670979));
#25588=CARTESIAN_POINT('Ctrl Pts',(0.00505795325030473,-0.0379002682191274,
-0.0130195051294584));
#25589=CARTESIAN_POINT('Ctrl Pts',(0.00504768223712076,-0.0378993088280312,
-0.0130078938034488));
#25590=CARTESIAN_POINT('Ctrl Pts',(0.00502124101069876,-0.0378968077630075,
-0.0129768708898569));
#25591=CARTESIAN_POINT('Ctrl Pts',(0.00500543411081777,-0.0378952804617343,
-0.0129571580784358));
#25592=CARTESIAN_POINT('Ctrl Pts',(0.00494841777285435,-0.0378896245345087,
-0.0128815159692503));
#25593=CARTESIAN_POINT('Ctrl Pts',(0.00491124810562928,-0.0378856370318531,
-0.0128226959007852));
#25594=CARTESIAN_POINT('Ctrl Pts',(0.00484562476919585,-0.0378775073953288,
-0.0126970131589097));
#25595=CARTESIAN_POINT('Ctrl Pts',(0.00481771841867601,-0.0378733786250769,
-0.0126301634951455));
#25596=CARTESIAN_POINT('Ctrl Pts',(0.00479117410996577,-0.0378680993773812,
-0.012547227339326));
#25597=CARTESIAN_POINT('Ctrl Pts',(0.004786915965074,-0.0378671928717547,
-0.0125330728285829));
#25598=CARTESIAN_POINT('Ctrl Pts',(0.00478053159706622,-0.0378657285249005,
-0.0125104183186729));
#25599=CARTESIAN_POINT('Ctrl Pts',(0.00477824380512941,-0.0378651791502191,
-0.0125019648266605));
#25600=CARTESIAN_POINT('Ctrl Pts',(0.00477383729648801,-0.0378640685188387,
-0.0124849850602577));
#25601=CARTESIAN_POINT('Ctrl Pts',(0.00477171926747377,-0.0378635072661903,
-0.0124764591088708));
#25602=CARTESIAN_POINT('Ctrl Pts',(0.00476624464236355,-0.0378619807567758,
-0.0124533970255423));
#25603=CARTESIAN_POINT('Ctrl Pts',(0.00476305627478935,-0.0378610071639272,
-0.012438822839294));
#25604=CARTESIAN_POINT('Ctrl Pts',(0.00474377988958161,-0.0378545343673484,
-0.0123425839117136));
#25605=CARTESIAN_POINT('Ctrl Pts',(0.0047355318393687,-0.0378487591530695,
-0.012259561528838));
#25606=CARTESIAN_POINT('Ctrl Pts',(0.00473550009199991,-0.0378430687134126,
-0.0121763356430332));
#25607=CARTESIAN_POINT('Ctrl Pts',(0.00473550035730815,-0.0379057743898623,
-0.0121768038822607));
#25608=CARTESIAN_POINT('Ctrl Pts',(0.00473571932336438,-0.0379241093214222,
-0.0124680765012176));
#25609=CARTESIAN_POINT('Ctrl Pts',(0.00484079203787322,-0.037942444252982,
-0.0127587586814847));
#25610=CARTESIAN_POINT('Ctrl Pts',(0.00502636095174794,-0.0379607791845419,
-0.0129826910978429));
#25611=CARTESIAN_POINT('Ctrl Pts',(0.00505164742211236,-0.0379632775863154,
-0.0130132051548131));
#25612=CARTESIAN_POINT('Ctrl Pts',(0.00507835596367472,-0.0379657759880888,
-0.0130425131526919));
#25613=CARTESIAN_POINT('Ctrl Pts',(0.00510636083680849,-0.0379682743898623,
-0.0130704868964847));
#25614=CARTESIAN_POINT('Ctrl Pts',(0.00530809385253593,-0.0379862716191963,
-0.0132719956721024));
#25615=CARTESIAN_POINT('Ctrl Pts',(0.00558160283114279,-0.0380042688485303,
-0.0134028631907799));
#25616=CARTESIAN_POINT('Ctrl Pts',(0.00586573071169492,-0.0380222660778642,
-0.0134332044738634));
#25617=CARTESIAN_POINT('Ctrl Pts',(0.00591050517133018,-0.0380251021818636,
-0.0134379858228534));
#25618=CARTESIAN_POINT('Ctrl Pts',(0.00595550318120118,-0.0380279382858629,
-0.0134403694067042));
#25619=CARTESIAN_POINT('Ctrl Pts',(0.00600045576433034,-0.0380307743898623,
-0.0134403532044224));
#25620=CARTESIAN_POINT('Ctrl Pts',(0.00628676884007308,-0.0380488381718,
-0.013440250008459));
#25621=CARTESIAN_POINT('Ctrl Pts',(0.00657366937610735,-0.0380669019537376,
-0.0133386517033703));
#25622=CARTESIAN_POINT('Ctrl Pts',(0.00679641352477234,-0.0380849657356753,
-0.0131580374584728));
#25623=CARTESIAN_POINT('Ctrl Pts',(0.00683056480992067,-0.038087735287071,
-0.0131303455589714));
#25624=CARTESIAN_POINT('Ctrl Pts',(0.00686324754914644,-0.0380905048384666,
-0.0131008889919923));
#25625=CARTESIAN_POINT('Ctrl Pts',(0.00689428383739052,-0.0380932743898623,
-0.013069842474514));
#25626=CARTESIAN_POINT('Ctrl Pts',(0.00709667301988905,-0.0381113347725488,
-0.0128673865866694));
#25627=CARTESIAN_POINT('Ctrl Pts',(0.00722774192794643,-0.0381293951552352,
-0.0125927582940303));
#25628=CARTESIAN_POINT('Ctrl Pts',(0.00725761654397931,-0.0381474555379217,
-0.012307613972309));
#25629=CARTESIAN_POINT('Ctrl Pts',(0.00726220342551396,-0.0381502284885686,
-0.0122638335527523));
#25630=CARTESIAN_POINT('Ctrl Pts',(0.0072644986415305,-0.0381530014392154,
-0.0122198429168089));
#25631=CARTESIAN_POINT('Ctrl Pts',(0.00726449999939651,-0.0381557743898623,
-0.0121758923536699));
#25632=CARTESIAN_POINT('Ctrl Pts',(0.00726450884325376,-0.0381738347725488,
-0.0118896398772787));
#25633=CARTESIAN_POINT('Ctrl Pts',(0.00716306358962789,-0.0381918951552352,
-0.0116027477647218));
#25634=CARTESIAN_POINT('Ctrl Pts',(0.00698259788633582,-0.0382099555379217,
-0.0113799502498957));
#25635=CARTESIAN_POINT('Ctrl Pts',(0.00695488958705057,-0.0382127284885686,
-0.011345742419221));
#25636=CARTESIAN_POINT('Ctrl Pts',(0.00692541153612805,-0.0382155014392154,
-0.011313005901592));
#25637=CARTESIAN_POINT('Ctrl Pts',(0.00689433907581853,-0.0382182743898623,
-0.0112819193586506));
#25638=CARTESIAN_POINT('Ctrl Pts',(0.00669192431307087,-0.0382363381718,
-0.0110794128576707));
#25639=CARTESIAN_POINT('Ctrl Pts',(0.00641728721568636,-0.0382544019537377,
-0.0109482278968322));
#25640=CARTESIAN_POINT('Ctrl Pts',(0.00613209413111397,-0.0382724657356753,
-0.0109182717223941));
#25641=CARTESIAN_POINT('Ctrl Pts',(0.00608836813242027,-0.038275235287071,
-0.0109136788212502));
#25642=CARTESIAN_POINT('Ctrl Pts',(0.00604443161399198,-0.0382780048384666,
-0.0109113719338119));
#25643=CARTESIAN_POINT('Ctrl Pts',(0.00600053389854783,-0.0382807743898623,
-0.0109113533992697));
#25644=CARTESIAN_POINT('Ctrl Pts',(0.00571527569632501,-0.0382987716191963,
-0.0109112329572345));
#25645=CARTESIAN_POINT('Ctrl Pts',(0.00542924685311941,-0.0383167688485304,
-0.0110118949021592));
#25646=CARTESIAN_POINT('Ctrl Pts',(0.00520678506047186,-0.0383347660778645,
-0.0111910841208602));
#25647=CARTESIAN_POINT('Ctrl Pts',(0.00517172828767079,-0.0383376021818637,
-0.011219321759574));
#25648=CARTESIAN_POINT('Ctrl Pts',(0.00513820829682603,-0.038340438285863,
-0.0112494115449752));
#25649=CARTESIAN_POINT('Ctrl Pts',(0.00510641611846888,-0.0383432743898623,
-0.0112811644598324));
#25650=CARTESIAN_POINT('Ctrl Pts',(0.00490088507501357,-0.0383616093214222,
-0.0114864416714168));
#25651=CARTESIAN_POINT('Ctrl Pts',(0.00476884759532968,-0.0383799442529821,
-0.0117657873933289));
#25652=CARTESIAN_POINT('Ctrl Pts',(0.00474120230281209,-0.038398279184542,
-0.0120559007644737));
#25653=CARTESIAN_POINT('Ctrl Pts',(0.00473743522860036,-0.0384007775863154,
-0.0120954329415422));
#25654=CARTESIAN_POINT('Ctrl Pts',(0.00473553270825591,-0.0384032759880889,
-0.012135134417089));
#25655=CARTESIAN_POINT('Ctrl Pts',(0.00473550041846002,-0.0384057743898623,
-0.012174824556656));
#25656=CARTESIAN_POINT('Origin',(0.006,-0.0412787743898723,-0.0121758532865581));
#25657=CARTESIAN_POINT('',(0.00473550000000009,-0.0389057758757622,-0.012175852808333));
#25658=CARTESIAN_POINT('',(0.0047355,-0.0388421555262979,-0.0121758532866954));
#25659=CARTESIAN_POINT('',(0.0047355,-0.0412787743898723,-0.0121758532865581));
#25660=CARTESIAN_POINT('Ctrl Pts',(0.0047355,-0.0388421555262979,-0.0121758532868327));
#25661=CARTESIAN_POINT('Ctrl Pts',(0.00473549999999784,-0.0388415399821669,
-0.0121659214854022));
#25662=CARTESIAN_POINT('Ctrl Pts',(0.00473561701135706,-0.0388409279571186,
-0.0121559896111397));
#25663=CARTESIAN_POINT('Ctrl Pts',(0.00473647966409911,-0.0388386844031961,
-0.0121193870295771));
#25664=CARTESIAN_POINT('Ctrl Pts',(0.00473795231692135,-0.0388370746953837,
-0.0120927396953085));
#25665=CARTESIAN_POINT('Ctrl Pts',(0.00474890807120219,-0.0388295530808997,
-0.011966925207738));
#25666=CARTESIAN_POINT('Ctrl Pts',(0.00476924275858377,-0.0388239662038009,
-0.0118690656231402));
#25667=CARTESIAN_POINT('Ctrl Pts',(0.0048147111782553,-0.0388156631344287,
-0.0117331810071438));
#25668=CARTESIAN_POINT('Ctrl Pts',(0.00483070807381028,-0.0388130966890162,
-0.0116925066000963));
#25669=CARTESIAN_POINT('Ctrl Pts',(0.00485405383383625,-0.0388096527575508,
-0.0116411286413657));
#25670=CARTESIAN_POINT('Ctrl Pts',(0.00485950769434488,-0.0388088658048069,
-0.0116295929694698));
#25671=CARTESIAN_POINT('Ctrl Pts',(0.00486881390676934,-0.0388075479586308,
-0.0116106561080116));
#25672=CARTESIAN_POINT('Ctrl Pts',(0.00487256677516668,-0.0388070227432049,
-0.0116032066689159));
#25673=CARTESIAN_POINT('Ctrl Pts',(0.00488073567539052,-0.0388058915850138,
-0.0115873830332447));
#25674=CARTESIAN_POINT('Ctrl Pts',(0.00488517243658042,-0.0388052845265961,
-0.0115790205141998));
#25675=CARTESIAN_POINT('Ctrl Pts',(0.00489838371634503,-0.0388034994482989,
-0.0115547809255278));
#25676=CARTESIAN_POINT('Ctrl Pts',(0.00490740618781849,-0.0388023081820033,
-0.0115390424823475));
#25677=CARTESIAN_POINT('Ctrl Pts',(0.00496020278593633,-0.038795510442991,
-0.0114513728159497));
#25678=CARTESIAN_POINT('Ctrl Pts',(0.00501073631349636,-0.0387896581593104,
-0.0113837630720211));
#25679=CARTESIAN_POINT('Ctrl Pts',(0.00510973743408634,-0.038779662886571,
-0.0112756967936718));
#25680=CARTESIAN_POINT('Ctrl Pts',(0.00515521074677647,-0.0387754799592953,
-0.0112328887650736));
#25681=CARTESIAN_POINT('Ctrl Pts',(0.00521942814439156,-0.0387701140558503,
-0.0111808257928679));
#25682=CARTESIAN_POINT('Ctrl Pts',(0.00523549907371174,-0.0387688111453847,
-0.0111684255995347));
#25683=CARTESIAN_POINT('Ctrl Pts',(0.00526372769663689,-0.0387665888654258,
-0.0111477093488344));
#25684=CARTESIAN_POINT('Ctrl Pts',(0.0052757445782097,-0.038765662667888,
-0.0111392091941519));
#25685=CARTESIAN_POINT('Ctrl Pts',(0.00530100112828759,-0.0387637554555407,
-0.0111219975620968));
#25686=CARTESIAN_POINT('Ctrl Pts',(0.00531426170359364,-0.0387627758460356,
-0.0111133212474295));
#25687=CARTESIAN_POINT('Ctrl Pts',(0.00535027879207148,-0.0387601699351522,
-0.0110907107018007));
#25688=CARTESIAN_POINT('Ctrl Pts',(0.00537331958859258,-0.0387585602274808,
-0.0110772433078822));
#25689=CARTESIAN_POINT('Ctrl Pts',(0.00548431338809092,-0.0387510386131901,
-0.0110169964038892));
#25690=CARTESIAN_POINT('Ctrl Pts',(0.00557716023196362,-0.0387454517361603,
-0.0109799901722844));
#25691=CARTESIAN_POINT('Ctrl Pts',(0.00571558786153034,-0.0387371486665608,
-0.0109429793781871));
#25692=CARTESIAN_POINT('Ctrl Pts',(0.005758339787551,-0.0387345822208101,
-0.0109338919464912));
#25693=CARTESIAN_POINT('Ctrl Pts',(0.00581407324498526,-0.0387311382889725,
-0.0109250318349941));
#25694=CARTESIAN_POINT('Ctrl Pts',(0.00582670382954977,-0.0387303513362258,
-0.0109232194731103));
#25695=CARTESIAN_POINT('Ctrl Pts',(0.00584763287841279,-0.0387290334900665,
-0.0109205389480718));
#25696=CARTESIAN_POINT('Ctrl Pts',(0.00585591672686075,-0.0387285082746606,
-0.0109195611885365));
#25697=CARTESIAN_POINT('Ctrl Pts',(0.00587362156668634,-0.0387273771165653,
-0.0109176488679723));
#25698=CARTESIAN_POINT('Ctrl Pts',(0.00588304424903874,-0.0387267700582242,
-0.0109167380390071));
#25699=CARTESIAN_POINT('Ctrl Pts',(0.00591055033710448,-0.0387249849802696,
-0.0109143906150102));
#25700=CARTESIAN_POINT('Ctrl Pts',(0.00592865484816423,-0.0387237937142453,
-0.0109132373085436));
#25701=CARTESIAN_POINT('Ctrl Pts',(0.00603090397030049,-0.0387169959796343,
-0.0109089297952436));
#25702=CARTESIAN_POINT('Ctrl Pts',(0.00611517146583091,-0.0387111437003502,
-0.0109137973953982));
#25703=CARTESIAN_POINT('Ctrl Pts',(0.00625991662077184,-0.0387011484259906,
-0.0109367840762009));
#25704=CARTESIAN_POINT('Ctrl Pts',(0.00632070451410851,-0.0386969654931938,
-0.0109511085802484));
#25705=CARTESIAN_POINT('Ctrl Pts',(0.00639954993701431,-0.0386915995844553,
-0.0109759649655577));
#25706=CARTESIAN_POINT('Ctrl Pts',(0.00641875694040768,-0.038690296673864,
-0.0109825323591412));
#25707=CARTESIAN_POINT('Ctrl Pts',(0.00645160591917498,-0.038688074393787,
-0.0109946551849937));
#25708=CARTESIAN_POINT('Ctrl Pts',(0.00646532380762949,-0.0386871481962535,
-0.0109999916261736));
#25709=CARTESIAN_POINT('Ctrl Pts',(0.00649361022399706,-0.0386852409840039,
-0.0110115679876082));
#25710=CARTESIAN_POINT('Ctrl Pts',(0.00650816094992898,-0.0386842613745905,
-0.0110178447398494));
#25711=CARTESIAN_POINT('Ctrl Pts',(0.00654688539386126,-0.0386816554641844,
-0.0110354198413622));
#25712=CARTESIAN_POINT('Ctrl Pts',(0.00657082646709165,-0.0386800457568886,
-0.0110472127913562));
#25713=CARTESIAN_POINT('Ctrl Pts',(0.00668229558573361,-0.0386725241427527,
-0.0111065756376862));
#25714=CARTESIAN_POINT('Ctrl Pts',(0.00676436989454704,-0.0386669372655562,
-0.0111636177792272));
#25715=CARTESIAN_POINT('Ctrl Pts',(0.00687158555002229,-0.0386586341956333,
-0.0112586799290506));
#25716=CARTESIAN_POINT('Ctrl Pts',(0.0069027435334229,-0.0386560677497,
-0.0112893310129275));
#25717=CARTESIAN_POINT('Ctrl Pts',(0.00694087113027838,-0.0386526238176475,
-0.0113309363805012));
#25718=CARTESIAN_POINT('Ctrl Pts',(0.00694934865823438,-0.0386518368648792,
-0.0113404730387649));
#25719=CARTESIAN_POINT('Ctrl Pts',(0.0069631269446376,-0.0386505190186614,
-0.0113564533129963));
#25720=CARTESIAN_POINT('Ctrl Pts',(0.00696851106549649,-0.0386499938032181,
-0.0113628242949652));
#25721=CARTESIAN_POINT('Ctrl Pts',(0.00697987040099121,-0.0386488626449133,
-0.0113765386647298));
#25722=CARTESIAN_POINT('Ctrl Pts',(0.00698582675136782,-0.0386482555863983,
-0.0113838965512263));
#25723=CARTESIAN_POINT('Ctrl Pts',(0.00700295437633025,-0.0386464705077923,
-0.0114055469623153));
#25724=CARTESIAN_POINT('Ctrl Pts',(0.00701390097689067,-0.0386452792412829,
-0.0114200133246907));
#25725=CARTESIAN_POINT('Ctrl Pts',(0.00707388407121027,-0.0386384814994386,
-0.0115029318892635));
#25726=CARTESIAN_POINT('Ctrl Pts',(0.00711629669748798,-0.0386326292130035,
-0.0115759105899205));
#25727=CARTESIAN_POINT('Ctrl Pts',(0.00717694776053939,-0.0386226339415916,
-0.0117093309288648));
#25728=CARTESIAN_POINT('Ctrl Pts',(0.00719852268134543,-0.0386184510180771,
-0.0117679386548639));
#25729=CARTESIAN_POINT('Ctrl Pts',(0.00722127077262911,-0.0386130851181356,
-0.0118474178516646));
#25730=CARTESIAN_POINT('Ctrl Pts',(0.00722638494385483,-0.0386117822076683,
-0.0118670618029199));
#25731=CARTESIAN_POINT('Ctrl Pts',(0.00723438836302389,-0.0386095599275956,
-0.0119011493902246));
#25732=CARTESIAN_POINT('Ctrl Pts',(0.00723750215415133,-0.0386086337299485,
-0.0119155355790618));
#25733=CARTESIAN_POINT('Ctrl Pts',(0.00724344519666881,-0.0386067265172649,
-0.0119455158088585));
#25734=CARTESIAN_POINT('Ctrl Pts',(0.00724623390578158,-0.0386057469075351,
-0.0119611153124359));
#25735=CARTESIAN_POINT('Ctrl Pts',(0.00725292944074801,-0.0386031409957286,
-0.0120031110091382));
#25736=CARTESIAN_POINT('Ctrl Pts',(0.00725629537802834,-0.0386015312873746,
-0.0120295859045205));
#25737=CARTESIAN_POINT('Ctrl Pts',(0.00726825072594748,-0.0385940096722593,
-0.0121553093567262));
#25738=CARTESIAN_POINT('Ctrl Pts',(0.00726593088788882,-0.0385884227950085,
-0.0122552324104382));
#25739=CARTESIAN_POINT('Ctrl Pts',(0.00724576087682851,-0.0385801197262389,
-0.0123970956294928));
#25740=CARTESIAN_POINT('Ctrl Pts',(0.00723737584686981,-0.0385775532816926,
-0.0124399908268264));
#25741=CARTESIAN_POINT('Ctrl Pts',(0.00722369669097977,-0.038574109351185,
-0.0124947411514895));
#25742=CARTESIAN_POINT('Ctrl Pts',(0.00722041672163876,-0.0385733223984535,
-0.0125070723361646));
#25743=CARTESIAN_POINT('Ctrl Pts',(0.0072146849627803,-0.0385720045522725,
-0.0125273789177083));
#25744=CARTESIAN_POINT('Ctrl Pts',(0.00721233973686755,-0.0385714793368279,
-0.01253538379649));
#25745=CARTESIAN_POINT('Ctrl Pts',(0.00720716411001813,-0.0385703481786079,
-0.0125524229067683));
#25746=CARTESIAN_POINT('Ctrl Pts',(0.00720431121107332,-0.0385697411201799,
-0.0125614493980619));
#25747=CARTESIAN_POINT('Ctrl Pts',(0.00719569668621866,-0.0385679560417007,
-0.0125876769729951));
#25748=CARTESIAN_POINT('Ctrl Pts',(0.0071896661421002,-0.0385667647752283,
-0.0126047865088812));
#25749=CARTESIAN_POINT('Ctrl Pts',(0.007153577568203,-0.0385599670326137,
-0.0127005522492241));
#25750=CARTESIAN_POINT('Ctrl Pts',(0.00711609060292571,-0.0385541147452527,
-0.0127761793013874));
#25751=CARTESIAN_POINT('Ctrl Pts',(0.00703824290463211,-0.0385441194736393,
-0.0129003536737599));
#25752=CARTESIAN_POINT('Ctrl Pts',(0.00700125203703263,-0.0385399365507607,
-0.0129506728278678));
#25753=CARTESIAN_POINT('Ctrl Pts',(0.00694749763281084,-0.038534570651652,
-0.0130134811100347));
#25754=CARTESIAN_POINT('Ctrl Pts',(0.0069339315050433,-0.0385332677413893,
-0.0130285807662616));
#25755=CARTESIAN_POINT('Ctrl Pts',(0.00690991020983994,-0.0385310454617495,
-0.0130540561511366));
#25756=CARTESIAN_POINT('Ctrl Pts',(0.00689962679789605,-0.0385301192643296,
-0.0130645875071032));
#25757=CARTESIAN_POINT('Ctrl Pts',(0.00687789548893505,-0.03852821205221,
-0.0130860789844425));
#25758=CARTESIAN_POINT('Ctrl Pts',(0.00686642067633903,-0.0385272324428148,
-0.0130970082989701));
#25759=CARTESIAN_POINT('Ctrl Pts',(0.00683508132462889,-0.0385246265322215,
-0.0131257539436761));
#25760=CARTESIAN_POINT('Ctrl Pts',(0.00681485283729608,-0.0385230168247289,
-0.0131431624805026));
#25761=CARTESIAN_POINT('Ctrl Pts',(0.00671657034115043,-0.0385154952111455,
-0.013222471125496));
#25762=CARTESIAN_POINT('Ctrl Pts',(0.00663193729418693,-0.0385099083346477,
-0.0132756429537757));
#25763=CARTESIAN_POINT('Ctrl Pts',(0.00650247435055353,-0.03850160526459,
-0.0133370543317233));
#25764=CARTESIAN_POINT('Ctrl Pts',(0.00646206775598794,-0.0384990388177094,
-0.0133537161899485));
#25765=CARTESIAN_POINT('Ctrl Pts',(0.00640885218508829,-0.0384955948846451,
-0.0133724998311427));
#25766=CARTESIAN_POINT('Ctrl Pts',(0.00639675688910823,-0.0384948079319144,
-0.0133765643276606));
#25767=CARTESIAN_POINT('Ctrl Pts',(0.00637665654127162,-0.0384934900858757,
-0.0133829819781396));
#25768=CARTESIAN_POINT('Ctrl Pts',(0.00636868566545609,-0.0384929648705775,
-0.0133854402843424));
#25769=CARTESIAN_POINT('Ctrl Pts',(0.00635161768346804,-0.0384918337129794,
-0.013390519854762));
#25770=CARTESIAN_POINT('Ctrl Pts',(0.0063425146265189,-0.0384912266550322,
-0.0133931180830601));
#25771=CARTESIAN_POINT('Ctrl Pts',(0.00631588531458509,-0.038489441578788,
-0.0134003963773452));
#25772=CARTESIAN_POINT('Ctrl Pts',(0.00629828712019421,-0.0384882503141049,
-0.0134048016303946));
#25773=CARTESIAN_POINT('Ctrl Pts',(0.00619849917277322,-0.0384814526010313,
-0.0134275114729418));
#25774=CARTESIAN_POINT('Ctrl Pts',(0.00611473927361995,-0.038475600343232,
-0.0134379485234275));
#25775=CARTESIAN_POINT('Ctrl Pts',(0.00596822298919365,-0.0384656050607384,
-0.0134414912394956));
#25776=CARTESIAN_POINT('Ctrl Pts',(0.00590584703805779,-0.038461422100753,
-0.0134383849690581));
#25777=CARTESIAN_POINT('Ctrl Pts',(0.00582380792404518,-0.0384560561659801,
-0.0134281825115457));
#25778=CARTESIAN_POINT('Ctrl Pts',(0.00580373045855541,-0.0384547532547983,
-0.0134251933036864));
#25779=CARTESIAN_POINT('Ctrl Pts',(0.00576923181709878,-0.0384525309742051,
-0.0134192047682781));
#25780=CARTESIAN_POINT('Ctrl Pts',(0.00575477554214615,-0.0384516047767307,
-0.0134164345436876));
#25781=CARTESIAN_POINT('Ctrl Pts',(0.00572486312737236,-0.0384496975650591,
-0.0134101591690809));
#25782=CARTESIAN_POINT('Ctrl Pts',(0.0057094178421176,-0.0384487179561564,
-0.0134066145771941));
#25783=CARTESIAN_POINT('Ctrl Pts',(0.00566815541335507,-0.0384461120483219,
-0.0133963250172466));
#25784=CARTESIAN_POINT('Ctrl Pts',(0.00564247772660968,-0.0384445023430334,
-0.0133890515577103));
#25785=CARTESIAN_POINT('Ctrl Pts',(0.00552211793547214,-0.0384369807299063,
-0.0133508046434737));
#25786=CARTESIAN_POINT('Ctrl Pts',(0.00543108847832245,-0.0384313938519931,
-0.0133095294927673));
#25787=CARTESIAN_POINT('Ctrl Pts',(0.00530846233895228,-0.0384230907802832,
-0.0132354022490875));
#25788=CARTESIAN_POINT('Ctrl Pts',(0.00527227936838826,-0.0384205243331082,
-0.0132108848382613));
#25789=CARTESIAN_POINT('Ctrl Pts',(0.00522726237521781,-0.0384170803996228,
-0.013176852599856));
#25790=CARTESIAN_POINT('Ctrl Pts',(0.0052172013724121,-0.0384162934467488,
-0.0131690045046441));
#25791=CARTESIAN_POINT('Ctrl Pts',(0.00520076267597678,-0.0384149756002612,
-0.0131557765121691));
#25792=CARTESIAN_POINT('Ctrl Pts',(0.00519431611448294,-0.0384144503846522,
-0.0131504831146578));
#25793=CARTESIAN_POINT('Ctrl Pts',(0.00518066593349501,-0.0384133192253875,
-0.0131390467017707));
#25794=CARTESIAN_POINT('Ctrl Pts',(0.00517347824851354,-0.0384127121660697,
-0.0131328860179246));
#25795=CARTESIAN_POINT('Ctrl Pts',(0.00515272088123464,-0.0384109270845197,
-0.0131146862910231));
#25796=CARTESIAN_POINT('Ctrl Pts',(0.00513934076934827,-0.0384097358158363,
-0.0131024356783558));
#25797=CARTESIAN_POINT('Ctrl Pts',(0.00506536359133869,-0.0384029380420105,
-0.0130317183837278));
#25798=CARTESIAN_POINT('Ctrl Pts',(0.00501046365503673,-0.038397085724011,
-0.0129676029021016));
#25799=CARTESIAN_POINT('Ctrl Pts',(0.00492670594677885,-0.0383870904657682,
-0.0128473359321362));
#25800=CARTESIAN_POINT('Ctrl Pts',(0.00489489778060487,-0.0383829075833806,
-0.0127935910754407));
#25801=CARTESIAN_POINT('Ctrl Pts',(0.00485816483979804,-0.0383775417223395,
-0.0127195302141824));
#25802=CARTESIAN_POINT('Ctrl Pts',(0.00484958576971037,-0.0383762388123558,
-0.0127011335064036));
#25803=CARTESIAN_POINT('Ctrl Pts',(0.00483555547002561,-0.0383740165321598,
-0.0126690528387957));
#25804=CARTESIAN_POINT('Ctrl Pts',(0.00482989377190817,-0.0383730903339322,
-0.0126554659486419));
#25805=CARTESIAN_POINT('Ctrl Pts',(0.00481863200601154,-0.0383711831191316,
-0.0126270527705208));
#25806=CARTESIAN_POINT('Ctrl Pts',(0.00481307082698056,-0.0383702035078833,
-0.0126122137848643));
#25807=CARTESIAN_POINT('Ctrl Pts',(0.00479889810317191,-0.0383675975894454,
-0.0125721187479176));
#25808=CARTESIAN_POINT('Ctrl Pts',(0.0047908043311595,-0.0383659878760986,
-0.0125466875661106));
#25809=CARTESIAN_POINT('Ctrl Pts',(0.00475633134804366,-0.038358466256127,
-0.0124251928999911));
#25810=CARTESIAN_POINT('Ctrl Pts',(0.00474055999840928,-0.0383528793783922,
-0.0123264950548821));
#25811=CARTESIAN_POINT('Ctrl Pts',(0.00473583885136971,-0.0383461116660483,
-0.0122097969690597));
#25812=CARTESIAN_POINT('Ctrl Pts',(0.00473549444331784,-0.038345110727623,
-0.0121926237908312));
#25813=CARTESIAN_POINT('Ctrl Pts',(0.00473550006772914,-0.0383440997603812,
-0.0121754394182212));
#25814=CARTESIAN_POINT('Ctrl Pts',(0.00473550000000377,-0.0384058394797894,
-0.0121758563747875));
#25815=CARTESIAN_POINT('Ctrl Pts',(0.004735500711359,-0.0384241673526885,
-0.0124671264108875));
#25816=CARTESIAN_POINT('Ctrl Pts',(0.00484035380825948,-0.0384424952255876,
-0.0127578851096797));
#25817=CARTESIAN_POINT('Ctrl Pts',(0.00502575196577548,-0.0384608230984867,
-0.0129819556484264));
#25818=CARTESIAN_POINT('Ctrl Pts',(0.00505106886622003,-0.0384633258468406,
-0.0130125534256536));
#25819=CARTESIAN_POINT('Ctrl Pts',(0.00507781477904601,-0.0384658285951946,
-0.0130419411008095));
#25820=CARTESIAN_POINT('Ctrl Pts',(0.00510586324542223,-0.0384683313435485,
-0.013069989581601));
#25821=CARTESIAN_POINT('Ctrl Pts',(0.00530747996683213,-0.0384863214864272,
-0.0132716064066304));
#25822=CARTESIAN_POINT('Ctrl Pts',(0.00558091029438798,-0.0385043116293058,
-0.0134026257481341));
#25823=CARTESIAN_POINT('Ctrl Pts',(0.00586501629191922,-0.0385223017721845,
-0.0134331279775277));
#25824=CARTESIAN_POINT('Ctrl Pts',(0.00590987402025746,-0.0385251422505589,
-0.0134379439994764));
#25825=CARTESIAN_POINT('Ctrl Pts',(0.00595495752153627,-0.0385279827289332,
-0.0134403531534092));
#25826=CARTESIAN_POINT('Ctrl Pts',(0.00599999626189027,-0.0385308232073076,
-0.0134403532865526));
#25827=CARTESIAN_POINT('Ctrl Pts',(0.00628630384487386,-0.0385488798956495,
-0.0134403541329339));
#25828=CARTESIAN_POINT('Ctrl Pts',(0.00657323720202342,-0.0385669365839914,
-0.0133388637369163));
#25829=CARTESIAN_POINT('Ctrl Pts',(0.0067960455807007,-0.0385849932723333,
-0.0131583356952794));
#25830=CARTESIAN_POINT('Ctrl Pts',(0.00683027419908225,-0.0385877672052444,
-0.0131306023331813));
#25831=CARTESIAN_POINT('Ctrl Pts',(0.00686302916172385,-0.0385905411381556,
-0.0131010968226352));
#25832=CARTESIAN_POINT('Ctrl Pts',(0.00689413146807798,-0.0385933150710667,
-0.0130699948680723));
#25833=CARTESIAN_POINT('Ctrl Pts',(0.00709655136093038,-0.038611368368988,
-0.0128675772647462));
#25834=CARTESIAN_POINT('Ctrl Pts',(0.00722766676949683,-0.0386294216669094,
-0.0125929766257428));
#25835=CARTESIAN_POINT('Ctrl Pts',(0.00725759263530149,-0.0386474749648307,
-0.0123078419740864));
#25836=CARTESIAN_POINT('Ctrl Pts',(0.00726219643709343,-0.0386502522881624,
-0.0122639767964235));
#25837=CARTESIAN_POINT('Ctrl Pts',(0.00726449963204807,-0.0386530296114941,
-0.0122199001673678));
#25838=CARTESIAN_POINT('Ctrl Pts',(0.00726449999995587,-0.0386558069348258,
-0.0121758638510069));
#25839=CARTESIAN_POINT('Ctrl Pts',(0.00726450239144878,-0.0386738602327476,
-0.0118896167549034));
#25840=CARTESIAN_POINT('Ctrl Pts',(0.00716305422865381,-0.0386919135306694,
-0.0116027309013437));
#25841=CARTESIAN_POINT('Ctrl Pts',(0.00698258861408054,-0.0387099668285911,
-0.0113799388027853));
#25842=CARTESIAN_POINT('Ctrl Pts',(0.0069548257441594,-0.0387127441519224,
-0.011345664417239));
#25843=CARTESIAN_POINT('Ctrl Pts',(0.0069252862090245,-0.0387155214752537,
-0.0113128671345093));
#25844=CARTESIAN_POINT('Ctrl Pts',(0.00689414640842451,-0.038718298798585,
-0.0112817266454711));
#25845=CARTESIAN_POINT('Ctrl Pts',(0.00669169188390851,-0.0387363554869269,
-0.0110792676450937));
#25846=CARTESIAN_POINT('Ctrl Pts',(0.00641703196999779,-0.0387544121752688,
-0.0109481421930123));
#25847=CARTESIAN_POINT('Ctrl Pts',(0.00613183714804358,-0.0387724688636107,
-0.0109182447558953));
#25848=CARTESIAN_POINT('Ctrl Pts',(0.00608802450157561,-0.0387752427965218,
-0.0109136518048953));
#25849=CARTESIAN_POINT('Ctrl Pts',(0.00604400098357289,-0.038778016729433,
-0.0109113538915882));
#25850=CARTESIAN_POINT('Ctrl Pts',(0.00600001739078789,-0.0387807906623441,
-0.0109113532866777));
#25851=CARTESIAN_POINT('Ctrl Pts',(0.00571476495539528,-0.0387987808052228,
-0.010911349363574));
#25852=CARTESIAN_POINT('Ctrl Pts',(0.00542878155389685,-0.0388167709481014,
-0.0110121243151745));
#25853=CARTESIAN_POINT('Ctrl Pts',(0.0052063944651628,-0.0388347610909801,
-0.0111913988665488));
#25854=CARTESIAN_POINT('Ctrl Pts',(0.00517128158581817,-0.0388376015693545,
-0.0112197046721053));
#25855=CARTESIAN_POINT('Ctrl Pts',(0.00513771214689819,-0.0388404420477288,
-0.0112498691377489));
#25856=CARTESIAN_POINT('Ctrl Pts',(0.00510587818592995,-0.0388432825261032,
-0.0112817020512494));
#25857=CARTESIAN_POINT('Ctrl Pts',(0.00490047306974454,-0.0388616103990027,
-0.011487100408765));
#25858=CARTESIAN_POINT('Ctrl Pts',(0.00476860361596144,-0.0388799382719021,
-0.0117665222560225));
#25859=CARTESIAN_POINT('Ctrl Pts',(0.00474113115607628,-0.0388982661448016,
-0.0120566497471888));
#25860=CARTESIAN_POINT('Ctrl Pts',(0.00473737967579684,-0.0389007688931551,
-0.0120962678799));
#25861=CARTESIAN_POINT('Ctrl Pts',(0.00473550076196831,-0.0389032716415087,
-0.0121360549173962));
#25862=CARTESIAN_POINT('Ctrl Pts',(0.0047355000002319,-0.0389057743898623,
-0.0121758290694312));
#25863=CARTESIAN_POINT('Origin',(0.006,-0.0412787743898723,-0.0121758532865581));
#25864=CARTESIAN_POINT('',(0.0047355001992714,-0.0394057384386304,-0.0121763324065659));
#25865=CARTESIAN_POINT('',(0.0047355,-0.0393437675787716,-0.0121758532867651));
#25866=CARTESIAN_POINT('',(0.0047355,-0.0412787743898723,-0.0121758532865581));
#25867=CARTESIAN_POINT('Ctrl Pts',(0.0047355,-0.0393437675787716,-0.0121758532869721));
#25868=CARTESIAN_POINT('Ctrl Pts',(0.00473549999996698,-0.0393368792520501,
-0.0120750100100196));
#25869=CARTESIAN_POINT('Ctrl Pts',(0.00474756385553538,-0.0393299061355532,
-0.0119745079232119));
#25870=CARTESIAN_POINT('Ctrl Pts',(0.00477755184814463,-0.0393215869486887,
-0.0118514365807625));
#25871=CARTESIAN_POINT('Ctrl Pts',(0.00478442452436168,-0.0393199148525418,
-0.0118265652977435));
#25872=CARTESIAN_POINT('Ctrl Pts',(0.00479669080145859,-0.0393172643588143,
-0.0117869405525387));
#25873=CARTESIAN_POINT('Ctrl Pts',(0.00480160630587968,-0.039316271275942,
-0.0117720479732546));
#25874=CARTESIAN_POINT('Ctrl Pts',(0.00481169360095976,-0.0393143587739872,
-0.0117432947660889));
#25875=CARTESIAN_POINT('Ctrl Pts',(0.004816834068814,-0.039313438528612,
-0.0117294259356251));
#25876=CARTESIAN_POINT('Ctrl Pts',(0.0048297763937074,-0.0393112442771047,
-0.011696303067854));
#25877=CARTESIAN_POINT('Ctrl Pts',(0.00483781180765669,-0.03930997809057,
-0.0116771445738722));
#25878=CARTESIAN_POINT('Ctrl Pts',(0.00487816114598391,-0.0393040353783285,
-0.0115872201779668));
#25879=CARTESIAN_POINT('Ctrl Pts',(0.00491648806626039,-0.0392995633061622,
-0.0115193360685833));
#25880=CARTESIAN_POINT('Ctrl Pts',(0.005002685429934,-0.0392908883637259,
-0.0113950046379901));
#25881=CARTESIAN_POINT('Ctrl Pts',(0.00504973713903184,-0.0392866964812674,
-0.01133838144694));
#25882=CARTESIAN_POINT('Ctrl Pts',(0.00511182488931374,-0.0392813460311627,
-0.0112756736266181));
#25883=CARTESIAN_POINT('Ctrl Pts',(0.00512240052643995,-0.0392804399826695,
-0.011265360250361));
#25884=CARTESIAN_POINT('Ctrl Pts',(0.00513955983757548,-0.0392789734717999,
-0.0112492031928951));
#25885=CARTESIAN_POINT('Ctrl Pts',(0.00514602839708126,-0.039278421422328,
-0.0112432385959332));
#25886=CARTESIAN_POINT('Ctrl Pts',(0.00515915984202016,-0.0392773010273396,
-0.0112313813770644));
#25887=CARTESIAN_POINT('Ctrl Pts',(0.00516582368660932,-0.0392767326225019,
-0.0112254906051568));
#25888=CARTESIAN_POINT('Ctrl Pts',(0.00518407325136593,-0.0392751777541251,
-0.0112096979887208));
#25889=CARTESIAN_POINT('Ctrl Pts',(0.00519577640481568,-0.0392741825385337,
-0.0111999348061444));
#25890=CARTESIAN_POINT('Ctrl Pts',(0.00524763988364612,-0.0392697906078088,
-0.0111582348957848));
#25891=CARTESIAN_POINT('Ctrl Pts',(0.00528954407807787,-0.0392662911493851,
-0.0111285498456279));
#25892=CARTESIAN_POINT('Ctrl Pts',(0.00541659758759926,-0.0392560383961803,
-0.0110496860891085));
#25893=CARTESIAN_POINT('Ctrl Pts',(0.00550583192612201,-0.0392493004493489,
-0.0110077715321705));
#25894=CARTESIAN_POINT('Ctrl Pts',(0.00561909156203013,-0.0392415326914313,
-0.0109699028372782));
#25895=CARTESIAN_POINT('Ctrl Pts',(0.00563931952154971,-0.0392401722724608,
-0.0109636992524275));
#25896=CARTESIAN_POINT('Ctrl Pts',(0.00567385475363577,-0.0392378934814224,
-0.0109540490084974));
#25897=CARTESIAN_POINT('Ctrl Pts',(0.00568808326808116,-0.0392369670037755,
-0.0109503393548326));
#25898=CARTESIAN_POINT('Ctrl Pts',(0.00571746463897593,-0.0392350780360863,
-0.0109432239377833));
#25899=CARTESIAN_POINT('Ctrl Pts',(0.00573262205985419,-0.0392341166031605,
-0.0109398474566256));
#25900=CARTESIAN_POINT('Ctrl Pts',(0.00577230440056622,-0.039231630955099,
-0.0109317719624973));
#25901=CARTESIAN_POINT('Ctrl Pts',(0.0057969136166969,-0.0392301205700967,
-0.0109275185278807));
#25902=CARTESIAN_POINT('Ctrl Pts',(0.00592192278943934,-0.039222576195595,
-0.0109097070701317));
#25903=CARTESIAN_POINT('Ctrl Pts',(0.00602356127081529,-0.0392168917562445,
-0.0109075207281582));
#25904=CARTESIAN_POINT('Ctrl Pts',(0.00616936153422826,-0.039208410553092,
-0.0109219311893075));
#25905=CARTESIAN_POINT('Ctrl Pts',(0.00621407476665838,-0.0392057579995878,
-0.0109287866592796));
#25906=CARTESIAN_POINT('Ctrl Pts',(0.00627080030939606,-0.0392022215200484,
-0.0109406245729384));
#25907=CARTESIAN_POINT('Ctrl Pts',(0.00628323962887484,-0.0392014352169469,
-0.0109434174600005));
#25908=CARTESIAN_POINT('Ctrl Pts',(0.00630374253640136,-0.0392001181318345,
-0.010948347575428));
#25909=CARTESIAN_POINT('Ctrl Pts',(0.00631183134614074,-0.0391995930131198,
-0.0109503774574023));
#25910=CARTESIAN_POINT('Ctrl Pts',(0.00632906257756724,-0.0391984616539607,
-0.0109548832734043));
#25911=CARTESIAN_POINT('Ctrl Pts',(0.00633819810882039,-0.0391978542911164,
-0.0109573821219044));
#25912=CARTESIAN_POINT('Ctrl Pts',(0.00636476977452516,-0.0391960673334699,
-0.0109649721236327));
#25913=CARTESIAN_POINT('Ctrl Pts',(0.00638212468408195,-0.0391948744523137,
-0.0109703364557284));
#25914=CARTESIAN_POINT('Ctrl Pts',(0.00647959719340917,-0.0391880504472392,
-0.011002780986944));
#25915=CARTESIAN_POINT('Ctrl Pts',(0.00655695261414959,-0.0391821717268837,
-0.0110374705535267));
#25916=CARTESIAN_POINT('Ctrl Pts',(0.0066839928791492,-0.0391721795097203,
-0.0111105106377234));
#25917=CARTESIAN_POINT('Ctrl Pts',(0.00673538331995836,-0.0391680233874533,
-0.011145312465849));
#25918=CARTESIAN_POINT('Ctrl Pts',(0.00679993633001906,-0.039162683153921,
-0.0111963260166604));
#25919=CARTESIAN_POINT('Ctrl Pts',(0.00681554870062379,-0.0391613807886448,
-0.0112092860631907));
#25920=CARTESIAN_POINT('Ctrl Pts',(0.00684193719639083,-0.0391591591292178,
-0.0112322863392827));
#25921=CARTESIAN_POINT('Ctrl Pts',(0.00685286188420044,-0.0391582330174713,
-0.011242149124597));
#25922=CARTESIAN_POINT('Ctrl Pts',(0.00687518836630212,-0.0391563257134717,
-0.0112630243160011));
#25923=CARTESIAN_POINT('Ctrl Pts',(0.00688656032466012,-0.0391553459312388,
-0.0112740649347519));
#25924=CARTESIAN_POINT('Ctrl Pts',(0.0069165233014155,-0.0391527388785663,
-0.0113042696800743));
#25925=CARTESIAN_POINT('Ctrl Pts',(0.00693472041425494,-0.0391511282289925,
-0.0113238140629616));
#25926=CARTESIAN_POINT('Ctrl Pts',(0.00701781098827082,-0.0391436066312714,
-0.011418925165053));
#25927=CARTESIAN_POINT('Ctrl Pts',(0.00707424304872707,-0.0391380205090514,
-0.0115014043557035));
#25928=CARTESIAN_POINT('Ctrl Pts',(0.0071406571208009,-0.0391297189542401,
-0.0116283422162969));
#25929=CARTESIAN_POINT('Ctrl Pts',(0.00715888078049186,-0.0391271533430565,
-0.0116680524727002));
#25930=CARTESIAN_POINT('Ctrl Pts',(0.00717972704713311,-0.0391237103596348,
-0.0117204774694981));
#25931=CARTESIAN_POINT('Ctrl Pts',(0.00718426154651319,-0.0391229234566766,
-0.0117324036261477));
#25932=CARTESIAN_POINT('Ctrl Pts',(0.00719146070534891,-0.0391216056688344,
-0.0117522364625896));
#25933=CARTESIAN_POINT('Ctrl Pts',(0.00719422907732423,-0.039121080460829,
-0.0117601048845008));
#25934=CARTESIAN_POINT('Ctrl Pts',(0.00719997289811524,-0.0391199492872855,
-0.011776961173683));
#25935=CARTESIAN_POINT('Ctrl Pts',(0.00720292555158233,-0.0391193422055784,
-0.0117859558920852));
#25936=CARTESIAN_POINT('Ctrl Pts',(0.00721124122763924,-0.0391175569835497,
-0.0118122820161948));
#25937=CARTESIAN_POINT('Ctrl Pts',(0.00721633239518159,-0.0391163655937595,
-0.0118296960833896));
#25938=CARTESIAN_POINT('Ctrl Pts',(0.00724293803934281,-0.0391095658515815,
-0.0119285479314783));
#25939=CARTESIAN_POINT('Ctrl Pts',(0.00725664701194782,-0.039103711552185,
-0.0120118638110337));
#25940=CARTESIAN_POINT('Ctrl Pts',(0.00726591125311987,-0.0390937165145658,
-0.012158128254658));
#25941=CARTESIAN_POINT('Ctrl Pts',(0.00726524688766458,-0.039089535634441,
-0.012220547935026));
#25942=CARTESIAN_POINT('Ctrl Pts',(0.00725826586979714,-0.0390841716900076,
-0.0123028930883928));
#25943=CARTESIAN_POINT('Ctrl Pts',(0.00725606487391386,-0.0390828688201593,
-0.0123230715557001));
#25944=CARTESIAN_POINT('Ctrl Pts',(0.00725143136136867,-0.0390806465864308,
-0.0123577774646468));
#25945=CARTESIAN_POINT('Ctrl Pts',(0.00724922911943015,-0.0390797203952848,
-0.0123723310076697));
#25946=CARTESIAN_POINT('Ctrl Pts',(0.00724412936254339,-0.0390778131761194,
-0.0124024662760157));
#25947=CARTESIAN_POINT('Ctrl Pts',(0.00724119199942449,-0.0390768335537556,
-0.012418038696931));
#25948=CARTESIAN_POINT('Ctrl Pts',(0.00723252509507326,-0.039074227557888,
-0.0124596737084334));
#25949=CARTESIAN_POINT('Ctrl Pts',(0.00722626194009152,-0.0390726177801117,
-0.0124856176198209));
#25950=CARTESIAN_POINT('Ctrl Pts',(0.00719275483556149,-0.0390650961386547,
-0.0126073828479602));
#25951=CARTESIAN_POINT('Ctrl Pts',(0.00715507431207189,-0.0390595092931116,
-0.0126999575651164));
#25952=CARTESIAN_POINT('Ctrl Pts',(0.00708580441172114,-0.0390512063305857,
-0.0128253892625129));
#25953=CARTESIAN_POINT('Ctrl Pts',(0.00706272287071529,-0.0390486399708224,
-0.0128625028294435));
#25954=CARTESIAN_POINT('Ctrl Pts',(0.00703047977242015,-0.0390451961366919,
-0.0129088161085037));
#25955=CARTESIAN_POINT('Ctrl Pts',(0.00702303156639845,-0.0390444091890612,
-0.0129191765306699));
#25956=CARTESIAN_POINT('Ctrl Pts',(0.00701045724425558,-0.0390430913488836,
-0.0129361203353359));
#25957=CARTESIAN_POINT('Ctrl Pts',(0.00700542025544153,-0.0390425661342271,
-0.0129427691456154));
#25958=CARTESIAN_POINT('Ctrl Pts',(0.00699452692244313,-0.0390414349744801,
-0.0129568565314825));
#25959=CARTESIAN_POINT('Ctrl Pts',(0.0069886522989608,-0.0390408279136841,
-0.0129642798758794));
#25960=CARTESIAN_POINT('Ctrl Pts',(0.00697127893065427,-0.0390390428207079,
-0.0129857338701434));
#25961=CARTESIAN_POINT('Ctrl Pts',(0.0069595613533048,-0.0390378515417997,
-0.0129995833726727));
#25962=CARTESIAN_POINT('Ctrl Pts',(0.0068917922961739,-0.0390310535983054,
-0.0130762738437472));
#25963=CARTESIAN_POINT('Ctrl Pts',(0.00682987300420974,-0.039025201108867,
-0.0131336428391805));
#25964=CARTESIAN_POINT('Ctrl Pts',(0.00671297625450975,-0.0390152058599817,
-0.0132220433428793));
#25965=CARTESIAN_POINT('Ctrl Pts',(0.0066605195592206,-0.0390110231415432,
-0.0132559294451103));
#25966=CARTESIAN_POINT('Ctrl Pts',(0.0065879554257665,-0.0390056574379195,
-0.0132955320573579));
#25967=CARTESIAN_POINT('Ctrl Pts',(0.00656990867918295,-0.0390043545315766,
-0.0133048246350736));
#25968=CARTESIAN_POINT('Ctrl Pts',(0.0065384018589696,-0.0390021322563034,
-0.0133200998943206));
#25969=CARTESIAN_POINT('Ctrl Pts',(0.00652504701818892,-0.0390012060594077,
-0.0133262890817003));
#25970=CARTESIAN_POINT('Ctrl Pts',(0.00649709646367876,-0.0389992988463479,
-0.0133386543947277));
#25971=CARTESIAN_POINT('Ctrl Pts',(0.00648248653954957,-0.0389983192355242,
-0.0133447921580197));
#25972=CARTESIAN_POINT('Ctrl Pts',(0.00644297698056191,-0.038995713315959,
-0.0133605234847858));
#25973=CARTESIAN_POINT('Ctrl Pts',(0.00641788208130595,-0.0389941036011306,
-0.0133696065257176));
#25974=CARTESIAN_POINT('Ctrl Pts',(0.00629782994506804,-0.0389865819837905,
-0.0134088087890464));
#25975=CARTESIAN_POINT('Ctrl Pts',(0.00619982514309347,-0.0389809951097283,
-0.0134284314121707));
#25976=CARTESIAN_POINT('Ctrl Pts',(0.00605698897966107,-0.0389726920510793,
-0.0134398234525344));
#25977=CARTESIAN_POINT('Ctrl Pts',(0.00601329892582182,-0.038970125614426,
-0.0134410373652243));
#25978=CARTESIAN_POINT('Ctrl Pts',(0.0059568820447084,-0.0389666816929195,
-0.0134396823508011));
#25979=CARTESIAN_POINT('Ctrl Pts',(0.00594413188113673,-0.0389658947407048,
-0.0134391829293478));
#25980=CARTESIAN_POINT('Ctrl Pts',(0.00592306296437831,-0.0389645768951545,
-0.0134380381068915));
#25981=CARTESIAN_POINT('Ctrl Pts',(0.00591473878583227,-0.0389640516798132,
-0.0134375031391276));
#25982=CARTESIAN_POINT('Ctrl Pts',(0.00589697979758102,-0.0389629205214791,
-0.0134361852687505));
#25983=CARTESIAN_POINT('Ctrl Pts',(0.0058875476123952,-0.0389623134628286,
-0.0134353787189763));
#25984=CARTESIAN_POINT('Ctrl Pts',(0.00586007003285857,-0.0389605283830802,
-0.0134327180044229));
#25985=CARTESIAN_POINT('Ctrl Pts',(0.00584205506212158,-0.0389593371155352,
-0.0134305813989566));
#25986=CARTESIAN_POINT('Ctrl Pts',(0.00574070996510327,-0.0389525393563457,
-0.0134163446907461));
#25987=CARTESIAN_POINT('Ctrl Pts',(0.00565870828341002,-0.0389466870523613,
-0.0133963325207105));
#25988=CARTESIAN_POINT('Ctrl Pts',(0.0055204981265756,-0.0389366917816797,
-0.0133475729906142));
#25989=CARTESIAN_POINT('Ctrl Pts',(0.00546329891601119,-0.03893250887473,
-0.0133225018295304));
#25990=CARTESIAN_POINT('Ctrl Pts',(0.00539024210262064,-0.0389271429907183,
-0.0132838097122881));
#25991=CARTESIAN_POINT('Ctrl Pts',(0.00537253770468859,-0.0389258400806388,
-0.0132738802801265));
#25992=CARTESIAN_POINT('Ctrl Pts',(0.00534241952148878,-0.038923617801115,
-0.0132560221509658));
#25993=CARTESIAN_POINT('Ctrl Pts',(0.00532989150757916,-0.0389226916036335,
-0.0132482951258556));
#25994=CARTESIAN_POINT('Ctrl Pts',(0.00530416206566204,-0.0389207843912085,
-0.0132317987775011));
#25995=CARTESIAN_POINT('Ctrl Pts',(0.00529098480118406,-0.0389198047815729,
-0.0132229964445133));
#25996=CARTESIAN_POINT('Ctrl Pts',(0.00525607287374027,-0.0389171988698475,
-0.0131987142295685));
#25997=CARTESIAN_POINT('Ctrl Pts',(0.00523465638688125,-0.0389155891614845,
-0.0131827899170279));
#25998=CARTESIAN_POINT('Ctrl Pts',(0.00513574665300983,-0.0389080675468332,
-0.0131042648912665));
#25999=CARTESIAN_POINT('Ctrl Pts',(0.00506532873808064,-0.0389024806700257,
-0.0130333331341246));
#26000=CARTESIAN_POINT('Ctrl Pts',(0.00497705226703553,-0.0388941776015515,
-0.0129204647775152));
#26001=CARTESIAN_POINT('Ctrl Pts',(0.00495194474516104,-0.0388916111568294,
-0.0128846888173399));
#26002=CARTESIAN_POINT('Ctrl Pts',(0.00492196140382903,-0.0388881672261529,
-0.0128368796453873));
#26003=CARTESIAN_POINT('Ctrl Pts',(0.00491534636472717,-0.0388873802734561,
-0.0128259682954244));
#26004=CARTESIAN_POINT('Ctrl Pts',(0.00490468196062504,-0.038886062427337,
-0.0128077616824293));
#26005=CARTESIAN_POINT('Ctrl Pts',(0.00490053748232425,-0.0388855372119199,
-0.0128005227970824));
#26006=CARTESIAN_POINT('Ctrl Pts',(0.00489184284321092,-0.0388844060537095,
-0.0127849818306632));
#26007=CARTESIAN_POINT('Ctrl Pts',(0.00488731385568098,-0.0388837989952631,
-0.0127766688976815));
#26008=CARTESIAN_POINT('Ctrl Pts',(0.00487437964994546,-0.0388820139168246,
-0.012752280334548));
#26009=CARTESIAN_POINT('Ctrl Pts',(0.0048662268156162,-0.038880822650414,
-0.0127360743190182));
#26010=CARTESIAN_POINT('Ctrl Pts',(0.00482221165324144,-0.0388740249096991,
-0.0126436831839392));
#26011=CARTESIAN_POINT('Ctrl Pts',(0.00479368198600604,-0.0388681726243199,
-0.0125642427849889));
#26012=CARTESIAN_POINT('Ctrl Pts',(0.0047581339497195,-0.0388581773517096,
-0.0124220602282504));
#26013=CARTESIAN_POINT('Ctrl Pts',(0.00474750267794351,-0.038853994426094,
-0.0123605190018496));
#26014=CARTESIAN_POINT('Ctrl Pts',(0.00473948838005238,-0.0388486285242107,
-0.0122782378114584));
#26015=CARTESIAN_POINT('Ctrl Pts',(0.00473800742720685,-0.0388473256137542,
-0.0122579931495147));
#26016=CARTESIAN_POINT('Ctrl Pts',(0.00473629429393456,-0.0388451033337848,
-0.0122230205404961));
#26017=CARTESIAN_POINT('Ctrl Pts',(0.00473583088644126,-0.0388441771362282,
-0.0122083085272168));
#26018=CARTESIAN_POINT('Ctrl Pts',(0.00473554147278037,-0.0388428896926793,
-0.0121876789223812));
#26019=CARTESIAN_POINT('Ctrl Pts',(0.00473550000000128,-0.0388425219863233,
-0.0121817661174845));
#26020=CARTESIAN_POINT('Ctrl Pts',(0.0047355,-0.0388421555262979,-0.0121758532868327));
#26021=CARTESIAN_POINT('Ctrl Pts',(0.00473550000000009,-0.0389057758757622,
-0.012175852808333));
#26022=CARTESIAN_POINT('Ctrl Pts',(0.0047354998898438,-0.038924103588367,
-0.0124671228095654));
#26023=CARTESIAN_POINT('Ctrl Pts',(0.00484035214344072,-0.0389424313009718,
-0.012757881776193));
#26024=CARTESIAN_POINT('Ctrl Pts',(0.00502574963092566,-0.0389607590135766,
-0.0129819528265397));
#26025=CARTESIAN_POINT('Ctrl Pts',(0.00505106714236682,-0.0389632618094875,
-0.0130125515226587));
#26026=CARTESIAN_POINT('Ctrl Pts',(0.00507781374867609,-0.0389657646053984,
-0.01304194005383));
#26027=CARTESIAN_POINT('Ctrl Pts',(0.00510586298069669,-0.0389682674013093,
-0.0130699893168753));
#26028=CARTESIAN_POINT('Ctrl Pts',(0.00530747958806939,-0.0389862573847828,
-0.0132716061472521));
#26029=CARTESIAN_POINT('Ctrl Pts',(0.00558090980094445,-0.0390042473682563,
-0.0134026255654758));
#26030=CARTESIAN_POINT('Ctrl Pts',(0.00586501572457188,-0.0390222373517298,
-0.013433127916616));
#26031=CARTESIAN_POINT('Ctrl Pts',(0.00590987457571402,-0.039025077876772,
-0.0134379440795872));
#26032=CARTESIAN_POINT('Ctrl Pts',(0.00595495921214838,-0.0390279184018141,
-0.0134403532537739));
#26033=CARTESIAN_POINT('Ctrl Pts',(0.00599999907958751,-0.0390307589268563,
-0.0134403532865578));
#26034=CARTESIAN_POINT('Ctrl Pts',(0.0062863065904634,-0.0390488154554528,
-0.0134403534949571));
#26035=CARTESIAN_POINT('Ctrl Pts',(0.00657323966808948,-0.0390668719840494,
-0.013338862507273));
#26036=CARTESIAN_POINT('Ctrl Pts',(0.00679604762633477,-0.0390849285126459,
-0.0131583340378234));
#26037=CARTESIAN_POINT('Ctrl Pts',(0.00683027706300004,-0.039087702492565,
-0.0131305998946627));
#26038=CARTESIAN_POINT('Ctrl Pts',(0.00686303276466382,-0.0390904764724841,
-0.013101093515359));
#26039=CARTESIAN_POINT('Ctrl Pts',(0.00689413571764325,-0.0390932504524032,
-0.0130699906185349));
#26040=CARTESIAN_POINT('Ctrl Pts',(0.00709655459888521,-0.0391113035907076,
-0.0128675721027531));
#26041=CARTESIAN_POINT('Ctrl Pts',(0.00722766869842946,-0.0391293567290121,
-0.0125929709100995));
#26042=CARTESIAN_POINT('Ctrl Pts',(0.00725759324381091,-0.0391474098673166,
-0.0123078361760596));
#26043=CARTESIAN_POINT('Ctrl Pts',(0.00726219696087802,-0.0391501872375278,
-0.0122639698574641));
#26044=CARTESIAN_POINT('Ctrl Pts',(0.00726449995254541,-0.039152964607739,
-0.0122198920873515));
#26045=CARTESIAN_POINT('Ctrl Pts',(0.00726449999999927,-0.0391557419779502,
-0.012175854649158));
#26046=CARTESIAN_POINT('Ctrl Pts',(0.00726450030845333,-0.0391737951162547,
-0.011889607623441));
#26047=CARTESIAN_POINT('Ctrl Pts',(0.00716305010451997,-0.0391918482545591,
-0.0116027225601036));
#26048=CARTESIAN_POINT('Ctrl Pts',(0.00698258293554201,-0.0392099013928636,
-0.011379931792451));
#26049=CARTESIAN_POINT('Ctrl Pts',(0.00695481911238977,-0.0392126787630748,
-0.0113456567300777));
#26050=CARTESIAN_POINT('Ctrl Pts',(0.00692527854380358,-0.039215456133286,
-0.0113128588587458));
#26051=CARTESIAN_POINT('Ctrl Pts',(0.00689413764465013,-0.0392182335034972,
-0.0112817178815888));
#26052=CARTESIAN_POINT('Ctrl Pts',(0.00669168118644839,-0.0392362900320937,
-0.0110792609162627));
#26053=CARTESIAN_POINT('Ctrl Pts',(0.00641702005861165,-0.0392543465606902,
-0.0109481381604391));
#26054=CARTESIAN_POINT('Ctrl Pts',(0.00613182500527585,-0.0392724030892866,
-0.0109182434830085));
#26055=CARTESIAN_POINT('Ctrl Pts',(0.00608801119318087,-0.0392751770692058,
-0.0109136508375041));
#26056=CARTESIAN_POINT('Ctrl Pts',(0.00604398652098787,-0.039277951049125,
-0.0109113533493376));
#26057=CARTESIAN_POINT('Ctrl Pts',(0.00600000180478717,-0.0392807250290442,
-0.0109113532865594));
#26058=CARTESIAN_POINT('Ctrl Pts',(0.0057147494451515,-0.0392987150125177,
-0.0109113528794263));
#26059=CARTESIAN_POINT('Ctrl Pts',(0.00542876734207387,-0.0393167049959913,
-0.0110121313060387));
#26060=CARTESIAN_POINT('Ctrl Pts',(0.0052063824825844,-0.0393346949794648,
-0.0111914085262739));
#26061=CARTESIAN_POINT('Ctrl Pts',(0.00517126906720493,-0.039337535504507,
-0.0112197154690965));
#26062=CARTESIAN_POINT('Ctrl Pts',(0.00513769919244742,-0.0393403760295491,
-0.0112498811464967));
#26063=CARTESIAN_POINT('Ctrl Pts',(0.00510586490770486,-0.0393432165545913,
-0.0112817153292348));
#26064=CARTESIAN_POINT('Ctrl Pts',(0.00490046287355843,-0.0393615442671949,
-0.0114871167052248));
#26065=CARTESIAN_POINT('Ctrl Pts',(0.00476859756919286,-0.0393798719797985,
-0.0117665404683745));
#26066=CARTESIAN_POINT('Ctrl Pts',(0.00474112939608375,-0.039398199692402,
-0.0120566683353456));
#26067=CARTESIAN_POINT('Ctrl Pts',(0.00473737839709893,-0.0394007024883141,
-0.0120962876187305));
#26068=CARTESIAN_POINT('Ctrl Pts',(0.0047355000706813,-0.0394032052842262,
-0.0121360757886226));
#26069=CARTESIAN_POINT('Ctrl Pts',(0.004735500000002,-0.0394057080801383,
-0.0121758510395836));
#26070=CARTESIAN_POINT('Origin',(0.006,-0.0412787743898723,-0.0121758532865581));
#26071=CARTESIAN_POINT('',(0.00473550016783225,-0.0399058036708604,-0.0121753956645968));
#26072=CARTESIAN_POINT('',(0.0047355,-0.0398434635507866,-0.0121758533388321));
#26073=CARTESIAN_POINT('',(0.0047355,-0.0412787743898723,-0.0121758532865581));
#26074=CARTESIAN_POINT('Ctrl Pts',(0.0047355,-0.0398434635507866,-0.0121758533911061));
#26075=CARTESIAN_POINT('Ctrl Pts',(0.00473549999871623,-0.0398425730336631,
-0.0121603262647505));
#26076=CARTESIAN_POINT('Ctrl Pts',(0.00473578598915216,-0.0398416814807293,
-0.012144793103517));
#26077=CARTESIAN_POINT('Ctrl Pts',(0.00473771522235276,-0.0398386660407253,
-0.0120924690080894));
#26078=CARTESIAN_POINT('Ctrl Pts',(0.00474067799968203,-0.0398365301708808,
-0.0120557550046254));
#26079=CARTESIAN_POINT('Ctrl Pts',(0.00474728561309504,-0.039833359682442,
-0.0120028209337214));
#26080=CARTESIAN_POINT('Ctrl Pts',(0.00474965465898228,-0.0398323669216644,
-0.0119864594887893));
#26081=CARTESIAN_POINT('Ctrl Pts',(0.00475452352385184,-0.0398305444041562,
-0.0119569282734438));
#26082=CARTESIAN_POINT('Ctrl Pts',(0.00475691333422698,-0.0398297194916137,
-0.0119437427036166));
#26083=CARTESIAN_POINT('Ctrl Pts',(0.00476116729457608,-0.0398283514289037,
-0.0119222263852539));
#26084=CARTESIAN_POINT('Ctrl Pts',(0.00476290714918767,-0.0398278147399946,
-0.0119138717000038));
#26085=CARTESIAN_POINT('Ctrl Pts',(0.00476671193992603,-0.0398266853100518,
-0.0118964849961814));
#26086=CARTESIAN_POINT('Ctrl Pts',(0.00476879178473736,-0.0398260918779022,
-0.0118874570328898));
#26087=CARTESIAN_POINT('Ctrl Pts',(0.00477499028516025,-0.0398243897368797,
-0.0118618412498231));
#26088=CARTESIAN_POINT('Ctrl Pts',(0.00477934617361855,-0.0398232694909095,
-0.0118453135270823));
#26089=CARTESIAN_POINT('Ctrl Pts',(0.00480578068815565,-0.0398168843935129,
-0.0117526739949715));
#26090=CARTESIAN_POINT('Ctrl Pts',(0.00483464047371733,-0.0398113905697856,
-0.0116786846484056));
#26091=CARTESIAN_POINT('Ctrl Pts',(0.00489875860328867,-0.0398016296401179,
-0.0115511445764787));
#26092=CARTESIAN_POINT('Ctrl Pts',(0.00493152138538451,-0.0397973468153562,
-0.0114966266299599));
#26093=CARTESIAN_POINT('Ctrl Pts',(0.00498141345853777,-0.0397917130586943,
-0.0114262131066627));
#26094=CARTESIAN_POINT('Ctrl Pts',(0.00499508073012373,-0.03979024395799,
-0.0114079885137661));
#26095=CARTESIAN_POINT('Ctrl Pts',(0.00501863257896625,-0.0397878299586647,
-0.0113782900942377));
#26096=CARTESIAN_POINT('Ctrl Pts',(0.0050282438112329,-0.0397868749026981,
-0.0113666073400606));
#26097=CARTESIAN_POINT('Ctrl Pts',(0.00504792040127838,-0.0397849774233039,
-0.0113435460458716));
#26098=CARTESIAN_POINT('Ctrl Pts',(0.0050579857586511,-0.0397840352233526,
-0.0113321708195238));
#26099=CARTESIAN_POINT('Ctrl Pts',(0.00508388079154384,-0.0397816792831149,
-0.0113039472512419));
#26100=CARTESIAN_POINT('Ctrl Pts',(0.00509997236014619,-0.0397802765930414,
-0.011287346176422));
#26101=CARTESIAN_POINT('Ctrl Pts',(0.00516472607808981,-0.0397748485377832,
-0.0112241077160463));
#26102=CARTESIAN_POINT('Ctrl Pts',(0.00521663022018865,-0.0397709616916161,
-0.0111809487226794));
#26103=CARTESIAN_POINT('Ctrl Pts',(0.0053175467035916,-0.039763879742537,
-0.0111098520483408));
#26104=CARTESIAN_POINT('Ctrl Pts',(0.00536545503199703,-0.0397606840681993,
-0.0110806577759889));
#26105=CARTESIAN_POINT('Ctrl Pts',(0.00543353668269892,-0.0397561672907358,
-0.0110451410517151));
#26106=CARTESIAN_POINT('Ctrl Pts',(0.0054521671259105,-0.0397549333418394,
-0.0110359980736416));
#26107=CARTESIAN_POINT('Ctrl Pts',(0.00548539780306348,-0.0397527217937917,
-0.0110206928469228));
#26108=CARTESIAN_POINT('Ctrl Pts',(0.00549990494336334,-0.0397517528569151,
-0.0110143387814702));
#26109=CARTESIAN_POINT('Ctrl Pts',(0.00552285116151035,-0.039750209131006,
-0.0110047979888791));
#26110=CARTESIAN_POINT('Ctrl Pts',(0.00553121198453355,-0.0397496443658862,
-0.0110014260604236));
#26111=CARTESIAN_POINT('Ctrl Pts',(0.00554770725849822,-0.0397485243246831,
-0.0109949776997911));
#26112=CARTESIAN_POINT('Ctrl Pts',(0.00555583872891021,-0.0397479694011279,
-0.0109918952523875));
#26113=CARTESIAN_POINT('Ctrl Pts',(0.00557738388106423,-0.0397464929144523,
-0.010983981173393));
#26114=CARTESIAN_POINT('Ctrl Pts',(0.00559084833603183,-0.0397455639606821,
-0.010979292216427));
#26115=CARTESIAN_POINT('Ctrl Pts',(0.0056791097279547,-0.0397394467852465,
-0.0109502192724743));
#26116=CARTESIAN_POINT('Ctrl Pts',(0.00575595980303853,-0.0397340033639544,
-0.0109326347950351));
#26117=CARTESIAN_POINT('Ctrl Pts',(0.00590706589949332,-0.0397235632552518,
-0.0109126174506006));
#26118=CARTESIAN_POINT('Ctrl Pts',(0.00598090852293102,-0.0397185800004054,
-0.0109093463135961));
#26119=CARTESIAN_POINT('Ctrl Pts',(0.00607529272130587,-0.0397124420449962,
-0.0109134273496162));
#26120=CARTESIAN_POINT('Ctrl Pts',(0.00609593718780759,-0.0397111128179512,
-0.0109148281573623));
#26121=CARTESIAN_POINT('Ctrl Pts',(0.00613125247819444,-0.0397088604923665,
-0.010918096800554));
#26122=CARTESIAN_POINT('Ctrl Pts',(0.00614594142667959,-0.0397079300581504,
-0.0109197164626415));
#26123=CARTESIAN_POINT('Ctrl Pts',(0.00617617991867307,-0.0397060266754757,
-0.0109235882876082));
#26124=CARTESIAN_POINT('Ctrl Pts',(0.0061917226936039,-0.0397050549130296,
-0.0109258735131326));
#26125=CARTESIAN_POINT('Ctrl Pts',(0.00623281055152999,-0.0397025008524645,
-0.0109326990416615));
#26126=CARTESIAN_POINT('Ctrl Pts',(0.0062582659688675,-0.039700933933303,
-0.0109377369535174));
#26127=CARTESIAN_POINT('Ctrl Pts',(0.00638613651834869,-0.0396931087662235,
-0.010967159741422));
#26128=CARTESIAN_POINT('Ctrl Pts',(0.00648536860536396,-0.0396872264942755,
-0.0110034802865309));
#26129=CARTESIAN_POINT('Ctrl Pts',(0.00660349958051729,-0.039679502627529,
-0.0110643179275181));
#26130=CARTESIAN_POINT('Ctrl Pts',(0.00662762434558757,-0.0396778809542012,
-0.0110777594306216));
#26131=CARTESIAN_POINT('Ctrl Pts',(0.00666790371812734,-0.039675065084725,
-0.0111019628738786));
#26132=CARTESIAN_POINT('Ctrl Pts',(0.00668428623571204,-0.0396738878024674,
-0.0111123269564249));
#26133=CARTESIAN_POINT('Ctrl Pts',(0.0067084974580347,-0.0396720892137892,
-0.011128434719574));
#26134=CARTESIAN_POINT('Ctrl Pts',(0.00671650946002454,-0.0396714840729467,
-0.0111338991213237));
#26135=CARTESIAN_POINT('Ctrl Pts',(0.00673130877071756,-0.039670346048942,
-0.0111442440547512));
#26136=CARTESIAN_POINT('Ctrl Pts',(0.00673811183493579,-0.0396698146358723,
-0.011149100624618));
#26137=CARTESIAN_POINT('Ctrl Pts',(0.00675482836888941,-0.0396684888371073,
-0.0111612862015588));
#26138=CARTESIAN_POINT('Ctrl Pts',(0.00676468355633603,-0.0396676896058306,
-0.0111686932851221));
#26139=CARTESIAN_POINT('Ctrl Pts',(0.00680464683820562,-0.0396643808905084,
-0.0111996540506689));
#26140=CARTESIAN_POINT('Ctrl Pts',(0.00683378569181862,-0.0396618081250233,
-0.0112244215178391));
#26141=CARTESIAN_POINT('Ctrl Pts',(0.00692014223919626,-0.0396537749630439,
-0.0113048401799208));
#26142=CARTESIAN_POINT('Ctrl Pts',(0.00697325681895921,-0.039648246404119,
-0.0113646207921799));
#26143=CARTESIAN_POINT('Ctrl Pts',(0.00703821874619604,-0.0396408468536321,
-0.0114533756588055));
#26144=CARTESIAN_POINT('Ctrl Pts',(0.00705517603101273,-0.0396388386705201,
-0.0114783750817396));
#26145=CARTESIAN_POINT('Ctrl Pts',(0.00708425053212983,-0.0396352537588027,
-0.0115247295224242));
#26146=CARTESIAN_POINT('Ctrl Pts',(0.00709667192631941,-0.0396336676256535,
-0.011545875357773));
#26147=CARTESIAN_POINT('Ctrl Pts',(0.00711590296690817,-0.039631117287945,
-0.0115809084721999));
#26148=CARTESIAN_POINT('Ctrl Pts',(0.0071230862363398,-0.0396301403821461,
-0.011594582176817));
#26149=CARTESIAN_POINT('Ctrl Pts',(0.00713663772928902,-0.0396282471045765,
-0.0116215676697012));
#26150=CARTESIAN_POINT('Ctrl Pts',(0.00714302699238698,-0.0396273301303916,
-0.0116348660447212));
#26151=CARTESIAN_POINT('Ctrl Pts',(0.00715813635276517,-0.0396250978748872,
-0.0116677774909757));
#26152=CARTESIAN_POINT('Ctrl Pts',(0.00716659278890381,-0.0396237914863275,
-0.0116875069227721));
#26153=CARTESIAN_POINT('Ctrl Pts',(0.00721013120870794,-0.0396167166417189,
-0.0117966799196198));
#26154=CARTESIAN_POINT('Ctrl Pts',(0.0072354338234921,-0.0396112772785581,
-0.0118896807685754));
#26155=CARTESIAN_POINT('Ctrl Pts',(0.0072558130989148,-0.0396035244138168,
-0.0120229106952813));
#26156=CARTESIAN_POINT('Ctrl Pts',(0.00725990514803603,-0.0396012840645187,
-0.01206141263571));
#26157=CARTESIAN_POINT('Ctrl Pts',(0.00726324526001623,-0.039597977473665,
-0.0121170220094639));
#26158=CARTESIAN_POINT('Ctrl Pts',(0.00726392241684811,-0.0395969570287086,
-0.0121340229278381));
#26159=CARTESIAN_POINT('Ctrl Pts',(0.0072645250694901,-0.0395950893226703,
-0.0121647180974538));
#26160=CARTESIAN_POINT('Ctrl Pts',(0.00726457150264754,-0.0395942472916623,
-0.0121784074785993));
#26161=CARTESIAN_POINT('Ctrl Pts',(0.0072642854083989,-0.0395928586620499,
-0.0122006805328556));
#26162=CARTESIAN_POINT('Ctrl Pts',(0.00726408766330845,-0.0395923189253832,
-0.0122092652738219));
#26163=CARTESIAN_POINT('Ctrl Pts',(0.00726349787575642,-0.0395911924954774,
-0.0122270148535366));
#26164=CARTESIAN_POINT('Ctrl Pts',(0.00726309351885227,-0.0395906052602424,
-0.012236178559888));
#26165=CARTESIAN_POINT('Ctrl Pts',(0.00726167599879556,-0.0395889401289352,
-0.0122619364391194));
#26166=CARTESIAN_POINT('Ctrl Pts',(0.00726043524798963,-0.0395878514253083,
-0.0122785156510738));
#26167=CARTESIAN_POINT('Ctrl Pts',(0.00725134964668775,-0.0395814704873993,
-0.0123744593002325));
#26168=CARTESIAN_POINT('Ctrl Pts',(0.0072363376653185,-0.039575941740716,
-0.0124529604966164));
#26169=CARTESIAN_POINT('Ctrl Pts',(0.00719620774994823,-0.0395661299325991,
-0.0125907142888971));
#26170=CARTESIAN_POINT('Ctrl Pts',(0.00717377829703182,-0.0395618309659139,
-0.012650478373365));
#26171=CARTESIAN_POINT('Ctrl Pts',(0.00713733155497881,-0.0395561799438829,
-0.0127289873250513));
#26172=CARTESIAN_POINT('Ctrl Pts',(0.00712717055428588,-0.0395547087992434,
-0.0127494097170517));
#26173=CARTESIAN_POINT('Ctrl Pts',(0.00710935760137422,-0.0395522924220401,
-0.0127829075984756));
#26174=CARTESIAN_POINT('Ctrl Pts',(0.00710201354731257,-0.039551336989218,
-0.0127961398319851));
#26175=CARTESIAN_POINT('Ctrl Pts',(0.00708682902470908,-0.0395494394621625,
-0.0128223773809974));
#26176=CARTESIAN_POINT('Ctrl Pts',(0.00707898830310865,-0.0395484975792306,
-0.0128353796364852));
#26177=CARTESIAN_POINT('Ctrl Pts',(0.00705864079456163,-0.0395461438317747,
-0.0128677873537415));
#26178=CARTESIAN_POINT('Ctrl Pts',(0.00704583301386208,-0.0395447429720405,
-0.0128869977801207));
#26179=CARTESIAN_POINT('Ctrl Pts',(0.00698583206638948,-0.0395385094726972,
-0.0129718632616287));
#26180=CARTESIAN_POINT('Ctrl Pts',(0.00693293409140296,-0.0395338901262536,
-0.0130332517492821));
#26181=CARTESIAN_POINT('Ctrl Pts',(0.00682714716296224,-0.0395254893060913,
-0.0131345461167398));
#26182=CARTESIAN_POINT('Ctrl Pts',(0.00677630714365207,-0.0395217215608465,
-0.0131761581254128));
#26183=CARTESIAN_POINT('Ctrl Pts',(0.00671045394004568,-0.0395168546820953,
-0.0132220033762255));
#26184=CARTESIAN_POINT('Ctrl Pts',(0.00669828840301553,-0.039515955937636,
-0.0132301625750231));
#26185=CARTESIAN_POINT('Ctrl Pts',(0.00667861392344697,-0.0395144983718384,
-0.0132428679882191));
#26186=CARTESIAN_POINT('Ctrl Pts',(0.00667119423118024,-0.0395139477819667,
-0.0132475507839627));
#26187=CARTESIAN_POINT('Ctrl Pts',(0.00665613270458966,-0.0395128270377177,
-0.0132568388191417));
#26188=CARTESIAN_POINT('Ctrl Pts',(0.00664848970368741,-0.0395122567739995,
-0.0132614411184432));
#26189=CARTESIAN_POINT('Ctrl Pts',(0.00662754417199865,-0.0395106911447898,
-0.0132737535363856));
#26190=CARTESIAN_POINT('Ctrl Pts',(0.00661414908460164,-0.0395096868342676,
-0.013281302290321));
#26191=CARTESIAN_POINT('Ctrl Pts',(0.00655479806369439,-0.0395052342659157,
-0.0133133376927267));
#26192=CARTESIAN_POINT('Ctrl Pts',(0.00650749513530756,-0.0395016806859326,
-0.0133352149716183));
#26193=CARTESIAN_POINT('Ctrl Pts',(0.00639812382988118,-0.0394936316428007,
-0.0133778197987371));
#26194=CARTESIAN_POINT('Ctrl Pts',(0.0063355151022178,-0.0394891416010819,
-0.0133967778756529));
#26195=CARTESIAN_POINT('Ctrl Pts',(0.00623279140903417,-0.0394820943926213,
-0.0134193793675272));
#26196=CARTESIAN_POINT('Ctrl Pts',(0.00619347787933736,-0.0394794682015931,
-0.0134260995806315));
#26197=CARTESIAN_POINT('Ctrl Pts',(0.00613602802260432,-0.0394757355256694,
-0.0134331444884616));
#26198=CARTESIAN_POINT('Ctrl Pts',(0.00611810148456964,-0.0394745852880538,
-0.0134349549035853));
#26199=CARTESIAN_POINT('Ctrl Pts',(0.00608570790750952,-0.0394725316288873,
-0.0134375283839546));
#26200=CARTESIAN_POINT('Ctrl Pts',(0.00607125512256349,-0.039471624232183,
-0.0134384270989329));
#26201=CARTESIAN_POINT('Ctrl Pts',(0.00603970574223539,-0.0394696614215763,
-0.0134398454353331));
#26202=CARTESIAN_POINT('Ctrl Pts',(0.00602260747440094,-0.0394686091635386,
-0.0134402668435503));
#26203=CARTESIAN_POINT('Ctrl Pts',(0.00597167916045773,-0.0394655048936305,
-0.0134404885728341));
#26204=CARTESIAN_POINT('Ctrl Pts',(0.00593785901844548,-0.0394634831632167,
-0.013439278492207));
#26205=CARTESIAN_POINT('Ctrl Pts',(0.0058092500041775,-0.0394558856409178,
-0.0134294992381665));
#26206=CARTESIAN_POINT('Ctrl Pts',(0.00571549661962608,-0.039450558819576,
-0.013411600348725));
#26207=CARTESIAN_POINT('Ctrl Pts',(0.00559996511864355,-0.0394435080227075,
-0.0133756866073562));
#26208=CARTESIAN_POINT('Ctrl Pts',(0.00557553294453327,-0.0394419860402525,
-0.0133672623191858));
#26209=CARTESIAN_POINT('Ctrl Pts',(0.00553406780674108,-0.0394393232001577,
-0.0133515276482681));
#26210=CARTESIAN_POINT('Ctrl Pts',(0.00551690559551872,-0.0394381968929906,
-0.0133445802572899));
#26211=CARTESIAN_POINT('Ctrl Pts',(0.00549114348868031,-0.0394364604351813,
-0.0133334871916281));
#26212=CARTESIAN_POINT('Ctrl Pts',(0.00548242716578311,-0.0394358648299555,
-0.0133296165011747));
#26213=CARTESIAN_POINT('Ctrl Pts',(0.00546619414138775,-0.0394347388617283,
-0.0133221868815999));
#26214=CARTESIAN_POINT('Ctrl Pts',(0.00545866737347649,-0.039434209828916,
-0.0133186517717289));
#26215=CARTESIAN_POINT('Ctrl Pts',(0.00543983056793416,-0.0394328690056492,
-0.0133095768246517));
#26216=CARTESIAN_POINT('Ctrl Pts',(0.00542856759815566,-0.0394320519386242,
-0.0133039418625878));
#26217=CARTESIAN_POINT('Ctrl Pts',(0.00538083664955803,-0.0394285290246062,
-0.0132791634578248));
#26218=CARTESIAN_POINT('Ctrl Pts',(0.00534523407302543,-0.0394257497932153,
-0.0132584139485412));
#26219=CARTESIAN_POINT('Ctrl Pts',(0.00522751145313689,-0.0394161724752054,
-0.0131818702838085));
#26220=CARTESIAN_POINT('Ctrl Pts',(0.00515095620933812,-0.0394092972822839,
-0.0131181580656726));
#26221=CARTESIAN_POINT('Ctrl Pts',(0.0050630308980468,-0.0394008679125229,
-0.0130254771495794));
#26222=CARTESIAN_POINT('Ctrl Pts',(0.00504412706169264,-0.0393990143680964,
-0.013004152107354));
#26223=CARTESIAN_POINT('Ctrl Pts',(0.00501564290776988,-0.0393961533420522,
-0.0129697443686626));
#26224=CARTESIAN_POINT('Ctrl Pts',(0.00500556699254515,-0.0393951266523914,
-0.0129570862656416));
#26225=CARTESIAN_POINT('Ctrl Pts',(0.00498685784296865,-0.0393931905709259,
-0.0129326337710019));
#26226=CARTESIAN_POINT('Ctrl Pts',(0.00497818084244687,-0.0393922795941065,
-0.0129208763527132));
#26227=CARTESIAN_POINT('Ctrl Pts',(0.00495860067613465,-0.0393901914088626,
-0.0128933592580963));
#26228=CARTESIAN_POINT('Ctrl Pts',(0.00494784793025412,-0.0393890199001457,
-0.012877496680104));
#26229=CARTESIAN_POINT('Ctrl Pts',(0.00491170333890462,-0.0393849852979684,
-0.0128214751653821));
#26230=CARTESIAN_POINT('Ctrl Pts',(0.00488821600920942,-0.0393821884938485,
-0.0127801332073064));
#26231=CARTESIAN_POINT('Ctrl Pts',(0.00482209191386929,-0.0393735525985662,
-0.0126467703460761));
#26232=CARTESIAN_POINT('Ctrl Pts',(0.00478815756692421,-0.039367910615778,
-0.0125509052735547));
#26233=CARTESIAN_POINT('Ctrl Pts',(0.00476205822316223,-0.0393607301401242,
-0.0124342924930554));
#26234=CARTESIAN_POINT('Ctrl Pts',(0.00475847130345653,-0.0393596235685395,
-0.0124164714237126));
#26235=CARTESIAN_POINT('Ctrl Pts',(0.0047536012484247,-0.0393579112099727,
-0.0123892546764662));
#26236=CARTESIAN_POINT('Ctrl Pts',(0.00475203747938668,-0.0393573193617461,
-0.0123799109631057));
#26237=CARTESIAN_POINT('Ctrl Pts',(0.00474929492120454,-0.0393561956113855,
-0.01236231131214));
#26238=CARTESIAN_POINT('Ctrl Pts',(0.00474809257008097,-0.0393556649419783,
-0.0123540597978812));
#26239=CARTESIAN_POINT('Ctrl Pts',(0.0047452593922461,-0.0393543126707145,
-0.0123331702702483));
#26240=CARTESIAN_POINT('Ctrl Pts',(0.0047437378656051,-0.039353485598572,
-0.0123205185784411));
#26241=CARTESIAN_POINT('Ctrl Pts',(0.00473787898038878,-0.0393498070643418,
-0.0122646969183499));
#26242=CARTESIAN_POINT('Ctrl Pts',(0.00473557428322698,-0.0393468741467418,
-0.0122213462701389));
#26243=CARTESIAN_POINT('Ctrl Pts',(0.00473550058894212,-0.0393438638310085,
-0.0121772625009416));
#26244=CARTESIAN_POINT('Ctrl Pts',(0.00473550000000023,-0.039343815707962,
-0.0121765578855601));
#26245=CARTESIAN_POINT('Ctrl Pts',(0.0047355,-0.0393437675787716,-0.0121758532869721));
#26246=CARTESIAN_POINT('Ctrl Pts',(0.00473550043525086,-0.0394057743898623,
-0.0121769024525323));
#26247=CARTESIAN_POINT('Ctrl Pts',(0.00473574210657924,-0.0394241093002937,
-0.0124681750414799));
#26248=CARTESIAN_POINT('Ctrl Pts',(0.00484083747198399,-0.0394424442107252,
-0.0127588490205952));
#26249=CARTESIAN_POINT('Ctrl Pts',(0.00502642382811335,-0.0394607791211566,
-0.0129827669669072));
#26250=CARTESIAN_POINT('Ctrl Pts',(0.00505171291824375,-0.0394632775440585,
-0.013013279345318));
#26251=CARTESIAN_POINT('Ctrl Pts',(0.00507842401280127,-0.0394657759669604,
-0.0130425855306932));
#26252=CARTESIAN_POINT('Ctrl Pts',(0.00510643135848585,-0.0394682743898623,
-0.01307055733422));
#26253=CARTESIAN_POINT('Ctrl Pts',(0.0053081802385946,-0.0394862715977439,
-0.0132720501889767));
#26254=CARTESIAN_POINT('Ctrl Pts',(0.00558169950567516,-0.0395042688056254,
-0.0134028961466365));
#26255=CARTESIAN_POINT('Ctrl Pts',(0.00586582975456806,-0.0395222660135069,
-0.0134332150464509));
#26256=CARTESIAN_POINT('Ctrl Pts',(0.00591060497947018,-0.0395251021389587,
-0.013437992909995));
#26257=CARTESIAN_POINT('Ctrl Pts',(0.00595560356959221,-0.0395279382644105,
-0.0134403729491083));
#26258=CARTESIAN_POINT('Ctrl Pts',(0.00600055654076817,-0.0395307743898623,
-0.0134403531640837));
#26259=CARTESIAN_POINT('Ctrl Pts',(0.00628686958246528,-0.0395488381503545,
-0.0134402271499314));
#26260=CARTESIAN_POINT('Ctrl Pts',(0.00657376200210831,-0.0395669019108467,
-0.0133386059966377));
#26261=CARTESIAN_POINT('Ctrl Pts',(0.00679649174944665,-0.0395849656713389,
-0.0131579740240764));
#26262=CARTESIAN_POINT('Ctrl Pts',(0.00683064113154301,-0.03958773524418,
-0.0131302791592299));
#26263=CARTESIAN_POINT('Ctrl Pts',(0.00686332180109535,-0.0395905048170212,
-0.0131008197125847));
#26264=CARTESIAN_POINT('Ctrl Pts',(0.00689435586231493,-0.0395932743898623,
-0.0130697704200458));
#26265=CARTESIAN_POINT('Ctrl Pts',(0.00709672871535894,-0.0396113347511412,
-0.0128672982436964));
#26266=CARTESIAN_POINT('Ctrl Pts',(0.00722777549510725,-0.0396293951124201,
-0.0125926594158705));
#26267=CARTESIAN_POINT('Ctrl Pts',(0.00725762714925349,-0.039647455473699,
-0.0123075127087828));
#26268=CARTESIAN_POINT('Ctrl Pts',(0.00726221054608859,-0.0396502284457534,
-0.0122637315330931));
#26269=CARTESIAN_POINT('Ctrl Pts',(0.00726450221993153,-0.0396530014178079,
-0.0122197403218513));
#26270=CARTESIAN_POINT('Ctrl Pts',(0.00726449999838466,-0.0396557743898623,
-0.0121757893710805));
#26271=CARTESIAN_POINT('Ctrl Pts',(0.00726448552945449,-0.0396738347511412,
-0.0118895369192389));
#26272=CARTESIAN_POINT('Ctrl Pts',(0.0071630169273656,-0.0396918951124201,
-0.0116026530874273));
#26273=CARTESIAN_POINT('Ctrl Pts',(0.00698253310284427,-0.039709955473699,
-0.0113798702768053));
#26274=CARTESIAN_POINT('Ctrl Pts',(0.00695482177448543,-0.0397127284457534,
-0.0113456643991637));
#26275=CARTESIAN_POINT('Ctrl Pts',(0.00692534078294909,-0.0397155014178078,
-0.0113129300046642));
#26276=CARTESIAN_POINT('Ctrl Pts',(0.00689426548978842,-0.0397182743898623,
-0.0112818457453296));
#26277=CARTESIAN_POINT('Ctrl Pts',(0.00669183407618031,-0.0397363381503545,
-0.011079355924058));
#26278=CARTESIAN_POINT('Ctrl Pts',(0.00641718620603428,-0.0397544019108467,
-0.010948193571508));
#26279=CARTESIAN_POINT('Ctrl Pts',(0.00613199067792525,-0.0397724656713389,
-0.0109182608601572));
#26280=CARTESIAN_POINT('Ctrl Pts',(0.00608826391408728,-0.03977523524418,
-0.0109136715154051));
#26281=CARTESIAN_POINT('Ctrl Pts',(0.00604432681486676,-0.0397780048170212,
-0.0109113682422291));
#26282=CARTESIAN_POINT('Ctrl Pts',(0.00600042870982249,-0.0397807743898623,
-0.0109113533592319));
#26283=CARTESIAN_POINT('Ctrl Pts',(0.00571517052474766,-0.0397987715977441,
-0.0109112566467029));
#26284=CARTESIAN_POINT('Ctrl Pts',(0.00542915007564361,-0.0398167688056259,
-0.0110119423676297));
#26285=CARTESIAN_POINT('Ctrl Pts',(0.00520670319655887,-0.0398347660135076,
-0.0111911500664709));
#26286=CARTESIAN_POINT('Ctrl Pts',(0.00517164846698451,-0.0398376021389592,
-0.0112193908646622));
#26287=CARTESIAN_POINT('Ctrl Pts',(0.00513813070007935,-0.0398404382644107,
-0.0112494837139568));
#26288=CARTESIAN_POINT('Ctrl Pts',(0.00510634091554443,-0.0398432743898623,
-0.0112812395761948));
#26289=CARTESIAN_POINT('Ctrl Pts',(0.00490082713907305,-0.0398616093002942,
-0.0114865340526787));
#26290=CARTESIAN_POINT('Ctrl Pts',(0.00476881314118491,-0.0398799442107259,
-0.0117658908578301));
#26291=CARTESIAN_POINT('Ctrl Pts',(0.00474119222774112,-0.0398982791211577,
-0.0120560065406672));
#26292=CARTESIAN_POINT('Ctrl Pts',(0.0047374284393678,-0.0399007775440592,
-0.0120955394126051));
#26293=CARTESIAN_POINT('Ctrl Pts',(0.00473552925481075,-0.0399032759669608,
-0.0121352414295939));
#26294=CARTESIAN_POINT('Ctrl Pts',(0.00473550033564982,-0.0399057743898623,
-0.0121749319515005));
#26295=CARTESIAN_POINT('Origin',(0.006,-0.0412787743898723,-0.0121758532865581));
#26296=CARTESIAN_POINT('',(0.004735500019377,-0.0404057743898623,-0.0121756319171353));
#26297=CARTESIAN_POINT('',(0.00473550010973655,-0.0403432744616866,-0.0121763800917601));
#26298=CARTESIAN_POINT('',(0.0047355,-0.0412787743898723,-0.0121758532865581));
#26299=CARTESIAN_POINT('',(0.00510586347519225,-0.0408432743898673,-0.0112817167617504));
#26300=CARTESIAN_POINT('Ctrl Pts',(0.00473550000000687,-0.0404057879868072,
-0.0121758491190739));
#26301=CARTESIAN_POINT('Ctrl Pts',(0.00473549904534208,-0.0404240165869345,
-0.0124655139528556));
#26302=CARTESIAN_POINT('Ctrl Pts',(0.00483905593806693,-0.0404422451870618,
-0.0127544805821245));
#26303=CARTESIAN_POINT('Ctrl Pts',(0.00502252596838094,-0.0404604737871891,
-0.0129780407755595));
#26304=CARTESIAN_POINT('Ctrl Pts',(0.00520599599869494,-0.0404787023873164,
-0.0132016009689945));
#26305=CARTESIAN_POINT('Ctrl Pts',(0.00546957359064989,-0.0404969309874437,
-0.0133596172042219));
#26306=CARTESIAN_POINT('Ctrl Pts',(0.00575330522225602,-0.040515159587571,
-0.0134160556638473));
#26307=CARTESIAN_POINT('Ctrl Pts',(0.00603703685386215,-0.0405333881876983,
-0.0134724941234728));
#26308=CARTESIAN_POINT('Ctrl Pts',(0.00634094837841056,-0.0405516167878256,
-0.0134274133698865));
#26309=CARTESIAN_POINT('Ctrl Pts',(0.00659607887659464,-0.0405698453879529,
-0.0132910439531608));
#26310=CARTESIAN_POINT('Ctrl Pts',(0.00685120937477873,-0.0405880739880802,
-0.013154674536435));
#26311=CARTESIAN_POINT('Ctrl Pts',(0.00705754117506496,-0.0406063025882075,
-0.012927019531437));
#26312=CARTESIAN_POINT('Ctrl Pts',(0.00716824487144537,-0.0406245311883348,
-0.0126597584119098));
#26313=CARTESIAN_POINT('Ctrl Pts',(0.00727894856782577,-0.0406427597884621,
-0.0123924972923825));
#26314=CARTESIAN_POINT('Ctrl Pts',(0.00729402736185934,-0.0406609883885893,
-0.0120856223291149));
#26315=CARTESIAN_POINT('Ctrl Pts',(0.00721005150819125,-0.0406792169887166,
-0.0118087898076828));
#26316=CARTESIAN_POINT('Ctrl Pts',(0.00712607565452316,-0.0406974455888439,
-0.0115319572862506));
#26317=CARTESIAN_POINT('Ctrl Pts',(0.00694305547450676,-0.0407156741889712,
-0.0112851818766085));
#26318=CARTESIAN_POINT('Ctrl Pts',(0.00670251942593715,-0.0407339027890985,
-0.0111244605406344));
#26319=CARTESIAN_POINT('Ctrl Pts',(0.00646198337736753,-0.0407521313892258,
-0.0109637392046603));
#26320=CARTESIAN_POINT('Ctrl Pts',(0.00616387176926783,-0.0407703599893531,
-0.0108890950709833));
#26321=CARTESIAN_POINT('Ctrl Pts',(0.00587605784448035,-0.0407885885894804,
-0.0109174421486206));
#26322=CARTESIAN_POINT('Ctrl Pts',(0.00558824391969287,-0.0408068171896077,
-0.0109457892262579));
#26323=CARTESIAN_POINT('Ctrl Pts',(0.00531068744342894,-0.040825045789735,
-0.0110768927935084));
#26324=CARTESIAN_POINT('Ctrl Pts',(0.00510586347518962,-0.0408432743898623,
-0.0112817167617477));
#26325=CARTESIAN_POINT('',(0.00473533362745302,-0.0408432571870886,-0.0121758704359914));
#26326=CARTESIAN_POINT('Origin',(0.00600000000001,-0.0408432743898623,-0.0121758532865681));
#26327=CARTESIAN_POINT('Ctrl Pts',(0.00473550000001551,-0.0408432557077308,
-0.0121758470227837));
#26328=CARTESIAN_POINT('Ctrl Pts',(0.00473550144284202,-0.0408249249258773,
-0.011884576297668));
#26329=CARTESIAN_POINT('Ctrl Pts',(0.00484035572904346,-0.0408065941440237,
-0.0115938173109497));
#26330=CARTESIAN_POINT('Ctrl Pts',(0.00502575520119273,-0.0407882633621702,
-0.0113697470144097));
#26331=CARTESIAN_POINT('Ctrl Pts',(0.00505105839927943,-0.0407857615891126,
-0.0113391660476304));
#26332=CARTESIAN_POINT('Ctrl Pts',(0.00507778904461344,-0.0407832598160549,
-0.0113097938647511));
#26333=CARTESIAN_POINT('Ctrl Pts',(0.00510582088914852,-0.0407807580429973,
-0.0112817593498172));
#26334=CARTESIAN_POINT('Ctrl Pts',(0.00530742913308967,-0.0407627650039641,
-0.0110801319000609));
#26335=CARTESIAN_POINT('Ctrl Pts',(0.0055808547532575,-0.040744771964931,
-0.0109490995219394));
#26336=CARTESIAN_POINT('Ctrl Pts',(0.00586496058746709,-0.0407267789258978,
-0.0109185845773862));
#26337=CARTESIAN_POINT('Ctrl Pts',(0.00590979587214559,-0.0407239394100198,
-0.0109137689556662));
#26338=CARTESIAN_POINT('Ctrl Pts',(0.00595485681374009,-0.0407210998941418,
-0.0109113578041007));
#26339=CARTESIAN_POINT('Ctrl Pts',(0.00599987328184339,-0.0407182603782637,
-0.0109113532929074));
#26340=CARTESIAN_POINT('Ctrl Pts',(0.00628618228829214,-0.0407002007879828,
-0.0109113246012904));
#26341=CARTESIAN_POINT('Ctrl Pts',(0.00657312656936524,-0.0406821411977019,
-0.0110127880335355));
#26342=CARTESIAN_POINT('Ctrl Pts',(0.00679595286337989,-0.0406640816074211,
-0.0111932957618923));
#26343=CARTESIAN_POINT('Ctrl Pts',(0.00683016678642004,-0.0406613086427908,
-0.0112210118694256));
#26344=CARTESIAN_POINT('Ctrl Pts',(0.00686290871373913,-0.0406585356781604,
-0.0112504984712462));
#26345=CARTESIAN_POINT('Ctrl Pts',(0.00689399989489287,-0.0406557627135301,
-0.0112815801527049));
#26346=CARTESIAN_POINT('Ctrl Pts',(0.00709645054913169,-0.0406377065161534,
-0.011483968949549));
#26347=CARTESIAN_POINT('Ctrl Pts',(0.00722760643875915,-0.0406196503187767,
-0.0117585516667657));
#26348=CARTESIAN_POINT('Ctrl Pts',(0.00725757357256424,-0.0406015941214,
-0.0120436830948051));
#26349=CARTESIAN_POINT('Ctrl Pts',(0.00726218137984443,-0.0405988177638655,
-0.0120875254815505));
#26350=CARTESIAN_POINT('Ctrl Pts',(0.00726449093380774,-0.040596041406331,
-0.0121315794393803));
#26351=CARTESIAN_POINT('Ctrl Pts',(0.0072644999733317,-0.0405932650487966,
-0.0121755935864718));
#26352=CARTESIAN_POINT('Ctrl Pts',(0.00726455876238414,-0.0405752088514199,
-0.0124618420675824));
#26353=CARTESIAN_POINT('Ctrl Pts',(0.00716316620513801,-0.0405571526540431,
-0.0127487489303258));
#26354=CARTESIAN_POINT('Ctrl Pts',(0.00698274316807724,-0.0405390964566663,
-0.0129715769292868));
#26355=CARTESIAN_POINT('Ctrl Pts',(0.00695500095592264,-0.0405363200991319,
-0.0130058394143989));
#26356=CARTESIAN_POINT('Ctrl Pts',(0.00692548358500305,-0.0405335437415975,
-0.0130386266339102));
#26357=CARTESIAN_POINT('Ctrl Pts',(0.00689436714696436,-0.040530767384063,
-0.0130697591297154));
#26358=CARTESIAN_POINT('Ctrl Pts',(0.00669196161561386,-0.0405127077937821,
-0.0132722691132774));
#26359=CARTESIAN_POINT('Ctrl Pts',(0.00641733267734601,-0.0404946482035013,
-0.0134034624598366));
#26360=CARTESIAN_POINT('Ctrl Pts',(0.00613214402769639,-0.0404765886132204,
-0.0134334296086731));
#26361=CARTESIAN_POINT('Ctrl Pts',(0.00608835466004441,-0.0404738156485901,
-0.0134380309225735));
#26362=CARTESIAN_POINT('Ctrl Pts',(0.00604435407325099,-0.0404710426839597,
-0.0134403395736692));
#26363=CARTESIAN_POINT('Ctrl Pts',(0.00600039268201306,-0.0404682697193294,
-0.0134403532255857));
#26364=CARTESIAN_POINT('Ctrl Pts',(0.00571513876285686,-0.0404502766802965,
-0.0134404418092857));
#26365=CARTESIAN_POINT('Ctrl Pts',(0.00542912435281271,-0.0404322836412635,
-0.0133397507523118));
#26366=CARTESIAN_POINT('Ctrl Pts',(0.0052066836807388,-0.0404142906022307,
-0.0131605407839875));
#26367=CARTESIAN_POINT('Ctrl Pts',(0.0051715798931479,-0.0404114510863525,
-0.0131322593163783));
#26368=CARTESIAN_POINT('Ctrl Pts',(0.00513801746798488,-0.0404086115704742,
-0.0131021205785883));
#26369=CARTESIAN_POINT('Ctrl Pts',(0.00510618821846458,-0.0404057720545959,
-0.0130703144367421));
#26370=CARTESIAN_POINT('Ctrl Pts',(0.00490071127995417,-0.0403874412727424,
-0.0128649866721582));
#26371=CARTESIAN_POINT('Ctrl Pts',(0.00476874496696427,-0.0403691104908888,
-0.012585609720854));
#26372=CARTESIAN_POINT('Ctrl Pts',(0.00474117235696595,-0.0403507797090353,
-0.0122954911364775));
#26373=CARTESIAN_POINT('Ctrl Pts',(0.00473740930129016,-0.040348277959919,
-0.0122558963217082));
#26374=CARTESIAN_POINT('Ctrl Pts',(0.00473551667089936,-0.0403457762108028,
-0.0122161321452331));
#26375=CARTESIAN_POINT('Ctrl Pts',(0.00473550010973655,-0.0403432744616866,
-0.0121763800917601));
#26376=CARTESIAN_POINT('Origin',(-0.0125,-0.0412787743898723,-0.0121758532865581));
#26377=CARTESIAN_POINT('',(-0.0137644998890966,-0.0306412974549308,-0.0121754725361131));
#26378=CARTESIAN_POINT('',(-0.013764499947573,-0.0305787585919128,-0.0121761158277784));
#26379=CARTESIAN_POINT('',(-0.0137645,-0.0412787743898723,-0.0121758532865581));
#26380=CARTESIAN_POINT('',(-0.0123336368679221,-0.0302142743898643,-0.0134293617860556));
#26381=CARTESIAN_POINT('Ctrl Pts',(-0.0137644999999586,-0.0305787427939633,
-0.0121758635184457));
#26382=CARTESIAN_POINT('Ctrl Pts',(-0.013764502313608,-0.0305607502112303,
-0.0118899329282279));
#26383=CARTESIAN_POINT('Ctrl Pts',(-0.0136631184159084,-0.0305427576284972,
-0.0116030220978715));
#26384=CARTESIAN_POINT('Ctrl Pts',(-0.0134829588914643,-0.0305247650457642,
-0.0113803961427148));
#26385=CARTESIAN_POINT('Ctrl Pts',(-0.0133590002535709,-0.0305123852614888,
-0.0112272185061392));
#26386=CARTESIAN_POINT('Ctrl Pts',(-0.0131991673647667,-0.0305000054772134,
-0.0111044564592225));
#26387=CARTESIAN_POINT('Ctrl Pts',(-0.0130221765475669,-0.0304876256929381,
-0.0110242058130789));
#26388=CARTESIAN_POINT('Ctrl Pts',(-0.0127747915104563,-0.0304703221206916,
-0.0109120372306151));
#26389=CARTESIAN_POINT('Ctrl Pts',(-0.0124846583937566,-0.0304530185484451,
-0.0108815539625805));
#26390=CARTESIAN_POINT('Ctrl Pts',(-0.0122152033504749,-0.0304357149761986,
-0.0109438422807553));
#26391=CARTESIAN_POINT('Ctrl Pts',(-0.0120116931961525,-0.0304226461814367,
-0.0109908865115473));
#26392=CARTESIAN_POINT('Ctrl Pts',(-0.0118210695107719,-0.0304095773866747,
-0.0110895293206415));
#26393=CARTESIAN_POINT('Ctrl Pts',(-0.0116667589653249,-0.0303965085919128,
-0.0112247120624838));
#26394=CARTESIAN_POINT('Ctrl Pts',(-0.011462446041281,-0.0303792050196663,
-0.0114036990603331));
#26395=CARTESIAN_POINT('Ctrl Pts',(-0.0113148742128925,-0.0303619014474198,
-0.0116553505295554));
#26396=CARTESIAN_POINT('Ctrl Pts',(-0.0112603333855932,-0.0303445978751733,
-0.0119264802023544));
#26397=CARTESIAN_POINT('Ctrl Pts',(-0.0112191405689906,-0.0303315290804114,
-0.0121312551469266));
#26398=CARTESIAN_POINT('Ctrl Pts',(-0.011230262856726,-0.0303184602856495,
-0.0123456017572798));
#26399=CARTESIAN_POINT('Ctrl Pts',(-0.011289660285933,-0.0303053914908876,
-0.0125419653275403));
#26400=CARTESIAN_POINT('Ctrl Pts',(-0.0113714362399216,-0.0302873989081545,
-0.0128123106690992));
#26401=CARTESIAN_POINT('Ctrl Pts',(-0.0115490474424576,-0.0302694063254215,
-0.0130573513611474));
#26402=CARTESIAN_POINT('Ctrl Pts',(-0.0117859367401441,-0.0302514137426883,
-0.0132194403269739));
#26403=CARTESIAN_POINT('Ctrl Pts',(-0.0119489282598164,-0.030239033958413,
-0.0133309655293373));
#26404=CARTESIAN_POINT('Ctrl Pts',(-0.0121386126078993,-0.0302266541741377,
-0.0134034785576961));
#26405=CARTESIAN_POINT('Ctrl Pts',(-0.0123336368679193,-0.0302142743898623,
-0.0134293617860444));
#26406=CARTESIAN_POINT('',(-0.0132689117770196,-0.0302142793348334,-0.0131800804819545));
#26407=CARTESIAN_POINT('Origin',(-0.01249999999999,-0.0302142743898623,
-0.0121758532865681));
#26408=CARTESIAN_POINT('Ctrl Pts',(-0.0132687256619633,-0.0302142800428447,
-0.0131798558297018));
#26409=CARTESIAN_POINT('Ctrl Pts',(-0.0130442789756256,-0.0302320714739704,
-0.0133517059198322));
#26410=CARTESIAN_POINT('Ctrl Pts',(-0.0127604773556288,-0.0302498629050961,
-0.0134450228840146));
#26411=CARTESIAN_POINT('Ctrl Pts',(-0.01247824326561,-0.0302676543362219,
-0.0134401661016908));
#26412=CARTESIAN_POINT('Ctrl Pts',(-0.0121960091755913,-0.0302854457673476,
-0.0134353093193669));
#26413=CARTESIAN_POINT('Ctrl Pts',(-0.0119153315214627,-0.0303032371984734,
-0.0133320736205398));
#26414=CARTESIAN_POINT('Ctrl Pts',(-0.0116971852644419,-0.0303210286295991,
-0.0131528122162838));
#26415=CARTESIAN_POINT('Ctrl Pts',(-0.0114790390074211,-0.0303388200607248,
-0.0129735508120277));
#26416=CARTESIAN_POINT('Ctrl Pts',(-0.0113233711528139,-0.0303566114918506,
-0.0127182793274862));
#26417=CARTESIAN_POINT('Ctrl Pts',(-0.0112638836495351,-0.0303744029229763,
-0.0124422676595061));
#26418=CARTESIAN_POINT('Ctrl Pts',(-0.0112043961462563,-0.030392194354102,
-0.0121662559915259));
#26419=CARTESIAN_POINT('Ctrl Pts',(-0.0112410972350849,-0.0304099857852278,
-0.0118695173223329));
#26420=CARTESIAN_POINT('Ctrl Pts',(-0.0113660322898324,-0.0304277772163535,
-0.0116163200147169));
#26421=CARTESIAN_POINT('Ctrl Pts',(-0.01149096734458,-0.0304455686474792,
-0.0113631227071009));
#26422=CARTESIAN_POINT('Ctrl Pts',(-0.0117041396255603,-0.030463360078605,
-0.0111534601536076));
#26423=CARTESIAN_POINT('Ctrl Pts',(-0.011959383315386,-0.0304811515097307,
-0.011032746182951));
#26424=CARTESIAN_POINT('Ctrl Pts',(-0.0122146270052117,-0.0304989429408564,
-0.0109120322122944));
#26425=CARTESIAN_POINT('Ctrl Pts',(-0.0125119266283734,-0.0305167343719822,
-0.0108802683043807));
#26426=CARTESIAN_POINT('Ctrl Pts',(-0.0127869140293121,-0.0305345258031079,
-0.0109443336603304));
#26427=CARTESIAN_POINT('Ctrl Pts',(-0.0130619014302509,-0.0305523172342336,
-0.0110083990162802));
#26428=CARTESIAN_POINT('Ctrl Pts',(-0.013314596450261,-0.0305701086653594,
-0.0111683452006722));
#26429=CARTESIAN_POINT('Ctrl Pts',(-0.0134901617902954,-0.0305879000964851,
-0.0113893802234218));
#26430=CARTESIAN_POINT('Ctrl Pts',(-0.0136657271303297,-0.0306056915276108,
-0.0116104152461713));
#26431=CARTESIAN_POINT('Ctrl Pts',(-0.0137643323694026,-0.0306234829587366,
-0.0118924230867439));
#26432=CARTESIAN_POINT('Ctrl Pts',(-0.0137644997782563,-0.0306412743898623,
-0.0121751044275857));
#26433=CARTESIAN_POINT('Origin',(-0.0125,-0.0412787743898723,-0.0121758532865581));
#26434=CARTESIAN_POINT('',(-0.0137647273224036,-0.0311411440628488,-0.012176494611068));
#26435=CARTESIAN_POINT('',(-0.01376449983248,-0.0310787450976138,-0.0121763100166715));
#26436=CARTESIAN_POINT('',(-0.0137645,-0.0412787743898723,-0.0121758532865581));
#26437=CARTESIAN_POINT('Ctrl Pts',(-0.0137644999999806,-0.0310787158053654,
-0.0121758462757411));
#26438=CARTESIAN_POINT('Ctrl Pts',(-0.0137644983850769,-0.0310603865105392,
-0.0118845755643713));
#26439=CARTESIAN_POINT('Ctrl Pts',(-0.0136596439362594,-0.0310420572157129,
-0.0115938166505956));
#26440=CARTESIAN_POINT('Ctrl Pts',(-0.0134742443467336,-0.0310237279208867,
-0.0113697464680424));
#26441=CARTESIAN_POINT('Ctrl Pts',(-0.0134489408557085,-0.0310212263234003,
-0.0113391651821412));
#26442=CARTESIAN_POINT('Ctrl Pts',(-0.0134222098869974,-0.0310187247259139,
-0.0113097927073432));
#26443=CARTESIAN_POINT('Ctrl Pts',(-0.0133941776929318,-0.0310162231284275,
-0.0112817579317647));
#26444=CARTESIAN_POINT('Ctrl Pts',(-0.013192569150655,-0.0309982315498371,
-0.0110801308231549));
#26445=CARTESIAN_POINT('Ctrl Pts',(-0.0129191433525998,-0.0309802399712467,
-0.0109490988803221));
#26446=CARTESIAN_POINT('Ctrl Pts',(-0.0126350374955696,-0.0309622483926564,
-0.0109185843714925));
#26447=CARTESIAN_POINT('Ctrl Pts',(-0.0125902017600955,-0.0309594090789341,
-0.0109137687705038));
#26448=CARTESIAN_POINT('Ctrl Pts',(-0.0125451403669309,-0.0309565697652119,
-0.0109113576876354));
#26449=CARTESIAN_POINT('Ctrl Pts',(-0.0125001234545288,-0.0309537304514896,
-0.0109113532925846));
#26450=CARTESIAN_POINT('Ctrl Pts',(-0.0122138144764302,-0.030935672326955,
-0.0109113253399233));
#26451=CARTESIAN_POINT('Ctrl Pts',(-0.0119268704782712,-0.0309176142024204,
-0.0110127894939568));
#26452=CARTESIAN_POINT('Ctrl Pts',(-0.011704044657302,-0.0308995560778858,
-0.0111932977703503));
#26453=CARTESIAN_POINT('Ctrl Pts',(-0.01166983045885,-0.0308967833101078,
-0.0112210142439792));
#26454=CARTESIAN_POINT('Ctrl Pts',(-0.0116370882903576,-0.0308940105423297,
-0.0112505012439437));
#26455=CARTESIAN_POINT('Ctrl Pts',(-0.0116059969071438,-0.0308912377745517,
-0.0112815833497026));
#26456=CARTESIAN_POINT('Ctrl Pts',(-0.0114035469962073,-0.0308731830426072,
-0.0114839728509779));
#26457=CARTESIAN_POINT('Ctrl Pts',(-0.0112723920900571,-0.0308551283106627,
-0.0117585560098165));
#26458=CARTESIAN_POINT('Ctrl Pts',(-0.0112424259622087,-0.0308370735787181,
-0.0120436875214248));
#26459=CARTESIAN_POINT('Ctrl Pts',(-0.0112378182628657,-0.03083429741835,
-0.012087530365764));
#26460=CARTESIAN_POINT('Ctrl Pts',(-0.0112355088639121,-0.0308315212579819,
-0.0121315847773326));
#26461=CARTESIAN_POINT('Ctrl Pts',(-0.0112355000254944,-0.0308287450976138,
-0.0121755993666846));
#26462=CARTESIAN_POINT('Ctrl Pts',(-0.0112354425449309,-0.0308106903656693,
-0.0124618478203132));
#26463=CARTESIAN_POINT('Ctrl Pts',(-0.011336836395326,-0.0307926356337248,
-0.0127487541990847));
#26464=CARTESIAN_POINT('Ctrl Pts',(-0.0115172604246094,-0.0307745809017803,
-0.0129715813663448));
#26465=CARTESIAN_POINT('Ctrl Pts',(-0.0115450030707529,-0.0307718047414122,
-0.0130058440711354));
#26466=CARTESIAN_POINT('Ctrl Pts',(-0.0115745209047644,-0.030769028581044,
-0.0130386314725521));
#26467=CARTESIAN_POINT('Ctrl Pts',(-0.0116056378287405,-0.0307662524206759,
-0.0130697641079603));
#26468=CARTESIAN_POINT('Ctrl Pts',(-0.0118080444673294,-0.0307481942961413,
-0.0132722729448952));
#26469=CARTESIAN_POINT('Ctrl Pts',(-0.0120826741077508,-0.0307301361716068,
-0.0134034647611449));
#26470=CARTESIAN_POINT('Ctrl Pts',(-0.0123678628998988,-0.0307120780470722,
-0.0134334303365939));
#26471=CARTESIAN_POINT('Ctrl Pts',(-0.0124116527348847,-0.0307093052792942,
-0.0134380314557133));
#26472=CARTESIAN_POINT('Ctrl Pts',(-0.0124556537806187,-0.0307065325115161,
-0.0134403398645289));
#26473=CARTESIAN_POINT('Ctrl Pts',(-0.0124996156147847,-0.0307037597437381,
-0.013440353228135));
#26474=CARTESIAN_POINT('Ctrl Pts',(-0.0127848695046488,-0.0306857681651477,
-0.0134404399401816));
#26475=CARTESIAN_POINT('Ctrl Pts',(-0.0130708832318396,-0.0306677765865574,
-0.013339747026259));
#26476=CARTESIAN_POINT('Ctrl Pts',(-0.0132933227203511,-0.030649785007967,
-0.0131605356268967));
#26477=CARTESIAN_POINT('Ctrl Pts',(-0.0133284266712874,-0.0306469456942447,
-0.0131322536513692));
#26478=CARTESIAN_POINT('Ctrl Pts',(-0.0133619892171701,-0.0306441063805225,
-0.0131021143789215));
#26479=CARTESIAN_POINT('Ctrl Pts',(-0.0133938185404324,-0.0306412670668002,
-0.013070307682701));
#26480=CARTESIAN_POINT('Ctrl Pts',(-0.0135992939148588,-0.0306229377719739,
-0.0128649783779801));
#26481=CARTESIAN_POINT('Ctrl Pts',(-0.0137312581167778,-0.0306046084771476,
-0.0125856004461779));
#26482=CARTESIAN_POINT('Ctrl Pts',(-0.0137588285430525,-0.0305862791823214,
-0.012295481666119));
#26483=CARTESIAN_POINT('Ctrl Pts',(-0.0137625913778871,-0.030583777584835,
-0.0122558860123952));
#26484=CARTESIAN_POINT('Ctrl Pts',(-0.0137644837095114,-0.0305812759873487,
-0.0122161210040892));
#26485=CARTESIAN_POINT('Ctrl Pts',(-0.0137644998951874,-0.0305787743898623,
-0.0121763681371112));
#26486=CARTESIAN_POINT('Ctrl Pts',(-0.0137644999999368,-0.0306413205199993,
-0.0121758406446405));
#26487=CARTESIAN_POINT('Ctrl Pts',(-0.0137645029300491,-0.0306597087123115,
-0.0124689233200942));
#26488=CARTESIAN_POINT('Ctrl Pts',(-0.0136584023059271,-0.0306781182315215,
-0.0127613134836949));
#26489=CARTESIAN_POINT('Ctrl Pts',(-0.0134708289910776,-0.0306965228322482,
-0.0129860701217839));
#26490=CARTESIAN_POINT('Ctrl Pts',(-0.0134465321684366,-0.0306989068244488,
-0.0130151833897208));
#26491=CARTESIAN_POINT('Ctrl Pts',(-0.0134209340716843,-0.0307012907341239,
-0.0130431918626772));
#26492=CARTESIAN_POINT('Ctrl Pts',(-0.0133941432291651,-0.0307036745042324,
-0.0130699831069635));
#26493=CARTESIAN_POINT('Ctrl Pts',(-0.0131934054241877,-0.0307215355617486,
-0.0132707239222924));
#26494=CARTESIAN_POINT('Ctrl Pts',(-0.0129214992936078,-0.030739388783757,
-0.0134014108571587));
#26495=CARTESIAN_POINT('Ctrl Pts',(-0.0126391600155025,-0.0307573061545645,
-0.0134326725814789));
#26496=CARTESIAN_POINT('Ctrl Pts',(-0.0125929135130964,-0.0307602409772988,
-0.0134377931775883));
#26497=CARTESIAN_POINT('Ctrl Pts',(-0.0125464294253273,-0.0307631775211235,
-0.013440353054484));
#26498=CARTESIAN_POINT('Ctrl Pts',(-0.0125000063209412,-0.0307661161023836,
-0.0134403532865423));
#26499=CARTESIAN_POINT('Ctrl Pts',(-0.012224309899828,-0.030783567678431,
-0.0134403546646845));
#26500=CARTESIAN_POINT('Ctrl Pts',(-0.0119465654693464,-0.0308010911129074,
-0.0133458957658519));
#26501=CARTESIAN_POINT('Ctrl Pts',(-0.0117277890330815,-0.0308184434524664,
-0.0131771776458797));
#26502=CARTESIAN_POINT('Ctrl Pts',(-0.0116848234390513,-0.0308218512855479,
-0.0131440430251133));
#26503=CARTESIAN_POINT('Ctrl Pts',(-0.0116440699024505,-0.0308252525196365,
-0.0131081960476507));
#26504=CARTESIAN_POINT('Ctrl Pts',(-0.0116058657099795,-0.030828645314453,
-0.0130699920461528));
#26505=CARTESIAN_POINT('Ctrl Pts',(-0.011489497681923,-0.0308389795949825,
-0.0129536245997907));
#26506=CARTESIAN_POINT('Ctrl Pts',(-0.0113964889249869,-0.0308492355775799,
-0.0128160390688021));
#26507=CARTESIAN_POINT('Ctrl Pts',(-0.011331754935869,-0.030859942775707,
-0.0126597579467274));
#26508=CARTESIAN_POINT('Ctrl Pts',(-0.0112670209467511,-0.0308706499738341,
-0.0125034768246526));
#26509=CARTESIAN_POINT('Ctrl Pts',(-0.0112355,-0.030881808387491,-0.0123257398452038));
#26510=CARTESIAN_POINT('Ctrl Pts',(-0.0112355,-0.0308912621404406,-0.0121758532865581));
#26511=CARTESIAN_POINT('Ctrl Pts',(-0.0112355,-0.0309007158933902,-0.0120259667279124));
#26512=CARTESIAN_POINT('Ctrl Pts',(-0.0112576964300095,-0.0309084649856326,
-0.0119036839263425));
#26513=CARTESIAN_POINT('Ctrl Pts',(-0.0113007457940289,-0.0309169920427827,
-0.0117749173821287));
#26514=CARTESIAN_POINT('Ctrl Pts',(-0.0113437951580483,-0.0309255190999327,
-0.0116461508379148));
#26515=CARTESIAN_POINT('Ctrl Pts',(-0.0114125317794308,-0.0309348241219903,
-0.0115133602798955));
#26516=CARTESIAN_POINT('Ctrl Pts',(-0.0115051746667562,-0.0309442973412607,
-0.0113952875901965));
#26517=CARTESIAN_POINT('Ctrl Pts',(-0.011680968239998,-0.0309622731526125,
-0.0111712399528259));
#26518=CARTESIAN_POINT('Ctrl Pts',(-0.0119429575015307,-0.0309808545845356,
-0.0109986148069392));
#26519=CARTESIAN_POINT('Ctrl Pts',(-0.0122485416715191,-0.0310004508145921,
-0.0109366079682141));
#26520=CARTESIAN_POINT('Ctrl Pts',(-0.012265042084108,-0.0310015089383854,
-0.0109332598287396));
#26521=CARTESIAN_POINT('Ctrl Pts',(-0.0122816566882631,-0.0310025700209238,
-0.0109302316696991));
#26522=CARTESIAN_POINT('Ctrl Pts',(-0.012298374142954,-0.0310036341266249,
-0.0109275315076203));
#26523=CARTESIAN_POINT('Ctrl Pts',(-0.0125577285204244,-0.0310201426488116,
-0.0108856412277915));
#26524=CARTESIAN_POINT('Ctrl Pts',(-0.0128442652884611,-0.0310373787972624,
-0.0109263878319273));
#26525=CARTESIAN_POINT('Ctrl Pts',(-0.0130949673908159,-0.0310552769721772,
-0.0110600692331384));
#26526=CARTESIAN_POINT('Ctrl Pts',(-0.0131597001439185,-0.0310598983859064,
-0.0110945865549228));
#26527=CARTESIAN_POINT('Ctrl Pts',(-0.0132219563480234,-0.0310645639371177,
-0.011135041042932));
#26528=CARTESIAN_POINT('Ctrl Pts',(-0.013280570940992,-0.0310692724965332,
-0.0111810320684094));
#26529=CARTESIAN_POINT('Ctrl Pts',(-0.0134918342552102,-0.0310862434557593,
-0.011346796530373));
#26530=CARTESIAN_POINT('Ctrl Pts',(-0.0136575068172827,-0.0311037731269602,
-0.0115906304950738));
#26531=CARTESIAN_POINT('Ctrl Pts',(-0.0137271531481506,-0.0311218791353568,
-0.0118708034529504));
#26532=CARTESIAN_POINT('Ctrl Pts',(-0.0137516666134372,-0.0311282519191458,
-0.0119694161148319));
#26533=CARTESIAN_POINT('Ctrl Pts',(-0.0137645010939262,-0.0311346961015161,
-0.0120721097217937));
#26534=CARTESIAN_POINT('Ctrl Pts',(-0.0137644999999297,-0.0311412124509856,
-0.012175866619248));
#26535=CARTESIAN_POINT('Origin',(-0.0125,-0.0412787743898723,-0.0121758532865581));
#26536=CARTESIAN_POINT('',(-0.013764499973714,-0.0316412626404869,-0.0121760322553932));
#26537=CARTESIAN_POINT('',(-0.0137644998147527,-0.0315788051416157,-0.0121753723444795));
#26538=CARTESIAN_POINT('',(-0.0137645,-0.0412787743898723,-0.0121758532865581));
#26539=CARTESIAN_POINT('Ctrl Pts',(-0.0137644996295201,-0.0315787743898623,
-0.0121748853280777));
#26540=CARTESIAN_POINT('Ctrl Pts',(-0.0137642766641099,-0.0315604396759252,
-0.0118836128362491));
#26541=CARTESIAN_POINT('Ctrl Pts',(-0.0136592000410348,-0.0315421049619881,
-0.0115929321979826));
#26542=CARTESIAN_POINT('Ctrl Pts',(-0.0134736281878384,-0.0315237702480509,
-0.0113690023698167));
#26543=CARTESIAN_POINT('Ctrl Pts',(-0.0134483388141738,-0.0315212716286547,
-0.0113384856454234));
#26544=CARTESIAN_POINT('Ctrl Pts',(-0.0134216271051845,-0.0315187730092585,
-0.0113091752375175));
#26545=CARTESIAN_POINT('Ctrl Pts',(-0.0133936188401708,-0.0315162743898623,
-0.0112811993766623));
#26546=CARTESIAN_POINT('Ctrl Pts',(-0.0131918814404613,-0.0314982773814931,
-0.0110796953770112));
#26547=CARTESIAN_POINT('Ctrl Pts',(-0.0129183697591856,-0.031480280373124,
-0.0109488340864079));
#26548=CARTESIAN_POINT('Ctrl Pts',(-0.0126342414202779,-0.0314622833647548,
-0.0109184991236104));
#26549=CARTESIAN_POINT('Ctrl Pts',(-0.0125894628501879,-0.0314594470397906,
-0.0109137183394654));
#26550=CARTESIAN_POINT('Ctrl Pts',(-0.0125444607432362,-0.0314566107148265,
-0.0109113357548491));
#26551=CARTESIAN_POINT('Ctrl Pts',(-0.0124995041488628,-0.0314537743898623,
-0.0109113533837777));
#26552=CARTESIAN_POINT('Ctrl Pts',(-0.0122131913331388,-0.0314357108288182,
-0.0109114656562539));
#26553=CARTESIAN_POINT('Ctrl Pts',(-0.0119262942079631,-0.0314176472677742,
-0.0110130728866724));
#26554=CARTESIAN_POINT('Ctrl Pts',(-0.0117035558497281,-0.0313995837067301,
-0.0111936939484171));
#26555=CARTESIAN_POINT('Ctrl Pts',(-0.0116694023109608,-0.0313968139344408,
-0.0112213894404884));
#26556=CARTESIAN_POINT('Ctrl Pts',(-0.0116367176417391,-0.0313940441621516,
-0.0112508498765764));
#26557=CARTESIAN_POINT('Ctrl Pts',(-0.0116056797895326,-0.0313912743898623,
-0.0112819004851476));
#26558=CARTESIAN_POINT('Ctrl Pts',(-0.011403299020959,-0.0313732142276789,
-0.011484364430962));
#26559=CARTESIAN_POINT('Ctrl Pts',(-0.0112722413007821,-0.0313551540654955,
-0.0117589978088282));
#26560=CARTESIAN_POINT('Ctrl Pts',(-0.0112423781627974,-0.0313370939033121,
-0.0120441431328445));
#26561=CARTESIAN_POINT('Ctrl Pts',(-0.0112377926229853,-0.0313343207321622,
-0.0120879277222667));
#26562=CARTESIAN_POINT('Ctrl Pts',(-0.011235499174881,-0.0313315475610122,
-0.0121319224740286));
#26563=CARTESIAN_POINT('Ctrl Pts',(-0.0112355000002229,-0.0313287743898623,
-0.012175877030283));
#26564=CARTESIAN_POINT('Ctrl Pts',(-0.0112355053752281,-0.0313107142276789,
-0.0124621292562503));
#26565=CARTESIAN_POINT('Ctrl Pts',(-0.0113369647137236,-0.0312926540654955,
-0.0127490161444656));
#26566=CARTESIAN_POINT('Ctrl Pts',(-0.0115174412457287,-0.031274593903312,
-0.0129718046320591));
#26567=CARTESIAN_POINT('Ctrl Pts',(-0.0115451537494544,-0.0312718207321621,
-0.0130060142144567));
#26568=CARTESIAN_POINT('Ctrl Pts',(-0.0115746362548937,-0.0312690475610122,
-0.0130387521283998));
#26569=CARTESIAN_POINT('Ctrl Pts',(-0.0116057133619614,-0.0312662743898623,
-0.0130698396729341));
#26570=CARTESIAN_POINT('Ctrl Pts',(-0.0118081398225887,-0.0312482108288182,
-0.0132723341199225));
#26571=CARTESIAN_POINT('Ctrl Pts',(-0.0120827843608681,-0.0312301472677741,
-0.0134035029559604));
#26572=CARTESIAN_POINT('Ctrl Pts',(-0.0123679789827087,-0.0312120837067301,
-0.0134334425283192));
#26573=CARTESIAN_POINT('Ctrl Pts',(-0.0124117092393669,-0.0312093139344408,
-0.0134380333062765));
#26574=CARTESIAN_POINT('Ctrl Pts',(-0.0124556499210143,-0.0312065441621516,
-0.0134403376404914));
#26575=CARTESIAN_POINT('Ctrl Pts',(-0.0124995516363092,-0.0312037743898623,
-0.0134403532070682));
#26576=CARTESIAN_POINT('Ctrl Pts',(-0.012784809576339,-0.0311857773814931,
-0.0134404543532215));
#26577=CARTESIAN_POINT('Ctrl Pts',(-0.0130708314094809,-0.031167780373124,
-0.0133397732383392));
#26578=CARTESIAN_POINT('Ctrl Pts',(-0.0132932810111053,-0.0311497833647548,
-0.0131605692290612));
#26579=CARTESIAN_POINT('Ctrl Pts',(-0.0133283390243824,-0.0311469470397906,
-0.0131323267125959));
#26580=CARTESIAN_POINT('Ctrl Pts',(-0.0133618598559568,-0.0311441107148265,
-0.0131022318210814));
#26581=CARTESIAN_POINT('Ctrl Pts',(-0.0133936524376684,-0.0311412743898623,
-0.0130704736365666));
#26582=CARTESIAN_POINT('Ctrl Pts',(-0.0135991676372248,-0.0311229396759248,
-0.0128651807890925));
#26583=CARTESIAN_POINT('Ctrl Pts',(-0.0137311837108138,-0.0311046049619872,
-0.0125858251007971));
#26584=CARTESIAN_POINT('Ctrl Pts',(-0.013758806849294,-0.0310862702480498,
-0.0122957097263953));
#26585=CARTESIAN_POINT('Ctrl Pts',(-0.0137625712772429,-0.0310837716286539,
-0.0122561733636258));
#26586=CARTESIAN_POINT('Ctrl Pts',(-0.0137644707703676,-0.0310812730092581,
-0.012216467811213));
#26587=CARTESIAN_POINT('Ctrl Pts',(-0.0137644996649794,-0.0310787743898623,
-0.0121767737576019));
#26588=CARTESIAN_POINT('Ctrl Pts',(-0.0137644996042272,-0.0311412743898623,
-0.0121768537410499));
#26589=CARTESIAN_POINT('Ctrl Pts',(-0.0137642691544413,-0.0311596061323621,
-0.0124681250237667));
#26590=CARTESIAN_POINT('Ctrl Pts',(-0.0136591858638433,-0.031177937874862,
-0.0127588019995018));
#26591=CARTESIAN_POINT('Ctrl Pts',(-0.0134736095695228,-0.0311962696173618,
-0.0129827266695208));
#26592=CARTESIAN_POINT('Ctrl Pts',(-0.0134482953225914,-0.0311987702290807,
-0.0130132719738746));
#26593=CARTESIAN_POINT('Ctrl Pts',(-0.0134215560483623,-0.0312012708407996,
-0.013042608617474));
#26594=CARTESIAN_POINT('Ctrl Pts',(-0.0133935178974578,-0.0312037714525185,
-0.0130706080110064));
#26595=CARTESIAN_POINT('Ctrl Pts',(-0.0131917596414352,-0.0312217654729198,
-0.0132720873748926));
#26596=CARTESIAN_POINT('Ctrl Pts',(-0.0129182358167704,-0.031239759493321,
-0.0134029176620471));
#26597=CARTESIAN_POINT('Ctrl Pts',(-0.0126341062951139,-0.0312577535137223,
-0.0134332218688007));
#26598=CARTESIAN_POINT('Ctrl Pts',(-0.0125892883827257,-0.0312605918475397,
-0.0134380019820229));
#26599=CARTESIAN_POINT('Ctrl Pts',(-0.0125442468058514,-0.0312634301813572,
-0.0134403797057756));
#26600=CARTESIAN_POINT('Ctrl Pts',(-0.0124992513169962,-0.0312662685151747,
-0.0134403530649186));
#26601=CARTESIAN_POINT('Ctrl Pts',(-0.0122129410176822,-0.0312843290858119,
-0.0134401835467751));
#26602=CARTESIAN_POINT('Ctrl Pts',(-0.0119260660550254,-0.0313023896564492,
-0.013338520601838));
#26603=CARTESIAN_POINT('Ctrl Pts',(-0.0117033644410345,-0.0313204502270865,
-0.0131578573782969));
#26604=CARTESIAN_POINT('Ctrl Pts',(-0.011669186081468,-0.0313232220106679,
-0.0131301307152342));
#26605=CARTESIAN_POINT('Ctrl Pts',(-0.0116364795416869,-0.0313259937942494,
-0.0131006362680639));
#26606=CARTESIAN_POINT('Ctrl Pts',(-0.0116054231994823,-0.0313287655778308,
-0.0130695493187611));
#26607=CARTESIAN_POINT('Ctrl Pts',(-0.0114031022707209,-0.0313468227535544,
-0.0128670289957348));
#26608=CARTESIAN_POINT('Ctrl Pts',(-0.0112721235294321,-0.031364879929278,
-0.0125923604050326));
#26609=CARTESIAN_POINT('Ctrl Pts',(-0.0112423410495547,-0.0313829371050016,
-0.0123072085847569));
#26610=CARTESIAN_POINT('Ctrl Pts',(-0.0112377638277925,-0.0313857122834967,
-0.0122633840569576));
#26611=CARTESIAN_POINT('Ctrl Pts',(-0.0112354828095669,-0.0313884874619919,
-0.0122193496457451));
#26612=CARTESIAN_POINT('Ctrl Pts',(-0.0112355000976358,-0.031391262640487,
-0.0121753563750721));
#26613=CARTESIAN_POINT('Ctrl Pts',(-0.011235612585427,-0.0314093198162106,
-0.0118891066002938));
#26614=CARTESIAN_POINT('Ctrl Pts',(-0.0113371776611666,-0.0314273769919342,
-0.0116022594903848));
#26615=CARTESIAN_POINT('Ctrl Pts',(-0.0115177352388894,-0.0314454341676578,
-0.0113795391594196));
#26616=CARTESIAN_POINT('Ctrl Pts',(-0.011545484844614,-0.0314482093461529,
-0.0113453096274937));
#26617=CARTESIAN_POINT('Ctrl Pts',(-0.0115750070352552,-0.031450984524648,
-0.0113125550224318));
#26618=CARTESIAN_POINT('Ctrl Pts',(-0.0116061258684813,-0.0314537597031431,
-0.0112814544454353));
#26619=CARTESIAN_POINT('Ctrl Pts',(-0.0118086439719538,-0.0314718202737804,
-0.0110790551515912));
#26620=CARTESIAN_POINT('Ctrl Pts',(-0.0120833465317326,-0.0314898808444177,
-0.0109480131716259));
#26621=CARTESIAN_POINT('Ctrl Pts',(-0.0123685528079687,-0.031507941415055,
-0.0109182039372929));
#26622=CARTESIAN_POINT('Ctrl Pts',(-0.0124123238542812,-0.0315107131986364,
-0.0109136290682061));
#26623=CARTESIAN_POINT('Ctrl Pts',(-0.0124563046506386,-0.0315134849822179,
-0.0109113447918782));
#26624=CARTESIAN_POINT('Ctrl Pts',(-0.0125002451399487,-0.0315162567657993,
-0.0109113533103199));
#26625=CARTESIAN_POINT('Ctrl Pts',(-0.0127855004774802,-0.0315342507862006,
-0.0109114086108182));
#26626=CARTESIAN_POINT('Ctrl Pts',(-0.0130714651086127,-0.0315522448066019,
-0.0110122448522433));
#26627=CARTESIAN_POINT('Ctrl Pts',(-0.0132938157207033,-0.0315702388270031,
-0.0111915683422639));
#26628=CARTESIAN_POINT('Ctrl Pts',(-0.0133288887753934,-0.0315730771608206,
-0.0112198544014457));
#26629=CARTESIAN_POINT('Ctrl Pts',(-0.0133624209683958,-0.031575915494638,
-0.0112499952146683));
#26630=CARTESIAN_POINT('Ctrl Pts',(-0.0133942208462703,-0.0315787538284555,
-0.0112818010911603));
#26631=CARTESIAN_POINT('Ctrl Pts',(-0.0135996044305191,-0.0315970855709553,
-0.0114872234182486));
#26632=CARTESIAN_POINT('Ctrl Pts',(-0.013731442931389,-0.0316154173134552,
-0.0117666614940349));
#26633=CARTESIAN_POINT('Ctrl Pts',(-0.0137588824248632,-0.031633749055955,
-0.0120567932581251));
#26634=CARTESIAN_POINT('Ctrl Pts',(-0.0137626254143222,-0.0316362496676739,
-0.0120963697953423));
#26635=CARTESIAN_POINT('Ctrl Pts',(-0.0137644997916104,-0.0316387502793927,
-0.012136114664894));
#26636=CARTESIAN_POINT('Ctrl Pts',(-0.0137644999999826,-0.0316412508911116,
-0.0121758466549596));
#26637=CARTESIAN_POINT('Origin',(-0.0125,-0.0412787743898723,-0.0121758532865581));
#26638=CARTESIAN_POINT('',(-0.0137644997244071,-0.0321413104439873,-0.0121752554129869));
#26639=CARTESIAN_POINT('',(-0.0137644999999678,-0.0320788036733635,-0.0121758442670768));
#26640=CARTESIAN_POINT('',(-0.0137645,-0.0412787743898723,-0.0121758532865581));
#26641=CARTESIAN_POINT('Ctrl Pts',(-0.0137644999101415,-0.0320787743898623,
-0.0121753765769045));
#26642=CARTESIAN_POINT('Ctrl Pts',(-0.0137643901026805,-0.0320604452955693,
-0.011884105939584));
#26643=CARTESIAN_POINT('Ctrl Pts',(-0.0136594276941949,-0.0320421162012764,
-0.0115933860367519));
#26644=CARTESIAN_POINT('Ctrl Pts',(-0.0134739449447686,-0.0320237871069834,
-0.0113693847536569));
#26645=CARTESIAN_POINT('Ctrl Pts',(-0.0134486290285339,-0.0320212854305892,
-0.0113388115723943));
#26646=CARTESIAN_POINT('Ctrl Pts',(-0.0134218859628255,-0.0320187837541949,
-0.0113094478347642));
#26647=CARTESIAN_POINT('Ctrl Pts',(-0.0133938420641875,-0.0320162820778007,
-0.0112814223980658));
#26648=CARTESIAN_POINT('Ctrl Pts',(-0.0131921579459829,-0.0319982906992082,
-0.0110798710531277));
#26649=CARTESIAN_POINT('Ctrl Pts',(-0.0129186831052984,-0.0319802993206158,
-0.01094894174627));
#26650=CARTESIAN_POINT('Ctrl Pts',(-0.0126345659150311,-0.0319623079420234,
-0.0109185338106444));
#26651=CARTESIAN_POINT('Ctrl Pts',(-0.012589726654944,-0.0319594685499286,
-0.0109137348425392));
#26652=CARTESIAN_POINT('Ctrl Pts',(-0.0125446626218893,-0.0319566291578338,
-0.0109113406619024));
#26653=CARTESIAN_POINT('Ctrl Pts',(-0.0124996439863367,-0.031953789765739,
-0.010911353336675));
#26654=CARTESIAN_POINT('Ctrl Pts',(-0.0122133351285606,-0.0319357318415605,
-0.010911433945508));
#26655=CARTESIAN_POINT('Ctrl Pts',(-0.0119264297054606,-0.0319176739173819,
-0.0110130068215275));
#26656=CARTESIAN_POINT('Ctrl Pts',(-0.0117036723726936,-0.0318996159932033,
-0.0111935994700785));
#26657=CARTESIAN_POINT('Ctrl Pts',(-0.0116694673396937,-0.0318968431466947,
-0.0112213299938127));
#26658=CARTESIAN_POINT('Ctrl Pts',(-0.0116367351231188,-0.031894070300186,
-0.0112508306247152));
#26659=CARTESIAN_POINT('Ctrl Pts',(-0.0116056544324338,-0.0318912974536774,
-0.0112819258533877));
#26660=CARTESIAN_POINT('Ctrl Pts',(-0.0114032821352834,-0.0318732429219011,
-0.0114843928101436));
#26661=CARTESIAN_POINT('Ctrl Pts',(-0.0112722324208137,-0.0318551883901249,
-0.0117590260799309));
#26662=CARTESIAN_POINT('Ctrl Pts',(-0.0112423754584874,-0.0318371338583486,
-0.0120441689572507));
#26663=CARTESIAN_POINT('Ctrl Pts',(-0.0112377843640408,-0.0318343576194376,
-0.0120880152757821));
#26664=CARTESIAN_POINT('Ctrl Pts',(-0.0112354918306623,-0.0318315813805267,
-0.01213207229806));
#26665=CARTESIAN_POINT('Ctrl Pts',(-0.0112355000218958,-0.0318288051416157,
-0.0121760886042277));
#26666=CARTESIAN_POINT('Ctrl Pts',(-0.0112355532914055,-0.0318107506098395,
-0.0124623369509536));
#26667=CARTESIAN_POINT('Ctrl Pts',(-0.0113370580676153,-0.0317926960780632,
-0.012749203999261));
#26668=CARTESIAN_POINT('Ctrl Pts',(-0.0115175681933444,-0.031774641546287,
-0.0129719613164581));
#26669=CARTESIAN_POINT('Ctrl Pts',(-0.0115453251709876,-0.031771865307376,
-0.0130062146296634));
#26670=CARTESIAN_POINT('Ctrl Pts',(-0.0115748569046832,-0.0317690890684651,
-0.01303899183759));
#26671=CARTESIAN_POINT('Ctrl Pts',(-0.0116059872059909,-0.0317663128295541,
-0.0130701135250502));
#26672=CARTESIAN_POINT('Ctrl Pts',(-0.011808472884889,-0.0317482549053755,
-0.0132725431755552));
#26673=CARTESIAN_POINT('Ctrl Pts',(-0.0120831536604284,-0.031730196981197,
-0.0134036276597726));
#26674=CARTESIAN_POINT('Ctrl Pts',(-0.0123683540459796,-0.0317121390570185,
-0.0134334818457082));
#26675=CARTESIAN_POINT('Ctrl Pts',(-0.012412147390415,-0.0317093662105098,
-0.0134380660423424));
#26676=CARTESIAN_POINT('Ctrl Pts',(-0.012456151066559,-0.0317065933640011,
-0.0134403572664768));
#26677=CARTESIAN_POINT('Ctrl Pts',(-0.0125001146216738,-0.0317038205174925,
-0.0134403532813631));
#26678=CARTESIAN_POINT('Ctrl Pts',(-0.0127853684075842,-0.0316858291389,
-0.0134403274242919));
#26679=CARTESIAN_POINT('Ctrl Pts',(-0.0130713422901893,-0.0316678377603076,
-0.0133395217256917));
#26680=CARTESIAN_POINT('Ctrl Pts',(-0.0132937110097133,-0.0316498463817151,
-0.0131602226700011));
#26681=CARTESIAN_POINT('Ctrl Pts',(-0.0133288051511152,-0.0316470069896203,
-0.0131319257655304));
#26682=CARTESIAN_POINT('Ctrl Pts',(-0.0133623570364164,-0.0316441675975256,
-0.0131017720295453));
#26683=CARTESIAN_POINT('Ctrl Pts',(-0.0133941749012707,-0.0316413282054308,
-0.013069951433261));
#26684=CARTESIAN_POINT('Ctrl Pts',(-0.0135995683889091,-0.0316229991111379,
-0.012864540313455));
#26685=CARTESIAN_POINT('Ctrl Pts',(-0.0137314212509396,-0.0316046700168449,
-0.0125851098820988));
#26686=CARTESIAN_POINT('Ctrl Pts',(-0.0137588760985249,-0.0315863409225519,
-0.012294980187646));
#26687=CARTESIAN_POINT('Ctrl Pts',(-0.0137626233182736,-0.0315838392461577,
-0.0122553813620694));
#26688=CARTESIAN_POINT('Ctrl Pts',(-0.0137644998090151,-0.0315813375697634,
-0.0122156139127346));
#26689=CARTESIAN_POINT('Ctrl Pts',(-0.0137644999999854,-0.0315788358933692,
-0.0121758593608812));
#26690=CARTESIAN_POINT('Ctrl Pts',(-0.0137644999474453,-0.0316412743898623,
-0.0121762178558267));
#26691=CARTESIAN_POINT('Ctrl Pts',(-0.0137644159704943,-0.0316596082582658,
-0.012467489938709));
#26692=CARTESIAN_POINT('Ctrl Pts',(-0.0136594783866661,-0.0316779421266695,
-0.0127582202982457));
#26693=CARTESIAN_POINT('Ctrl Pts',(-0.0134740139348575,-0.031696275995073,
-0.0129822384951919));
#26694=CARTESIAN_POINT('Ctrl Pts',(-0.0134487294786364,-0.0316987754600028,
-0.0130127790016781));
#26695=CARTESIAN_POINT('Ctrl Pts',(-0.0134220210203026,-0.0317012749249325,
-0.0130421129465654));
#26696=CARTESIAN_POINT('Ctrl Pts',(-0.0133940144252717,-0.0317037743898623,
-0.0130701118942361));
#26697=CARTESIAN_POINT('Ctrl Pts',(-0.0131923669146546,-0.0317217705397123,
-0.0132717043438519));
#26698=CARTESIAN_POINT('Ctrl Pts',(-0.0129189141847026,-0.0317397666895621,
-0.0134026865273691));
#26699=CARTESIAN_POINT('Ctrl Pts',(-0.0126348001866975,-0.031757762839412,
-0.0134331476672289));
#26700=CARTESIAN_POINT('Ctrl Pts',(-0.0125900081867821,-0.0317606000228954,
-0.013437950019044));
#26701=CARTESIAN_POINT('Ctrl Pts',(-0.0125449914289418,-0.0317634372063788,
-0.0134403526020235));
#26702=CARTESIAN_POINT('Ctrl Pts',(-0.012500019243202,-0.0317662743898623,
-0.0134403532864117));
#26703=CARTESIAN_POINT('Ctrl Pts',(-0.0122137074025703,-0.0317843370926638,
-0.0134403576435145));
#26704=CARTESIAN_POINT('Ctrl Pts',(-0.0119267696495195,-0.0318023997954653,
-0.0133388679488294));
#26705=CARTESIAN_POINT('Ctrl Pts',(-0.0117039579848907,-0.0318204624982669,
-0.01315833858425));
#26706=CARTESIAN_POINT('Ctrl Pts',(-0.0116697809955634,-0.0318232331287987,
-0.0131306472594858));
#26707=CARTESIAN_POINT('Ctrl Pts',(-0.0116370731965135,-0.0318260037593305,
-0.0131011891364016));
#26708=CARTESIAN_POINT('Ctrl Pts',(-0.0116060127928554,-0.0318287743898623,
-0.0130701391041029));
#26709=CARTESIAN_POINT('Ctrl Pts',(-0.0114035573189597,-0.0318468336953203,
-0.0128677512319839));
#26710=CARTESIAN_POINT('Ctrl Pts',(-0.0112723973787259,-0.0318648930007784,
-0.0125931676450612));
#26711=CARTESIAN_POINT('Ctrl Pts',(-0.0112424275638582,-0.0318829523062364,
-0.0123080342907011));
#26712=CARTESIAN_POINT('Ctrl Pts',(-0.0112378240035466,-0.0318857263341117,
-0.0122642359356089));
#26713=CARTESIAN_POINT('Ctrl Pts',(-0.0112355140795679,-0.031888500361987,
-0.0122202264115989));
#26714=CARTESIAN_POINT('Ctrl Pts',(-0.0112355000642364,-0.0318912743898623,
-0.012176256342229));
#26715=CARTESIAN_POINT('Ctrl Pts',(-0.0112354088224881,-0.031909333695321,
-0.0118900051041403));
#26716=CARTESIAN_POINT('Ctrl Pts',(-0.0113367706805386,-0.0319273930007799,
-0.011603084706141));
#26717=CARTESIAN_POINT('Ctrl Pts',(-0.0115171710811969,-0.0319454523062386,
-0.0113802355602822));
#26718=CARTESIAN_POINT('Ctrl Pts',(-0.0115448817670342,-0.0319482263341132,
-0.0113460044685137));
#26719=CARTESIAN_POINT('Ctrl Pts',(-0.0115743642075006,-0.0319510003619877,
-0.0113132454868955));
#26720=CARTESIAN_POINT('Ctrl Pts',(-0.0116054428725726,-0.0319537743898623,
-0.0112821375623097));
#26721=CARTESIAN_POINT('Ctrl Pts',(-0.0118078073461992,-0.0319718370926638,
-0.0110795825693637));
#26722=CARTESIAN_POINT('Ctrl Pts',(-0.0120824111931275,-0.0319898997954653,
-0.010948330687204));
#26723=CARTESIAN_POINT('Ctrl Pts',(-0.0123675958891875,-0.0320079624982668,
-0.0109183043207361));
#26724=CARTESIAN_POINT('Ctrl Pts',(-0.0124113402520771,-0.0320107331287986,
-0.0109136985887695));
#26725=CARTESIAN_POINT('Ctrl Pts',(-0.0124552958852648,-0.0320135037593305,
-0.0109113808600401));
#26726=CARTESIAN_POINT('Ctrl Pts',(-0.0124992131318974,-0.0320162743898623,
-0.0109113535313827));
#26727=CARTESIAN_POINT('Ctrl Pts',(-0.0127844699867276,-0.0320342705397125,
-0.0109111760228311));
#26728=CARTESIAN_POINT('Ctrl Pts',(-0.0130705179832772,-0.0320522666895627,
-0.0110117798761921));
#26729=CARTESIAN_POINT('Ctrl Pts',(-0.0132930152789238,-0.0320702628394128,
-0.0111909233309809));
#26730=CARTESIAN_POINT('Ctrl Pts',(-0.0133280930959852,-0.032073100022896,
-0.011219166197109));
#26731=CARTESIAN_POINT('Ctrl Pts',(-0.0133616331609475,-0.0320759372063791,
-0.0112492631415283));
#26732=CARTESIAN_POINT('Ctrl Pts',(-0.0133934441590142,-0.0320787743898623,
-0.0112810249316635));
#26733=CARTESIAN_POINT('Ctrl Pts',(-0.0135990067022201,-0.0320971082582658,
-0.0114862694934108));
#26734=CARTESIAN_POINT('Ctrl Pts',(-0.0137310878026323,-0.0321154421266692,
-0.0117655938573517));
#26735=CARTESIAN_POINT('Ctrl Pts',(-0.0137587787741663,-0.0321337759950726,
-0.012055702349365));
#26736=CARTESIAN_POINT('Ctrl Pts',(-0.0137625538973809,-0.0321362754600025,
-0.0120952529769626));
#26737=CARTESIAN_POINT('Ctrl Pts',(-0.0137644626950543,-0.0321387749249324,
-0.012134973360974));
#26738=CARTESIAN_POINT('Ctrl Pts',(-0.013764499458089,-0.0321412743898623,
-0.0121746826060963));
#26739=CARTESIAN_POINT('Origin',(-0.0125,-0.0412787743898723,-0.0121758532865581));
#26740=CARTESIAN_POINT('',(-0.0137644999963171,-0.0326412702050577,-0.012175922879839));
#26741=CARTESIAN_POINT('',(-0.013764499952579,-0.0325787109363731,-0.0121759694420946));
#26742=CARTESIAN_POINT('',(-0.0137645,-0.0412787743898723,-0.0121758532865581));
#26743=CARTESIAN_POINT('Ctrl Pts',(-0.0137644999999542,-0.0325787043142338,
-0.012175864048403));
#26744=CARTESIAN_POINT('Ctrl Pts',(-0.0137645024788849,-0.0325603935516432,
-0.0118845935557882));
#26745=CARTESIAN_POINT('Ctrl Pts',(-0.0136596522608517,-0.0325420806179084,
-0.0115938333359118));
#26746=CARTESIAN_POINT('Ctrl Pts',(-0.013448947159338,-0.0325212608798433,
-0.0113391718965068));
#26747=CARTESIAN_POINT('Ctrl Pts',(-0.0134222101122967,-0.0325187599996857,
-0.0113097925285742));
#26748=CARTESIAN_POINT('Ctrl Pts',(-0.0131925610498707,-0.0324982758277494,
-0.0110801256275606));
#26749=CARTESIAN_POINT('Ctrl Pts',(-0.0129191339088165,-0.0324802863335813,
-0.0109490955450475));
#26750=CARTESIAN_POINT('Ctrl Pts',(-0.012590183010145,-0.0324594626929304,
-0.0109137671230538));
#26751=CARTESIAN_POINT('Ctrl Pts',(-0.0125451129513083,-0.0324566240194546,
-0.0109113564037182));
#26752=CARTESIAN_POINT('Ctrl Pts',(-0.0122137837892425,-0.0324357362376009,
-0.0109113334877237));
#26753=CARTESIAN_POINT('Ctrl Pts',(-0.0119268474756361,-0.0324176933911951,
-0.0110128022239468));
#26754=CARTESIAN_POINT('Ctrl Pts',(-0.0116698041003138,-0.0323968396734784,
-0.0112210365037981));
#26755=CARTESIAN_POINT('Ctrl Pts',(-0.0116370522931408,-0.0323940622327908,
-0.011250534140304));
#26756=CARTESIAN_POINT('Ctrl Pts',(-0.0114035049818775,-0.0323731976062524,
-0.0114840349847706));
#26757=CARTESIAN_POINT('Ctrl Pts',(-0.0112723614861413,-0.0323550709023229,
-0.0117586372462776));
#26758=CARTESIAN_POINT('Ctrl Pts',(-0.01123781175723,-0.0323342853331126,
-0.0120876245901732));
#26759=CARTESIAN_POINT('Ctrl Pts',(-0.0112355057241986,-0.0323315180760419,
-0.012131676815311));
#26760=CARTESIAN_POINT('Ctrl Pts',(-0.0112354628440165,-0.032310773620894,
-0.012461989545241));
#26761=CARTESIAN_POINT('Ctrl Pts',(-0.0113369123537346,-0.0322929275911575,
-0.0127489399162024));
#26762=CARTESIAN_POINT('Ctrl Pts',(-0.0115451460559283,-0.0322722716324522,
-0.013006006497036));
#26763=CARTESIAN_POINT('Ctrl Pts',(-0.0115746430676899,-0.0322695200073974,
-0.0130387605517719));
#26764=CARTESIAN_POINT('Ctrl Pts',(-0.0118081008913406,-0.0322488442021525,
-0.0132722847039332));
#26765=CARTESIAN_POINT('Ctrl Pts',(-0.0120826511136037,-0.0322308326812266,
-0.0134034390928158));
#26766=CARTESIAN_POINT('Ctrl Pts',(-0.0124116737763742,-0.0322100048075982,
-0.013438037243111));
#26767=CARTESIAN_POINT('Ctrl Pts',(-0.0124557985794072,-0.0322072241920666,
-0.0134403492115628));
#26768=CARTESIAN_POINT('Ctrl Pts',(-0.0127851468318433,-0.0321864457028237,
-0.013440379614818));
#26769=CARTESIAN_POINT('Ctrl Pts',(-0.0130711473210704,-0.0321684202301248,
-0.013339619647662));
#26770=CARTESIAN_POINT('Ctrl Pts',(-0.0133286756983239,-0.0321474987910244,
-0.0131320394832236));
#26771=CARTESIAN_POINT('Ctrl Pts',(-0.0133622552364703,-0.0321446443052363,
-0.0131018683857812));
#26772=CARTESIAN_POINT('Ctrl Pts',(-0.0135995104230382,-0.0321233679731723,
-0.0128646334078737));
#26773=CARTESIAN_POINT('Ctrl Pts',(-0.0137313874371309,-0.0321049007542866,
-0.012585212686444));
#26774=CARTESIAN_POINT('Ctrl Pts',(-0.0137626205171119,-0.0320838633766418,
-0.0122554456853946));
#26775=CARTESIAN_POINT('Ctrl Pts',(-0.0137645002838139,-0.0320813339055445,
-0.0122156385036423));
#26776=CARTESIAN_POINT('Ctrl Pts',(-0.0137644999999678,-0.0320788036733635,
-0.0121758442670768));
#26777=CARTESIAN_POINT('Ctrl Pts',(-0.0137644999999896,-0.0321413477523234,
-0.012175848146052));
#26778=CARTESIAN_POINT('Ctrl Pts',(-0.0137645011763883,-0.0321595625621079,
-0.012465227487546));
#26779=CARTESIAN_POINT('Ctrl Pts',(-0.013663043056052,-0.0321767871020658,
-0.0127350696305296));
#26780=CARTESIAN_POINT('Ctrl Pts',(-0.0135072112013381,-0.0321930214076091,
-0.012940370026662));
#26781=CARTESIAN_POINT('Ctrl Pts',(-0.013496896303629,-0.0321940959966356,
-0.012953959370058));
#26782=CARTESIAN_POINT('Ctrl Pts',(-0.0134863491201398,-0.0321951662470044,
-0.0129672835872208));
#26783=CARTESIAN_POINT('Ctrl Pts',(-0.0134755850392324,-0.0321962321587258,
-0.0129803370223949));
#26784=CARTESIAN_POINT('Ctrl Pts',(-0.0133022030885797,-0.0322134012839923,
-0.0131905946442644));
#26785=CARTESIAN_POINT('Ctrl Pts',(-0.0130732963736853,-0.0322294447466978,
-0.0133276013131048));
#26786=CARTESIAN_POINT('Ctrl Pts',(-0.0128451691284769,-0.0322443624180834,
-0.0133923312036394));
#26787=CARTESIAN_POINT('Ctrl Pts',(-0.0126170418832684,-0.0322592800894691,
-0.013457061094174));
#26788=CARTESIAN_POINT('Ctrl Pts',(-0.0123906040206081,-0.0322730719695349,
-0.0134516000849701));
#26789=CARTESIAN_POINT('Ctrl Pts',(-0.0121952022194095,-0.0322857385303962,
-0.0134030690634071));
#26790=CARTESIAN_POINT('Ctrl Pts',(-0.0119998004182109,-0.0322984050912574,
-0.0133545380418441));
#26791=CARTESIAN_POINT('Ctrl Pts',(-0.0118352558919743,-0.0323099463329141,
-0.0132641994845881));
#26792=CARTESIAN_POINT('Ctrl Pts',(-0.0117063400195007,-0.0323203604956642,
-0.0131602638133983));
#26793=CARTESIAN_POINT('Ctrl Pts',(-0.0115774241470271,-0.0323307746584143,
-0.0130563281422085));
#26794=CARTESIAN_POINT('Ctrl Pts',(-0.011483731425446,-0.032340061742258,
-0.0129394138527007));
#26795=CARTESIAN_POINT('Ctrl Pts',(-0.0114167366022701,-0.0323482283138874,
-0.0128281574036222));
#26796=CARTESIAN_POINT('Ctrl Pts',(-0.0113497417790943,-0.0323563948855168,
-0.0127169009545437));
#26797=CARTESIAN_POINT('Ctrl Pts',(-0.0113092033223697,-0.032363440944932,
-0.01261149502709));
#26798=CARTESIAN_POINT('Ctrl Pts',(-0.0112835578380688,-0.0323693419850658,
-0.0125211484018958));
#26799=CARTESIAN_POINT('Ctrl Pts',(-0.0112707350959183,-0.0323722925051327,
-0.0124759750892987));
#26800=CARTESIAN_POINT('Ctrl Pts',(-0.0112616568978935,-0.0323749567703793,
-0.0124345685527524));
#26801=CARTESIAN_POINT('Ctrl Pts',(-0.0112549627958923,-0.0323773660155132,
-0.0123968569299392));
#26802=CARTESIAN_POINT('Ctrl Pts',(-0.0112482686938912,-0.0323797752606472,
-0.012359145307126));
#26803=CARTESIAN_POINT('Ctrl Pts',(-0.0112440228544091,-0.0323819294856686,
-0.0123251081982629));
#26804=CARTESIAN_POINT('Ctrl Pts',(-0.0112413201089934,-0.0323837015091994,
-0.0122970357191774));
#26805=CARTESIAN_POINT('Ctrl Pts',(-0.0112386173635777,-0.0323854735327302,
-0.012268963240092));
#26806=CARTESIAN_POINT('Ctrl Pts',(-0.0112372750835179,-0.0323868633547704,
-0.0122468834046135));
#26807=CARTESIAN_POINT('Ctrl Pts',(-0.0112363886520364,-0.0323883484661244,
-0.0122232517179404));
#26808=CARTESIAN_POINT('Ctrl Pts',(-0.0112359454362956,-0.0323890910218015,
-0.0122114358746039));
#26809=CARTESIAN_POINT('Ctrl Pts',(-0.0112357127140258,-0.0323898573998069,
-0.0121992251218495));
#26810=CARTESIAN_POINT('Ctrl Pts',(-0.0112356659453741,-0.0323900387433015,
-0.0121963386060175));
#26811=CARTESIAN_POINT('Ctrl Pts',(-0.0112356542532112,-0.0323900840791751,
-0.0121956169770595));
#26812=CARTESIAN_POINT('Ctrl Pts',(-0.0112356522835067,-0.0323900928503918,
-0.0121954780672));
#26813=CARTESIAN_POINT('Ctrl Pts',(-0.0112356496095871,-0.0323901037947021,
-0.0121953042572958));
#26814=CARTESIAN_POINT('Ctrl Pts',(-0.0112356415878281,-0.0323901366276331,
-0.0121947828275831));
#26815=CARTESIAN_POINT('Ctrl Pts',(-0.0112355037950207,-0.0323901890184068,
-0.0121939554867409));
#26816=CARTESIAN_POINT('Ctrl Pts',(-0.0112355000282024,-0.0323913068862882,
-0.0121761203516306));
#26817=CARTESIAN_POINT('Ctrl Pts',(-0.0112354950057779,-0.0323927973767968,
-0.0121523401714834));
#26818=CARTESIAN_POINT('Ctrl Pts',(-0.0112370398539334,-0.0323961820488304,
-0.0120982736572059));
#26819=CARTESIAN_POINT('Ctrl Pts',(-0.0112415429565992,-0.0323990751630377,
-0.0120523781072101));
#26820=CARTESIAN_POINT('Ctrl Pts',(-0.0112460460592651,-0.0324019682772451,
-0.0120064825572144));
#26821=CARTESIAN_POINT('Ctrl Pts',(-0.0112519691979474,-0.0324043698336261,
-0.0119685882970341));
#26822=CARTESIAN_POINT('Ctrl Pts',(-0.0112597084231613,-0.0324068590142232,
-0.0119296073639056));
#26823=CARTESIAN_POINT('Ctrl Pts',(-0.0112751868735891,-0.0324118373754174,
-0.0118516454976486));
#26824=CARTESIAN_POINT('Ctrl Pts',(-0.0112995326251591,-0.0324171662334758,
-0.011769813820212));
#26825=CARTESIAN_POINT('Ctrl Pts',(-0.0113315921296918,-0.0324224324680165,
-0.0116923418610448));
#26826=CARTESIAN_POINT('Ctrl Pts',(-0.0113957111387573,-0.0324329649370979,
-0.0115373979427105));
#26827=CARTESIAN_POINT('Ctrl Pts',(-0.0114889334793173,-0.0324432469121083,
-0.0113987138484009));
#26828=CARTESIAN_POINT('Ctrl Pts',(-0.0116056067900746,-0.0324536023812925,
-0.011281973520572));
#26829=CARTESIAN_POINT('Ctrl Pts',(-0.0117222801008318,-0.0324639578504768,
-0.0111652331927431));
#26830=CARTESIAN_POINT('Ctrl Pts',(-0.0118627766610855,-0.0324743868138348,
-0.0110711577771328));
#26831=CARTESIAN_POINT('Ctrl Pts',(-0.012015817714252,-0.0324848029688212,
-0.0110077232577651));
#26832=CARTESIAN_POINT('Ctrl Pts',(-0.0121688587674185,-0.0324952191238075,
-0.0109442887383975));
#26833=CARTESIAN_POINT('Ctrl Pts',(-0.0123343565668412,-0.0325056224704221,
-0.010911384850466));
#26834=CARTESIAN_POINT('Ctrl Pts',(-0.0124997588698091,-0.0325160342306024,
-0.0109113533095489));
#26835=CARTESIAN_POINT('Ctrl Pts',(-0.0127867621774742,-0.0325341005425989,
-0.0109112985802775));
#26836=CARTESIAN_POINT('Ctrl Pts',(-0.0130739461331377,-0.0325521921866719,
-0.0110131918049057));
#26837=CARTESIAN_POINT('Ctrl Pts',(-0.0132966463397878,-0.0325702980756418,
-0.0111938579406919));
#26838=CARTESIAN_POINT('Ctrl Pts',(-0.0133306339556649,-0.0325730613240854,
-0.0112214304845951));
#26839=CARTESIAN_POINT('Ctrl Pts',(-0.0133631604934758,-0.0325758249043161,
-0.0112507465619568));
#26840=CARTESIAN_POINT('Ctrl Pts',(-0.0133940522332139,-0.0325785887769225,
-0.0112816324780967));
#26841=CARTESIAN_POINT('Ctrl Pts',(-0.0135978692208023,-0.032596824207931,
-0.0114854110428495));
#26842=CARTESIAN_POINT('Ctrl Pts',(-0.0137295669170478,-0.0326150723662705,
-0.0117624467162534));
#26843=CARTESIAN_POINT('Ctrl Pts',(-0.0137582680854385,-0.0326333370250046,
-0.0120504671821971));
#26844=CARTESIAN_POINT('Ctrl Pts',(-0.013762420756471,-0.0326359796741892,
-0.012092139849644));
#26845=CARTESIAN_POINT('Ctrl Pts',(-0.0137645000903062,-0.0326386226687959,
-0.0121340072957658));
#26846=CARTESIAN_POINT('Ctrl Pts',(-0.0137644999999971,-0.032641266020253,
-0.0121758560153365));
#26847=CARTESIAN_POINT('Origin',(-0.0125,-0.0412787743898723,-0.0121758532865581));
#26848=CARTESIAN_POINT('',(-0.0137644997766436,-0.0331412349785624,-0.012176354624468));
#26849=CARTESIAN_POINT('',(-0.0137644999997312,-0.0330787743898623,-0.0121758793595363));
#26850=CARTESIAN_POINT('',(-0.0137645,-0.0412787743898723,-0.0121758532865581));
#26851=CARTESIAN_POINT('Ctrl Pts',(-0.0137644999999999,-0.0330787727022437,
-0.0121758527106564));
#26852=CARTESIAN_POINT('Ctrl Pts',(-0.0137644998673437,-0.0330604398739191,
-0.0118845811735839));
#26853=CARTESIAN_POINT('Ctrl Pts',(-0.0136596463479785,-0.0330421070455945,
-0.0115938210656056));
#26854=CARTESIAN_POINT('Ctrl Pts',(-0.0134742469976217,-0.0330237742172699,
-0.0113697496718626));
#26855=CARTESIAN_POINT('Ctrl Pts',(-0.0134489601755792,-0.0330212737825786,
-0.0113391883271358));
#26856=CARTESIAN_POINT('Ctrl Pts',(-0.0134222477406572,-0.0330187733478873,
-0.0113098342031574));
#26857=CARTESIAN_POINT('Ctrl Pts',(-0.0133942356918425,-0.033016272913196,
-0.0112818159397795));
#26858=CARTESIAN_POINT('Ctrl Pts',(-0.0131926389430079,-0.032998277817308,
-0.0110801744660571));
#26859=CARTESIAN_POINT('Ctrl Pts',(-0.0129192198486113,-0.03298028272142,
-0.010949124685627));
#26860=CARTESIAN_POINT('Ctrl Pts',(-0.0126351144353285,-0.032962287625532,
-0.0109185926376209));
#26861=CARTESIAN_POINT('Ctrl Pts',(-0.012590305635762,-0.0329594494584041,
-0.0109137771559177));
#26862=CARTESIAN_POINT('Ctrl Pts',(-0.0125452712982326,-0.0329566112912762,
-0.0109113633184062));
#26863=CARTESIAN_POINT('Ctrl Pts',(-0.0125002810781795,-0.0329537731241484,
-0.0109113533177977));
#26864=CARTESIAN_POINT('Ctrl Pts',(-0.0122139703982751,-0.0329357114752144,
-0.010911289675499));
#26865=CARTESIAN_POINT('Ctrl Pts',(-0.0119270124904289,-0.0329176498262805,
-0.0110127191898094));
#26866=CARTESIAN_POINT('Ctrl Pts',(-0.0117041637398992,-0.0328995881773465,
-0.01119320131505));
#26867=CARTESIAN_POINT('Ctrl Pts',(-0.0116699669322119,-0.0328968165632646,
-0.0112208968372963));
#26868=CARTESIAN_POINT('Ctrl Pts',(-0.0116372401521535,-0.0328940449491827,
-0.0112503609161892));
#26869=CARTESIAN_POINT('Ctrl Pts',(-0.0116061618569985,-0.0328912733351008,
-0.0112814184794784));
#26870=CARTESIAN_POINT('Ctrl Pts',(-0.0114036734472617,-0.0328732150817423,
-0.0114837718122265));
#26871=CARTESIAN_POINT('Ctrl Pts',(-0.0112724678069508,-0.0328551568283838,
-0.0117583324226996));
#26872=CARTESIAN_POINT('Ctrl Pts',(-0.0112424499134969,-0.0328370985750254,
-0.0120434598201938));
#26873=CARTESIAN_POINT('Ctrl Pts',(-0.0112378370673606,-0.0328343235653679,
-0.0120872753136389));
#26874=CARTESIAN_POINT('Ctrl Pts',(-0.0112355197009196,-0.0328315485557105,
-0.0121313025356128));
#26875=CARTESIAN_POINT('Ctrl Pts',(-0.0112355001252145,-0.032828773546053,
-0.0121752905543113));
#26876=CARTESIAN_POINT('Ctrl Pts',(-0.0112353727371744,-0.0328107152926946,
-0.0124615406523085));
#26877=CARTESIAN_POINT('Ctrl Pts',(-0.0113366976187793,-0.0327926570393361,
-0.0127484730157758));
#26878=CARTESIAN_POINT('Ctrl Pts',(-0.0115170688076744,-0.0327745987859777,
-0.0129713446574436));
#26879=CARTESIAN_POINT('Ctrl Pts',(-0.0115447864269355,-0.0327718237763202,
-0.0130055933162549));
#26880=CARTESIAN_POINT('Ctrl Pts',(-0.0115742774409676,-0.0327690487666628,
-0.0130383688860161));
#26881=CARTESIAN_POINT('Ctrl Pts',(-0.0116053661220587,-0.0327662737570053,
-0.0130694921814366));
#26882=CARTESIAN_POINT('Ctrl Pts',(-0.0118077123885585,-0.0327482121080714,
-0.0132720637415188));
#26883=CARTESIAN_POINT('Ctrl Pts',(-0.0120823038219357,-0.0327301504591375,
-0.0134033391389739));
#26884=CARTESIAN_POINT('Ctrl Pts',(-0.0123674849516029,-0.0327120888102036,
-0.0134333905670982));
#26885=CARTESIAN_POINT('Ctrl Pts',(-0.0124112468494109,-0.0327093171961216,
-0.0134380020486787));
#26886=CARTESIAN_POINT('Ctrl Pts',(-0.0124552203917516,-0.0327065455820396,
-0.0134403236663119));
#26887=CARTESIAN_POINT('Ctrl Pts',(-0.0124991556137138,-0.0327037739679577,
-0.0134403530046331));
#26888=CARTESIAN_POINT('Ctrl Pts',(-0.0127844112476858,-0.0326857788720697,
-0.0134405434878273));
#26889=CARTESIAN_POINT('Ctrl Pts',(-0.0130704629193013,-0.0326677837761816,
-0.0133399534447622));
#26890=CARTESIAN_POINT('Ctrl Pts',(-0.0132929680502495,-0.0326497886802936,
-0.0131608212663846));
#26891=CARTESIAN_POINT('Ctrl Pts',(-0.0133280613196807,-0.0326469505131657,
-0.0131325687322843));
#26892=CARTESIAN_POINT('Ctrl Pts',(-0.0133616156871987,-0.0326441123460379,
-0.0131024605546831));
#26893=CARTESIAN_POINT('Ctrl Pts',(-0.0133934396024196,-0.03264127417891,
-0.0130706861909757));
#26894=CARTESIAN_POINT('Ctrl Pts',(-0.0135990026817153,-0.0326229413505854,
-0.0128654431842294));
#26895=CARTESIAN_POINT('Ctrl Pts',(-0.0137310852050748,-0.0326046085222609,
-0.0125861201701978));
#26896=CARTESIAN_POINT('Ctrl Pts',(-0.0137587780000869,-0.0325862756939363,
-0.0122960123332303));
#26897=CARTESIAN_POINT('Ctrl Pts',(-0.0137625550509665,-0.032583775259245,
-0.0122564442051196));
#26898=CARTESIAN_POINT('Ctrl Pts',(-0.013764464121777,-0.0325812748245536,
-0.0122167061575427));
#26899=CARTESIAN_POINT('Ctrl Pts',(-0.0137644994986291,-0.0325787743898623,
-0.0121769793268418));
#26900=CARTESIAN_POINT('Ctrl Pts',(-0.0137644999926371,-0.0326412743898623,
-0.0121759897443414));
#26901=CARTESIAN_POINT('Ctrl Pts',(-0.0137644685603842,-0.0326596023068526,
-0.0124672599279237));
#26902=CARTESIAN_POINT('Ctrl Pts',(-0.0136595846977029,-0.032677930223843,
-0.0127580076853526));
#26903=CARTESIAN_POINT('Ctrl Pts',(-0.0134741627452126,-0.0326962581408333,
-0.0129820587168547));
#26904=CARTESIAN_POINT('Ctrl Pts',(-0.0134488456013029,-0.0326987605980978,
-0.0130126501982381));
#26905=CARTESIAN_POINT('Ctrl Pts',(-0.0134220999108933,-0.0327012630553624,
-0.0130420317130972));
#26906=CARTESIAN_POINT('Ctrl Pts',(-0.0133940521006994,-0.0327037655126269,
-0.0130700742275089));
#26907=CARTESIAN_POINT('Ctrl Pts',(-0.0131924160601591,-0.0327217557076172,
-0.0132716721966082));
#26908=CARTESIAN_POINT('Ctrl Pts',(-0.0129189730052593,-0.0327397459026075,
-0.0134026656693521));
#26909=CARTESIAN_POINT('Ctrl Pts',(-0.0126348638437601,-0.0327577360975978,
-0.0134331408406388));
#26910=CARTESIAN_POINT('Ctrl Pts',(-0.0125900104694752,-0.0327605762768623,
-0.0134379520697344));
#26911=CARTESIAN_POINT('Ctrl Pts',(-0.0125449315998565,-0.0327634164561269,
-0.0134403569263869));
#26912=CARTESIAN_POINT('Ctrl Pts',(-0.0124998976816101,-0.0327662566353914,
-0.0134403532824185));
#26913=CARTESIAN_POINT('Ctrl Pts',(-0.0122135897910585,-0.0327843133749709,
-0.0134403301155047));
#26914=CARTESIAN_POINT('Ctrl Pts',(-0.0119266647188268,-0.0328023701145505,
-0.0133388154499535));
#26915=CARTESIAN_POINT('Ctrl Pts',(-0.0117038714045645,-0.03282042685413,
-0.0131582684276924));
#26916=CARTESIAN_POINT('Ctrl Pts',(-0.0116696488773386,-0.0328232004888053,
-0.0131305352104486));
#26917=CARTESIAN_POINT('Ctrl Pts',(-0.0116368998322642,-0.0328259741234807,
-0.0131010303575405));
#26918=CARTESIAN_POINT('Ctrl Pts',(-0.0116058031972925,-0.032828747758156,
-0.0130699295294075));
#26919=CARTESIAN_POINT('Ctrl Pts',(-0.0114033978839815,-0.032846801106886,
-0.0128674969231715));
#26920=CARTESIAN_POINT('Ctrl Pts',(-0.0112723025246776,-0.0328648544556159,
-0.0125928864066233));
#26921=CARTESIAN_POINT('Ctrl Pts',(-0.0112423976430418,-0.0328829078043458,
-0.012307749312932));
#26922=CARTESIAN_POINT('Ctrl Pts',(-0.0112377975757155,-0.0328856848298707,
-0.0122638885866408));
#26923=CARTESIAN_POINT('Ctrl Pts',(-0.0112354976277577,-0.0328884618553957,
-0.012219816624342));
#26924=CARTESIAN_POINT('Ctrl Pts',(-0.011235500001838,-0.0328912388809206,
-0.0121757851075616));
#26925=CARTESIAN_POINT('Ctrl Pts',(-0.011235515435654,-0.0329092922296505,
-0.0118895377106938));
#26926=CARTESIAN_POINT('Ctrl Pts',(-0.0113369816624679,-0.0329273455783804,
-0.011602657952783));
#26927=CARTESIAN_POINT('Ctrl Pts',(-0.0115174614365488,-0.0329453989271104,
-0.0113798770172314));
#26928=CARTESIAN_POINT('Ctrl Pts',(-0.011545223429454,-0.0329481759526353,
-0.0113456081204329));
#26929=CARTESIAN_POINT('Ctrl Pts',(-0.0115747616064416,-0.0329509529781602,
-0.0113128161149497));
#26930=CARTESIAN_POINT('Ctrl Pts',(-0.0116058996156524,-0.0329537300036851,
-0.0112816806227456));
#26931=CARTESIAN_POINT('Ctrl Pts',(-0.0118083647778547,-0.0329717867432646,
-0.0110792318265923));
#26932=CARTESIAN_POINT('Ctrl Pts',(-0.0120830317457008,-0.0329898434828442,
-0.0109481204941999));
#26933=CARTESIAN_POINT('Ctrl Pts',(-0.0123682283698876,-0.0330079002224237,
-0.0109182378892694));
#26934=CARTESIAN_POINT('Ctrl Pts',(-0.0124120364584216,-0.033010673857099,
-0.010913647723428));
#26935=CARTESIAN_POINT('Ctrl Pts',(-0.0124560552530744,-0.0330134474917744,
-0.010911352103133));
#26936=CARTESIAN_POINT('Ctrl Pts',(-0.012500034039603,-0.0330162211264497,
-0.0109113532870163));
#26937=CARTESIAN_POINT('Ctrl Pts',(-0.0127852867991391,-0.03303421132144,
-0.0109113609658543));
#26938=CARTESIAN_POINT('Ctrl Pts',(-0.0130712663423404,-0.0330522015164303,
-0.0110121477627849));
#26939=CARTESIAN_POINT('Ctrl Pts',(-0.0132936462228542,-0.0330701917114207,
-0.0111914316680687));
#26940=CARTESIAN_POINT('Ctrl Pts',(-0.013328754165032,-0.0330730318906852,
-0.0112197358877021));
#26941=CARTESIAN_POINT('Ctrl Pts',(-0.0133623189218372,-0.0330758720699498,
-0.0112498983046016));
#26942=CARTESIAN_POINT('Ctrl Pts',(-0.0133941485242657,-0.0330787122492143,
-0.011281728761364));
#26943=CARTESIAN_POINT('Ctrl Pts',(-0.0135995476405913,-0.0330970401662046,
-0.0114871333907787));
#26944=CARTESIAN_POINT('Ctrl Pts',(-0.0137314087469587,-0.0331153680831949,
-0.0117665593582989));
#26945=CARTESIAN_POINT('Ctrl Pts',(-0.0137588724472994,-0.0331336960001852,
-0.0120566878073691));
#26946=CARTESIAN_POINT('Ctrl Pts',(-0.0137626222862181,-0.0331361984574497,
-0.0120963013676778));
#26947=CARTESIAN_POINT('Ctrl Pts',(-0.0137644999968615,-0.0331387009147143,
-0.0121360837360722));
#26948=CARTESIAN_POINT('Ctrl Pts',(-0.0137645,-0.0331412033719788,-0.0121758531867676));
#26949=CARTESIAN_POINT('Origin',(-0.0125,-0.0412787743898723,-0.0121758532865581));
#26950=CARTESIAN_POINT('',(-0.0137644017347287,-0.0336414716603326,-0.012175630710863));
#26951=CARTESIAN_POINT('',(-0.0137644996589709,-0.0335787980895467,-0.0121750921833385));
#26952=CARTESIAN_POINT('',(-0.0137645,-0.0412787743898723,-0.0121758532865581));
#26953=CARTESIAN_POINT('Ctrl Pts',(-0.0137644994877345,-0.0335787743898623,
-0.0121747150778228));
#26954=CARTESIAN_POINT('Ctrl Pts',(-0.0137642373067409,-0.0335604414094987,
-0.0118834436073164));
#26955=CARTESIAN_POINT('Ctrl Pts',(-0.0136591222073282,-0.033542108429135,
-0.0115927779094656));
#26956=CARTESIAN_POINT('Ctrl Pts',(-0.013473521285526,-0.0335237754487713,
-0.0113688733880304));
#26957=CARTESIAN_POINT('Ctrl Pts',(-0.0134482080082087,-0.0335212750958016,
-0.0113383360545481));
#26958=CARTESIAN_POINT('Ctrl Pts',(-0.0134214703210877,-0.033518774742832,
-0.0113090071252378));
#26959=CARTESIAN_POINT('Ctrl Pts',(-0.0133934343230916,-0.0335162743898623,
-0.0112810151110639));
#26960=CARTESIAN_POINT('Ctrl Pts',(-0.0131916569149418,-0.0334982791416907,
-0.0110795542581383));
#26961=CARTESIAN_POINT('Ctrl Pts',(-0.0129181204047335,-0.0334802838935192,
-0.0109487494930919));
#26962=CARTESIAN_POINT('Ctrl Pts',(-0.0126339876547543,-0.0334622886453476,
-0.0109184720562332));
#26963=CARTESIAN_POINT('Ctrl Pts',(-0.0125891762170904,-0.0334594505601858,
-0.0109136969098464));
#26964=CARTESIAN_POINT('Ctrl Pts',(-0.0125441414103058,-0.0334566124750241,
-0.0109113234307162));
#26965=CARTESIAN_POINT('Ctrl Pts',(-0.0124991528616412,-0.0334537743898623,
-0.0109113535703238));
#26966=CARTESIAN_POINT('Ctrl Pts',(-0.0122128421325712,-0.0334357125884496,
-0.0109115453812021));
#26967=CARTESIAN_POINT('Ctrl Pts',(-0.0119259747580602,-0.0334176507870369,
-0.0110132309561064));
#26968=CARTESIAN_POINT('Ctrl Pts',(-0.011703287099886,-0.0333995889856242,
-0.0111939119416744));
#26969=CARTESIAN_POINT('Ctrl Pts',(-0.0116691163137691,-0.0333968174537036,
-0.0112216369236687));
#26970=CARTESIAN_POINT('Ctrl Pts',(-0.0116364170215967,-0.0333940459217829,
-0.0112511290160514));
#26971=CARTESIAN_POINT('Ctrl Pts',(-0.0116053675044745,-0.0333912743898623,
-0.0112822130077267));
#26972=CARTESIAN_POINT('Ctrl Pts',(-0.0114030588925162,-0.0333732159841984,
-0.0114847462447237));
#26973=CARTESIAN_POINT('Ctrl Pts',(-0.0112720972453575,-0.0333551575785346,
-0.0117594234255462));
#26974=CARTESIAN_POINT('Ctrl Pts',(-0.011242332750728,-0.0333370991728707,
-0.0120445774696354));
#26975=CARTESIAN_POINT('Ctrl Pts',(-0.0112377590180712,-0.0333343242452012,
-0.0120883953936389));
#26976=CARTESIAN_POINT('Ctrl Pts',(-0.0112354807791195,-0.0333315493175318,
-0.0121324229903591));
#26977=CARTESIAN_POINT('Ctrl Pts',(-0.0112355001222663,-0.0333287743898623,
-0.0121764093544956));
#26978=CARTESIAN_POINT('Ctrl Pts',(-0.0112356260017247,-0.0333107159841984,
-0.0124626595569768));
#26979=CARTESIAN_POINT('Ctrl Pts',(-0.0113372047834033,-0.0332926575785346,
-0.0127495022348612));
#26980=CARTESIAN_POINT('Ctrl Pts',(-0.0115177731919476,-0.0332745991728708,
-0.0129722142270512));
#26981=CARTESIAN_POINT('Ctrl Pts',(-0.0115455200640928,-0.0332718242452013,
-0.0130064370527511));
#26982=CARTESIAN_POINT('Ctrl Pts',(-0.0115750388929873,-0.0332690493175318,
-0.0130391853319111));
#26983=CARTESIAN_POINT('Ctrl Pts',(-0.011606153812779,-0.0332662743898623,
-0.0130702800547121));
#26984=CARTESIAN_POINT('Ctrl Pts',(-0.0118086785518679,-0.0332482125884496,
-0.0132726733330642));
#26985=CARTESIAN_POINT('Ctrl Pts',(-0.0120833856444131,-0.0332301507870369,
-0.0134037067560259));
#26986=CARTESIAN_POINT('Ctrl Pts',(-0.0123685932311997,-0.0332120889856242,
-0.0134335068601281));
#26987=CARTESIAN_POINT('Ctrl Pts',(-0.0124123575220764,-0.0332093174537036,
-0.0134380796011228));
#26988=CARTESIAN_POINT('Ctrl Pts',(-0.012456331423678,-0.0332065459217829,
-0.0134403624658187));
#26989=CARTESIAN_POINT('Ctrl Pts',(-0.0125002649974867,-0.0332037743898623,
-0.0134403532587907));
#26990=CARTESIAN_POINT('Ctrl Pts',(-0.0127855208005565,-0.0331857791416907,
-0.0134402934785831));
#26991=CARTESIAN_POINT('Ctrl Pts',(-0.0130714841943955,-0.0331677838935192,
-0.0133394524388388));
#26992=CARTESIAN_POINT('Ctrl Pts',(-0.0132938321104615,-0.0331497886453476,
-0.0131601250124551));
#26993=CARTESIAN_POINT('Ctrl Pts',(-0.0133288992745993,-0.0331469505601858,
-0.0131318427402095));
#26994=CARTESIAN_POINT('Ctrl Pts',(-0.0133624260233035,-0.0331441124750241,
-0.0131017063130526));
#26995=CARTESIAN_POINT('Ctrl Pts',(-0.0133942209933907,-0.0331412743898623,
-0.0130699053348077));
#26996=CARTESIAN_POINT('Ctrl Pts',(-0.0135996047394909,-0.0331229414094986,
-0.0128644827782311));
#26997=CARTESIAN_POINT('Ctrl Pts',(-0.0137314431939203,-0.0331046084291349,
-0.0125850444201865));
#26998=CARTESIAN_POINT('Ctrl Pts',(-0.0137588825062962,-0.0330862754487713,
-0.0122949124539553));
#26999=CARTESIAN_POINT('Ctrl Pts',(-0.0137626248310478,-0.0330837750958016,
-0.0122553426563026));
#27000=CARTESIAN_POINT('Ctrl Pts',(-0.0137644991806288,-0.033081274742832,
-0.0122156045851513));
#27001=CARTESIAN_POINT('Ctrl Pts',(-0.0137644999997312,-0.0330787743898623,
-0.0121758793595363));
#27002=CARTESIAN_POINT('Ctrl Pts',(-0.013764499498133,-0.0331412743898623,
-0.0121769798838072));
#27003=CARTESIAN_POINT('Ctrl Pts',(-0.0137642399910612,-0.0331596088050655,
-0.012468252175019));
#27004=CARTESIAN_POINT('Ctrl Pts',(-0.0136591270148841,-0.0331779432202687,
-0.012758919492331));
#27005=CARTESIAN_POINT('Ctrl Pts',(-0.0134735272558264,-0.0331962776354719,
-0.0129828259826037));
#27006=CARTESIAN_POINT('Ctrl Pts',(-0.0134482306429966,-0.033198776553602,
-0.0130133436719761));
#27007=CARTESIAN_POINT('Ctrl Pts',(-0.0134215114608746,-0.0332012754717322,
-0.0130426545398078));
#27008=CARTESIAN_POINT('Ctrl Pts',(-0.0133934955569117,-0.0332037743898623,
-0.0130706303201139));
#27009=CARTESIAN_POINT('Ctrl Pts',(-0.0131917306594618,-0.0332217710949099,
-0.0132721062550693));
#27010=CARTESIAN_POINT('Ctrl Pts',(-0.0129182013201166,-0.0332397677999575,
-0.0134029298366984));
#27011=CARTESIAN_POINT('Ctrl Pts',(-0.0126340691208629,-0.0332577645050051,
-0.0134332258331134));
#27012=CARTESIAN_POINT('Ctrl Pts',(-0.0125892843988171,-0.0332606011332908,
-0.0134380010672548));
#27013=CARTESIAN_POINT('Ctrl Pts',(-0.012544276414023,-0.0332634377615766,
-0.0134403774816797));
#27014=CARTESIAN_POINT('Ctrl Pts',(-0.0124993143156266,-0.0332662743898624,
-0.0134403531006494));
#27015=CARTESIAN_POINT('Ctrl Pts',(-0.0122130018722459,-0.0332843376476823,
-0.0134401978456101));
#27016=CARTESIAN_POINT('Ctrl Pts',(-0.0119261202647265,-0.0333024009055021,
-0.0133385477790772));
#27017=CARTESIAN_POINT('Ctrl Pts',(-0.0117034091133121,-0.033320464163322,
-0.0131578936163031));
#27018=CARTESIAN_POINT('Ctrl Pts',(-0.0116692554344324,-0.0333232342388354,
-0.0131301895510847));
#27019=CARTESIAN_POINT('Ctrl Pts',(-0.0116365712576102,-0.0333260043143489,
-0.0131007203188604));
#27020=CARTESIAN_POINT('Ctrl Pts',(-0.0116055345699018,-0.0333287743898623,
-0.0130696607850493));
#27021=CARTESIAN_POINT('Ctrl Pts',(-0.0114031869384003,-0.033346834249358,
-0.0128671642054773));
#27022=CARTESIAN_POINT('Ctrl Pts',(-0.0112721738559381,-0.0333648941088535,
-0.0125925098791858));
#27023=CARTESIAN_POINT('Ctrl Pts',(-0.011242356873197,-0.0333829539683491,
-0.0123073599997148));
#27024=CARTESIAN_POINT('Ctrl Pts',(-0.0112377778441314,-0.0333857274421868,
-0.0122635691977578));
#27025=CARTESIAN_POINT('Ctrl Pts',(-0.0112354915142712,-0.0333885009160246,
-0.0122195685521193));
#27026=CARTESIAN_POINT('Ctrl Pts',(-0.0112355000236904,-0.0333912743898623,
-0.0121756085151439));
#27027=CARTESIAN_POINT('Ctrl Pts',(-0.0112355554339538,-0.0334093342493578,
-0.0118893566383836));
#27028=CARTESIAN_POINT('Ctrl Pts',(-0.0113370646897218,-0.0334273941088534,
-0.0116024877429456));
#27029=CARTESIAN_POINT('Ctrl Pts',(-0.0115175798344913,-0.0334454539683489,
-0.011379730891193));
#27030=CARTESIAN_POINT('Ctrl Pts',(-0.0115453017573263,-0.0334482274421867,
-0.0113455218597949));
#27031=CARTESIAN_POINT('Ctrl Pts',(-0.0115747938682146,-0.0334510009160245,
-0.0113127851735476));
#27032=CARTESIAN_POINT('Ctrl Pts',(-0.0116058806685998,-0.0334537743898623,
-0.0112816995686681));
#27033=CARTESIAN_POINT('Ctrl Pts',(-0.0118083447706616,-0.0334718376476825,
-0.0110792432527729));
#27034=CARTESIAN_POINT('Ctrl Pts',(-0.012083013501435,-0.0334899009055026,
-0.0109481258335134));
#27035=CARTESIAN_POINT('Ctrl Pts',(-0.0123682134196918,-0.0335079641633228,
-0.0109182394558252));
#27036=CARTESIAN_POINT('Ctrl Pts',(-0.0124119500101667,-0.033510734238836,
-0.0109136562558379));
#27037=CARTESIAN_POINT('Ctrl Pts',(-0.0124558966516803,-0.0335135043143491,
-0.0109113601123901));
#27038=CARTESIAN_POINT('Ctrl Pts',(-0.0124998038584254,-0.0335162743898623,
-0.0109113533017702));
#27039=CARTESIAN_POINT('Ctrl Pts',(-0.0127850614427392,-0.0335342710949099,
-0.0109113090543425));
#27040=CARTESIAN_POINT('Ctrl Pts',(-0.0130710629130146,-0.0335522677999575,
-0.0110120469742265));
#27041=CARTESIAN_POINT('Ctrl Pts',(-0.0132934766700397,-0.0335702645050051,
-0.0111912949977287));
#27042=CARTESIAN_POINT('Ctrl Pts',(-0.0133285333736225,-0.0335731011332908,
-0.0112195479480487));
#27043=CARTESIAN_POINT('Ctrl Pts',(-0.0133620521491485,-0.0335759377615766,
-0.0112496534229335));
#27044=CARTESIAN_POINT('Ctrl Pts',(-0.0133938418969691,-0.0335787743898624,
-0.0112814222309576));
#27045=CARTESIAN_POINT('Ctrl Pts',(-0.0135993134558177,-0.0335971088050655,
-0.0114867584464037));
#27046=CARTESIAN_POINT('Ctrl Pts',(-0.0137312703595708,-0.0336154432202687,
-0.0117661418824352));
#27047=CARTESIAN_POINT('Ctrl Pts',(-0.0137588321571824,-0.033633777635472,
-0.0120562629439565));
#27048=CARTESIAN_POINT('Ctrl Pts',(-0.0137625887359981,-0.0336362765536021,
-0.0120958054530865));
#27049=CARTESIAN_POINT('Ctrl Pts',(-0.0137644798389691,-0.0336387754717322,
-0.0121355168034981));
#27050=CARTESIAN_POINT('Ctrl Pts',(-0.0137644998395261,-0.0336412743898623,
-0.0121752162320185));
#27051=CARTESIAN_POINT('Origin',(-0.0125,-0.0412787743898723,-0.0121758532865581));
#27052=CARTESIAN_POINT('',(-0.0137644998637729,-0.0341412999856959,-0.0121754316468409));
#27053=CARTESIAN_POINT('',(-0.013764499925554,-0.0340787743898623,-0.0121762871919379));
#27054=CARTESIAN_POINT('',(-0.0137645,-0.0412787743898723,-0.0121758532865581));
#27055=CARTESIAN_POINT('Ctrl Pts',(-0.0137644999999728,-0.0340787477436506,
-0.0121758615870606));
#27056=CARTESIAN_POINT('Ctrl Pts',(-0.0137645018988856,-0.0340606084504782,
-0.0118865808727149));
#27057=CARTESIAN_POINT('Ctrl Pts',(-0.0136610153723787,-0.0340424568279764,
-0.0115976083349243));
#27058=CARTESIAN_POINT('Ctrl Pts',(-0.0134779938396196,-0.0340242900869158,
-0.011374299607965));
#27059=CARTESIAN_POINT('Ctrl Pts',(-0.0134515698526924,-0.0340216672385489,
-0.0113420591016543));
#27060=CARTESIAN_POINT('Ctrl Pts',(-0.0134235693534653,-0.0340190440750426,
-0.0113111498801886));
#27061=CARTESIAN_POINT('Ctrl Pts',(-0.0133941409267945,-0.0340164205880029,
-0.0112817211637535));
#27062=CARTESIAN_POINT('Ctrl Pts',(-0.013191714932659,-0.0339983747040669,
-0.011079293176449));
#27063=CARTESIAN_POINT('Ctrl Pts',(-0.0129168426251142,-0.0339803135121575,
-0.0109479341169463));
#27064=CARTESIAN_POINT('Ctrl Pts',(-0.0126310167083062,-0.0339622452080805,
-0.0109181590184052));
#27065=CARTESIAN_POINT('Ctrl Pts',(-0.0125874794070605,-0.033959493025191,
-0.0109136236443941));
#27066=CARTESIAN_POINT('Ctrl Pts',(-0.0125437266583471,-0.0339567406772872,
-0.0109113534300671));
#27067=CARTESIAN_POINT('Ctrl Pts',(-0.01250000415023,-0.0339539881933339,
-0.0109113532865649));
#27068=CARTESIAN_POINT('Ctrl Pts',(-0.0123346219886952,-0.0339435768110642,
-0.0109113527437622));
#27069=CARTESIAN_POINT('Ctrl Pts',(-0.0121691218361513,-0.0339331634822505,
-0.0109442230135551));
#27070=CARTESIAN_POINT('Ctrl Pts',(-0.0120160996755066,-0.0339227325313663,
-0.0110076064265344));
#27071=CARTESIAN_POINT('Ctrl Pts',(-0.0118630775148619,-0.033912301580482,
-0.0110709898395137));
#27072=CARTESIAN_POINT('Ctrl Pts',(-0.0117226409181171,-0.033901853007527,
-0.0111649397020928));
#27073=CARTESIAN_POINT('Ctrl Pts',(-0.011605864942515,-0.0338914505596433,
-0.0112817152944248));
#27074=CARTESIAN_POINT('Ctrl Pts',(-0.0114890889669128,-0.0338810481117596,
-0.0113984908867567));
#27075=CARTESIAN_POINT('Ctrl Pts',(-0.0113956972487478,-0.0338706917889472,
-0.0115375785856883));
#27076=CARTESIAN_POINT('Ctrl Pts',(-0.0113317547281944,-0.0338601422781651,
-0.0116919491277582));
#27077=CARTESIAN_POINT('Ctrl Pts',(-0.0112997834679177,-0.033854867522774,
-0.0117691343987931));
#27078=CARTESIAN_POINT('Ctrl Pts',(-0.011275473578601,-0.0338495444703905,
-0.011850350325652));
#27079=CARTESIAN_POINT('Ctrl Pts',(-0.0112597971141385,-0.0338444782712676,
-0.0119291610655605));
#27080=CARTESIAN_POINT('Ctrl Pts',(-0.0112519588819072,-0.0338419451717062,
-0.0119685664355147));
#27081=CARTESIAN_POINT('Ctrl Pts',(-0.0112459846027741,-0.0338394762854599,
-0.0120072805204668));
#27082=CARTESIAN_POINT('Ctrl Pts',(-0.0112415889385475,-0.0338366438012794,
-0.0120519103544722));
#27083=CARTESIAN_POINT('Ctrl Pts',(-0.011237193274321,-0.0338338113170988,
-0.0120965401884777));
#27084=CARTESIAN_POINT('Ctrl Pts',(-0.0112355,-0.0338306152349841,-0.0121472179637786));
#27085=CARTESIAN_POINT('Ctrl Pts',(-0.0112355,-0.0338288076869315,-0.0121758532865581));
#27086=CARTESIAN_POINT('Ctrl Pts',(-0.0112355,-0.0338270001388788,-0.0122044886093376));
#27087=CARTESIAN_POINT('Ctrl Pts',(-0.0112359205269678,-0.0338265811248883,
-0.0122111179060965));
#27088=CARTESIAN_POINT('Ctrl Pts',(-0.0112364374006413,-0.0338257345815302,
-0.0122245339552262));
#27089=CARTESIAN_POINT('Ctrl Pts',(-0.0112369542743149,-0.033824888038172,
-0.0122379500043559));
#27090=CARTESIAN_POINT('Ctrl Pts',(-0.0112380215535703,-0.0338236139654462,
-0.0122581221936209));
#27091=CARTESIAN_POINT('Ctrl Pts',(-0.0112396320697024,-0.0338223557845349,
-0.0122779950031942));
#27092=CARTESIAN_POINT('Ctrl Pts',(-0.0112428531019667,-0.0338198394227122,
-0.0123177406223408));
#27093=CARTESIAN_POINT('Ctrl Pts',(-0.0112477128926463,-0.0338173866281474,
-0.0123563628814054));
#27094=CARTESIAN_POINT('Ctrl Pts',(-0.0112552843905968,-0.0338146811157623,
-0.0123986610550672));
#27095=CARTESIAN_POINT('Ctrl Pts',(-0.0112704273864978,-0.0338092700909921,
-0.0124832574023907));
#27096=CARTESIAN_POINT('Ctrl Pts',(-0.0112971842349235,-0.0338028481949406,
-0.012582311247989));
#27097=CARTESIAN_POINT('Ctrl Pts',(-0.0113432673161325,-0.033795663479089,
-0.0126866661173217));
#27098=CARTESIAN_POINT('Ctrl Pts',(-0.0113893503973415,-0.0337884787632373,
-0.0127910209866544));
#27099=CARTESIAN_POINT('Ctrl Pts',(-0.0114546927022284,-0.0337805312275854,
-0.0129009041684455));
#27100=CARTESIAN_POINT('Ctrl Pts',(-0.0115461452173229,-0.0337717547769112,
-0.0130059865912531));
#27101=CARTESIAN_POINT('Ctrl Pts',(-0.0116375977324173,-0.033762978326237,
-0.0131110690140608));
#27102=CARTESIAN_POINT('Ctrl Pts',(-0.0117547887102928,-0.0337533729605404,
-0.0132109764039506));
#27103=CARTESIAN_POINT('Ctrl Pts',(-0.0119018449572601,-0.0337429550092292,
-0.0132899317374963));
#27104=CARTESIAN_POINT('Ctrl Pts',(-0.0120983071384933,-0.0337290369779943,
-0.0133954133975296));
#27105=CARTESIAN_POINT('Ctrl Pts',(-0.012346185450533,-0.0337136686392474,
-0.0134590161788762));
#27106=CARTESIAN_POINT('Ctrl Pts',(-0.0126119809515327,-0.0336968458212211,
-0.0134353851505829));
#27107=CARTESIAN_POINT('Ctrl Pts',(-0.0127440929622223,-0.0336884841435156,
-0.0134236394940509));
#27108=CARTESIAN_POINT('Ctrl Pts',(-0.0128798762734508,-0.0336797631329847,
-0.0133904081463402));
#27109=CARTESIAN_POINT('Ctrl Pts',(-0.0130108174784532,-0.0336706822773521,
-0.013332583917996));
#27110=CARTESIAN_POINT('Ctrl Pts',(-0.0132080080623682,-0.0336570069852651,
-0.0132455036642943));
#27111=CARTESIAN_POINT('Ctrl Pts',(-0.0133984744886159,-0.0336425156084047,
-0.0130983842065243));
#27112=CARTESIAN_POINT('Ctrl Pts',(-0.0135377000870961,-0.0336272093131572,
-0.012898444996475));
#27113=CARTESIAN_POINT('Ctrl Pts',(-0.0136769256855764,-0.0336119030179097,
-0.0126985057864257));
#27114=CARTESIAN_POINT('Ctrl Pts',(-0.013764502164571,-0.033595781804275,
-0.0124452108403644));
#27115=CARTESIAN_POINT('Ctrl Pts',(-0.0137644999999592,-0.0335788452834579,
-0.0121758431251633));
#27116=CARTESIAN_POINT('Ctrl Pts',(-0.0137644999999694,-0.0336413152440371,
-0.0121758620877456));
#27117=CARTESIAN_POINT('Ctrl Pts',(-0.0137644979726606,-0.033659645947366,
-0.0124671332318196));
#27118=CARTESIAN_POINT('Ctrl Pts',(-0.0136596428238356,-0.0336779766506949,
-0.0127578923433247));
#27119=CARTESIAN_POINT('Ctrl Pts',(-0.013474242444834,-0.0336963073540238,
-0.0129819624036657));
#27120=CARTESIAN_POINT('Ctrl Pts',(-0.0134489475642251,-0.033698808281771,
-0.0130125331363409));
#27121=CARTESIAN_POINT('Ctrl Pts',(-0.0134222261882464,-0.0337013092095181,
-0.0130418958856302));
#27122=CARTESIAN_POINT('Ctrl Pts',(-0.0133942044369489,-0.0337038101372653,
-0.0130699218940714));
#27123=CARTESIAN_POINT('Ctrl Pts',(-0.0131926012515593,-0.0337218031240314,
-0.0132715557075881));
#27124=CARTESIAN_POINT('Ctrl Pts',(-0.0129191784313342,-0.0337397961107975,
-0.0134025958817728));
#27125=CARTESIAN_POINT('Ctrl Pts',(-0.0126350726820894,-0.0337577890975637,
-0.0134331184219027));
#27126=CARTESIAN_POINT('Ctrl Pts',(-0.0125902510424699,-0.0337606277418736,
-0.0134379337777961));
#27127=CARTESIAN_POINT('Ctrl Pts',(-0.0125452038176885,-0.0337634663861835,
-0.0134403461209176));
#27128=CARTESIAN_POINT('Ctrl Pts',(-0.0125002008930168,-0.0337663050304934,
-0.0134403532706));
#27129=CARTESIAN_POINT('Ctrl Pts',(-0.0122138910223444,-0.0337843645653168,
-0.0134403987570803));
#27130=CARTESIAN_POINT('Ctrl Pts',(-0.011926940148603,-0.03380242410014,
-0.0133389515838582));
#27131=CARTESIAN_POINT('Ctrl Pts',(-0.0117041030481573,-0.0338204836349634,
-0.0131584561015589));
#27132=CARTESIAN_POINT('Ctrl Pts',(-0.0116698980757059,-0.0338232557312161,
-0.0131307504682182));
#27133=CARTESIAN_POINT('Ctrl Pts',(-0.0116371640909388,-0.0338260278274689,
-0.0131012753468492));
#27134=CARTESIAN_POINT('Ctrl Pts',(-0.0116060796922359,-0.0338287999237216,
-0.0130702059761426));
#27135=CARTESIAN_POINT('Ctrl Pts',(-0.0114036104318054,-0.0338468560644724,
-0.0128678346010635));
#27136=CARTESIAN_POINT('Ctrl Pts',(-0.0112724300594571,-0.0338649122052232,
-0.0125932627217097));
#27137=CARTESIAN_POINT('Ctrl Pts',(-0.0112424379684191,-0.0338829683459741,
-0.012308133242432));
#27138=CARTESIAN_POINT('Ctrl Pts',(-0.0112378277496764,-0.0338857438362993,
-0.012264304712178));
#27139=CARTESIAN_POINT('Ctrl Pts',(-0.0112355143538179,-0.0338885193266245,
-0.012220264539437));
#27140=CARTESIAN_POINT('Ctrl Pts',(-0.0112355000666595,-0.0338912948169497,
-0.0121762638737737));
#27141=CARTESIAN_POINT('Ctrl Pts',(-0.0112354071205807,-0.0339093509577008,
-0.0118900145559006));
#27142=CARTESIAN_POINT('Ctrl Pts',(-0.0113367660008467,-0.0339274070984519,
-0.0116030949718573));
#27143=CARTESIAN_POINT('Ctrl Pts',(-0.0115171632508829,-0.033945463239203,
-0.0113802452331895));
#27144=CARTESIAN_POINT('Ctrl Pts',(-0.0115448929207517,-0.033948238729528,
-0.0113459900010152));
#27145=CARTESIAN_POINT('Ctrl Pts',(-0.0115743968327725,-0.0339510142198529,
-0.0113132089188103));
#27146=CARTESIAN_POINT('Ctrl Pts',(-0.0116054990823748,-0.0339537897101779,
-0.0112820813031262));
#27147=CARTESIAN_POINT('Ctrl Pts',(-0.0118078749129517,-0.0339718492450012,
-0.0110795404207626));
#27148=CARTESIAN_POINT('Ctrl Pts',(-0.0120824850703501,-0.0339899087798247,
-0.0109483059244207));
#27149=CARTESIAN_POINT('Ctrl Pts',(-0.0123676699728074,-0.034007968314648,
-0.0109182965228678));
#27150=CARTESIAN_POINT('Ctrl Pts',(-0.012411445186685,-0.0340107404109007,
-0.01091369015009));
#27151=CARTESIAN_POINT('Ctrl Pts',(-0.0124554318294686,-0.0340135125071533,
-0.0109113749966697));
#27152=CARTESIAN_POINT('Ctrl Pts',(-0.0124993797185969,-0.034016284603406,
-0.0109113534386929));
#27153=CARTESIAN_POINT('Ctrl Pts',(-0.0127846345277401,-0.0340342775901722,
-0.0109112135112319));
#27154=CARTESIAN_POINT('Ctrl Pts',(-0.0130706677330489,-0.0340522705769383,
-0.0110118536863371));
#27155=CARTESIAN_POINT('Ctrl Pts',(-0.013293140892811,-0.0340702635637044,
-0.0111910244820692));
#27156=CARTESIAN_POINT('Ctrl Pts',(-0.0133282391328796,-0.0340731022080143,
-0.0112192911709975));
#27157=CARTESIAN_POINT('Ctrl Pts',(-0.013361797272371,-0.0340759408523243,
-0.0112494142841308));
#27158=CARTESIAN_POINT('Ctrl Pts',(-0.0133936236345209,-0.0340787794966342,
-0.0112812041654912));
#27159=CARTESIAN_POINT('Ctrl Pts',(-0.0135991441361798,-0.034097110199963,
-0.0114864890904258));
#27160=CARTESIAN_POINT('Ctrl Pts',(-0.0137311692055575,-0.0341154409032919,
-0.0117658387884295));
#27161=CARTESIAN_POINT('Ctrl Pts',(-0.0137588025739744,-0.0341337716066208,
-0.0120559519531405));
#27162=CARTESIAN_POINT('Ctrl Pts',(-0.0137625726997891,-0.034136272534368,
-0.0120955331983566));
#27163=CARTESIAN_POINT('Ctrl Pts',(-0.0137644736441105,-0.0341387734621151,
-0.012135284086788));
#27164=CARTESIAN_POINT('Ctrl Pts',(-0.0137644997276158,-0.0341412743898623,
-0.0121750233109846));
#27165=CARTESIAN_POINT('Origin',(-0.0125,-0.0412787743898723,-0.0121758532865581));
#27166=CARTESIAN_POINT('',(-0.0137644998286153,-0.0346412456228672,-0.0121763255635047));
#27167=CARTESIAN_POINT('',(-0.0137644998230799,-0.0345787397706929,-0.0121762999529358));
#27168=CARTESIAN_POINT('',(-0.0137645,-0.0412787743898723,-0.0121758532865581));
#27169=CARTESIAN_POINT('Ctrl Pts',(-0.0137644999999884,-0.0345787112306013,
-0.0121758478627298));
#27170=CARTESIAN_POINT('Ctrl Pts',(-0.0137644987506394,-0.0345603823010006,
-0.0118845772640469));
#27171=CARTESIAN_POINT('Ctrl Pts',(-0.0136596447418225,-0.0345420533713999,
-0.0115938183088325));
#27172=CARTESIAN_POINT('Ctrl Pts',(-0.0134742455564904,-0.0345237244417992,
-0.0113697479301321));
#27173=CARTESIAN_POINT('Ctrl Pts',(-0.0134489398502257,-0.0345212226697025,
-0.0113391638734878));
#27174=CARTESIAN_POINT('Ctrl Pts',(-0.0134222064093296,-0.0345187208976057,
-0.0113097888422845));
#27175=CARTESIAN_POINT('Ctrl Pts',(-0.0133941715204833,-0.034516219125509,
-0.0112817517587904));
#27176=CARTESIAN_POINT('Ctrl Pts',(-0.0131925617618852,-0.0344982279120871,
-0.0110801262176284));
#27177=CARTESIAN_POINT('Ctrl Pts',(-0.0129191353045024,-0.0344802366986654,
-0.0109490961761));
#27178=CARTESIAN_POINT('Ctrl Pts',(-0.0126350294464768,-0.0344622454852435,
-0.0109185835070023));
#27179=CARTESIAN_POINT('Ctrl Pts',(-0.012590190044376,-0.0344594059969679,
-0.0109137678025732));
#27180=CARTESIAN_POINT('Ctrl Pts',(-0.012545124963572,-0.0344565665086922,
-0.0109113570081699));
#27181=CARTESIAN_POINT('Ctrl Pts',(-0.0125001044084758,-0.0344537270204166,
-0.0109113532908685));
#27182=CARTESIAN_POINT('Ctrl Pts',(-0.0122137956630281,-0.0344356692615957,
-0.0109113296506473));
#27183=CARTESIAN_POINT('Ctrl Pts',(-0.011926853365667,-0.0344176115027748,
-0.0110127979724812));
#27184=CARTESIAN_POINT('Ctrl Pts',(-0.0117040303222684,-0.0343995537439538,
-0.0111933093831462));
#27185=CARTESIAN_POINT('Ctrl Pts',(-0.0116698136967697,-0.0343967808010773,
-0.011221028649712));
#27186=CARTESIAN_POINT('Ctrl Pts',(-0.0116370693711646,-0.0343940078582007,
-0.0112505187143577));
#27187=CARTESIAN_POINT('Ctrl Pts',(-0.0116059761418116,-0.0343912349153242,
-0.0112816041093206));
#27188=CARTESIAN_POINT('Ctrl Pts',(-0.0114035310908213,-0.0343731805487076,
-0.0114839981513443));
#27189=CARTESIAN_POINT('Ctrl Pts',(-0.0112723825734531,-0.034355126182091,
-0.0117585841309941));
#27190=CARTESIAN_POINT('Ctrl Pts',(-0.011242422954328,-0.0343370718154744,
-0.0120437161449255));
#27191=CARTESIAN_POINT('Ctrl Pts',(-0.0112378158726534,-0.0343342954803935,
-0.0120875627128921));
#27192=CARTESIAN_POINT('Ctrl Pts',(-0.0112355074760351,-0.0343315191453126,
-0.0121316208304898));
#27193=CARTESIAN_POINT('Ctrl Pts',(-0.0112355000181491,-0.0343287428102318,
-0.0121756390457791));
#27194=CARTESIAN_POINT('Ctrl Pts',(-0.0112354515198935,-0.0343106884436152,
-0.0124618872735694));
#27195=CARTESIAN_POINT('Ctrl Pts',(-0.0113368542227572,-0.0342926340769986,
-0.0127487903025532));
#27196=CARTESIAN_POINT('Ctrl Pts',(-0.0115172850280278,-0.0342745797103819,
-0.0129716117510821));
#27197=CARTESIAN_POINT('Ctrl Pts',(-0.0115450310234966,-0.0342718033753011,
-0.0130058764260746));
#27198=CARTESIAN_POINT('Ctrl Pts',(-0.0115745524544448,-0.0342690270402203,
-0.0130386654988026));
#27199=CARTESIAN_POINT('Ctrl Pts',(-0.0116056731727549,-0.0342662507051395,
-0.0130697994684224));
#27200=CARTESIAN_POINT('Ctrl Pts',(-0.0118080876541539,-0.0342481929463185,
-0.0132723001386087));
#27201=CARTESIAN_POINT('Ctrl Pts',(-0.0120827222510488,-0.0342301351874976,
-0.0134034810829045));
#27202=CARTESIAN_POINT('Ctrl Pts',(-0.0123679120285065,-0.0342120774286767,
-0.0134334354977024));
#27203=CARTESIAN_POINT('Ctrl Pts',(-0.012411705667003,-0.0342093044858002,
-0.0134380352867437));
#27204=CARTESIAN_POINT('Ctrl Pts',(-0.0124557104613993,-0.0342065315429236,
-0.0134403419773165));
#27205=CARTESIAN_POINT('Ctrl Pts',(-0.0124996759269194,-0.0342037586000471,
-0.0134403532450305));
#27206=CARTESIAN_POINT('Ctrl Pts',(-0.0127849295756885,-0.0341857673866254,
-0.0134404263514217));
#27207=CARTESIAN_POINT('Ctrl Pts',(-0.0130709383179884,-0.0341677761732036,
-0.0133397199571894));
#27208=CARTESIAN_POINT('Ctrl Pts',(-0.0132933691953534,-0.0341497849597818,
-0.0131604981818703));
#27209=CARTESIAN_POINT('Ctrl Pts',(-0.0133284746578713,-0.0341469454715061,
-0.0131322122559665));
#27210=CARTESIAN_POINT('Ctrl Pts',(-0.0133620383771549,-0.0341441059832304,
-0.0131020688045103));
#27211=CARTESIAN_POINT('Ctrl Pts',(-0.0133938684987958,-0.0341412664949547,
-0.0130702577570638));
#27212=CARTESIAN_POINT('Ctrl Pts',(-0.0135993323014577,-0.034122937565354,
-0.0128649170785468));
#27213=CARTESIAN_POINT('Ctrl Pts',(-0.0137312808987023,-0.0341046086357533,
-0.0125855319131322));
#27214=CARTESIAN_POINT('Ctrl Pts',(-0.0137588351903264,-0.0340862797061526,
-0.0122954116973699));
#27215=CARTESIAN_POINT('Ctrl Pts',(-0.0137625961605212,-0.0340837779340558,
-0.0122558122948785));
#27216=CARTESIAN_POINT('Ctrl Pts',(-0.013764486283383,-0.034081276161959,
-0.0122160436113997));
#27217=CARTESIAN_POINT('Ctrl Pts',(-0.013764499925554,-0.0340787743898623,
-0.0121762871919379));
#27218=CARTESIAN_POINT('Ctrl Pts',(-0.01376449999993,-0.0341413255815296,
-0.0121758399826972));
#27219=CARTESIAN_POINT('Ctrl Pts',(-0.0137645030485197,-0.0341595105759365,
-0.0124656011047135));
#27220=CARTESIAN_POINT('Ctrl Pts',(-0.0136606891579716,-0.0341776961989851,
-0.012755005442436));
#27221=CARTESIAN_POINT('Ctrl Pts',(-0.0134770965549167,-0.0341959072895615,
-0.0129785005144048));
#27222=CARTESIAN_POINT('Ctrl Pts',(-0.0134509381871666,-0.0341985020150379,
-0.0130103442062835));
#27223=CARTESIAN_POINT('Ctrl Pts',(-0.0134232395263884,-0.0342010972575229,
-0.0130408863505521));
#27224=CARTESIAN_POINT('Ctrl Pts',(-0.0133941435802119,-0.0342036930888617,
-0.0130699827559113));
#27225=CARTESIAN_POINT('Ctrl Pts',(-0.0131915881066192,-0.0342217643295428,
-0.0132725414261682));
#27226=CARTESIAN_POINT('Ctrl Pts',(-0.0129165508093684,-0.0342398641086831,
-0.0134038931150264));
#27227=CARTESIAN_POINT('Ctrl Pts',(-0.0126306236596915,-0.0342579197062186,
-0.0134335884373465));
#27228=CARTESIAN_POINT('Ctrl Pts',(-0.0125872163046045,-0.0342606607741249,
-0.0134380965625869));
#27229=CARTESIAN_POINT('Ctrl Pts',(-0.0125435961840299,-0.0342634008237744,
-0.0134403530572374));
#27230=CARTESIAN_POINT('Ctrl Pts',(-0.0125000066519147,-0.0342661396007313,
-0.0134403532865406));
#27231=CARTESIAN_POINT('Ctrl Pts',(-0.0122040785829089,-0.0342847330780403,
-0.0134403548432731));
#27232=CARTESIAN_POINT('Ctrl Pts',(-0.0119088287462426,-0.0343032678967875,
-0.0133322605654254));
#27233=CARTESIAN_POINT('Ctrl Pts',(-0.0116827236707415,-0.0343220359752789,
-0.0131407468825747));
#27234=CARTESIAN_POINT('Ctrl Pts',(-0.0116561432766619,-0.0343242423075397,
-0.0131182329732759));
#27235=CARTESIAN_POINT('Ctrl Pts',(-0.0116304947029669,-0.0343264518634068,
-0.0130946209095796));
#27236=CARTESIAN_POINT('Ctrl Pts',(-0.0116058658269969,-0.0343286651171383,
-0.0130699921631696));
#27237=CARTESIAN_POINT('Ctrl Pts',(-0.0114333146555468,-0.0343441712865858,
-0.0128974418994232));
#27238=CARTESIAN_POINT('Ctrl Pts',(-0.011310324410609,-0.0343598589648035,
-0.0126683334263073));
#27239=CARTESIAN_POINT('Ctrl Pts',(-0.0112614280346616,-0.0343751202607046,
-0.0124306075537998));
#27240=CARTESIAN_POINT('Ctrl Pts',(-0.0112439772708908,-0.0343805669070961,
-0.0123457649051789));
#27241=CARTESIAN_POINT('Ctrl Pts',(-0.0112355,-0.0343859592441231,-0.0122600429339026));
#27242=CARTESIAN_POINT('Ctrl Pts',(-0.0112355,-0.034391269638083,-0.0121758532865581));
#27243=CARTESIAN_POINT('Ctrl Pts',(-0.0112355,-0.0344114595538166,-0.0118557674514308));
#27244=CARTESIAN_POINT('Ctrl Pts',(-0.0113533279721126,-0.0344304649895133,
-0.0115562112741644));
#27245=CARTESIAN_POINT('Ctrl Pts',(-0.0115664721147305,-0.0344502780039842,
-0.0113229254247642));
#27246=CARTESIAN_POINT('Ctrl Pts',(-0.0117451590437316,-0.0344668880157188,
-0.0111273529286274));
#27247=CARTESIAN_POINT('Ctrl Pts',(-0.0119943711986191,-0.03448406560298,
-0.0109844551616016));
#27248=CARTESIAN_POINT('Ctrl Pts',(-0.012265501352359,-0.0345014958683265,
-0.0109332871377135));
#27249=CARTESIAN_POINT('Ctrl Pts',(-0.0123177849171256,-0.0345048570452173,
-0.0109234201175608));
#27250=CARTESIAN_POINT('Ctrl Pts',(-0.0123707825304687,-0.0345082276180931,
-0.0109168422232236));
#27251=CARTESIAN_POINT('Ctrl Pts',(-0.0124240318569026,-0.034511605328916,
-0.010913637341787));
#27252=CARTESIAN_POINT('Ctrl Pts',(-0.0127003824135621,-0.0345291347950834,
-0.0108970048164887));
#27253=CARTESIAN_POINT('Ctrl Pts',(-0.012989029181726,-0.0345468565109965,
-0.0109750528015166));
#27254=CARTESIAN_POINT('Ctrl Pts',(-0.0132239667471111,-0.0345648565559082,
-0.0111391120463842));
#27255=CARTESIAN_POINT('Ctrl Pts',(-0.013269055909737,-0.0345683111203197,
-0.011170598258306));
#27256=CARTESIAN_POINT('Ctrl Pts',(-0.0133121818315644,-0.0345717759364779,
-0.0112050969475248));
#27257=CARTESIAN_POINT('Ctrl Pts',(-0.0133529328811715,-0.0345752516128787,
-0.0112423299873221));
#27258=CARTESIAN_POINT('Ctrl Pts',(-0.0135629921327208,-0.0345931676663403,
-0.0114342549695773));
#27259=CARTESIAN_POINT('Ctrl Pts',(-0.0137095012841564,-0.0346113722860647,
-0.0117040258019251));
#27260=CARTESIAN_POINT('Ctrl Pts',(-0.0137515302674899,-0.0346298376912104,
-0.0119952093285727));
#27261=CARTESIAN_POINT('Ctrl Pts',(-0.0137601388925848,-0.034633619884771,
-0.0120548512617315));
#27262=CARTESIAN_POINT('Ctrl Pts',(-0.0137645006514589,-0.0346374130192336,
-0.0121152795154768));
#27263=CARTESIAN_POINT('Ctrl Pts',(-0.0137644999999269,-0.0346412168558721,
-0.0121758668844777));
#27264=CARTESIAN_POINT('Origin',(-0.0125,-0.0412787743898723,-0.0121758532865581));
#27265=CARTESIAN_POINT('',(-0.0137644999524637,-0.0351412586228095,-0.0121760944261459));
#27266=CARTESIAN_POINT('',(-0.0137644998439392,-0.0350788026914135,-0.0121754128237017));
#27267=CARTESIAN_POINT('',(-0.0137645,-0.0412787743898723,-0.0121758532865581));
#27268=CARTESIAN_POINT('Ctrl Pts',(-0.0137644996879007,-0.0350787743898623,
-0.0121749648615133));
#27269=CARTESIAN_POINT('Ctrl Pts',(-0.0137642950427078,-0.0350604396877818,
-0.011883692363005));
#27270=CARTESIAN_POINT('Ctrl Pts',(-0.013659236707341,-0.0350421049857011,
-0.0115930051217057));
#27271=CARTESIAN_POINT('Ctrl Pts',(-0.0134736789464501,-0.0350237702836206,
-0.0113690636242298));
#27272=CARTESIAN_POINT('Ctrl Pts',(-0.0134483913569099,-0.0350212716523678,
-0.0113385451450134));
#27273=CARTESIAN_POINT('Ctrl Pts',(-0.0134216813408798,-0.0350187730211151,
-0.0113092329057806));
#27274=CARTESIAN_POINT('Ctrl Pts',(-0.0133936746716602,-0.0350162743898623,
-0.0112812551470379));
#27275=CARTESIAN_POINT('Ctrl Pts',(-0.0131919498582662,-0.0349982773935308,
-0.0110797385683511));
#27276=CARTESIAN_POINT('Ctrl Pts',(-0.0129184463589703,-0.0349802803971992,
-0.0109488602095992));
#27277=CARTESIAN_POINT('Ctrl Pts',(-0.0126343199263155,-0.0349622834008676,
-0.0109185075077866));
#27278=CARTESIAN_POINT('Ctrl Pts',(-0.0125895414366565,-0.0349594470638658,
-0.0109137239044747));
#27279=CARTESIAN_POINT('Ctrl Pts',(-0.0125445392582302,-0.0349566107268641,
-0.0109113385101257));
#27280=CARTESIAN_POINT('Ctrl Pts',(-0.0124995824442955,-0.0349537743898623,
-0.0109113533554995));
#27281=CARTESIAN_POINT('Ctrl Pts',(-0.0122132696361486,-0.0349357108408525,
-0.0109114479000252));
#27282=CARTESIAN_POINT('Ctrl Pts',(-0.0119263662305414,-0.0349176472918427,
-0.0110130373568707));
#27283=CARTESIAN_POINT('Ctrl Pts',(-0.0117036166925373,-0.0348995837428329,
-0.0111936446134164));
#27284=CARTESIAN_POINT('Ctrl Pts',(-0.0116694612683676,-0.0348968139585094,
-0.0112213381274444));
#27285=CARTESIAN_POINT('Ctrl Pts',(-0.0116367746190418,-0.0348940441741858,
-0.0112507966940394));
#27286=CARTESIAN_POINT('Ctrl Pts',(-0.0116057347054632,-0.0348912743898623,
-0.0112818455500216));
#27287=CARTESIAN_POINT('Ctrl Pts',(-0.0114033415098123,-0.0348732142396919,
-0.011484297053878));
#27288=CARTESIAN_POINT('Ctrl Pts',(-0.0112722669203073,-0.0348551540895215,
-0.0117589223670615));
#27289=CARTESIAN_POINT('Ctrl Pts',(-0.0112423862595724,-0.034837093939351,
-0.0120440658444863));
#27290=CARTESIAN_POINT('Ctrl Pts',(-0.0112377980061822,-0.0348343207561881,
-0.0120878503691525));
#27291=CARTESIAN_POINT('Ctrl Pts',(-0.0112355018543397,-0.0348315475730252,
-0.0121318451990947));
#27292=CARTESIAN_POINT('Ctrl Pts',(-0.0112355000011239,-0.0348287743898623,
-0.0121757999728644));
#27293=CARTESIAN_POINT('Ctrl Pts',(-0.0112354879321933,-0.0348107142396919,
-0.0124620521849796));
#27294=CARTESIAN_POINT('Ctrl Pts',(-0.0113369297788642,-0.0347926540895215,
-0.0127489452454201));
#27295=CARTESIAN_POINT('Ctrl Pts',(-0.0115173927210527,-0.0347745939393511,
-0.0129717447272457));
#27296=CARTESIAN_POINT('Ctrl Pts',(-0.011545103276507,-0.0347718207561882,
-0.0130059561687829));
#27297=CARTESIAN_POINT('Ctrl Pts',(-0.0115745839409616,-0.0347690475730252,
-0.0130386960351572));
#27298=CARTESIAN_POINT('Ctrl Pts',(-0.0116056593225539,-0.0347662743898623,
-0.0130697856121092));
#27299=CARTESIAN_POINT('Ctrl Pts',(-0.0118080735322945,-0.0347482108408525,
-0.013272292285478));
#27300=CARTESIAN_POINT('Ctrl Pts',(-0.0120827101271603,-0.0347301472918427,
-0.0134034777225892));
#27301=CARTESIAN_POINT('Ctrl Pts',(-0.0123679029266934,-0.0347120837428329,
-0.013433434541676));
#27302=CARTESIAN_POINT('Ctrl Pts',(-0.0124116331230631,-0.0347093139585094,
-0.0134380279871747));
#27303=CARTESIAN_POINT('Ctrl Pts',(-0.0124555738847812,-0.0347065441741858,
-0.013440334978898));
#27304=CARTESIAN_POINT('Ctrl Pts',(-0.0124994758169154,-0.0347037743898623,
-0.0134403531779112));
#27305=CARTESIAN_POINT('Ctrl Pts',(-0.012784733735675,-0.0346857773935313,
-0.0134404714281197));
#27306=CARTESIAN_POINT('Ctrl Pts',(-0.0130707615942272,-0.0346677803972003,
-0.0133398074729649));
#27307=CARTESIAN_POINT('Ctrl Pts',(-0.0132932219367298,-0.0346497834008692,
-0.0131606168160872));
#27308=CARTESIAN_POINT('Ctrl Pts',(-0.0133282818150218,-0.0346469470638669,
-0.0131323762652073));
#27309=CARTESIAN_POINT('Ctrl Pts',(-0.0133618046077298,-0.0346441107268646,
-0.0131022832290055));
#27310=CARTESIAN_POINT('Ctrl Pts',(-0.0133935992326092,-0.0346412743898623,
-0.0130705267809012));
#27311=CARTESIAN_POINT('Ctrl Pts',(-0.0135991266344828,-0.0346229396877819,
-0.0128652461620435));
#27312=CARTESIAN_POINT('Ctrl Pts',(-0.0137311593212538,-0.0346046049857014,
-0.0125858983335253));
#27313=CARTESIAN_POINT('Ctrl Pts',(-0.0137587997171842,-0.034586270283621,
-0.0122957846086425));
#27314=CARTESIAN_POINT('Ctrl Pts',(-0.0137625665172561,-0.0345837716523681,
-0.0122562482574811));
#27315=CARTESIAN_POINT('Ctrl Pts',(-0.0137644683725183,-0.0345812730211152,
-0.0122165426039117));
#27316=CARTESIAN_POINT('Ctrl Pts',(-0.0137644996084897,-0.0345787743898623,
-0.0121768483389608));
#27317=CARTESIAN_POINT('Ctrl Pts',(-0.0137644996573036,-0.0346412743898623,
-0.0121767842425317));
#27318=CARTESIAN_POINT('Ctrl Pts',(-0.013764285216229,-0.0346596056746789,
-0.0124680554444549));
#27319=CARTESIAN_POINT('Ctrl Pts',(-0.0136592179638055,-0.0346779369594955,
-0.0127587381208865));
#27320=CARTESIAN_POINT('Ctrl Pts',(-0.0134736540784892,-0.0346962682443121,
-0.0129826729599929));
#27321=CARTESIAN_POINT('Ctrl Pts',(-0.013448339648412,-0.0346987689789078,
-0.0130132219152314));
#27322=CARTESIAN_POINT('Ctrl Pts',(-0.0134215999140004,-0.0347012697135035,
-0.0130425621095678));
#27323=CARTESIAN_POINT('Ctrl Pts',(-0.0133935610472872,-0.0347037704480992,
-0.0130705649187452));
#27324=CARTESIAN_POINT('Ctrl Pts',(-0.0131918126532027,-0.0347217640137402,
-0.0132720538676103));
#27325=CARTESIAN_POINT('Ctrl Pts',(-0.0129182953407975,-0.0347397575793813,
-0.0134028973345348));
#27326=CARTESIAN_POINT('Ctrl Pts',(-0.0126341674539392,-0.0347577511450224,
-0.0134332153443217));
#27327=CARTESIAN_POINT('Ctrl Pts',(-0.0125893467725896,-0.0347605895987936,
-0.0134379979577808));
#27328=CARTESIAN_POINT('Ctrl Pts',(-0.0125443022800829,-0.0347634280525648,
-0.0134403778704686));
#27329=CARTESIAN_POINT('Ctrl Pts',(-0.0124993037832106,-0.034766266506336,
-0.0134403530948943));
#27330=CARTESIAN_POINT('Ctrl Pts',(-0.0122129936694684,-0.0347843266211966,
-0.0134401954563507));
#27331=CARTESIAN_POINT('Ctrl Pts',(-0.0119261146312032,-0.0348023867360572,
-0.0133385445417751));
#27332=CARTESIAN_POINT('Ctrl Pts',(-0.0117034055697304,-0.0348204468509179,
-0.0131578907418842));
#27333=CARTESIAN_POINT('Ctrl Pts',(-0.0116692237128628,-0.0348232187554695,
-0.0131301636153379));
#27334=CARTESIAN_POINT('Ctrl Pts',(-0.0116365138032983,-0.0348259906600211,
-0.0131006684012419));
#27335=CARTESIAN_POINT('Ctrl Pts',(-0.0116054542621016,-0.0348287625645727,
-0.0130695804109131));
#27336=CARTESIAN_POINT('Ctrl Pts',(-0.0114031264267015,-0.0348468192848671,
-0.0128670672523849));
#27337=CARTESIAN_POINT('Ctrl Pts',(-0.011272138149275,-0.0348648760051615,
-0.0125924033996814));
#27338=CARTESIAN_POINT('Ctrl Pts',(-0.0112423456656896,-0.0348829327254559,
-0.0123072527743432));
#27339=CARTESIAN_POINT('Ctrl Pts',(-0.0112377665919671,-0.0348857080245738,
-0.0122634254199813));
#27340=CARTESIAN_POINT('Ctrl Pts',(-0.0112354840278291,-0.0348884833236916,
-0.0122193880730684));
#27341=CARTESIAN_POINT('Ctrl Pts',(-0.0112355000842078,-0.0348912586228095,
-0.0121753918089769));
#27342=CARTESIAN_POINT('Ctrl Pts',(-0.0112356045506192,-0.0349093153431039,
-0.0118891422189465));
#27343=CARTESIAN_POINT('Ctrl Pts',(-0.0113371614640519,-0.0349273720633983,
-0.0116022924016807));
#27344=CARTESIAN_POINT('Ctrl Pts',(-0.0115177126222287,-0.0349454287836927,
-0.0113795670582009));
#27345=CARTESIAN_POINT('Ctrl Pts',(-0.0115454631473433,-0.0349482040828106,
-0.0113453344046954));
#27346=CARTESIAN_POINT('Ctrl Pts',(-0.0115749865410915,-0.0349509793819284,
-0.0113125768291603));
#27347=CARTESIAN_POINT('Ctrl Pts',(-0.0116061068293765,-0.0349537546810463,
-0.0112814734737757));
#27348=CARTESIAN_POINT('Ctrl Pts',(-0.0118086204890069,-0.0349718147959071,
-0.011079070004115));
#27349=CARTESIAN_POINT('Ctrl Pts',(-0.0120833200690478,-0.0349898749107678,
-0.0109480221876352));
#27350=CARTESIAN_POINT('Ctrl Pts',(-0.0123685255462422,-0.0350079350256286,
-0.010918206786937));
#27351=CARTESIAN_POINT('Ctrl Pts',(-0.0124122994849158,-0.0350107069301801,
-0.0109136306563012));
#27352=CARTESIAN_POINT('Ctrl Pts',(-0.0124562832517799,-0.0350134788347316,
-0.0109113454273497));
#27353=CARTESIAN_POINT('Ctrl Pts',(-0.0125002267383571,-0.0350162507392831,
-0.0109113533068864));
#27354=CARTESIAN_POINT('Ctrl Pts',(-0.0127854818745024,-0.0350342443049242,
-0.0109114044561802));
#27355=CARTESIAN_POINT('Ctrl Pts',(-0.0130714478229443,-0.0350522378705653,
-0.0110122364028001));
#27356=CARTESIAN_POINT('Ctrl Pts',(-0.0132938009925633,-0.0350702314362064,
-0.0111915564643518));
#27357=CARTESIAN_POINT('Ctrl Pts',(-0.0133288768194129,-0.0350730698899776,
-0.011219843893042));
#27358=CARTESIAN_POINT('Ctrl Pts',(-0.013362411605519,-0.0350759083437487,
-0.0112499863474084));
#27359=CARTESIAN_POINT('Ctrl Pts',(-0.0133942138568448,-0.0350787467975199,
-0.011281794100471));
#27360=CARTESIAN_POINT('Ctrl Pts',(-0.0135995989622101,-0.0350970780823365,
-0.0114872147371192));
#27361=CARTESIAN_POINT('Ctrl Pts',(-0.0137314396478263,-0.0351154093671531,
-0.0117666516692974));
#27362=CARTESIAN_POINT('Ctrl Pts',(-0.0137588814672488,-0.0351337406519698,
-0.0120567831332134));
#27363=CARTESIAN_POINT('Ctrl Pts',(-0.0137626250513938,-0.0351362413865654,
-0.0120963625623891));
#27364=CARTESIAN_POINT('Ctrl Pts',(-0.0137644997485598,-0.0351387421211611,
-0.0121361103638794));
#27365=CARTESIAN_POINT('Ctrl Pts',(-0.0137644999999747,-0.0351412428557567,
-0.0121758452856833));
#27366=CARTESIAN_POINT('Origin',(-0.0125,-0.0412787743898723,-0.0121758532865581));
#27367=CARTESIAN_POINT('',(-0.0137644997162062,-0.0356413083664635,-0.0121752330744908));
#27368=CARTESIAN_POINT('',(-0.0137644999999548,-0.035578810380488,-0.0121758425904543));
#27369=CARTESIAN_POINT('',(-0.0137645,-0.0412787743898723,-0.0121758532865581));
#27370=CARTESIAN_POINT('Ctrl Pts',(-0.0137644998645128,-0.0355787743898623,
-0.0121752679258704));
#27371=CARTESIAN_POINT('Ctrl Pts',(-0.0137643650298108,-0.0355604448524855,
-0.0118839971487647));
#27372=CARTESIAN_POINT('Ctrl Pts',(-0.0136593775416596,-0.0355421153151086,
-0.0115932861456091));
#27373=CARTESIAN_POINT('Ctrl Pts',(-0.0134738753817643,-0.0355237857777318,
-0.0113693007521294));
#27374=CARTESIAN_POINT('Ctrl Pts',(-0.0134485598460573,-0.0355212843402379,
-0.0113387333979288));
#27375=CARTESIAN_POINT('Ctrl Pts',(-0.0134218176053227,-0.035518782902744,
-0.0113093753215851));
#27376=CARTESIAN_POINT('Ctrl Pts',(-0.0133937749411315,-0.0355162814652501,
-0.0112813553242321));
#27377=CARTESIAN_POINT('Ctrl Pts',(-0.0131920754641933,-0.0354982896428374,
-0.011079818880641));
#27378=CARTESIAN_POINT('Ctrl Pts',(-0.0129185904718619,-0.0354802978204246,
-0.0109489100783296));
#27379=CARTESIAN_POINT('Ctrl Pts',(-0.012634470720931,-0.0354623059980119,
-0.0109185236260425));
#27380=CARTESIAN_POINT('Ctrl Pts',(-0.01258963594707,-0.0354594668455539,
-0.0109137285714492));
#27381=CARTESIAN_POINT('Ctrl Pts',(-0.0125445766306353,-0.0354566276930959,
-0.0109113378005705));
#27382=CARTESIAN_POINT('Ctrl Pts',(-0.0124995628543102,-0.0354537885406379,
-0.0109113533621201));
#27383=CARTESIAN_POINT('Ctrl Pts',(-0.0122132536914851,-0.0354357301720729,
-0.010911452341024));
#27384=CARTESIAN_POINT('Ctrl Pts',(-0.0119263545560491,-0.0354176718035078,
-0.0110130438307979));
#27385=CARTESIAN_POINT('Ctrl Pts',(-0.0117036087326358,-0.0353996134349428,
-0.011193651067427));
#27386=CARTESIAN_POINT('Ctrl Pts',(-0.0116694092714644,-0.0353968408286371,
-0.0112213807464024));
#27387=CARTESIAN_POINT('Ctrl Pts',(-0.0116366824156856,-0.0353940682223314,
-0.0112508800461999));
#27388=CARTESIAN_POINT('Ctrl Pts',(-0.011605606805275,-0.0353912956160257,
-0.0112819735053629));
#27389=CARTESIAN_POINT('Ctrl Pts',(-0.0114032450821832,-0.0353732406403693,
-0.0114844514580067));
#27390=CARTESIAN_POINT('Ctrl Pts',(-0.0112722099834925,-0.0353551856647129,
-0.0117590920093227));
#27391=CARTESIAN_POINT('Ctrl Pts',(-0.0112423683634143,-0.0353371306890566,
-0.0120442367349436));
#27392=CARTESIAN_POINT('Ctrl Pts',(-0.0112377801371288,-0.0353343546898422,
-0.0120880784741608));
#27393=CARTESIAN_POINT('Ctrl Pts',(-0.0112354899766516,-0.0353315786906279,
-0.0121321307471615));
#27394=CARTESIAN_POINT('Ctrl Pts',(-0.0112355000330095,-0.0353288026914135,
-0.012176142217244));
#27395=CARTESIAN_POINT('Ctrl Pts',(-0.0112355654391149,-0.0353107477157571,
-0.0124623908648782));
#27396=CARTESIAN_POINT('Ctrl Pts',(-0.0113370825786684,-0.0352926927401007,
-0.0127492538332294));
#27397=CARTESIAN_POINT('Ctrl Pts',(-0.0115176024370534,-0.0352746377644444,
-0.012972003572821));
#27398=CARTESIAN_POINT('Ctrl Pts',(-0.0115453578322745,-0.03527186176523,
-0.013006251921524));
#27399=CARTESIAN_POINT('Ctrl Pts',(-0.0115748875291204,-0.0352690857660157,
-0.0130390244141873));
#27400=CARTESIAN_POINT('Ctrl Pts',(-0.0116060153910218,-0.0352663097668013,
-0.0130701417013942));
#27401=CARTESIAN_POINT('Ctrl Pts',(-0.0118085076683799,-0.0352482513982362,
-0.013272565188484));
#27402=CARTESIAN_POINT('Ctrl Pts',(-0.0120831928824371,-0.0352301930296712,
-0.0134036410334657));
#27403=CARTESIAN_POINT('Ctrl Pts',(-0.0123683944744434,-0.0352121346611062,
-0.0134334860770192));
#27404=CARTESIAN_POINT('Ctrl Pts',(-0.012412183132845,-0.0352093620548005,
-0.0134380683600561));
#27405=CARTESIAN_POINT('Ctrl Pts',(-0.0124561820031353,-0.0352065894484948,
-0.0134403581705277));
#27406=CARTESIAN_POINT('Ctrl Pts',(-0.012500140715678,-0.0352038168421891,
-0.0134403532787286));
#27407=CARTESIAN_POINT('Ctrl Pts',(-0.0127853948276369,-0.035185825019777,
-0.013440321535173));
#27408=CARTESIAN_POINT('Ctrl Pts',(-0.0130713668724668,-0.0351678331973647,
-0.0133395097199173));
#27409=CARTESIAN_POINT('Ctrl Pts',(-0.0132937319760708,-0.0351498413749526,
-0.0131602057641609));
#27410=CARTESIAN_POINT('Ctrl Pts',(-0.0133288217194071,-0.035147002222494,
-0.0131319111725874));
#27411=CARTESIAN_POINT('Ctrl Pts',(-0.0133623695013503,-0.0351441630700355,
-0.0131017601841739));
#27412=CARTESIAN_POINT('Ctrl Pts',(-0.0133941836226608,-0.0351413239175769,
-0.0130699427110371));
#27413=CARTESIAN_POINT('Ctrl Pts',(-0.0135995752436411,-0.0351229943802,
-0.0128645294507032));
#27414=CARTESIAN_POINT('Ctrl Pts',(-0.013731425379661,-0.0351046648428231,
-0.0125850975507378));
#27415=CARTESIAN_POINT('Ctrl Pts',(-0.0137588773038086,-0.0350863353054463,
-0.0122949674500972));
#27416=CARTESIAN_POINT('Ctrl Pts',(-0.0137626236761763,-0.0350838338679524,
-0.0122553733077617));
#27417=CARTESIAN_POINT('Ctrl Pts',(-0.0137644997642347,-0.0350813324304586,
-0.012215610600945));
#27418=CARTESIAN_POINT('Ctrl Pts',(-0.0137644999999778,-0.0350788309929647,
-0.01217586078589));
#27419=CARTESIAN_POINT('Ctrl Pts',(-0.0137644999049527,-0.0351412743898623,
-0.0121763435666085));
#27420=CARTESIAN_POINT('Ctrl Pts',(-0.0137643869710071,-0.0351596085328665,
-0.0124676157963035));
#27421=CARTESIAN_POINT('Ctrl Pts',(-0.013659420380221,-0.0351779426758707,
-0.0127583358472446));
#27422=CARTESIAN_POINT('Ctrl Pts',(-0.0134739334875397,-0.0351962768188749,
-0.0129823356557694));
#27423=CARTESIAN_POINT('Ctrl Pts',(-0.0134486491288289,-0.035198776009204,
-0.0130128698429997));
#27424=CARTESIAN_POINT('Ctrl Pts',(-0.0134219412424153,-0.0352012751995332,
-0.0130421976272212));
#27425=CARTESIAN_POINT('Ctrl Pts',(-0.0133939356586194,-0.0352037743898623,
-0.0130701906324454));
#27426=CARTESIAN_POINT('Ctrl Pts',(-0.0131922701491049,-0.0352217708185307,
-0.0132717655648774));
#27427=CARTESIAN_POINT('Ctrl Pts',(-0.0129188055429118,-0.0352397672471992,
-0.0134027236820722));
#27428=CARTESIAN_POINT('Ctrl Pts',(-0.0126346885717544,-0.0352577636758676,
-0.0134331596289579));
#27429=CARTESIAN_POINT('Ctrl Pts',(-0.0125899011988981,-0.0352606005805325,
-0.0134379574630889));
#27430=CARTESIAN_POINT('Ctrl Pts',(-0.0125448893315503,-0.0352634374851974,
-0.0134403560505243));
#27431=CARTESIAN_POINT('Ctrl Pts',(-0.012499922208476,-0.0352662743898623,
-0.0134403532841652));
#27432=CARTESIAN_POINT('Ctrl Pts',(-0.0122136100445227,-0.0352843373713921,
-0.0134403356703577));
#27433=CARTESIAN_POINT('Ctrl Pts',(-0.0119266798407084,-0.0353024003529218,
-0.0133388237427738));
#27434=CARTESIAN_POINT('Ctrl Pts',(-0.0117038819485851,-0.0353204633344516,
-0.0131582769722515));
#27435=CARTESIAN_POINT('Ctrl Pts',(-0.0116697110371408,-0.0353232336862552,
-0.0131305861909417));
#27436=CARTESIAN_POINT('Ctrl Pts',(-0.0116370091137744,-0.0353260040380587,
-0.0131011291320357));
#27437=CARTESIAN_POINT('Ctrl Pts',(-0.0116059543096101,-0.0353287743898623,
-0.0130700806365621));
#27438=CARTESIAN_POINT('Ctrl Pts',(-0.0114035118493503,-0.0353468339735561,
-0.0128676793018832));
#27439=CARTESIAN_POINT('Ctrl Pts',(-0.01127236984912,-0.0353648935572498,
-0.0125930868256952));
#27440=CARTESIAN_POINT('Ctrl Pts',(-0.0112424188376614,-0.0353829531409437,
-0.0123079512431328));
#27441=CARTESIAN_POINT('Ctrl Pts',(-0.011237818697999,-0.0353857268905832,
-0.0122641576135141));
#27442=CARTESIAN_POINT('Ctrl Pts',(-0.011235511681278,-0.0353885006402228,
-0.0122201530146197));
#27443=CARTESIAN_POINT('Ctrl Pts',(-0.011235500044295,-0.0353912743898623,
-0.0121761879835687));
#27444=CARTESIAN_POINT('Ctrl Pts',(-0.0112354242771583,-0.0354093339735561,
-0.0118899364248321));
#27445=CARTESIAN_POINT('Ctrl Pts',(-0.0113368018549001,-0.0354273935572499,
-0.011603021273402));
#27446=CARTESIAN_POINT('Ctrl Pts',(-0.0115172146027577,-0.0354454531409437,
-0.0113801818009766));
#27447=CARTESIAN_POINT('Ctrl Pts',(-0.0115449239787224,-0.0354482268905832,
-0.0113459561556465));
#27448=CARTESIAN_POINT('Ctrl Pts',(-0.0115744046216873,-0.0354510006402228,
-0.0113132023786766));
#27449=CARTESIAN_POINT('Ctrl Pts',(-0.0116054810537669,-0.0354537743898623,
-0.0112820993468017));
#27450=CARTESIAN_POINT('Ctrl Pts',(-0.0118078544081118,-0.0354718373713921,
-0.0110795527714841));
#27451=CARTESIAN_POINT('Ctrl Pts',(-0.0120824641821012,-0.0354899003529219,
-0.0109483126018268));
#27452=CARTESIAN_POINT('Ctrl Pts',(-0.0123676504375781,-0.0355079633344517,
-0.0109182985786719));
#27453=CARTESIAN_POINT('Ctrl Pts',(-0.0124113899639629,-0.0355107336862552,
-0.0109136952742262));
#27454=CARTESIAN_POINT('Ctrl Pts',(-0.0124553406130904,-0.0355135040380588,
-0.0109113794547743));
#27455=CARTESIAN_POINT('Ctrl Pts',(-0.0124992528144902,-0.0355162743898623,
-0.0109113535073118));
#27456=CARTESIAN_POINT('Ctrl Pts',(-0.0127845100150923,-0.0355342708185307,
-0.0109111849505036));
#27457=CARTESIAN_POINT('Ctrl Pts',(-0.0130705551071837,-0.0355522672471992,
-0.011011798004815));
#27458=CARTESIAN_POINT('Ctrl Pts',(-0.0132930468687106,-0.0355702636758676,
-0.0111909487662982));
#27459=CARTESIAN_POINT('Ctrl Pts',(-0.0133281198227843,-0.0355731005805325,
-0.0112191895712011));
#27460=CARTESIAN_POINT('Ctrl Pts',(-0.0133616553129469,-0.0355759374851974,
-0.011249283986549));
#27461=CARTESIAN_POINT('Ctrl Pts',(-0.0133934620940176,-0.0355787743898623,
-0.0112810428392825));
#27462=CARTESIAN_POINT('Ctrl Pts',(-0.0135990206663115,-0.0355971085328665,
-0.0114862916637728));
#27463=CARTESIAN_POINT('Ctrl Pts',(-0.0137310961679854,-0.0356154426758706,
-0.0117656188650991));
#27464=CARTESIAN_POINT('Ctrl Pts',(-0.0137587812276437,-0.0356337768188748,
-0.0120557280563526));
#27465=CARTESIAN_POINT('Ctrl Pts',(-0.0137625550737048,-0.035636276009204,
-0.0120952738417772));
#27466=CARTESIAN_POINT('Ctrl Pts',(-0.0137644630553627,-0.0356387751995331,
-0.0121349893031318));
#27467=CARTESIAN_POINT('Ctrl Pts',(-0.013764499468231,-0.0356412743898623,
-0.0121746936126288));
#27468=CARTESIAN_POINT('Origin',(-0.0125,-0.0412787743898723,-0.0121758532865581));
#27469=CARTESIAN_POINT('',(-0.0137644999998975,-0.0361412743898623,-0.0121758693894333));
#27470=CARTESIAN_POINT('',(-0.0137644999785623,-0.0360787101931254,-0.0121759146659024));
#27471=CARTESIAN_POINT('',(-0.0137645,-0.0412787743898723,-0.0121758532865581));
#27472=CARTESIAN_POINT('',(-0.0133941365248078,-0.0365787743898683,-0.0112817167617503));
#27473=CARTESIAN_POINT('Ctrl Pts',(-0.0137644999998975,-0.0361412743898623,
-0.0121758693894333));
#27474=CARTESIAN_POINT('Ctrl Pts',(-0.0137644963111485,-0.036159503556529,
-0.0124655333785947));
#27475=CARTESIAN_POINT('Ctrl Pts',(-0.0136609354141153,-0.0361777327231956,
-0.0127544975137962));
#27476=CARTESIAN_POINT('Ctrl Pts',(-0.0134774627796051,-0.0361959618898623,
-0.0129780544860627));
#27477=CARTESIAN_POINT('Ctrl Pts',(-0.013293990145095,-0.036214191056529,
-0.0132016114583292));
#27478=CARTESIAN_POINT('Ctrl Pts',(-0.0130304113544186,-0.0362324202231956,
-0.013359623744977));
#27479=CARTESIAN_POINT('Ctrl Pts',(-0.012746679867081,-0.0362506493898623,
-0.0134160586297077));
#27480=CARTESIAN_POINT('Ctrl Pts',(-0.0124629483797433,-0.036268878556529,
-0.0134724935144385));
#27481=CARTESIAN_POINT('Ctrl Pts',(-0.0121590383423167,-0.0362871077231956,
-0.0134274095583513));
#27482=CARTESIAN_POINT('Ctrl Pts',(-0.0119039099503849,-0.0363053368898623,
-0.0132910379810145));
#27483=CARTESIAN_POINT('Ctrl Pts',(-0.011648781558453,-0.036323566056529,
-0.0131546664036777));
#27484=CARTESIAN_POINT('Ctrl Pts',(-0.0114424524832276,-0.0363417952231956,
-0.0129270102800231));
#27485=CARTESIAN_POINT('Ctrl Pts',(-0.0113317512500114,-0.0363600243898623,
-0.0126597490482156));
#27486=CARTESIAN_POINT('Ctrl Pts',(-0.0112210500167952,-0.036378253556529,
-0.012392487816408));
#27487=CARTESIAN_POINT('Ctrl Pts',(-0.0112059734241391,-0.0363964827231956,
-0.0120856137473264));
#27488=CARTESIAN_POINT('Ctrl Pts',(-0.0112899506983871,-0.0364147118898623,
-0.011808782533615));
#27489=CARTESIAN_POINT('Ctrl Pts',(-0.0113739279726352,-0.036432941056529,
-0.0115319513199036));
#27490=CARTESIAN_POINT('Ctrl Pts',(-0.0115569487924721,-0.0364511702231956,
-0.0112851776311697));
#27491=CARTESIAN_POINT('Ctrl Pts',(-0.0117974847876132,-0.0364693993898623,
-0.0111244577252373));
#27492=CARTESIAN_POINT('Ctrl Pts',(-0.0120380207827542,-0.036487628556529,
-0.0109637378193049));
#27493=CARTESIAN_POINT('Ctrl Pts',(-0.0123361316429891,-0.0365058577231956,
-0.0108890948247504));
#27494=CARTESIAN_POINT('Ctrl Pts',(-0.0126239446771135,-0.0365240868898623,
-0.0109174423969774));
#27495=CARTESIAN_POINT('Ctrl Pts',(-0.0129117577112379,-0.036542316056529,
-0.0109457899692044));
#27496=CARTESIAN_POINT('Ctrl Pts',(-0.0131893131537922,-0.0365605452231956,
-0.0110768933907296));
#27497=CARTESIAN_POINT('Ctrl Pts',(-0.0133941365248104,-0.0365787743898623,
-0.0112817167617477));
#27498=CARTESIAN_POINT('',(-0.0137648283188305,-0.0365787649813118,-0.0121757910623594));
#27499=CARTESIAN_POINT('Origin',(-0.01249999999999,-0.0365787743898623,
-0.0121758532865681));
#27500=CARTESIAN_POINT('Ctrl Pts',(-0.0137644999970264,-0.0365787634361464,
-0.0121757665671622));
#27501=CARTESIAN_POINT('Ctrl Pts',(-0.0137644800216386,-0.0365604308650495,
-0.011884495191133));
#27502=CARTESIAN_POINT('Ctrl Pts',(-0.0136596068291505,-0.0365420982939525,
-0.0115937425877689));
#27503=CARTESIAN_POINT('Ctrl Pts',(-0.0134741927136686,-0.0365237657228555,
-0.0113696840694362));
#27504=CARTESIAN_POINT('Ctrl Pts',(-0.0134489204127944,-0.0365212669581236,
-0.0113391444620604));
#27505=CARTESIAN_POINT('Ctrl Pts',(-0.0134222244523923,-0.0365187681933917,
-0.0113098105901343));
#27506=CARTESIAN_POINT('Ctrl Pts',(-0.0133942305890836,-0.0365162694286598,
-0.0112818108359177));
#27507=CARTESIAN_POINT('Ctrl Pts',(-0.0131926327748777,-0.0364982745737657,
-0.0110801705983359));
#27508=CARTESIAN_POINT('Ctrl Pts',(-0.0129192130519281,-0.0364802797188715,
-0.0109491223851327));
#27509=CARTESIAN_POINT('Ctrl Pts',(-0.0126351075664765,-0.0364622848639774,
-0.0109185918994628));
#27510=CARTESIAN_POINT('Ctrl Pts',(-0.0125902969703159,-0.0364594466217859,
-0.0109137764723275));
#27511=CARTESIAN_POINT('Ctrl Pts',(-0.0125452608315856,-0.0364566083795944,
-0.0109113628806159));
#27512=CARTESIAN_POINT('Ctrl Pts',(-0.0125002688378061,-0.036453770137403,
-0.0109113533151361));
#27513=CARTESIAN_POINT('Ctrl Pts',(-0.0122139582707617,-0.0364357087299618,
-0.010911292444352));
#27514=CARTESIAN_POINT('Ctrl Pts',(-0.011927001428768,-0.0364176473225207,
-0.0110127246613591));
#27515=CARTESIAN_POINT('Ctrl Pts',(-0.0117041544539178,-0.0363995859150795,
-0.0111932088357107));
#27516=CARTESIAN_POINT('Ctrl Pts',(-0.0116699565291717,-0.0363968142254351,
-0.0112209057977919));
#27517=CARTESIAN_POINT('Ctrl Pts',(-0.0116372287675296,-0.0363940425357906,
-0.0112503714453245));
#27518=CARTESIAN_POINT('Ctrl Pts',(-0.0116061496458173,-0.0363912708461462,
-0.0112814306826803));
#27519=CARTESIAN_POINT('Ctrl Pts',(-0.0114036640767703,-0.0363732128340805,
-0.0114837867018874));
#27520=CARTESIAN_POINT('Ctrl Pts',(-0.0112724621911305,-0.0363551548220149,
-0.0117583489942559));
#27521=CARTESIAN_POINT('Ctrl Pts',(-0.0112424481357505,-0.0363370968099492,
-0.0120434767073505));
#27522=CARTESIAN_POINT('Ctrl Pts',(-0.0112378356925221,-0.0363343217249293,
-0.0120872940246996));
#27523=CARTESIAN_POINT('Ctrl Pts',(-0.0112355189166647,-0.0363315466399093,
-0.0121313230566792));
#27524=CARTESIAN_POINT('Ctrl Pts',(-0.0112355001154928,-0.0363287715548894,
-0.0121753128410888));
#27525=CARTESIAN_POINT('Ctrl Pts',(-0.0112353777726506,-0.0363107135428238,
-0.0124615628305231));
#27526=CARTESIAN_POINT('Ctrl Pts',(-0.0113367076382122,-0.0362926555307582,
-0.0127484933262912));
#27527=CARTESIAN_POINT('Ctrl Pts',(-0.0115170826499863,-0.0362745975186926,
-0.0129713617610837));
#27528=CARTESIAN_POINT('Ctrl Pts',(-0.0115448019798509,-0.0362718224336726,
-0.013005611314831));
#27529=CARTESIAN_POINT('Ctrl Pts',(-0.0115742948215681,-0.0362690473486526,
-0.0130383876299737));
#27530=CARTESIAN_POINT('Ctrl Pts',(-0.0116053854225937,-0.0362662722636327,
-0.0130695115030437));
#27531=CARTESIAN_POINT('Ctrl Pts',(-0.0118077359843553,-0.0362482108561913,
-0.0132720786131075));
#27532=CARTESIAN_POINT('Ctrl Pts',(-0.0120823301407312,-0.0362301494487498,
-0.0134033480734044));
#27533=CARTESIAN_POINT('Ctrl Pts',(-0.0123675118223398,-0.0362120880413084,
-0.0134333933983558));
#27534=CARTESIAN_POINT('Ctrl Pts',(-0.0124112755830647,-0.0362093163516642,
-0.0134380041307306));
#27535=CARTESIAN_POINT('Ctrl Pts',(-0.0124552509563464,-0.0362065446620201,
-0.013440324809775));
#27536=CARTESIAN_POINT('Ctrl Pts',(-0.0124991879468924,-0.0362037729723759,
-0.0134403530258106));
#27537=CARTESIAN_POINT('Ctrl Pts',(-0.0127844434664075,-0.0361857781174813,
-0.0134405362149596));
#27538=CARTESIAN_POINT('Ctrl Pts',(-0.0130704924772702,-0.0361677832625866,
-0.0133399389361538));
#27539=CARTESIAN_POINT('Ctrl Pts',(-0.0132929929969568,-0.036149788407692,
-0.0131608011820214));
#27540=CARTESIAN_POINT('Ctrl Pts',(-0.013328086937207,-0.036146950165501,
-0.0131325466428907));
#27541=CARTESIAN_POINT('Ctrl Pts',(-0.0133616418066973,-0.0361441119233101,
-0.0131024363525336));
#27542=CARTESIAN_POINT('Ctrl Pts',(-0.013393466037558,-0.0361412736811191,
-0.0130706597962184));
#27543=CARTESIAN_POINT('Ctrl Pts',(-0.0135990230033344,-0.0361229410950005,
-0.012865410766711));
#27544=CARTESIAN_POINT('Ctrl Pts',(-0.0137310972748207,-0.0361046085088818,
-0.0125860839173667));
#27545=CARTESIAN_POINT('Ctrl Pts',(-0.0137587815333782,-0.0360862759227632,
-0.0122959753129568));
#27546=CARTESIAN_POINT('Ctrl Pts',(-0.0137625575850322,-0.0360837754117962,
-0.0122564053503643));
#27547=CARTESIAN_POINT('Ctrl Pts',(-0.0137644654887648,-0.0360812749008293,
-0.0122166655083911));
#27548=CARTESIAN_POINT('Ctrl Pts',(-0.0137644995356581,-0.0360787743898623,
-0.0121769369472666));
#27549=CARTESIAN_POINT('Origin',(-0.0125,-0.0412787743898723,-0.0121758532865581));
#27550=CARTESIAN_POINT('Ctrl Pts',(-0.0137644999999428,-0.0360787070941287,
-0.0121758653168742));
#27551=CARTESIAN_POINT('Ctrl Pts',(-0.0137645027710451,-0.0360604037462595,
-0.0118845962566965));
#27552=CARTESIAN_POINT('Ctrl Pts',(-0.0136596538279521,-0.0360420968508638,
-0.0115938372087226));
#27553=CARTESIAN_POINT('Ctrl Pts',(-0.0134489478207998,-0.0360212816143236,
-0.0113391724258185));
#27554=CARTESIAN_POINT('Ctrl Pts',(-0.0134222076012039,-0.0360187809718295,
-0.011309789642501));
#27555=CARTESIAN_POINT('Ctrl Pts',(-0.0131925528985201,-0.035998300488268,
-0.0110801201704503));
#27556=CARTESIAN_POINT('Ctrl Pts',(-0.0129191234392818,-0.0359803126804235,
-0.0109490916009595));
#27557=CARTESIAN_POINT('Ctrl Pts',(-0.0125901687238666,-0.0359594902232465,
-0.0109137660339032));
#27558=CARTESIAN_POINT('Ctrl Pts',(-0.0125450967097083,-0.0359566516063094,
-0.0109113557557444));
#27559=CARTESIAN_POINT('Ctrl Pts',(-0.0122137592380001,-0.0359357645411937,
-0.0109113376000308));
#27560=CARTESIAN_POINT('Ctrl Pts',(-0.011926818932112,-0.0359177219816858,
-0.0110128147670077));
#27561=CARTESIAN_POINT('Ctrl Pts',(-0.0116697789103805,-0.0358968631466295,
-0.0112210585362829));
#27562=CARTESIAN_POINT('Ctrl Pts',(-0.0116370299322194,-0.0358940851140304,
-0.0112505551257888));
#27563=CARTESIAN_POINT('Ctrl Pts',(-0.0114035277909905,-0.0358732173124676,
-0.0114840211069177));
#27564=CARTESIAN_POINT('Ctrl Pts',(-0.0112723991914978,-0.0358550825527723,
-0.0117585659288796));
#27565=CARTESIAN_POINT('Ctrl Pts',(-0.0112378150477382,-0.0358342964986842,
-0.0120875490318841));
#27566=CARTESIAN_POINT('Ctrl Pts',(-0.0112355044165741,-0.0358315258616311,
-0.0121316580707312));
#27567=CARTESIAN_POINT('Ctrl Pts',(-0.011235471344901,-0.035810775654875,
-0.0124621217168363));
#27568=CARTESIAN_POINT('Ctrl Pts',(-0.0113369931344784,-0.0357929409320698,
-0.0127491482396458));
#27569=CARTESIAN_POINT('Ctrl Pts',(-0.011545280568908,-0.0357722991176314,
-0.0130061558519736));
#27570=CARTESIAN_POINT('Ctrl Pts',(-0.0115747139842782,-0.0357695554470609,
-0.0130388315090776));
#27571=CARTESIAN_POINT('Ctrl Pts',(-0.0118080646633445,-0.0357489005707485,
-0.0132722483314945));
#27572=CARTESIAN_POINT('Ctrl Pts',(-0.0120825614129742,-0.0357308942040033,
-0.0134033983119082));
#27573=CARTESIAN_POINT('Ctrl Pts',(-0.0124115825287087,-0.0357100660326244,
-0.0134380324734021));
#27574=CARTESIAN_POINT('Ctrl Pts',(-0.012455753473972,-0.0357072824220144,
-0.0134403492366539));
#27575=CARTESIAN_POINT('Ctrl Pts',(-0.0127851523474117,-0.035686499711345,
-0.0134403794262162));
#27576=CARTESIAN_POINT('Ctrl Pts',(-0.0130711567415406,-0.0356684713902834,
-0.01333961612615));
#27577=CARTESIAN_POINT('Ctrl Pts',(-0.0133286829772299,-0.0356475433198898,
-0.0131320329729809));
#27578=CARTESIAN_POINT('Ctrl Pts',(-0.0133622591511792,-0.0356446881239693,
-0.0131018645347246));
#27579=CARTESIAN_POINT('Ctrl Pts',(-0.0135995132123415,-0.03562340395237,
-0.0128646302103059));
#27580=CARTESIAN_POINT('Ctrl Pts',(-0.0137313901983395,-0.0356049261749303,
-0.0125852062335056));
#27581=CARTESIAN_POINT('Ctrl Pts',(-0.0137626208620077,-0.0355838735829413,
-0.0122554389422992));
#27582=CARTESIAN_POINT('Ctrl Pts',(-0.0137645003365433,-0.0355813423894253,
-0.0122156342959332));
#27583=CARTESIAN_POINT('Ctrl Pts',(-0.0137644999999548,-0.035578810380488,
-0.0121758425904543));
#27584=CARTESIAN_POINT('Ctrl Pts',(-0.0137644999999968,-0.0356413472503601,
-0.0121758504516997));
#27585=CARTESIAN_POINT('Ctrl Pts',(-0.0137645006529895,-0.0356596747292774,
-0.0124671204460104));
#27586=CARTESIAN_POINT('Ctrl Pts',(-0.0136596489458883,-0.0356780022081948,
-0.0127578796025123));
#27587=CARTESIAN_POINT('Ctrl Pts',(-0.013474251883555,-0.0356963296871122,
-0.0129819509961378));
#27588=CARTESIAN_POINT('Ctrl Pts',(-0.0134489342907337,-0.0356988324648953,
-0.0130125499076594));
#27589=CARTESIAN_POINT('Ctrl Pts',(-0.0134221875850932,-0.0357013352426784,
-0.013041938643616));
#27590=CARTESIAN_POINT('Ctrl Pts',(-0.0133941382376717,-0.0357038380204616,
-0.0130699880985039));
#27591=CARTESIAN_POINT('Ctrl Pts',(-0.0131925219158135,-0.035721827774144,
-0.0132716051928208));
#27592=CARTESIAN_POINT('Ctrl Pts',(-0.0129190918965321,-0.0357398175278265,
-0.0134026249827858));
#27593=CARTESIAN_POINT('Ctrl Pts',(-0.0126349860273449,-0.0357578072815089,
-0.0134331277285244));
#27594=CARTESIAN_POINT('Ctrl Pts',(-0.012590126959616,-0.0357606477845269,
-0.0134379439779772));
#27595=CARTESIAN_POINT('Ctrl Pts',(-0.0125450421010048,-0.035763488287545,
-0.0134403532149679));
#27596=CARTESIAN_POINT('Ctrl Pts',(-0.0125000020098496,-0.035766328790563,
-0.0134403532865565));
#27597=CARTESIAN_POINT('Ctrl Pts',(-0.0122136945132895,-0.0357843850885679,
-0.0134403537416257));
#27598=CARTESIAN_POINT('Ctrl Pts',(-0.0119267613588196,-0.0358024413865726,
-0.0133388630106222));
#27599=CARTESIAN_POINT('Ctrl Pts',(-0.0117039532486444,-0.0358204976845775,
-0.013158334746768));
#27600=CARTESIAN_POINT('Ctrl Pts',(-0.0116697236133939,-0.0358232716432731,
-0.0131306004932021));
#27601=CARTESIAN_POINT('Ctrl Pts',(-0.0116369677265673,-0.0358260456019688,
-0.0131010939841645));
#27602=CARTESIAN_POINT('Ctrl Pts',(-0.0116058646046839,-0.0358288195606644,
-0.0130699909408613));
#27603=CARTESIAN_POINT('Ctrl Pts',(-0.0114034456603145,-0.03584687246844,
-0.0128675725078917));
#27604=CARTESIAN_POINT('Ctrl Pts',(-0.0112723314625597,-0.0358649253762156,
-0.0125929713762996));
#27605=CARTESIAN_POINT('Ctrl Pts',(-0.0112424068074952,-0.0358829782839913,
-0.0123078366649266));
#27606=CARTESIAN_POINT('Ctrl Pts',(-0.0112378030500505,-0.0358857556329161,
-0.0122639701258676));
#27607=CARTESIAN_POINT('Ctrl Pts',(-0.011235500041264,-0.035888532981841,
-0.012219892132267));
#27608=CARTESIAN_POINT('Ctrl Pts',(-0.0112355000000006,-0.0358913103307658,
-0.0121758544713988));
#27609=CARTESIAN_POINT('Ctrl Pts',(-0.0112354997317862,-0.0359093632385414,
-0.0118896074596547));
#27610=CARTESIAN_POINT('Ctrl Pts',(-0.0113369499668099,-0.035927416146317,
-0.0116027224208943));
#27611=CARTESIAN_POINT('Ctrl Pts',(-0.0115174171538356,-0.0359454690540927,
-0.0113799316821124));
#27612=CARTESIAN_POINT('Ctrl Pts',(-0.0115451811215069,-0.0359482464030175,
-0.0113456564491964));
#27613=CARTESIAN_POINT('Ctrl Pts',(-0.0115747218524613,-0.0359510237519424,
-0.0113128584225173));
#27614=CARTESIAN_POINT('Ctrl Pts',(-0.0116058629290656,-0.0359538011008673,
-0.0112817173078721));
#27615=CARTESIAN_POINT('Ctrl Pts',(-0.01180831950711,-0.0359718573988721,
-0.011079260482513));
#27616=CARTESIAN_POINT('Ctrl Pts',(-0.0120829807049326,-0.035989913696877,
-0.0109481379037549));
#27617=CARTESIAN_POINT('Ctrl Pts',(-0.0123681757652149,-0.0360079699948819,
-0.0109182434022445));
#27618=CARTESIAN_POINT('Ctrl Pts',(-0.0124119898026876,-0.0360107439535774,
-0.0109136507602537));
#27619=CARTESIAN_POINT('Ctrl Pts',(-0.0124560147009807,-0.036013517912273,
-0.0109113532990747));
#27620=CARTESIAN_POINT('Ctrl Pts',(-0.0124999996401681,-0.0360162918709686,
-0.0109113532865581));
#27621=CARTESIAN_POINT('Ctrl Pts',(-0.0127852519847615,-0.036034281624651,
-0.0109113532053854));
#27622=CARTESIAN_POINT('Ctrl Pts',(-0.0130712339615104,-0.0360522713783335,
-0.0110121319488751));
#27623=CARTESIAN_POINT('Ctrl Pts',(-0.0132936186122632,-0.0360702611320159,
-0.0111914094088944));
#27624=CARTESIAN_POINT('Ctrl Pts',(-0.0133287321709466,-0.0360731016350339,
-0.0112197165316733));
#27625=CARTESIAN_POINT('Ctrl Pts',(-0.0133623021715428,-0.036075942138052,
-0.011249882405828));
#27626=CARTESIAN_POINT('Ctrl Pts',(-0.0133941365620555,-0.03607878264107,
-0.0112817167989928));
#27627=CARTESIAN_POINT('Ctrl Pts',(-0.0135995382522714,-0.0360971101199873,
-0.0114871185063207));
#27628=CARTESIAN_POINT('Ctrl Pts',(-0.0137314030973446,-0.0361154375989046,
-0.011766542477848));
#27629=CARTESIAN_POINT('Ctrl Pts',(-0.013758870797837,-0.036133765077822,
-0.0120566703836178));
#27630=CARTESIAN_POINT('Ctrl Pts',(-0.0137626217529387,-0.0361362678556051,
-0.0120962898904854));
#27631=CARTESIAN_POINT('Ctrl Pts',(-0.0137645000146323,-0.0361387706333883,
-0.0121360782826731));
#27632=CARTESIAN_POINT('Ctrl Pts',(-0.0137644999999999,-0.0361412734111714,
-0.0121758537517351));
#27633=CARTESIAN_POINT('Origin',(0.006,-0.0412787743898723,-0.0121758532865581));
#27634=CARTESIAN_POINT('Ctrl Pts',(0.0047355001379818,-0.040342276368498,
-0.0121764440115014));
#27635=CARTESIAN_POINT('Ctrl Pts',(0.00473549271943105,-0.0403412424985884,
-0.0121605639364976));
#27636=CARTESIAN_POINT('Ctrl Pts',(0.00473578444258578,-0.0403402172682197,
-0.0121446845106245));
#27637=CARTESIAN_POINT('Ctrl Pts',(0.0047369331751707,-0.0403382411308512,
-0.0121138258203437));
#27638=CARTESIAN_POINT('Ctrl Pts',(0.00473775776908206,-0.0403372894215712,
-0.0120988481449022));
#27639=CARTESIAN_POINT('Ctrl Pts',(0.00473986108795072,-0.0403354700358818,
-0.0120700045674296));
#27640=CARTESIAN_POINT('Ctrl Pts',(0.00474110272091954,-0.0403346013649773,
-0.0120561382338009));
#27641=CARTESIAN_POINT('Ctrl Pts',(0.00474452974249035,-0.0403325926739768,
-0.0120238735032967));
#27642=CARTESIAN_POINT('Ctrl Pts',(0.00474689101229707,-0.0403314581869107,
-0.0120054967770707));
#27643=CARTESIAN_POINT('Ctrl Pts',(0.00475602882948269,-0.0403277450889632,
-0.0119449408307062));
#27644=CARTESIAN_POINT('Ctrl Pts',(0.00476453872318097,-0.0403252185090613,
-0.0119030516012084));
#27645=CARTESIAN_POINT('Ctrl Pts',(0.00478729586255755,-0.0403198814868954,
-0.0118143325619181));
#27646=CARTESIAN_POINT('Ctrl Pts',(0.00480217272520959,-0.0403170874643592,
-0.0117677374022093));
#27647=CARTESIAN_POINT('Ctrl Pts',(0.004836235694752,-0.0403116415692896,
-0.0116791298839421));
#27648=CARTESIAN_POINT('Ctrl Pts',(0.00485509760512865,-0.0403089944262697,
-0.0116370773149042));
#27649=CARTESIAN_POINT('Ctrl Pts',(0.00488480398366416,-0.0403051653446008,
-0.0115794897132839));
#27650=CARTESIAN_POINT('Ctrl Pts',(0.00489376706054111,-0.0403040456476962,
-0.0115630235509855));
#27651=CARTESIAN_POINT('Ctrl Pts',(0.00491040869319124,-0.0403020170262455,
-0.0115340064952627));
#27652=CARTESIAN_POINT('Ctrl Pts',(0.00491794662652621,-0.0403011148206083,
-0.0115213787076834));
#27653=CARTESIAN_POINT('Ctrl Pts',(0.00493033822018665,-0.0402996528403234,
-0.0115014193281616));
#27654=CARTESIAN_POINT('Ctrl Pts',(0.0049350513299327,-0.0402991013752712,
-0.0114940015369747));
#27655=CARTESIAN_POINT('Ctrl Pts',(0.00494469910014684,-0.0402979803582356,
-0.011479161320187));
#27656=CARTESIAN_POINT('Ctrl Pts',(0.00494963566221157,-0.0402974107182029,
-0.011471740772816));
#27657=CARTESIAN_POINT('Ctrl Pts',(0.00496327391120557,-0.0402958489017943,
-0.0114517026232173));
#27658=CARTESIAN_POINT('Ctrl Pts',(0.0049721269766726,-0.0402948478511739,
-0.0114391904285324));
#27659=CARTESIAN_POINT('Ctrl Pts',(0.00502133612707275,-0.0402893640310613,
-0.0113722567160644));
#27660=CARTESIAN_POINT('Ctrl Pts',(0.00506578674114777,-0.0402846996568197,
-0.0113209879373225));
#27661=CARTESIAN_POINT('Ctrl Pts',(0.00515330688422206,-0.0402762854850955,
-0.0112350632685026));
#27662=CARTESIAN_POINT('Ctrl Pts',(0.00519495448414556,-0.0402725374139024,
-0.0111991866755963));
#27663=CARTESIAN_POINT('Ctrl Pts',(0.00525914395718843,-0.0402671742323331,
-0.0111507965466428));
#27664=CARTESIAN_POINT('Ctrl Pts',(0.00527994217087957,-0.0402654935732286,
-0.0111360812655809));
#27665=CARTESIAN_POINT('Ctrl Pts',(0.00531924561335684,-0.0402624222863743,
-0.0111100183937852));
#27666=CARTESIAN_POINT('Ctrl Pts',(0.0053376255429344,-0.0402610261596243,
-0.0110984997120659));
#27667=CARTESIAN_POINT('Ctrl Pts',(0.00536915088632124,-0.0402586968112379,
-0.0110798547561693));
#27668=CARTESIAN_POINT('Ctrl Pts',(0.00538214231516302,-0.0402577549323554,
-0.0110724787832965));
#27669=CARTESIAN_POINT('Ctrl Pts',(0.00540719955890394,-0.0402559712545489,
-0.0110588337452892));
#27670=CARTESIAN_POINT('Ctrl Pts',(0.00541924165519825,-0.0402551281995443,
-0.0110525257360996));
#27671=CARTESIAN_POINT('Ctrl Pts',(0.00545158747941527,-0.0402528994045979,
-0.0110362412378471));
#27672=CARTESIAN_POINT('Ctrl Pts',(0.00547206159725739,-0.0402515255059595,
-0.0110266130809181));
#27673=CARTESIAN_POINT('Ctrl Pts',(0.00557222838599391,-0.040244960657379,
-0.0109827508947513));
#27674=CARTESIAN_POINT('Ctrl Pts',(0.00565504138380275,-0.0402400234900514,
-0.0109562275729702));
#27675=CARTESIAN_POINT('Ctrl Pts',(0.00578220288660786,-0.0402325642945694,
-0.0109295021139085));
#27676=CARTESIAN_POINT('Ctrl Pts',(0.00582490850553635,-0.0402300747754092,
-0.0109227892860348));
#27677=CARTESIAN_POINT('Ctrl Pts',(0.00588587353753644,-0.0402264467684285,
-0.0109163839295228));
#27678=CARTESIAN_POINT('Ctrl Pts',(0.00590391357925132,-0.0402253639854568,
-0.0109148793571764));
#27679=CARTESIAN_POINT('Ctrl Pts',(0.00593628266020448,-0.0402233950372136,
-0.0109128783336088));
#27680=CARTESIAN_POINT('Ctrl Pts',(0.00595059980214547,-0.0402225150214586,
-0.0109122373589607));
#27681=CARTESIAN_POINT('Ctrl Pts',(0.00597363092048177,-0.04022108035792,
-0.010911598253091));
#27682=CARTESIAN_POINT('Ctrl Pts',(0.00598233984228549,-0.0402205334828755,
-0.0109114466155501));
#27683=CARTESIAN_POINT('Ctrl Pts',(0.00600004443411616,-0.0402194116056112,
-0.0109113212932764));
#27684=CARTESIAN_POINT('Ctrl Pts',(0.00600903953982635,-0.040218836361299,
-0.010911353607111));
#27685=CARTESIAN_POINT('Ctrl Pts',(0.00603377225323582,-0.0402172416144852,
-0.0109117063596917));
#27686=CARTESIAN_POINT('Ctrl Pts',(0.00604950493082304,-0.0402162126347371,
-0.0109122246907602));
#27687=CARTESIAN_POINT('Ctrl Pts',(0.0061458423710201,-0.0402098384888006,
-0.0109172004050394));
#27688=CARTESIAN_POINT('Ctrl Pts',(0.00622587325787001,-0.0402042417685395,
-0.0109290745724271));
#27689=CARTESIAN_POINT('Ctrl Pts',(0.0063665197513422,-0.0401943307249478,
-0.01096393621316));
#27690=CARTESIAN_POINT('Ctrl Pts',(0.0064275580821258,-0.0401900001654303,
-0.0109841000941119));
#27691=CARTESIAN_POINT('Ctrl Pts',(0.00650790904439407,-0.0401843154598997,
-0.0110176169562622));
#27692=CARTESIAN_POINT('Ctrl Pts',(0.00652876882235517,-0.040182840398907,
-0.0110269900943405));
#27693=CARTESIAN_POINT('Ctrl Pts',(0.0065630017512803,-0.0401804195353464,
-0.0110435023973629));
#27694=CARTESIAN_POINT('Ctrl Pts',(0.00657652061754807,-0.0401794634479277,
-0.0110503251805717));
#27695=CARTESIAN_POINT('Ctrl Pts',(0.00660333125990088,-0.0401775660167492,
-0.0110644659833282));
#27696=CARTESIAN_POINT('Ctrl Pts',(0.00661662035832072,-0.0401766248599926,
-0.011071783673063));
#27697=CARTESIAN_POINT('Ctrl Pts',(0.00664973530513637,-0.0401742757247778,
-0.0110908030019563));
#27698=CARTESIAN_POINT('Ctrl Pts',(0.00666937967289366,-0.0401728786595907,
-0.0111028103992557));
#27699=CARTESIAN_POINT('Ctrl Pts',(0.00675741459774797,-0.0401665822612498,
-0.011159979789202));
#27700=CARTESIAN_POINT('Ctrl Pts',(0.00682164282701327,-0.0401619034134789,
-0.0112111873792264));
#27701=CARTESIAN_POINT('Ctrl Pts',(0.00691338440002574,-0.0401545712312639,
-0.0113001864769143));
#27702=CARTESIAN_POINT('Ctrl Pts',(0.00694453757430276,-0.0401519351448475,
-0.0113338843193444));
#27703=CARTESIAN_POINT('Ctrl Pts',(0.00698572010051996,-0.0401481201158153,
-0.0113835996129995));
#27704=CARTESIAN_POINT('Ctrl Pts',(0.00699732879665733,-0.0401470030138161,
-0.0113982639307353));
#27705=CARTESIAN_POINT('Ctrl Pts',(0.00701746110916463,-0.0401449786394995,
-0.011424888161371));
#27706=CARTESIAN_POINT('Ctrl Pts',(0.00702610975923346,-0.0401440780522466,
-0.0114367494723579));
#27707=CARTESIAN_POINT('Ctrl Pts',(0.00703959790356993,-0.0401426182624365,
-0.011455941117517));
#27708=CARTESIAN_POINT('Ctrl Pts',(0.00704457116197873,-0.0401420673383676,
-0.0114631763534981));
#27709=CARTESIAN_POINT('Ctrl Pts',(0.0070544414291497,-0.0401409467378313,
-0.0114778611724585));
#27710=CARTESIAN_POINT('Ctrl Pts',(0.00705933577515871,-0.0401403769648988,
-0.0114853118879558));
#27711=CARTESIAN_POINT('Ctrl Pts',(0.00707243634367353,-0.0401388142200958,
-0.0115057220887536));
#27712=CARTESIAN_POINT('Ctrl Pts',(0.00708048594282326,-0.0401378123555242,
-0.0115187797649281));
#27713=CARTESIAN_POINT('Ctrl Pts',(0.00711409794524443,-0.0401334548791656,
-0.0115755918612047));
#27714=CARTESIAN_POINT('Ctrl Pts',(0.00713725348116252,-0.0401299997159101,
-0.0116207121017299));
#27715=CARTESIAN_POINT('Ctrl Pts',(0.00717947034994673,-0.0401228062373415,
-0.01171677327409));
#27716=CARTESIAN_POINT('Ctrl Pts',(0.00719808325444494,-0.0401190732544188,
-0.0117678070107088));
#27717=CARTESIAN_POINT('Ctrl Pts',(0.00722722024219893,-0.0401120758577486,
-0.011867122544748));
#27718=CARTESIAN_POINT('Ctrl Pts',(0.00723831046276647,-0.0401088055543218,
-0.0119151382140673));
#27719=CARTESIAN_POINT('Ctrl Pts',(0.00724978609844917,-0.0401043799255059,
-0.0119825616146551));
#27720=CARTESIAN_POINT('Ctrl Pts',(0.00725257010034125,-0.0401031536918412,
-0.0120015111804207));
#27721=CARTESIAN_POINT('Ctrl Pts',(0.00725671266056455,-0.0401010176302278,
-0.0120349779954311));
#27722=CARTESIAN_POINT('Ctrl Pts',(0.00725825257418958,-0.0401001024217962,
-0.0120494687684206));
#27723=CARTESIAN_POINT('Ctrl Pts',(0.00726098865407339,-0.0400981760496522,
-0.0120802742635309));
#27724=CARTESIAN_POINT('Ctrl Pts',(0.00726211942864145,-0.0400971670422458,
-0.0120965921922759));
#27725=CARTESIAN_POINT('Ctrl Pts',(0.00726435918403415,-0.0400944154724462,
-0.0121415449430569));
#27726=CARTESIAN_POINT('Ctrl Pts',(0.00726481202684669,-0.0400926927167552,
-0.0121702033736002));
#27727=CARTESIAN_POINT('Ctrl Pts',(0.00726243583940873,-0.0400849427395138,
-0.0123008158959845));
#27728=CARTESIAN_POINT('Ctrl Pts',(0.00724825423884516,-0.0400792444492893,
-0.0124021729668372));
#27729=CARTESIAN_POINT('Ctrl Pts',(0.00721527190557364,-0.0400717691464125,
-0.0125262409220381));
#27730=CARTESIAN_POINT('Ctrl Pts',(0.00720769174409166,-0.0400702154599285,
-0.012551536403038));
#27731=CARTESIAN_POINT('Ctrl Pts',(0.00719337014596564,-0.0400675037772246,
-0.0125943997583817));
#27732=CARTESIAN_POINT('Ctrl Pts',(0.00718701807920654,-0.0400663610634193,
-0.0126120888342709));
#27733=CARTESIAN_POINT('Ctrl Pts',(0.00717683320091959,-0.0400646045656637,
-0.0126385798058883));
#27734=CARTESIAN_POINT('Ctrl Pts',(0.00717329023461174,-0.0400640058384437,
-0.0126474910993906));
#27735=CARTESIAN_POINT('Ctrl Pts',(0.007166456822607,-0.0400628719191018,
-0.012664124916019));
#27736=CARTESIAN_POINT('Ctrl Pts',(0.00716319026798234,-0.0400623380319494,
-0.012671856399086));
#27737=CARTESIAN_POINT('Ctrl Pts',(0.00715484355182419,-0.040060994424708,
-0.0126910759576779));
#27738=CARTESIAN_POINT('Ctrl Pts',(0.00714966880082104,-0.0400601795575952,
-0.0127025217310663));
#27739=CARTESIAN_POINT('Ctrl Pts',(0.00712695889102837,-0.0400566836118754,
-0.0127508225356729));
#27740=CARTESIAN_POINT('Ctrl Pts',(0.00710781655954294,-0.0400539304569279,
-0.0127868916479098));
#27741=CARTESIAN_POINT('Ctrl Pts',(0.00703609736103444,-0.0400443593058478,
-0.0129075454907999));
#27742=CARTESIAN_POINT('Ctrl Pts',(0.00697529151291681,-0.0400374606480069,
-0.012986829619674));
#27743=CARTESIAN_POINT('Ctrl Pts',(0.0068858809777128,-0.0400290046129356,
-0.0130786217716277));
#27744=CARTESIAN_POINT('Ctrl Pts',(0.0068652630524394,-0.0400271460533999,
-0.0130984019844701));
#27745=CARTESIAN_POINT('Ctrl Pts',(0.00683193544471295,-0.0400242792359711,
-0.0131282742994764));
#27746=CARTESIAN_POINT('Ctrl Pts',(0.00681967256508146,-0.0400232516384117,
-0.0131388482475118));
#27747=CARTESIAN_POINT('Ctrl Pts',(0.00679596562509729,-0.0400213148444947,
-0.0131585090514449));
#27748=CARTESIAN_POINT('Ctrl Pts',(0.00678456063817248,-0.0400204040437298,
-0.0131676386773921));
#27749=CARTESIAN_POINT('Ctrl Pts',(0.00675785794922321,-0.0400183176685875,
-0.0131882650847784));
#27750=CARTESIAN_POINT('Ctrl Pts',(0.00674245219865486,-0.0400171477600379,
-0.0131996164972148));
#27751=CARTESIAN_POINT('Ctrl Pts',(0.00668813968113017,-0.0400131309187555,
-0.0132377644511274));
#27752=CARTESIAN_POINT('Ctrl Pts',(0.00664799219032947,-0.0400103494101557,
-0.0132627287563542));
#27753=CARTESIAN_POINT('Ctrl Pts',(0.00651827557113986,-0.0400017710078011,
-0.0133336395802402));
#27754=CARTESIAN_POINT('Ctrl Pts',(0.00642458109009128,-0.0399961688950079,
-0.013371179821941));
#27755=CARTESIAN_POINT('Ctrl Pts',(0.00630922579312222,-0.039989003941938,
-0.0134021058327556));
#27756=CARTESIAN_POINT('Ctrl Pts',(0.00629090447206087,-0.039987857430459,
-0.0134065808781319));
#27757=CARTESIAN_POINT('Ctrl Pts',(0.00626311524426538,-0.0399860963314647,
-0.0134127133450927));
#27758=CARTESIAN_POINT('Ctrl Pts',(0.00625371654119853,-0.0399854969227135,
-0.0134146754446956));
#27759=CARTESIAN_POINT('Ctrl Pts',(0.00623606578631421,-0.0399843626299647,
-0.0134181509844042));
#27760=CARTESIAN_POINT('Ctrl Pts',(0.00622781950864395,-0.0399838290695727,
-0.0134196896427894));
#27761=CARTESIAN_POINT('Ctrl Pts',(0.00620721657688126,-0.0399824876598383,
-0.013423322166915));
#27762=CARTESIAN_POINT('Ctrl Pts',(0.00619484316552589,-0.0399816746997847,
-0.0134253145425432));
#27763=CARTESIAN_POINT('Ctrl Pts',(0.0061424087369798,-0.0399782042462449,
-0.013432959804256));
#27764=CARTESIAN_POINT('Ctrl Pts',(0.00610212090450855,-0.0399754759248984,
-0.0134368718456499));
#27765=CARTESIAN_POINT('Ctrl Pts',(0.00598405628191336,-0.0399674172022816,
-0.0134426413127285));
#27766=CARTESIAN_POINT('Ctrl Pts',(0.0059062028711642,-0.0399620346527578,
-0.013439265177324));
#27767=CARTESIAN_POINT('Ctrl Pts',(0.00579953294236739,-0.0399547953882157,
-0.0134247194921208));
#27768=CARTESIAN_POINT('Ctrl Pts',(0.00577006500849551,-0.039952808313091,
-0.0134196313816113));
#27769=CARTESIAN_POINT('Ctrl Pts',(0.00571697847431758,-0.0399492560618952,
-0.0134085136556847));
#27770=CARTESIAN_POINT('Ctrl Pts',(0.00569330146227426,-0.0399476817606314,
-0.0134028369481928));
#27771=CARTESIAN_POINT('Ctrl Pts',(0.0056549252033243,-0.0399451452244423,
-0.0133924555803342));
#27772=CARTESIAN_POINT('Ctrl Pts',(0.00564012298897309,-0.0399441705532669,
-0.0133881594883199));
#27773=CARTESIAN_POINT('Ctrl Pts',(0.00561129287905744,-0.0399422783234251,
-0.0133792174278886));
#27774=CARTESIAN_POINT('Ctrl Pts',(0.00559726062251742,-0.0399413602208137,
-0.0133745940862731));
#27775=CARTESIAN_POINT('Ctrl Pts',(0.00556292993124942,-0.0399391192669821,
-0.0133626119165037));
#27776=CARTESIAN_POINT('Ctrl Pts',(0.00554273242799329,-0.0399378054813009,
-0.0133549770036265));
#27777=CARTESIAN_POINT('Ctrl Pts',(0.00543462590048533,-0.0399307805007482,
-0.0133109154432584));
#27778=CARTESIAN_POINT('Ctrl Pts',(0.00535084788926817,-0.0399253903871653,
-0.0132651727866826));
#27779=CARTESIAN_POINT('Ctrl Pts',(0.00524098846071442,-0.0399176686138853,
-0.0131879755351449));
#27780=CARTESIAN_POINT('Ctrl Pts',(0.00521004976903454,-0.039915405479245,
-0.0131640173708914));
#27781=CARTESIAN_POINT('Ctrl Pts',(0.00516172695295846,-0.039911639677013,
-0.0131228758919729));
#27782=CARTESIAN_POINT('Ctrl Pts',(0.00514364238231976,-0.0399101728170191,
-0.0131065546277538));
#27783=CARTESIAN_POINT('Ctrl Pts',(0.00511843279369019,-0.039908024690825,
-0.0130824460027521));
#27784=CARTESIAN_POINT('Ctrl Pts',(0.00511091542744187,-0.0399073702699722,
-0.0130750750045097));
#27785=CARTESIAN_POINT('Ctrl Pts',(0.00509768393009534,-0.0399061914819535,
-0.0130617730180069));
#27786=CARTESIAN_POINT('Ctrl Pts',(0.00509193427140479,-0.0399056697642076,
-0.0130558786739378));
#27787=CARTESIAN_POINT('Ctrl Pts',(0.00507873376660814,-0.0399044497631946,
-0.0130420788784797));
#27788=CARTESIAN_POINT('Ctrl Pts',(0.00507132675034842,-0.039903748547216,
-0.0130341330925903));
#27789=CARTESIAN_POINT('Ctrl Pts',(0.00504738415814247,-0.0399014294509445,
-0.0130077761693709));
#27790=CARTESIAN_POINT('Ctrl Pts',(0.00503128737206398,-0.0398997861222379,
-0.0129889758497332));
#27791=CARTESIAN_POINT('Ctrl Pts',(0.00495740729654985,-0.0398918758387407,
-0.0128973779929062));
#27792=CARTESIAN_POINT('Ctrl Pts',(0.00490721296573304,-0.039885396782596,
-0.0128188271002635));
#27793=CARTESIAN_POINT('Ctrl Pts',(0.00485197528692502,-0.0398769790983398,
-0.0127069041849032));
#27794=CARTESIAN_POINT('Ctrl Pts',(0.00483895619389082,-0.0398748546039561,
-0.0126778028119593));
#27795=CARTESIAN_POINT('Ctrl Pts',(0.0048175340927321,-0.0398710908308532,
-0.012624610959997));
#27796=CARTESIAN_POINT('Ctrl Pts',(0.00480873401065512,-0.0398694405380058,
-0.0126006998018542));
#27797=CARTESIAN_POINT('Ctrl Pts',(0.00479571193713884,-0.0398668154278319,
-0.0125617218165928));
#27798=CARTESIAN_POINT('Ctrl Pts',(0.00479103692849374,-0.0398658264381139,
-0.0125468149925733));
#27799=CARTESIAN_POINT('Ctrl Pts',(0.00478251409657398,-0.0398639267311554,
-0.0125177641570955));
#27800=CARTESIAN_POINT('Ctrl Pts',(0.00477863361939101,-0.0398630151078194,
-0.0125036324205847));
#27801=CARTESIAN_POINT('Ctrl Pts',(0.00476983207840232,-0.0398608253939452,
-0.0124692494871266));
#27802=CARTESIAN_POINT('Ctrl Pts',(0.00476516418664008,-0.0398595553602545,
-0.0124489375850342));
#27803=CARTESIAN_POINT('Ctrl Pts',(0.0047440354368581,-0.0398531807795075,
-0.0123453281619604));
#27804=CARTESIAN_POINT('Ctrl Pts',(0.00473550000701352,-0.0398483286333551,
-0.0122606813520481));
#27805=CARTESIAN_POINT('Ctrl Pts',(0.0047355,-0.0398434635507866,-0.0121758533911061));
#27806=CARTESIAN_POINT('Ctrl Pts',(0.00473550000001467,-0.0399058329518585,
-0.0121758593776931));
#27807=CARTESIAN_POINT('Ctrl Pts',(0.00473550140307262,-0.0399241615430135,
-0.0124671296870887));
#27808=CARTESIAN_POINT('Ctrl Pts',(0.00484035537256781,-0.0399424901341685,
-0.0127578883555264));
#27809=CARTESIAN_POINT('Ctrl Pts',(0.00502575436044838,-0.0399608187253235,
-0.0129819585425977));
#27810=CARTESIAN_POINT('Ctrl Pts',(0.00505106586813013,-0.0399633210274187,
-0.0130125496171561));
#27811=CARTESIAN_POINT('Ctrl Pts',(0.00507780576562169,-0.0399658233295138,
-0.0130419311106039));
#27812=CARTESIAN_POINT('Ctrl Pts',(0.00510584767754908,-0.039968325631609,
-0.0130699740134488));
#27813=CARTESIAN_POINT('Ctrl Pts',(0.00530746131447154,-0.039986316495691,
-0.013271594774796));
#27814=CARTESIAN_POINT('Ctrl Pts',(0.00558088995559621,-0.040004307359773,
-0.0134026189102355));
#27815=CARTESIAN_POINT('Ctrl Pts',(0.00586499593047847,-0.0400222982238551,
-0.013433125791313));
#27816=CARTESIAN_POINT('Ctrl Pts',(0.00590984476329907,-0.0400251382530232,
-0.0134379415929162));
#27817=CARTESIAN_POINT('Ctrl Pts',(0.00595491931973503,-0.0400279782821913,
-0.0134403514774338));
#27818=CARTESIAN_POINT('Ctrl Pts',(0.00599994922599528,-0.0400308183113595,
-0.0134403532855387));
#27819=CARTESIAN_POINT('Ctrl Pts',(0.0062862573739437,-0.0400488757216182,
-0.0134403647817912));
#27820=CARTESIAN_POINT('Ctrl Pts',(0.00657319492440129,-0.0400669331318769,
-0.0133388846850336));
#27821=CARTESIAN_POINT('Ctrl Pts',(0.00679601016042393,-0.0400849905421356,
-0.013158364393112));
#27822=CARTESIAN_POINT('Ctrl Pts',(0.00683023291210797,-0.0400877640251271,
-0.013130637828113));
#27823=CARTESIAN_POINT('Ctrl Pts',(0.0068629826641763,-0.0400905375081185,
-0.0131011397728834));
#27824=CARTESIAN_POINT('Ctrl Pts',(0.00689408051555027,-0.0400933109911099,
-0.0130700458171204));
#27825=CARTESIAN_POINT('Ctrl Pts',(0.00709651233115139,-0.0401113650100434,
-0.0128676393600427));
#27826=CARTESIAN_POINT('Ctrl Pts',(0.00722764341798178,-0.0401294190289768,
-0.0125930456480888));
#27827=CARTESIAN_POINT('Ctrl Pts',(0.00725758525939554,-0.0401474730479103,
-0.0123079122330595));
#27828=CARTESIAN_POINT('Ctrl Pts',(0.00726219059024867,-0.040150249922227,
-0.0122640560888983));
#27829=CARTESIAN_POINT('Ctrl Pts',(0.00726449624762511,-0.0401530267965437,
-0.0122199884489719));
#27830=CARTESIAN_POINT('Ctrl Pts',(0.00726449999541867,-0.0401558036708604,
-0.0121759609257025));
#27831=CARTESIAN_POINT('Ctrl Pts',(0.00726452436192866,-0.040173857689794,
-0.0118897132788708));
#27832=CARTESIAN_POINT('Ctrl Pts',(0.00716309785865325,-0.0401919117087277,
-0.0116028192306949));
#27833=CARTESIAN_POINT('Ctrl Pts',(0.00698264882413635,-0.0402099657276614,
-0.0113800131402828));
#27834=CARTESIAN_POINT('Ctrl Pts',(0.00695489410142147,-0.0402127426019779,
-0.011345743512434));
#27835=CARTESIAN_POINT('Ctrl Pts',(0.0069253633130834,-0.0402155194762944,
-0.0113129502609626));
#27836=CARTESIAN_POINT('Ctrl Pts',(0.00689423273686524,-0.0402182963506109,
-0.0112818129841564));
#27837=CARTESIAN_POINT('Ctrl Pts',(0.00669179736447306,-0.0402363537608694,
-0.0110793340392964));
#27838=CARTESIAN_POINT('Ctrl Pts',(0.00641714955401632,-0.0402544111711278,
-0.0109481820350889));
#27839=CARTESIAN_POINT('Ctrl Pts',(0.00613195713696627,-0.0402724685813862,
-0.0109182573403164));
#27840=CARTESIAN_POINT('Ctrl Pts',(0.00608815371738732,-0.0402752420643779,
-0.0109136611312921));
#27841=CARTESIAN_POINT('Ctrl Pts',(0.00604413929143607,-0.0402780155473697,
-0.0109113590181293));
#27842=CARTESIAN_POINT('Ctrl Pts',(0.00600016450428374,-0.0402807890303614,
-0.0109113532972586));
#27843=CARTESIAN_POINT('Ctrl Pts',(0.00571491147729529,-0.0402987798944434,
-0.0109113161874561));
#27844=CARTESIAN_POINT('Ctrl Pts',(0.00542891591239803,-0.0403167707585254,
-0.0110120582582409));
#27845=CARTESIAN_POINT('Ctrl Pts',(0.00520650781506261,-0.0403347616226074,
-0.0111913075017196));
#27846=CARTESIAN_POINT('Ctrl Pts',(0.00517139857957576,-0.0403376016517755,
-0.0112196037012534));
#27847=CARTESIAN_POINT('Ctrl Pts',(0.00513783196264546,-0.0403404416809437,
-0.0112497580074664));
#27848=CARTESIAN_POINT('Ctrl Pts',(0.00510599991255491,-0.0403432817101119,
-0.0112815803451984));
#27849=CARTESIAN_POINT('Ctrl Pts',(0.00490056658874369,-0.0403616103012668,
-0.0114869509887204));
#27850=CARTESIAN_POINT('Ctrl Pts',(0.00476865909976607,-0.0403799388924218,
-0.011766355214167));
#27851=CARTESIAN_POINT('Ctrl Pts',(0.00474114731563261,-0.0403982674835768,
-0.0120564792145784));
#27852=CARTESIAN_POINT('Ctrl Pts',(0.00473739128253129,-0.040400769785672,
-0.0120960882542447));
#27853=CARTESIAN_POINT('Ctrl Pts',(0.00473550698092259,-0.0404032720877671,
-0.012135866378795));
#27854=CARTESIAN_POINT('Ctrl Pts',(0.004735500019377,-0.0404057743898623,
-0.0121756319171353));
#27855=CARTESIAN_POINT('Origin',(-0.015,-0.0412787743898723,-0.0201758532865581));
#27856=CARTESIAN_POINT('',(-0.015,-0.0379787743898623,-0.00457585328655813));
#27857=CARTESIAN_POINT('',(-0.0149999999999975,-0.0408787743898673,-0.00457585328656563));
#27858=CARTESIAN_POINT('',(-0.015,-0.0412787743898723,-0.00457585328656813));
#27859=CARTESIAN_POINT('',(-0.015,-0.0379787743898723,-0.0197758532865581));
#27860=CARTESIAN_POINT('',(-0.015,-0.0379787743898623,-0.0121758532865681));
#27861=CARTESIAN_POINT('',(-0.015,-0.0408787743898723,-0.0197758532865581));
#27862=CARTESIAN_POINT('',(-0.015,-0.0412787743898723,-0.0197758532865681));
#27863=CARTESIAN_POINT('',(-0.015,-0.0408787743898623,-0.0161758532865681));
#27864=CARTESIAN_POINT('Origin',(-0.0148,-0.0410787743898723,-0.0161758532865581));
#27865=CARTESIAN_POINT('',(-0.0145999999999925,-0.0412787743898673,-0.00457585328656563));
#27866=CARTESIAN_POINT('',(-0.01459999999999,-0.0412787743898723,-0.00457585328656813));
#27867=CARTESIAN_POINT('',(-0.0146,-0.0412787743898723,-0.0197758532865581));
#27868=CARTESIAN_POINT('',(-0.015,-0.0408787743898623,-0.0197758532865681));
#27869=CARTESIAN_POINT('',(-0.01459999999999,-0.0412787743898723,-0.0161758532865681));
#27870=CARTESIAN_POINT('Origin',(-0.0148,-0.0412787743898723,-0.0199758532865582));
#27871=CARTESIAN_POINT('',(-0.0146,-0.0379787743898723,-0.0201758532865581));
#27872=CARTESIAN_POINT('',(-0.0174042976073008,-0.0379787743898623,-0.0173715556792775));
#27873=CARTESIAN_POINT('',(-0.0146,-0.0408787743898723,-0.0201758532865581));
#27874=CARTESIAN_POINT('',(-0.01459999999999,-0.0412787743898723,-0.0201758532865681));
#27875=CARTESIAN_POINT('',(-0.01459999999999,-0.0408787743898623,-0.0201758532865681));
#27876=CARTESIAN_POINT('Origin',(-0.00941719042916296,-0.0379787743898723,
-0.00417585328655812));
#27877=CARTESIAN_POINT('',(-0.00982716095192005,-0.0379787743898677,-0.0201758532865654));
#27878=CARTESIAN_POINT('',(-0.00941719042915764,-0.0379787743898678,-0.0197758532865628));
#27879=CARTESIAN_POINT('Ctrl Pts',(-0.00941719042916247,-0.0379787743898723,
-0.0197758532865577));
#27880=CARTESIAN_POINT('Ctrl Pts',(-0.00960936411170753,-0.0379787743898723,
-0.0199627223623769));
#27881=CARTESIAN_POINT('Ctrl Pts',(-0.00982716095192546,-0.0379787743898723,
-0.0201758532865608));
#27882=CARTESIAN_POINT('',(-0.000708595214571501,-0.0379787743898623,-0.0201758532865681));
#27883=CARTESIAN_POINT('',(-0.0145999999999967,-0.0379787743898656,-0.00417585328655812));
#27884=CARTESIAN_POINT('',(-0.0134042976072807,-0.0379787743898623,-0.00298015089383886));
#27885=CARTESIAN_POINT('',(-0.00982716095192005,-0.0379787743898677,-0.00417585328655585));
#27886=CARTESIAN_POINT('',(-0.0122085952145715,-0.0379787743898623,-0.00417585328655812));
#27887=CARTESIAN_POINT('',(-0.00941719042915521,-0.0379787743898672,-0.00457585328656588));
#27888=CARTESIAN_POINT('Ctrl Pts',(-0.00982716095192254,-0.0379787743898723,
-0.0041758532865584));
#27889=CARTESIAN_POINT('Ctrl Pts',(-0.00960936411170209,-0.0379787743898723,
-0.00438898421074477));
#27890=CARTESIAN_POINT('Ctrl Pts',(-0.0094171904291551,-0.0379787743898723,
-0.00457585328656577));
#27891=CARTESIAN_POINT('',(-0.00941719042915296,-0.0379787743898623,-0.00417585328655812));
#27892=CARTESIAN_POINT('',(-0.014,-0.0379787743898623,-0.0121758532865581));
#27893=CARTESIAN_POINT('Origin',(-0.01249999999999,-0.0379787743898623,
-0.0121758532865681));
#27894=CARTESIAN_POINT('Origin',(-0.0148,-0.0412787743898723,-0.00437585328655813));
#27895=CARTESIAN_POINT('',(-0.01459999999999,-0.040878774389866,-0.00417585328655938));
#27896=CARTESIAN_POINT('',(-0.015,-0.0408787743898623,-0.00457585328656813));
#27897=CARTESIAN_POINT('',(-0.01459999999999,-0.0412787743898723,-0.00417585328655813));
#27898=CARTESIAN_POINT('Origin',(-0.0035,-0.0412787743898723,-0.0121758532865581));
#27899=CARTESIAN_POINT('',(0.007600000000005,-0.0412787743898698,-0.00457585328656563));
#27900=CARTESIAN_POINT('',(0.0076,-0.0412787743898723,-0.0116013970219043));
#27901=CARTESIAN_POINT('',(0.00760000000001,-0.0412787743898723,-0.00817585328656813));
#27902=CARTESIAN_POINT('',(-0.00924999999999,-0.0412787743898723,-0.00457585328656813));
#27903=CARTESIAN_POINT('',(0.0076,-0.0412787743898723,-0.0197758532865581));
#27904=CARTESIAN_POINT('',(0.00225000000001,-0.0412787743898723,-0.0197758532865681));
#27905=CARTESIAN_POINT('',(0.0076,-0.0412787743898723,-0.0127503095512119));
#27906=CARTESIAN_POINT('',(0.00760000000001,-0.0412787743898723,-0.00817585328656813));
#27907=CARTESIAN_POINT('',(0.0042999999999872,-0.0412787743898851,-0.0121758532865581));
#27908=CARTESIAN_POINT('Origin',(0.00600000000001,-0.0412787743898723,-0.0121758532865681));
#27909=CARTESIAN_POINT('Origin',(0.00600000000001,-0.0412787743898723,-0.0121758532865681));
#27910=CARTESIAN_POINT('',(-0.00320000000001261,-0.0412787743898849,-0.0121758532865581));
#27911=CARTESIAN_POINT('Origin',(1.00006808390063E-14,-0.0412787743898723,
-0.0121758532865681));
#27912=CARTESIAN_POINT('',(-0.0142000000000126,-0.0412787743898849,-0.0121758532865581));
#27913=CARTESIAN_POINT('Origin',(-0.01249999999999,-0.0412787743898723,
-0.0121758532865681));
#27914=CARTESIAN_POINT('Origin',(-0.015,-0.0408787743898723,-0.0197758532865581));
#27915=CARTESIAN_POINT('',(-0.01459999999999,-0.0412787743898723,-0.0197758532865681));
#27916=CARTESIAN_POINT('Origin',(-0.0146,-0.0412787743898723,-0.00457585328655813));
#27917=CARTESIAN_POINT('',(-0.01459999999999,-0.0408787743898623,-0.00417585328655813));
#27918=CARTESIAN_POINT('Origin',(0.008,-0.0412787743898723,-0.0201758532865581));
#27919=CARTESIAN_POINT('',(0.00760000000000835,-0.03664344923035,-0.0201758532865647));
#27920=CARTESIAN_POINT('',(0.00404999999998256,-0.0355287743898723,-0.0201758532865756));
#27921=CARTESIAN_POINT('Origin',(0.00600000000001,-0.0355287743898623,-0.0201758532865681));
#27922=CARTESIAN_POINT('',(0.0076,-0.0408787743898723,-0.0201758532865581));
#27923=CARTESIAN_POINT('',(0.00760000000001,-0.0412787743898723,-0.0201758532865681));
#27924=CARTESIAN_POINT('',(0.00225000000001,-0.0408787743898623,-0.0201758532865681));
#27925=CARTESIAN_POINT('',(-0.00982716095192098,-0.0365787743898654,-0.0201758532865681));
#27926=CARTESIAN_POINT('Origin',(-0.00649999999999,-0.0372787743898623,
-0.0201758532865681));
#27927=CARTESIAN_POINT('',(-0.0146,-0.0365787743898723,-0.0201758532865581));
#27928=CARTESIAN_POINT('',(-0.00349999999999,-0.0365787743898623,-0.0201758532865681));
#27929=CARTESIAN_POINT('',(-0.0146,-0.0301787743898723,-0.0201758532865581));
#27930=CARTESIAN_POINT('',(-0.01459999999999,-0.0412787743898723,-0.0201758532865681));
#27931=CARTESIAN_POINT('',(0.0076,-0.0301787743898723,-0.0201758532865581));
#27932=CARTESIAN_POINT('',(0.00225000000001,-0.0301787743898623,-0.0201758532865681));
#27933=CARTESIAN_POINT('',(0.0076000000000095,-0.0344140995493838,-0.0201758532865661));
#27934=CARTESIAN_POINT('',(0.00760000000001,-0.0412787743898723,-0.0201758532865681));
#27935=CARTESIAN_POINT('Origin',(0.00600000000001,-0.0355287743898623,-0.0201758532865681));
#27936=CARTESIAN_POINT('Origin',(-0.0125,-0.0412787743898723,-0.0121758532865581));
#27937=CARTESIAN_POINT('',(-0.014,-0.0410787743898623,-0.0121758532865581));
#27938=CARTESIAN_POINT('Origin',(-0.01249999999999,-0.0410787743898623,
-0.0121758532865681));
#27939=CARTESIAN_POINT('',(-0.014,-0.0412787743898723,-0.0121758532865581));
#27940=CARTESIAN_POINT('Origin',(-0.0065,-0.0372787743898723,-0.00417585328655812));
#27941=CARTESIAN_POINT('',(-0.00941719042915714,-0.0365787743898654,-0.0197758532865648));
#27942=CARTESIAN_POINT('Origin',(-0.00649999999999,-0.0372787743898623,
-0.0197758532865681));
#27943=CARTESIAN_POINT('',(-0.00941719042915714,-0.0365787743898654,-0.00457585328656813));
#27944=CARTESIAN_POINT('Origin',(-0.00649999999999,-0.0372787743898623,
-0.00457585328656813));
#27945=CARTESIAN_POINT('',(-0.00941719042915296,-0.0365787743898623,-0.00417585328655812));
#27946=CARTESIAN_POINT('Origin',(-0.0065,-0.0372787743898723,-0.00437585328655812));
#27947=CARTESIAN_POINT('',(-0.00982716095192024,-0.0365787743898655,-0.00417585328655479));
#27948=CARTESIAN_POINT('Origin',(-0.00649999999999,-0.0372787743898623,
-0.00417585328655812));
#27949=CARTESIAN_POINT('Ctrl Pts',(-0.00982716095192317,-0.0365787743898723,
-0.00417585328655778));
#27950=CARTESIAN_POINT('Ctrl Pts',(-0.00960936411170229,-0.0365787743898723,
-0.00438898421074458));
#27951=CARTESIAN_POINT('Ctrl Pts',(-0.00941719042915497,-0.0365787743898723,
-0.0045758532865659));
#27952=CARTESIAN_POINT('Origin',(-0.015,-0.0412787743898723,-0.00417585328655813));
#27953=CARTESIAN_POINT('',(0.00760000000001035,-0.034414099549385,-0.00417585328655513));
#27954=CARTESIAN_POINT('',(0.00404999999998751,-0.0355287743898723,-0.00417585328654563));
#27955=CARTESIAN_POINT('Origin',(0.00600000000001,-0.0355287743898623,-0.00417585328655812));
#27956=CARTESIAN_POINT('',(0.007600000000005,-0.0301787743898623,-0.00417585328655812));
#27957=CARTESIAN_POINT('',(0.00760000000001,-0.0412787743898723,-0.00417585328655813));
#27958=CARTESIAN_POINT('',(-0.01459999999999,-0.0301787743898673,-0.00417585328655812));
#27959=CARTESIAN_POINT('',(-0.00924999999999,-0.0301787743898623,-0.00417585328655812));
#27960=CARTESIAN_POINT('',(-0.0145999999999933,-0.0365787743898623,-0.00417585328656146));
#27961=CARTESIAN_POINT('',(-0.01459999999999,-0.0412787743898723,-0.00417585328655813));
#27962=CARTESIAN_POINT('',(-0.015,-0.0365787743898623,-0.00417585328655812));
#27963=CARTESIAN_POINT('',(0.00760000000000625,-0.0408787743898623,-0.00417585328655688));
#27964=CARTESIAN_POINT('',(-0.00924999999999,-0.0408787743898623,-0.00417585328655813));
#27965=CARTESIAN_POINT('',(0.00760000000000835,-0.03664344923035,-0.00417585328655657));
#27966=CARTESIAN_POINT('',(0.00760000000001,-0.0412787743898723,-0.00417585328655813));
#27967=CARTESIAN_POINT('Origin',(0.00600000000001,-0.0355287743898623,-0.00417585328655812));
#27968=CARTESIAN_POINT('Origin',(-0.0065,-0.0372787743898723,-0.0199758532865582));
#27969=CARTESIAN_POINT('Ctrl Pts',(-0.00941719042916361,-0.0365787743898723,
-0.0197758532865588));
#27970=CARTESIAN_POINT('Ctrl Pts',(-0.00960936411170878,-0.0365787743898723,
-0.0199627223623781));
#27971=CARTESIAN_POINT('Ctrl Pts',(-0.00982716095192684,-0.0365787743898723,
-0.0201758532865621));
#27972=CARTESIAN_POINT('Origin',(-0.0125,-0.0411787743898723,-0.0121758532865581));
#27973=CARTESIAN_POINT('',(-0.0141,-0.0411787743898723,-0.0121758532865581));
#27974=CARTESIAN_POINT('Origin',(0.,-0.0411787743898723,-0.0121758532865581));
#27975=CARTESIAN_POINT('',(-0.00249999922097496,-0.0405787743898623,-0.012173879679554));
#27976=CARTESIAN_POINT('',(-0.00176776695296376,-0.0405787743898673,-0.0104080863335944));
#27977=CARTESIAN_POINT('Origin',(1.00006808390063E-14,-0.0405787743898623,
-0.0121758532865681));
#27978=CARTESIAN_POINT('Origin',(1.00006808390063E-14,-0.0405787743898623,
-0.0121758532865681));
#27979=CARTESIAN_POINT('',(-0.0031,-0.0411787743898723,-0.0121758532865581));
#27980=CARTESIAN_POINT('Origin',(0.006,-0.0411787743898723,-0.0121758532865581));
#27981=CARTESIAN_POINT('Origin',(0.00600000000001,-0.0408432743898623,-0.0121758532865681));
#27982=CARTESIAN_POINT('',(0.0044,-0.0411787743898723,-0.0121758532865581));
#27983=CARTESIAN_POINT('Ctrl Pts',(0.00760000000001,-0.0412787743898623,
-0.0116013970219143));
#27984=CARTESIAN_POINT('Ctrl Pts',(0.00770000000001,-0.0411787743898623,
-0.0121758532865681));
#27985=CARTESIAN_POINT('Ctrl Pts',(0.00760000000001,-0.0412787743898623,
-0.0127503095512219));
#27986=CARTESIAN_POINT('Origin',(0.0078,-0.0410787743898723,-0.00817585328655813));
#27987=CARTESIAN_POINT('',(0.008,-0.0408787743898723,-0.0197758532865581));
#27988=CARTESIAN_POINT('',(0.00760000000001,-0.0412787743898723,-0.0197758532865681));
#27989=CARTESIAN_POINT('',(0.00800000000000625,-0.0408787743898673,-0.0045758532865625));
#27990=CARTESIAN_POINT('',(0.00800000000001,-0.0408787743898623,-0.00817585328656813));
#27991=CARTESIAN_POINT('',(0.00800000000001,-0.0408787743898623,-0.00457585328656813));
#27992=CARTESIAN_POINT('Origin',(0.00225,-0.0410787743898723,-0.0199758532865582));
#27993=CARTESIAN_POINT('',(0.00760000000001,-0.0408787743898623,-0.0201758532865681));
#27994=CARTESIAN_POINT('Origin',(-0.00925,-0.0410787743898723,-0.00437585328655813));
#27995=CARTESIAN_POINT('',(0.00760000000001,-0.0412787743898723,-0.00457585328656813));
#27996=CARTESIAN_POINT('Origin',(0.0078,-0.0412787743898723,-0.0199758532865582));
#27997=CARTESIAN_POINT('Ctrl Pts',(0.0076,-0.0366434492303427,-0.0201758532865581));
#27998=CARTESIAN_POINT('Ctrl Pts',(0.00783333333333333,-0.0359003326700224,
-0.0199425199532248));
#27999=CARTESIAN_POINT('Ctrl Pts',(0.00783333333333333,-0.0351572161097022,
-0.0199425199532248));
#28000=CARTESIAN_POINT('Ctrl Pts',(0.0076,-0.0344140995493819,-0.0201758532865581));
#28001=CARTESIAN_POINT('',(0.00800000000001126,-0.0301787743898623,-0.0197758532865643));
#28002=CARTESIAN_POINT('',(0.00760000000001,-0.0301787743898623,-0.0201758532865681));
#28003=CARTESIAN_POINT('',(0.00800000000001,-0.0412787743898723,-0.0197758532865681));
#28004=CARTESIAN_POINT('',(0.00800000000001,-0.0408787743898623,-0.0197758532865681));
#28005=CARTESIAN_POINT('Origin',(0.00225,-0.0299787743898723,-0.0199758532865581));
#28006=CARTESIAN_POINT('',(-0.0145999999999931,-0.0297787743898623,-0.019775853286565));
#28007=CARTESIAN_POINT('',(-0.01459999999999,-0.0301787743898623,-0.0201758532865681));
#28008=CARTESIAN_POINT('',(0.00760000000001,-0.0297787743898617,-0.0197758532865649));
#28009=CARTESIAN_POINT('',(0.00225000000001,-0.0297787743898623,-0.0197758532865681));
#28010=CARTESIAN_POINT('',(0.00760000000001,-0.0297787743898623,-0.0197758532865681));
#28011=CARTESIAN_POINT('Origin',(-0.0148,-0.0412787743898723,-0.0199758532865582));
#28012=CARTESIAN_POINT('',(-0.015,-0.0365787743898723,-0.0197758532865581));
#28013=CARTESIAN_POINT('',(-0.01880000000001,-0.0365787743898623,-0.0159758532865681));
#28014=CARTESIAN_POINT('',(-0.0150000000000006,-0.030178774389866,-0.0197758532865649));
#28015=CARTESIAN_POINT('',(-0.015,-0.0412787743898723,-0.0197758532865681));
#28016=CARTESIAN_POINT('',(-0.015,-0.0301787743898623,-0.0197758532865681));
#28017=CARTESIAN_POINT('Origin',(-0.015,-0.0365787743898723,-0.00417585328655812));
#28018=CARTESIAN_POINT('',(-0.0149999999999967,-0.0365787743898623,-0.00457585328656813));
#28019=CARTESIAN_POINT('',(-0.01479999999999,-0.0365787743898623,-0.00437585328656812));
#28020=CARTESIAN_POINT('',(-0.015,-0.0365787743898623,-0.0121758532865681));
#28021=CARTESIAN_POINT('Ctrl Pts',(-0.0118291591918131,-0.0365787743898723,
-0.0135653933579744));
#28022=CARTESIAN_POINT('Ctrl Pts',(-0.012060061067293,-0.0365787743898723,
-0.0136524861577944));
#28023=CARTESIAN_POINT('Ctrl Pts',(-0.0123125894300976,-0.0365787743898723,
-0.0136792436280273));
#28024=CARTESIAN_POINT('Ctrl Pts',(-0.0125574025636052,-0.0365787743898723,
-0.0136472777291935));
#28025=CARTESIAN_POINT('Ctrl Pts',(-0.0127250974036528,-0.0365787743898723,
-0.0136253813700599));
#28026=CARTESIAN_POINT('Ctrl Pts',(-0.0128891708546214,-0.0365787743898723,
-0.0135758966937495));
#28027=CARTESIAN_POINT('Ctrl Pts',(-0.0130392347235788,-0.0365787743898723,
-0.0134989032831501));
#28028=CARTESIAN_POINT('Ctrl Pts',(-0.0131082450132257,-0.0365787743898723,
-0.0134634961088363));
#28029=CARTESIAN_POINT('Ctrl Pts',(-0.0131753067095831,-0.0365787743898723,
-0.0134214203887249));
#28030=CARTESIAN_POINT('Ctrl Pts',(-0.0132355458760869,-0.0365787743898723,
-0.0133757167396176));
#28031=CARTESIAN_POINT('Ctrl Pts',(-0.0133533787985701,-0.0365787743898723,
-0.0132863165228648));
#28032=CARTESIAN_POINT('Ctrl Pts',(-0.0134424576307166,-0.0365787743898723,
-0.0131870659007685));
#28033=CARTESIAN_POINT('Ctrl Pts',(-0.0135097162431771,-0.0365787743898723,
-0.0130944668684115));
#28034=CARTESIAN_POINT('Ctrl Pts',(-0.0135610488334419,-0.0365787743898723,
-0.0130237941617795));
#28035=CARTESIAN_POINT('Ctrl Pts',(-0.0136022225954696,-0.0365787743898723,
-0.0129542292552571));
#28036=CARTESIAN_POINT('Ctrl Pts',(-0.0136385197303841,-0.0365787743898723,
-0.0128791079143929));
#28037=CARTESIAN_POINT('Ctrl Pts',(-0.0137280481667466,-0.0365787743898723,
-0.0126938179128299));
#28038=CARTESIAN_POINT('Ctrl Pts',(-0.0137761444620793,-0.0365787743898723,
-0.012487113971115));
#28039=CARTESIAN_POINT('Ctrl Pts',(-0.0137738110437006,-0.0365787743898723,
-0.0122905106090682));
#28040=CARTESIAN_POINT('Ctrl Pts',(-0.0137734593352465,-0.0365787743898723,
-0.0122608772329151));
#28041=CARTESIAN_POINT('Ctrl Pts',(-0.0137720035177717,-0.0365787743898723,
-0.0122313476771935));
#28042=CARTESIAN_POINT('Ctrl Pts',(-0.0137694124812826,-0.0365787743898723,
-0.0122019199453004));
#28043=CARTESIAN_POINT('Ctrl Pts',(-0.0137686492173546,-0.0365787743898723,
-0.0121932511649365));
#28044=CARTESIAN_POINT('Ctrl Pts',(-0.0137677873061495,-0.0365787743898723,
-0.012184591241161));
#28045=CARTESIAN_POINT('Ctrl Pts',(-0.0137668274805527,-0.0365787743898723,
-0.0121759402143804));
#28046=CARTESIAN_POINT('Ctrl Pts',(-0.0133941365248104,-0.0365787743898724,
-0.0112817167617477));
#28047=CARTESIAN_POINT('Ctrl Pts',(-0.0132597060893964,-0.0365787743898723,
-0.011114394916356));
#28048=CARTESIAN_POINT('Ctrl Pts',(-0.0130804465300667,-0.0365787743898723,
-0.0109853813929878));
#28049=CARTESIAN_POINT('Ctrl Pts',(-0.0128820499211865,-0.0365787743898723,
-0.0109023634156306));
#28050=CARTESIAN_POINT('Ctrl Pts',(-0.0127886426167731,-0.0365787743898723,
-0.0108632776392831));
#28051=CARTESIAN_POINT('Ctrl Pts',(-0.0126927759244174,-0.0365787743898723,
-0.0108346803378181));
#28052=CARTESIAN_POINT('Ctrl Pts',(-0.0125911049282069,-0.0365787743898723,
-0.0108163699769736));
#28053=CARTESIAN_POINT('Ctrl Pts',(-0.0124768272788988,-0.0365787743898723,
-0.0107957892305141));
#28054=CARTESIAN_POINT('Ctrl Pts',(-0.0123453825492587,-0.0365787743898723,
-0.0107866442237817));
#28055=CARTESIAN_POINT('Ctrl Pts',(-0.0122012816269697,-0.0365787743898723,
-0.0108034555473256));
#28056=CARTESIAN_POINT('Ctrl Pts',(-0.0120960331525637,-0.0365787743898723,
-0.0108157342068071));
#28057=CARTESIAN_POINT('Ctrl Pts',(-0.0119859286825378,-0.0365787743898723,
-0.0108427326623353));
#28058=CARTESIAN_POINT('Ctrl Pts',(-0.0118828353784451,-0.0365787743898723,
-0.0108814909939163));
#28059=CARTESIAN_POINT('Ctrl Pts',(-0.0117210892635519,-0.0365787743898723,
-0.0109423000795124));
#28060=CARTESIAN_POINT('Ctrl Pts',(-0.0115703802921963,-0.0365787743898723,
-0.0110322107690672));
#28061=CARTESIAN_POINT('Ctrl Pts',(-0.0114382293014629,-0.0365787743898723,
-0.0111440745982799));
#28062=CARTESIAN_POINT('Ctrl Pts',(-0.0113874539496207,-0.0365787743898723,
-0.011187055171147));
#28063=CARTESIAN_POINT('Ctrl Pts',(-0.0113394391814985,-0.0365787743898723,
-0.0112332851966829));
#28064=CARTESIAN_POINT('Ctrl Pts',(-0.0112946598499865,-0.0365787743898723,
-0.0112823688862808));
#28065=CARTESIAN_POINT('Ctrl Pts',(-0.0112586129422819,-0.0365787743898723,
-0.0113218807585887));
#28066=CARTESIAN_POINT('Ctrl Pts',(-0.0112180794482739,-0.0365787743898723,
-0.0113702875028219));
#28067=CARTESIAN_POINT('Ctrl Pts',(-0.0111761548550522,-0.0365787743898723,
-0.0114297153330889));
#28068=CARTESIAN_POINT('Ctrl Pts',(-0.0111346114653199,-0.0365787743898723,
-0.0114886028099613));
#28069=CARTESIAN_POINT('Ctrl Pts',(-0.0110920966712173,-0.0365787743898723,
-0.0115579296649615));
#28070=CARTESIAN_POINT('Ctrl Pts',(-0.0110538234060338,-0.0365787743898723,
-0.0116378502540936));
#28071=CARTESIAN_POINT('Ctrl Pts',(-0.0110495499905092,-0.0365787743898723,
-0.0116467738169172));
#28072=CARTESIAN_POINT('Ctrl Pts',(-0.0110453304317794,-0.0365787743898723,
-0.011655828468478));
#28073=CARTESIAN_POINT('Ctrl Pts',(-0.0110411708242858,-0.0365787743898723,
-0.0116650129552322));
#28074=CARTESIAN_POINT('Origin',(0.006,-0.0355287743898723,-0.0199758532865582));
#28075=CARTESIAN_POINT('',(0.00444999999999767,-0.0355287743898723,-0.0197758532865605));
#28076=CARTESIAN_POINT('Origin',(0.00600000000001,-0.0355287743898623,-0.0197758532865681));
#28077=CARTESIAN_POINT('',(0.00425,-0.0355287743898723,-0.0199758532865582));
#28078=CARTESIAN_POINT('Origin',(0.0078,-0.0412787743898723,-0.00437585328655813));
#28079=CARTESIAN_POINT('Ctrl Pts',(0.0076,-0.0344140995493819,-0.00417585328655812));
#28080=CARTESIAN_POINT('Ctrl Pts',(0.00783333333334,-0.0351572161097022,
-0.00440918661989812));
#28081=CARTESIAN_POINT('Ctrl Pts',(0.00783333333334,-0.0359003326700224,
-0.00440918661989812));
#28082=CARTESIAN_POINT('Ctrl Pts',(0.0076,-0.0366434492303427,-0.00417585328655813));
#28083=CARTESIAN_POINT('',(0.00760000000001,-0.0408787743898623,-0.00417585328655813));
#28084=CARTESIAN_POINT('',(0.00800000000000625,-0.030178774389861,-0.00457585328656312));
#28085=CARTESIAN_POINT('',(0.00800000000001,-0.0412787743898723,-0.00457585328656813));
#28086=CARTESIAN_POINT('',(0.00800000000001,-0.0301787743898623,-0.00457585328656812));
#28087=CARTESIAN_POINT('Origin',(-0.0148,-0.0412787743898723,-0.00437585328655813));
#28088=CARTESIAN_POINT('',(-0.015,-0.030178774389866,-0.00457585328656624));
#28089=CARTESIAN_POINT('',(-0.01459999999999,-0.0301787743898623,-0.00417585328655812));
#28090=CARTESIAN_POINT('',(-0.015,-0.0412787743898723,-0.00457585328656813));
#28091=CARTESIAN_POINT('Origin',(-0.00925,-0.0299787743898723,-0.00437585328655811));
#28092=CARTESIAN_POINT('',(0.0076000000000075,-0.0297787743898636,-0.00457585328656249));
#28093=CARTESIAN_POINT('',(0.00760000000001,-0.0301787743898623,-0.00417585328655812));
#28094=CARTESIAN_POINT('',(-0.0145999999999956,-0.0297787743898661,-0.00457585328656312));
#28095=CARTESIAN_POINT('',(-0.00924999999999,-0.0297787743898623,-0.00457585328656812));
#28096=CARTESIAN_POINT('',(-0.01459999999999,-0.0297787743898623,-0.00457585328656812));
#28097=CARTESIAN_POINT('Origin',(0.006,-0.0355287743898723,-0.00437585328655812));
#28098=CARTESIAN_POINT('',(0.00445000000000762,-0.0355287743898723,-0.00457585328656574));
#28099=CARTESIAN_POINT('Origin',(0.00600000000001,-0.0355287743898623,-0.00457585328656812));
#28100=CARTESIAN_POINT('',(0.00425,-0.0355287743898723,-0.00437585328655812));
#28101=CARTESIAN_POINT('Origin',(0.,-0.0412787743898723,-0.0121758532865581));
#28102=CARTESIAN_POINT('',(-0.00249999955320377,-0.0395787127102368,-0.0121769399287834));
#28103=CARTESIAN_POINT('',(-0.00249999997283516,-0.0385787905737985,-0.0121755877114987));
#28104=CARTESIAN_POINT('Ctrl Pts',(-0.00249999999999882,-0.0395786432478283,
-0.0121758508550077));
#28105=CARTESIAN_POINT('Ctrl Pts',(-0.00249999952765863,-0.0395477317163263,
-0.0116902140117491));
#28106=CARTESIAN_POINT('Ctrl Pts',(-0.00235420867782621,-0.0395168201848242,
-0.0112046011700908));
#28107=CARTESIAN_POINT('Ctrl Pts',(-0.00208694474875081,-0.0394859086533222,
-0.0107993862089782));
#28108=CARTESIAN_POINT('Ctrl Pts',(-0.00199401377133162,-0.0394751603310703,
-0.0106584879496008));
#28109=CARTESIAN_POINT('Ctrl Pts',(-0.00188684506187664,-0.0394644120088185,
-0.0105271641201691));
#28110=CARTESIAN_POINT('Ctrl Pts',(-0.00176776456039862,-0.0394536636865666,
-0.0104080839410272));
#28111=CARTESIAN_POINT('Ctrl Pts',(-0.00143160692048451,-0.0394233217699943,
-0.0100719272110501));
#28112=CARTESIAN_POINT('Ctrl Pts',(-0.000995195371062074,-0.0393929798534221,
-0.00983340281983273));
#28113=CARTESIAN_POINT('Ctrl Pts',(-0.000529040034186219,-0.0393626379368499,
-0.00973247107285754));
#28114=CARTESIAN_POINT('Ctrl Pts',(-0.000355157912828381,-0.0393513199996682,
-0.00969482219299269));
#28115=CARTESIAN_POINT('Ctrl Pts',(-0.000177402100138263,-0.0393400020624865,
-0.00967585297889307));
#28116=CARTESIAN_POINT('Ctrl Pts',(4.33564861886497E-9,-0.0393286841253049,
-0.00967585328656186));
#28117=CARTESIAN_POINT('Ctrl Pts',(0.000477367164465555,-0.0392982299735971,
-0.00967585411443285));
#28118=CARTESIAN_POINT('Ctrl Pts',(0.000956261322705523,-0.0392677758218892,
-0.00981689817770217));
#28119=CARTESIAN_POINT('Ctrl Pts',(0.00135812160581124,-0.0392373216701814,
-0.0100769236298453));
#28120=CARTESIAN_POINT('Ctrl Pts',(0.00150598737596406,-0.0392261159681353,
-0.0101726008225335));
#28121=CARTESIAN_POINT('Ctrl Pts',(0.00164356551969349,-0.0392149102660893,
-0.0102838843749181));
#28122=CARTESIAN_POINT('Ctrl Pts',(0.00176777069192936,-0.0392037045640432,
-0.0104080900725626));
#28123=CARTESIAN_POINT('Ctrl Pts',(0.00210526431200422,-0.0391732561303674,
-0.0107455851202919));
#28124=CARTESIAN_POINT('Ctrl Pts',(0.00234413374807478,-0.0391428076966918,
-0.0111838614835386));
#28125=CARTESIAN_POINT('Ctrl Pts',(0.00244445215636216,-0.039112359263016,
-0.0116517791932694));
#28126=CARTESIAN_POINT('Ctrl Pts',(0.00248139040510301,-0.0391011478429379,
-0.0118240712087365));
#28127=CARTESIAN_POINT('Ctrl Pts',(0.00250000043860317,-0.0390899364228596,
-0.0120001268556178));
#28128=CARTESIAN_POINT('Ctrl Pts',(0.00249999999999221,-0.0390787250027815,
-0.012175859526305));
#28129=CARTESIAN_POINT('Ctrl Pts',(0.00249999880879463,-0.0390482765691058,
-0.0126531215083521));
#28130=CARTESIAN_POINT('Ctrl Pts',(0.00235901179047531,-0.0390178281354301,
-0.0131319317915853));
#28131=CARTESIAN_POINT('Ctrl Pts',(0.00209907640032062,-0.0389873797017544,
-0.0135337480783653));
#28132=CARTESIAN_POINT('Ctrl Pts',(0.00200336557055327,-0.0389761682816762,
-0.0136817008838638));
#28133=CARTESIAN_POINT('Ctrl Pts',(0.0018920310394174,-0.0389649568615981,
-0.0138193568680316));
#28134=CARTESIAN_POINT('Ctrl Pts',(0.00176776186759135,-0.0389537454415199,
-0.0139436253248849));
#28135=CARTESIAN_POINT('Ctrl Pts',(0.00143020318323218,-0.038923291289812,
-0.0142811820671271));
#28136=CARTESIAN_POINT('Ctrl Pts',(0.00099183243510392,-0.0388928371381041,
-0.0145200730555509));
#28137=CARTESIAN_POINT('Ctrl Pts',(0.000523815083728861,-0.0388623829863963,
-0.0146203609584745));
#28138=CARTESIAN_POINT('Ctrl Pts',(0.000351606609750884,-0.0388511772843502,
-0.0146572622115374));
#28139=CARTESIAN_POINT('Ctrl Pts',(0.000175639028300414,-0.0388399715823042,
-0.0146758538587222));
#28140=CARTESIAN_POINT('Ctrl Pts',(-8.14384507266024E-9,-0.0388287658802581,
-0.0146758532865448));
#28141=CARTESIAN_POINT('Ctrl Pts',(-0.000475611709019986,-0.0387984239636858,
-0.0146758517372481));
#28142=CARTESIAN_POINT('Ctrl Pts',(-0.000952894728007072,-0.0387680820471136,
-0.014535808823928));
#28143=CARTESIAN_POINT('Ctrl Pts',(-0.00135378915737485,-0.0387377401305413,
-0.0142775799379984));
#28144=CARTESIAN_POINT('Ctrl Pts',(-0.0015033280949442,-0.0387264221933597,
-0.0141812571397182));
#28145=CARTESIAN_POINT('Ctrl Pts',(-0.00164238275388543,-0.038715104256178,
-0.0140690053510172));
#28146=CARTESIAN_POINT('Ctrl Pts',(-0.00176777338472311,-0.0387037863189964,
-0.0139436138077443));
#28147=CARTESIAN_POINT('Ctrl Pts',(-0.00211024007039254,-0.0386728747874944,
-0.0136011446300332));
#28148=CARTESIAN_POINT('Ctrl Pts',(-0.00235093239488195,-0.0386419632559923,
-0.0131553245197027));
#28149=CARTESIAN_POINT('Ctrl Pts',(-0.00244879874153802,-0.0386110517244903,
-0.0126792266305502));
#28150=CARTESIAN_POINT('Ctrl Pts',(-0.00248282808205786,-0.0386003034022384,
-0.0125136814994166));
#28151=CARTESIAN_POINT('Ctrl Pts',(-0.0025000006786659,-0.0385895550799866,
-0.0123447051822019));
#28152=CARTESIAN_POINT('Ctrl Pts',(-0.00249999999997981,-0.0385788067577347,
-0.0121758432386148));
#28153=CARTESIAN_POINT('',(-0.00249999979604092,-0.0375788205392406,-0.0121751469739251));
#28154=CARTESIAN_POINT('Ctrl Pts',(-0.0024999999456905,-0.0385787743898623,
-0.0121753321843825));
#28155=CARTESIAN_POINT('Ctrl Pts',(-0.00249989871899367,-0.0385478595459227,
-0.0116896947250819));
#28156=CARTESIAN_POINT('Ctrl Pts',(-0.00235400676731844,-0.0385169447019829,
-0.0112041116200849));
#28157=CARTESIAN_POINT('Ctrl Pts',(-0.00208665818069438,-0.0384860298580432,
-0.0107989518242373));
#28158=CARTESIAN_POINT('Ctrl Pts',(-0.00199371071341842,-0.0384752818810978,
-0.0106580923667716));
#28159=CARTESIAN_POINT('Ctrl Pts',(-0.0018865314487592,-0.0384645339041523,
-0.0105268076403119));
#28160=CARTESIAN_POINT('Ctrl Pts',(-0.0017674458724513,-0.0384537859272069,
-0.0104077653113841));
#28161=CARTESIAN_POINT('Ctrl Pts',(-0.00143122666542549,-0.0384234407217021,
-0.0100716682064659));
#28162=CARTESIAN_POINT('Ctrl Pts',(-0.000994770813954565,-0.0383930955161973,
-0.00983322226997918));
#28163=CARTESIAN_POINT('Ctrl Pts',(-0.000528596084364588,-0.0383627503106924,
-0.00973237499125969));
#28164=CARTESIAN_POINT('Ctrl Pts',(-0.000354730519714355,-0.0383514326953121,
-0.00969476276574625));
#28165=CARTESIAN_POINT('Ctrl Pts',(-0.00017699570173726,-0.0383401150799318,
-0.00967582585992544));
#28166=CARTESIAN_POINT('Ctrl Pts',(3.86968202952469E-7,-0.0383287974645515,
-0.00967585331650698));
#28167=CARTESIAN_POINT('Ctrl Pts',(0.000477751087115689,-0.0382983400162786,
-0.00967592720640196));
#28168=CARTESIAN_POINT('Ctrl Pts',(0.000956624670283315,-0.0382678825680056,
-0.00981704529372479));
#28169=CARTESIAN_POINT('Ctrl Pts',(0.00135844566361926,-0.0382374251197327,
-0.0100771333483591));
#28170=CARTESIAN_POINT('Ctrl Pts',(0.00150627662809758,-0.0382262197471205,
-0.0101728204045447));
#28171=CARTESIAN_POINT('Ctrl Pts',(0.00164382035946017,-0.0382150143745082,
-0.0102841079865441));
#28172=CARTESIAN_POINT('Ctrl Pts',(0.00176799314281305,-0.038203809001896,
-0.0104083125523836));
#28173=CARTESIAN_POINT('Ctrl Pts',(0.00210544517894053,-0.038173357274058,
-0.0107458509606174));
#28174=CARTESIAN_POINT('Ctrl Pts',(0.00234425965674057,-0.0381429055462199,
-0.0111841585824246));
#28175=CARTESIAN_POINT('Ctrl Pts',(0.00244451877559458,-0.0381124538183818,
-0.0116520900234653));
#28176=CARTESIAN_POINT('Ctrl Pts',(0.00248143012316302,-0.0381012427253347,
-0.0118243634311701));
#28177=CARTESIAN_POINT('Ctrl Pts',(0.00250001775731488,-0.0380900316322877,
-0.0120003971208957));
#28178=CARTESIAN_POINT('Ctrl Pts',(0.00249999998721497,-0.0380788205392406,
-0.0121761061207873));
#28179=CARTESIAN_POINT('Ctrl Pts',(0.00249995171982089,-0.0380483688114026,
-0.0126533693654073));
#28180=CARTESIAN_POINT('Ctrl Pts',(0.0023589167616459,-0.0380179170835647,
-0.0131321667312888));
#28181=CARTESIAN_POINT('Ctrl Pts',(0.00209894066755153,-0.0379874653557266,
-0.0135339578753503));
#28182=CARTESIAN_POINT('Ctrl Pts',(0.00200322799743868,-0.0379762542626795,
-0.0136818811040601));
#28183=CARTESIAN_POINT('Ctrl Pts',(0.00189189689820637,-0.0379650431696323,
-0.0138195087500959));
#28184=CARTESIAN_POINT('Ctrl Pts',(0.00176763559080942,-0.0379538320765852,
-0.0139437515919207));
#28185=CARTESIAN_POINT('Ctrl Pts',(0.00143005188452377,-0.0379233746283123,
-0.0142812851323386));
#28186=CARTESIAN_POINT('Ctrl Pts',(0.000991662842117688,-0.0378929171800394,
-0.0145201450129968));
#28187=CARTESIAN_POINT('Ctrl Pts',(0.000523637186059175,-0.0378624597317665,
-0.014620399072052));
#28188=CARTESIAN_POINT('Ctrl Pts',(0.000351449357938283,-0.0378512543591542,
-0.0146572827951248));
#28189=CARTESIAN_POINT('Ctrl Pts',(0.000175504773985148,-0.037840048986542,
-0.0146758616223606));
#28190=CARTESIAN_POINT('Ctrl Pts',(-1.18700254736605E-7,-0.0378288436139298,
-0.0146758532837401));
#28191=CARTESIAN_POINT('Ctrl Pts',(-0.00047572362672246,-0.037798498408425,
-0.0146758307019698));
#28192=CARTESIAN_POINT('Ctrl Pts',(-0.000953001524368115,-0.0377681532029201,
-0.0145357659183382));
#28193=CARTESIAN_POINT('Ctrl Pts',(-0.00135388507917457,-0.0377378079974153,
-0.0142775181486112));
#28194=CARTESIAN_POINT('Ctrl Pts',(-0.00150339950196762,-0.037726490382035,
-0.0141812014856665));
#28195=CARTESIAN_POINT('Ctrl Pts',(-0.00164243175618251,-0.0377151727666547,
-0.0140689606143419));
#28196=CARTESIAN_POINT('Ctrl Pts',(-0.0017678034628228,-0.0377038551512744,
-0.013943583728914));
#28197=CARTESIAN_POINT('Ctrl Pts',(-0.00211026489263892,-0.0376729403073345,
-0.0136011081528836));
#28198=CARTESIAN_POINT('Ctrl Pts',(-0.00235094972065609,-0.0376420254633948,
-0.0131552832078728));
#28199=CARTESIAN_POINT('Ctrl Pts',(-0.00244880770272406,-0.0376111106194549,
-0.0126791830344166));
#28200=CARTESIAN_POINT('Ctrl Pts',(-0.00248282939590269,-0.0376003626425096,
-0.0125136601646279));
#28201=CARTESIAN_POINT('Ctrl Pts',(-0.00249999895762901,-0.0375896146655642,
-0.0123447073642587));
#28202=CARTESIAN_POINT('Ctrl Pts',(-0.00249999999995236,-0.0375788666886189,
-0.0121758687202782));
#28203=CARTESIAN_POINT('',(-0.00249999943132573,-0.0365786614003052,-0.0121771638243569));
#28204=CARTESIAN_POINT('Ctrl Pts',(-0.00249999959212947,-0.0375787743898623,
-0.012174425227572));
#28205=CARTESIAN_POINT('Ctrl Pts',(-0.00249972218252544,-0.0375478504116054,
-0.0116887842955938));
#28206=CARTESIAN_POINT('Ctrl Pts',(-0.00235365206766289,-0.0375169264333485,
-0.0112032512070332));
#28207=CARTESIAN_POINT('Ctrl Pts',(-0.00208615315541311,-0.0374860024550917,
-0.0107981867767815));
#28208=CARTESIAN_POINT('Ctrl Pts',(-0.0019932266425179,-0.0374752597666819,
-0.010657471344765));
#28209=CARTESIAN_POINT('Ctrl Pts',(-0.00188609410542575,-0.0374645170782721,
-0.0105263208120313));
#28210=CARTESIAN_POINT('Ctrl Pts',(-0.0017670763035595,-0.0374537743898623,
-0.0104073959539095));
#28211=CARTESIAN_POINT('Ctrl Pts',(-0.00143078133828147,-0.0374234200061557,
-0.0100713636091205));
#28212=CARTESIAN_POINT('Ctrl Pts',(-0.000994268242573484,-0.0373930656224491,
-0.0098330076723254));
#28213=CARTESIAN_POINT('Ctrl Pts',(-0.000528065628921522,-0.0373627112387425,
-0.00973226029844577));
#28214=CARTESIAN_POINT('Ctrl Pts',(-0.00035432413796164,-0.0373513989557824,
-0.00969471439364909));
#28215=CARTESIAN_POINT('Ctrl Pts',(-0.000176723339944004,-0.0373400866728224,
-0.00967581611874746));
#28216=CARTESIAN_POINT('Ctrl Pts',(5.25011049869234E-7,-0.0373287743898623,
-0.00967585334168542));
#28217=CARTESIAN_POINT('Ctrl Pts',(0.000477896448403842,-0.0372983077550749,
-0.00967595359179943));
#28218=CARTESIAN_POINT('Ctrl Pts',(0.000956767990482746,-0.0372678411202875,
-0.00981710224408529));
#28219=CARTESIAN_POINT('Ctrl Pts',(0.0013585775187882,-0.0372373744855001,
-0.0100772187005848));
#28220=CARTESIAN_POINT('Ctrl Pts',(0.00150628925517822,-0.0372261744536208,
-0.0101728417526692));
#28221=CARTESIAN_POINT('Ctrl Pts',(0.00164372861443351,-0.0372149744217415,
-0.0102840407011479));
#28222=CARTESIAN_POINT('Ctrl Pts',(0.00176781891539311,-0.0372037743898623,
-0.0104081382975459));
#28223=CARTESIAN_POINT('Ctrl Pts',(0.00210530925518493,-0.0371733134873149,
-0.0107456484788562));
#28224=CARTESIAN_POINT('Ctrl Pts',(0.00234416805757305,-0.0371428525847675,
-0.0111839393494879));
#28225=CARTESIAN_POINT('Ctrl Pts',(0.00244447101894353,-0.0371123916822201,
-0.0116518671822145));
#28226=CARTESIAN_POINT('Ctrl Pts',(0.00248136983780919,-0.0371011859181008,
-0.0118240055129882));
#28227=CARTESIAN_POINT('Ctrl Pts',(0.00249997342184992,-0.0370899801539816,
-0.0119999000376457));
#28228=CARTESIAN_POINT('Ctrl Pts',(0.00249999997141761,-0.0370787743898623,
-0.0121754752496033));
#28229=CARTESIAN_POINT('Ctrl Pts',(0.00250007214175651,-0.0370483134873149,
-0.012652745640471));
#28230=CARTESIAN_POINT('Ctrl Pts',(0.00235915399073559,-0.0370178525847676,
-0.0131315841864723));
#28231=CARTESIAN_POINT('Ctrl Pts',(0.00209927324429766,-0.0369873916822203,
-0.0135334437423937));
#28232=CARTESIAN_POINT('Ctrl Pts',(0.00200366995942426,-0.036976185918101,
-0.0136812772934761));
#28233=CARTESIAN_POINT('Ctrl Pts',(0.00189246969922872,-0.0369649801539816,
-0.0138188349016734));
#28234=CARTESIAN_POINT('Ctrl Pts',(0.00176835344381461,-0.0369537743898623,
-0.013943033554032));
#28235=CARTESIAN_POINT('Ctrl Pts',(0.00143090170160338,-0.036923307755075,
-0.0142807093200213));
#28236=CARTESIAN_POINT('Ctrl Pts',(0.00099260274506201,-0.0368928411202877,
-0.014519748390164));
#28237=CARTESIAN_POINT('Ctrl Pts',(0.00052461138696062,-0.0368623744855004,
-0.0146201901890065));
#28238=CARTESIAN_POINT('Ctrl Pts',(0.000352570130465234,-0.036851174453621,
-0.0146571142325351));
#28239=CARTESIAN_POINT('Ctrl Pts',(0.000176770592362688,-0.0368399744217417,
-0.0146757630315266));
#28240=CARTESIAN_POINT('Ctrl Pts',(1.28108491020491E-6,-0.0368287743898624,
-0.0146758529583224));
#28241=CARTESIAN_POINT('Ctrl Pts',(-0.00047433147611545,-0.0367984200061557,
-0.0146760966783844));
#28242=CARTESIAN_POINT('Ctrl Pts',(-0.000951693785334355,-0.036768065622449,
-0.0145362948381555));
#28243=CARTESIAN_POINT('Ctrl Pts',(-0.0013527249599611,-0.0367377112387423,
-0.0142782650404013));
#28244=CARTESIAN_POINT('Ctrl Pts',(-0.00150217876429455,-0.0367263989557823,
-0.0141821040999417));
#28245=CARTESIAN_POINT('Ctrl Pts',(-0.00164117520491927,-0.0367150866728224,
-0.0140700374903543));
#28246=CARTESIAN_POINT('Ctrl Pts',(-0.00176654138897415,-0.0367037743898624,
-0.0139448449544416));
#28247=CARTESIAN_POINT('Ctrl Pts',(-0.00210925038622623,-0.0366728504116055,
-0.0136026106528273));
#28248=CARTESIAN_POINT('Ctrl Pts',(-0.00235025384378205,-0.0366419264333487,
-0.0131569534190921));
#28249=CARTESIAN_POINT('Ctrl Pts',(-0.0024484501037743,-0.0366110024550918,
-0.0126809197072669));
#28250=CARTESIAN_POINT('Ctrl Pts',(-0.00248256252667631,-0.036600259766682,
-0.0125155502390746));
#28251=CARTESIAN_POINT('Ctrl Pts',(-0.00249985165456606,-0.0365895170782721,
-0.0123467443051594));
#28252=CARTESIAN_POINT('Ctrl Pts',(-0.00249999904591269,-0.0365787743898623,
-0.0121780374192565));
#28253=CARTESIAN_POINT('',(-0.00250020961650365,-0.0355784048170972,-0.0121753040281057));
#28254=CARTESIAN_POINT('Ctrl Pts',(-0.00249999999990522,-0.0365784947127869,
-0.0121758750560007));
#28255=CARTESIAN_POINT('Ctrl Pts',(-0.00250000418566703,-0.0365458789096059,
-0.0116951827047534));
#28256=CARTESIAN_POINT('Ctrl Pts',(-0.00235822192526014,-0.0365179347736311,
-0.0112384571840363));
#28257=CARTESIAN_POINT('Ctrl Pts',(-0.00213008674960362,-0.0364908206152539,
-0.0108671400104112));
#28258=CARTESIAN_POINT('Ctrl Pts',(-0.00205373010295132,-0.036481745529816,
-0.0107428604724538));
#28259=CARTESIAN_POINT('Ctrl Pts',(-0.00196792392084753,-0.0364727634213843,
-0.01062757268742));
#28260=CARTESIAN_POINT('Ctrl Pts',(-0.00187459701875102,-0.0364637302489831,
-0.0105218018915616));
#28261=CARTESIAN_POINT('Ctrl Pts',(-0.0018621755065719,-0.0364625279626275,
-0.0105077241369224));
#28262=CARTESIAN_POINT('Ctrl Pts',(-0.0018496289474859,-0.036461326404273,
-0.0104938243014308));
#28263=CARTESIAN_POINT('Ctrl Pts',(-0.00183696178642117,-0.0364601257498979,
-0.0104801023038875));
#28264=CARTESIAN_POINT('Ctrl Pts',(-0.00150575505816513,-0.0364287323851718,
-0.0101213148938081));
#28265=CARTESIAN_POINT('Ctrl Pts',(-0.00109127169274443,-0.0363979570343344,
-0.00988588654905173));
#28266=CARTESIAN_POINT('Ctrl Pts',(-0.000677447847037822,-0.0363709454072252,
-0.00976939023582496));
#28267=CARTESIAN_POINT('Ctrl Pts',(-0.000632903748404836,-0.0363680378691636,
-0.00975685054455151));
#28268=CARTESIAN_POINT('Ctrl Pts',(-0.000588359671639667,-0.0363651739391918,
-0.00974564601115946));
#28269=CARTESIAN_POINT('Ctrl Pts',(-0.000543903940809233,-0.0363623575405296,
-0.00973573679278732));
#28270=CARTESIAN_POINT('Ctrl Pts',(-0.000213584020162325,-0.0363414308216289,
-0.00966210821520658));
#28271=CARTESIAN_POINT('Ctrl Pts',(0.000111819203387214,-0.0363215057164393,
-0.00966046320090738));
#28272=CARTESIAN_POINT('Ctrl Pts',(0.000407302089605617,-0.0363024018203738,
-0.00970925542557571));
#28273=CARTESIAN_POINT('Ctrl Pts',(0.000535161797734825,-0.0362941352889129,
-0.00973036852516975));
#28274=CARTESIAN_POINT('Ctrl Pts',(0.000657857796727303,-0.0362860225221071,
-0.00976084731948529));
#28275=CARTESIAN_POINT('Ctrl Pts',(0.000774427030647227,-0.0362780489031766,
-0.00979882514743081));
#28276=CARTESIAN_POINT('Ctrl Pts',(0.00116038694429653,-0.0362516483069783,
-0.00992456946865118));
#28277=CARTESIAN_POINT('Ctrl Pts',(0.00147418571268115,-0.0362274269837356,
-0.0101303574594857));
#28278=CARTESIAN_POINT('Ctrl Pts',(0.00171277270765056,-0.0362072415087562,
-0.0103547520669859));
#28279=CARTESIAN_POINT('Ctrl Pts',(0.00195135970261997,-0.0361870560337768,
-0.010579146674486));
#28280=CARTESIAN_POINT('Ctrl Pts',(0.0021156417199298,-0.0361696226856249,
-0.0108208939642838));
#28281=CARTESIAN_POINT('Ctrl Pts',(0.00222838256833176,-0.036153701563077,
-0.0110425787703198));
#28282=CARTESIAN_POINT('Ctrl Pts',(0.0022487466239749,-0.0361508257764383,
-0.0110826210601318));
#28283=CARTESIAN_POINT('Ctrl Pts',(0.00226743126048375,-0.0361480335409641,
-0.0111220294032082));
#28284=CARTESIAN_POINT('Ctrl Pts',(0.00228460794597736,-0.0361453234122333,
-0.0111606850575551));
#28285=CARTESIAN_POINT('Ctrl Pts',(0.00236252597684173,-0.0361330295448181,
-0.011336037425135));
#28286=CARTESIAN_POINT('Ctrl Pts',(0.0024096912660948,-0.0361224252468084,
-0.0114954903342938));
#28287=CARTESIAN_POINT('Ctrl Pts',(0.00244008456321309,-0.0361133756872451,
-0.0116318061154698));
#28288=CARTESIAN_POINT('Ctrl Pts',(0.00247717792833776,-0.0361023311922766,
-0.011798172108068));
#28289=CARTESIAN_POINT('Ctrl Pts',(0.00248947351924683,-0.0360934332308427,
-0.011929701616968));
#28290=CARTESIAN_POINT('Ctrl Pts',(0.00249509674334778,-0.0360874750694145,
-0.0120193533142409));
#28291=CARTESIAN_POINT('Ctrl Pts',(0.00249790835539826,-0.0360844959887004,
-0.0120641791628773));
#28292=CARTESIAN_POINT('Ctrl Pts',(0.00249896338344871,-0.0360822056816631,
-0.0120985365347907));
#28293=CARTESIAN_POINT('Ctrl Pts',(0.00249951757551438,-0.036080381945129,
-0.0121267422929342));
#28294=CARTESIAN_POINT('Ctrl Pts',(0.00249979467154721,-0.036079470076862,
-0.0121408451720059));
#28295=CARTESIAN_POINT('Ctrl Pts',(0.00249990418587905,-0.0360786573716534,
-0.0121534104681674));
#28296=CARTESIAN_POINT('Ctrl Pts',(0.00249993888064981,-0.0360783128037313,
-0.0121583720676249));
#28297=CARTESIAN_POINT('Ctrl Pts',(0.00249995622803519,-0.0360781405197703,
-0.0121608528673536));
#28298=CARTESIAN_POINT('Ctrl Pts',(0.00249995904440589,-0.0360780869820338,
-0.0121614328520031));
#28299=CARTESIAN_POINT('Ctrl Pts',(0.00249996804958266,-0.0360779674293166,
-0.0121632140197337));
#28300=CARTESIAN_POINT('Ctrl Pts',(0.00249997705475943,-0.0360778478765993,
-0.0121649951874644));
#28301=CARTESIAN_POINT('Ctrl Pts',(0.00249999820891719,-0.0360776647581573,
-0.0121679775971263));
#28302=CARTESIAN_POINT('Ctrl Pts',(0.00249999993021469,-0.0360772118286501,
-0.0121752625865014));
#28303=CARTESIAN_POINT('Ctrl Pts',(0.00250000337280969,-0.0360763059696357,
-0.0121898325652517));
#28304=CARTESIAN_POINT('Ctrl Pts',(0.00249978451240064,-0.0360742615648602,
-0.0122216107223804));
#28305=CARTESIAN_POINT('Ctrl Pts',(0.00249879466416602,-0.0360721820404578,
-0.0122534756179804));
#28306=CARTESIAN_POINT('Ctrl Pts',(0.0024978048159314,-0.0360701025160554,
-0.0122853405135803));
#28307=CARTESIAN_POINT('Ctrl Pts',(0.00249625951962489,-0.0360680761960123,
-0.0123173047059828));
#28308=CARTESIAN_POINT('Ctrl Pts',(0.00249367707095277,-0.0360658038812438,
-0.0123535459026242));
#28309=CARTESIAN_POINT('Ctrl Pts',(0.00248851217360852,-0.0360612592517069,
-0.0124260282959072));
#28310=CARTESIAN_POINT('Ctrl Pts',(0.00247902399267083,-0.0360556680737251,
-0.0125156086507209));
#28311=CARTESIAN_POINT('Ctrl Pts',(0.00246044666945603,-0.0360491838802819,
-0.0126188004467959));
#28312=CARTESIAN_POINT('Ctrl Pts',(0.00242329202302643,-0.0360362154933956,
-0.0128251840389459));
#28313=CARTESIAN_POINT('Ctrl Pts',(0.00235115394115315,-0.0360202690307048,
-0.0130862258480166));
#28314=CARTESIAN_POINT('Ctrl Pts',(0.00219473351942376,-0.0359993653520514,
-0.0133729935367869));
#28315=CARTESIAN_POINT('Ctrl Pts',(0.00216711349913969,-0.0359956742737252,
-0.0134236296960113));
#28316=CARTESIAN_POINT('Ctrl Pts',(0.00213682075988632,-0.0359918576501639,
-0.0134749978775204));
#28317=CARTESIAN_POINT('Ctrl Pts',(0.00210360074943439,-0.0359879202945817,
-0.0135267285165401));
#28318=CARTESIAN_POINT('Ctrl Pts',(0.00204275334083118,-0.0359807084400197,
-0.0136214809048422));
#28319=CARTESIAN_POINT('Ctrl Pts',(0.00197204693864971,-0.035973091536877,
-0.0137175048015559));
#28320=CARTESIAN_POINT('Ctrl Pts',(0.00189014621722043,-0.0359650991627008,
-0.0138121134362676));
#28321=CARTESIAN_POINT('Ctrl Pts',(0.00176353130196833,-0.035952743303542,
-0.0139583742268576));
#28322=CARTESIAN_POINT('Ctrl Pts',(0.00160994696874169,-0.0359387633021856,
-0.0141014178695565));
#28323=CARTESIAN_POINT('Ctrl Pts',(0.00142683534628718,-0.0359240898023569,
-0.014228690565688));
#28324=CARTESIAN_POINT('Ctrl Pts',(0.00133527953505993,-0.0359167530524426,
-0.0142923269137538));
#28325=CARTESIAN_POINT('Ctrl Pts',(0.00123634479103978,-0.0359093187201582,
-0.0143520079338338));
#28326=CARTESIAN_POINT('Ctrl Pts',(0.00113005941135025,-0.0359018750126493,
-0.0144058680234643));
#28327=CARTESIAN_POINT('Ctrl Pts',(0.00102377403166072,-0.0358944313051404,
-0.0144597281130948));
#28328=CARTESIAN_POINT('Ctrl Pts',(0.00091009824057508,-0.0358869588257101,
-0.0145077245907675));
#28329=CARTESIAN_POINT('Ctrl Pts',(0.000790462296476036,-0.0358793314169019,
-0.0145475972351853));
#28330=CARTESIAN_POINT('Ctrl Pts',(0.000670826352376991,-0.0358717040080937,
-0.0145874698796031));
#28331=CARTESIAN_POINT('Ctrl Pts',(0.000545326692536426,-0.0358638733479101,
-0.0146194111130419));
#28332=CARTESIAN_POINT('Ctrl Pts',(0.000411691870729785,-0.035855223196561,
-0.0146417222619043));
#28333=CARTESIAN_POINT('Ctrl Pts',(0.000350001179416516,-0.0358512299722691,
-0.0146520218992197));
#28334=CARTESIAN_POINT('Ctrl Pts',(0.000286547210286716,-0.0358471431795319,
-0.0146601474951376));
#28335=CARTESIAN_POINT('Ctrl Pts',(0.000224935218740908,-0.035843185019992,
-0.0146657135531935));
#28336=CARTESIAN_POINT('Ctrl Pts',(0.000183610600758106,-0.0358405301888983,
-0.0146694468398));
#28337=CARTESIAN_POINT('Ctrl Pts',(0.000144070717888571,-0.0358379940330427,
-0.0146721604783673));
#28338=CARTESIAN_POINT('Ctrl Pts',(9.60857070035578E-5,-0.0358349189925652,
-0.0146740061115289));
#28339=CARTESIAN_POINT('Ctrl Pts',(7.25285662780407E-5,-0.0358334093719581,
-0.0146749121828064));
#28340=CARTESIAN_POINT('Ctrl Pts',(4.77410863304185E-5,-0.0358318215863145,
-0.014675480515774));
#28341=CARTESIAN_POINT('Ctrl Pts',(2.73585790620338E-5,-0.0358305161258757,
-0.0146757035837062));
#28342=CARTESIAN_POINT('Ctrl Pts',(-1.52019121188965E-6,-0.0358286664961114,
-0.0146760196354797));
#28343=CARTESIAN_POINT('Ctrl Pts',(-1.68475855919575E-5,-0.0358276849859516,
-0.014675810629484));
#28344=CARTESIAN_POINT('Ctrl Pts',(-2.52470137588822E-5,-0.0358271470645206,
-0.0146757258009668));
#28345=CARTESIAN_POINT('Ctrl Pts',(-3.50302907154595E-5,-0.0358265205177801,
-0.0146756269965172));
#28346=CARTESIAN_POINT('Ctrl Pts',(-4.32145297488147E-5,-0.0358259963827926,
-0.0146755160720884));
#28347=CARTESIAN_POINT('Ctrl Pts',(-5.66846306278233E-5,-0.0358251336424485,
-0.0146752105744724));
#28348=CARTESIAN_POINT('Ctrl Pts',(-8.5164457235402E-5,-0.0358233095510309,
-0.0146745646610373));
#28349=CARTESIAN_POINT('Ctrl Pts',(-0.000113918265205585,-0.0358214675091151,
-0.0146734044237407));
#28350=CARTESIAN_POINT('Ctrl Pts',(-0.000141060502960187,-0.03581972767307,
-0.0146718705009428));
#28351=CARTESIAN_POINT('Ctrl Pts',(-0.000196336952449102,-0.0358161844147676,
-0.0146687465946965));
#28352=CARTESIAN_POINT('Ctrl Pts',(-0.000256766630260332,-0.0358123068140234,
-0.0146634154854298));
#28353=CARTESIAN_POINT('Ctrl Pts',(-0.000318665857405779,-0.0358083202692532,
-0.0146554605279017));
#28354=CARTESIAN_POINT('Ctrl Pts',(-0.000375972893758019,-0.0358046294789704,
-0.0146480957341674));
#28355=CARTESIAN_POINT('Ctrl Pts',(-0.000434357639183018,-0.0358008573708011,
-0.0146385946235638));
#28356=CARTESIAN_POINT('Ctrl Pts',(-0.000494476682713578,-0.0357969283946965,
-0.0146264639880471));
#28357=CARTESIAN_POINT('Ctrl Pts',(-0.000554595726244137,-0.0357929994185919,
-0.0146143333525305));
#28358=CARTESIAN_POINT('Ctrl Pts',(-0.000616439893323082,-0.0357886737530282,
-0.0145995489705675));
#28359=CARTESIAN_POINT('Ctrl Pts',(-0.00067953737948281,-0.0357842438436293,
-0.0145817271298603));
#28360=CARTESIAN_POINT('Ctrl Pts',(-0.000805732351802272,-0.0357753840248316,
-0.0145460834484459));
#28361=CARTESIAN_POINT('Ctrl Pts',(-0.000936956447855169,-0.035766127875995,
-0.0144983096416178));
#28362=CARTESIAN_POINT('Ctrl Pts',(-0.00107006174729965,-0.0357566455349307,
-0.0144352708789845));
#28363=CARTESIAN_POINT('Ctrl Pts',(-0.00120316704674414,-0.0357471631938664,
-0.0143722321163512));
#28364=CARTESIAN_POINT('Ctrl Pts',(-0.00133814273401691,-0.0357374711033914,
-0.0142939274948216));
#28365=CARTESIAN_POINT('Ctrl Pts',(-0.00147068513453818,-0.0357275803340383,
-0.0141975073704825));
#28366=CARTESIAN_POINT('Ctrl Pts',(-0.00168843994722776,-0.0357113307216925,
-0.0140390980913961));
#28367=CARTESIAN_POINT('Ctrl Pts',(-0.00189902193339737,-0.0356930246745004,
-0.013831540748202));
#28368=CARTESIAN_POINT('Ctrl Pts',(-0.00207353224951405,-0.0356730902563284,
-0.0135724434233646));
#28369=CARTESIAN_POINT('Ctrl Pts',(-0.00211146285195289,-0.0356687574208413,
-0.0135161274539705));
#28370=CARTESIAN_POINT('Ctrl Pts',(-0.00214768961790324,-0.035664347656259,
-0.0134573905581797));
#28371=CARTESIAN_POINT('Ctrl Pts',(-0.0021818901138409,-0.0356598653581442,
-0.0133962448348422));
#28372=CARTESIAN_POINT('Ctrl Pts',(-0.00235982569966132,-0.0356365452185082,
-0.0130781207900241));
#28373=CARTESIAN_POINT('Ctrl Pts',(-0.00248175197454682,-0.0356095958898492,
-0.0126936817681841));
#28374=CARTESIAN_POINT('Ctrl Pts',(-0.00249811171657688,-0.0355834167713905,
-0.0122730018918044));
#28375=CARTESIAN_POINT('Ctrl Pts',(-0.00249936339852753,-0.035581413810097,
-0.0122408157236303));
#28376=CARTESIAN_POINT('Ctrl Pts',(-0.0024999991528398,-0.0355794153574309,
-0.0122084456346896));
#28377=CARTESIAN_POINT('Ctrl Pts',(-0.00249999999915379,-0.0355774233837539,
-0.0121759183329917));
#28378=CARTESIAN_POINT('',(-0.00249999995263966,-0.0345787968006169,-0.0121755152554376));
#28379=CARTESIAN_POINT('Ctrl Pts',(-0.00249999969813745,-0.0355787743898623,
-0.0121746247456977));
#28380=CARTESIAN_POINT('Ctrl Pts',(-0.00249976104754906,-0.0355478566406557,
-0.0116889865238204));
#28381=CARTESIAN_POINT('Ctrl Pts',(-0.00235373123316885,-0.0355169388914492,
-0.0112034440484873));
#28382=CARTESIAN_POINT('Ctrl Pts',(-0.00208626723826142,-0.0354860211422426,
-0.0107983595440833));
#28383=CARTESIAN_POINT('Ctrl Pts',(-0.00199329640523685,-0.0354752740923454,
-0.0106575516426953));
#28384=CARTESIAN_POINT('Ctrl Pts',(-0.00188610159089402,-0.0354645270424482,
-0.0105263190663315));
#28385=CARTESIAN_POINT('Ctrl Pts',(-0.00176700773165438,-0.035453779992551,
-0.0104073274382105));
#28386=CARTESIAN_POINT('Ctrl Pts',(-0.0014307039947812,-0.0354234318867471,
-0.0100713123871473));
#28387=CARTESIAN_POINT('Ctrl Pts',(-0.000994187377721932,-0.0353930837809432,
-0.00983297432017851));
#28388=CARTESIAN_POINT('Ctrl Pts',(-0.00052798611458786,-0.0353627356751393,
-0.00973224311658367));
#28389=CARTESIAN_POINT('Ctrl Pts',(-0.000354141435614634,-0.0353514189818394,
-0.00969468083364645));
#28390=CARTESIAN_POINT('Ctrl Pts',(-0.000176433514161334,-0.0353401022885395,
-0.00967578830322123));
#28391=CARTESIAN_POINT('Ctrl Pts',(9.18400352385882E-7,-0.0353287855952396,
-0.00967585345524994));
#28392=CARTESIAN_POINT('Ctrl Pts',(0.000478284169225964,-0.035298325241806,
-0.00967602882041791));
#28393=CARTESIAN_POINT('Ctrl Pts',(0.000957129060230269,-0.0352678648883724,
-0.00981724964416271));
#28394=CARTESIAN_POINT('Ctrl Pts',(0.00135889541973528,-0.0352374045349388,
-0.0100774245319366));
#28395=CARTESIAN_POINT('Ctrl Pts',(0.00150667996061326,-0.0352262000892686,
-0.0101731264876329));
#28396=CARTESIAN_POINT('Ctrl Pts',(0.00164417755205256,-0.0352149956435984,
-0.0102844212731613));
#28397=CARTESIAN_POINT('Ctrl Pts',(0.00176830662644891,-0.0352037911979283,
-0.010408626171879));
#28398=CARTESIAN_POINT('Ctrl Pts',(0.00210569993998899,-0.0351733365677829,
-0.0107462255823322));
#28399=CARTESIAN_POINT('Ctrl Pts',(0.00234443692751372,-0.0351428819376375,
-0.0111845771105222));
#28400=CARTESIAN_POINT('Ctrl Pts',(0.00244461252497621,-0.0351124273074921,
-0.0116525277638388));
#28401=CARTESIAN_POINT('Ctrl Pts',(0.00248148656901149,-0.0351012171385337,
-0.0118247776274166));
#28402=CARTESIAN_POINT('Ctrl Pts',(0.00250004266924381,-0.0350900069695753,
-0.0120007831749893));
#28403=CARTESIAN_POINT('Ctrl Pts',(0.002499999926004,-0.0350787968006169,
-0.0121764615463884));
#28404=CARTESIAN_POINT('Ctrl Pts',(0.00249988380558114,-0.0350483421704715,
-0.0126537264159345));
#28405=CARTESIAN_POINT('Ctrl Pts',(0.00235877985707804,-0.0350178875403261,
-0.0131325050088043));
#28406=CARTESIAN_POINT('Ctrl Pts',(0.00209874525723065,-0.0349874329101807,
-0.0135342598329395));
#28407=CARTESIAN_POINT('Ctrl Pts',(0.00200302806134313,-0.0349762227412224,
-0.0136821434039069));
#28408=CARTESIAN_POINT('Ctrl Pts',(0.00189169940591702,-0.034965012572264,
-0.0138197327684265));
#28409=CARTESIAN_POINT('Ctrl Pts',(0.00176744647050627,-0.0349538024033056,
-0.0139439406638941));
#28410=CARTESIAN_POINT('Ctrl Pts',(0.00142982548175629,-0.034923342049872,
-0.0142814392697798));
#28411=CARTESIAN_POINT('Ctrl Pts',(0.000991409298149122,-0.0348928816964383,
-0.0145202525210834));
#28412=CARTESIAN_POINT('Ctrl Pts',(0.000523371442888126,-0.0348624213430047,
-0.0146204559808152));
#28413=CARTESIAN_POINT('Ctrl Pts',(0.00035120979242438,-0.0348512168973345,
-0.0146573145229517));
#28414=CARTESIAN_POINT('Ctrl Pts',(0.000175294693721739,-0.0348400124516644,
-0.0146758742078257));
#28415=CARTESIAN_POINT('Ctrl Pts',(-2.98119298794901E-7,-0.0348288080059942,
-0.0146758532687831));
#28416=CARTESIAN_POINT('Ctrl Pts',(-0.000475904804791021,-0.0347984599001903,
-0.01467579655377));
#28417=CARTESIAN_POINT('Ctrl Pts',(-0.000953174036178508,-0.0347681117943864,
-0.0145356965291672));
#28418=CARTESIAN_POINT('Ctrl Pts',(-0.00135403976161624,-0.0347377636885825,
-0.0142774184946738));
#28419=CARTESIAN_POINT('Ctrl Pts',(-0.00150352106692448,-0.0347264469952826,
-0.0141811075973368));
#28420=CARTESIAN_POINT('Ctrl Pts',(-0.00164252270203225,-0.0347151303019828,
-0.0140688788299219));
#28421=CARTESIAN_POINT('Ctrl Pts',(-0.00176786810101232,-0.0347038136086829,
-0.0139435190856907));
#28422=CARTESIAN_POINT('Ctrl Pts',(-0.00211031774660788,-0.0346728958594764,
-0.0136010302481805));
#28423=CARTESIAN_POINT('Ctrl Pts',(-0.0023509863876243,-0.03464197811027,
-0.0131551955459422));
#28424=CARTESIAN_POINT('Ctrl Pts',(-0.00244882661909244,-0.0346110603610635,
-0.0126790909934365));
#28425=CARTESIAN_POINT('Ctrl Pts',(-0.0024828360109965,-0.0346003133111662,
-0.0125135964308164));
#28426=CARTESIAN_POINT('Ctrl Pts',(-0.00249999918825629,-0.0345895662612688,
-0.0123446738066878));
#28427=CARTESIAN_POINT('Ctrl Pts',(-0.0024999999999711,-0.0345788192113715,
-0.0121758653077954));
#28428=CARTESIAN_POINT('',(-0.00249999974521768,-0.0335786873852289,-0.0121765002461478));
#28429=CARTESIAN_POINT('Ctrl Pts',(-0.00249999990530822,-0.0345787743898623,
-0.0121751652030797));
#28430=CARTESIAN_POINT('Ctrl Pts',(-0.00249986624097334,-0.0345478522652573,
-0.0116895252552616));
#28431=CARTESIAN_POINT('Ctrl Pts',(-0.00235394043889903,-0.0345169301406521,
-0.0112039498211489));
#28432=CARTESIAN_POINT('Ctrl Pts',(-0.00208656242431829,-0.0344860080160471,
-0.0107988067189276));
#28433=CARTESIAN_POINT('Ctrl Pts',(-0.00199365631386498,-0.0344752634739855,
-0.010658031233466));
#28434=CARTESIAN_POINT('Ctrl Pts',(-0.00188653476899345,-0.0344645189319239,
-0.010526820863554));
#28435=CARTESIAN_POINT('Ctrl Pts',(-0.00176751944018786,-0.0344537743898623,
-0.0104078388554637));
#28436=CARTESIAN_POINT('Ctrl Pts',(-0.00143131032715907,-0.0344234218882755,
-0.0100717238708825));
#28437=CARTESIAN_POINT('Ctrl Pts',(-0.000994859168403589,-0.0343930693866886,
-0.00983325890923276));
#28438=CARTESIAN_POINT('Ctrl Pts',(-0.00052868382947506,-0.0343627168851018,
-0.00973239397475206));
#28439=CARTESIAN_POINT('Ctrl Pts',(-0.000354912823296572,-0.034351402720022,
-0.00969479567280601));
#28440=CARTESIAN_POINT('Ctrl Pts',(-0.000177276052050649,-0.0343400885549421,
-0.00967585243990393));
#28441=CARTESIAN_POINT('Ctrl Pts',(1.19393685333613E-8,-0.0343287743898623,
-0.0096758532865866));
#28442=CARTESIAN_POINT('Ctrl Pts',(0.000477381226344273,-0.0342983096365892,
-0.00967585556638174));
#28443=CARTESIAN_POINT('Ctrl Pts',(0.000956280028606871,-0.034267844883316,
-0.00981690472123153));
#28444=CARTESIAN_POINT('Ctrl Pts',(0.00135814207659454,-0.0342373801300428,
-0.0100769368756966));
#28445=CARTESIAN_POINT('Ctrl Pts',(0.00150590706314561,-0.0342261782166493,
-0.0101725509004591));
#28446=CARTESIAN_POINT('Ctrl Pts',(0.00164339823397583,-0.0342149763032558,
-0.0102837500288529));
#28447=CARTESIAN_POINT('Ctrl Pts',(0.0017675363272879,-0.0342037743898623,
-0.0104078557379971));
#28448=CARTESIAN_POINT('Ctrl Pts',(0.00210507912693486,-0.0341733153655019,
-0.0107453104821375));
#28449=CARTESIAN_POINT('Ctrl Pts',(0.00234400765423946,-0.0341428563411416,
-0.0111835611625902));
#28450=CARTESIAN_POINT('Ctrl Pts',(0.00244438608379509,-0.0341123973167812,
-0.0116514711040338));
#28451=CARTESIAN_POINT('Ctrl Pts',(0.002481321132023,-0.0341011896744749,
-0.0118236423198025));
#28452=CARTESIAN_POINT('Ctrl Pts',(0.0024999532541214,-0.0340899820321686,
-0.0119995743940331));
#28453=CARTESIAN_POINT('Ctrl Pts',(0.00249999991176641,-0.0340787743898623,
-0.0121751890818159));
#28454=CARTESIAN_POINT('Ctrl Pts',(0.00250012671331015,-0.0340483153655019,
-0.0126524573517198));
#28455=CARTESIAN_POINT('Ctrl Pts',(0.00235926456083444,-0.0340178563411416,
-0.0131313103708889));
#28456=CARTESIAN_POINT('Ctrl Pts',(0.00209943160156203,-0.0339873973167811,
-0.0135331988396));
#28457=CARTESIAN_POINT('Ctrl Pts',(0.00200382398023952,-0.0339761896744748,
-0.0136810769249592));
#28458=CARTESIAN_POINT('Ctrl Pts',(0.00189261111142232,-0.0339649820321686,
-0.0138186762224371));
#28459=CARTESIAN_POINT('Ctrl Pts',(0.00176847552760974,-0.0339537743898624,
-0.013942911380749));
#28460=CARTESIAN_POINT('Ctrl Pts',(0.00143104863353808,-0.0339233096365892,
-0.0142806089394681));
#28461=CARTESIAN_POINT('Ctrl Pts',(0.000992768245731332,-0.033892844883316,
-0.0145196779453882));
#28462=CARTESIAN_POINT('Ctrl Pts',(0.000524785733290654,-0.0338623801300428,
-0.0146201527637365));
#28463=CARTESIAN_POINT('Ctrl Pts',(0.000352708200706007,-0.0338511782166493,
-0.014657097432327));
#28464=CARTESIAN_POINT('Ctrl Pts',(0.00017686938043608,-0.0338399763032558,
-0.0146757588191865));
#28465=CARTESIAN_POINT('Ctrl Pts',(1.34034880432785E-6,-0.0338287743898623,
-0.0146758529272511));
#28466=CARTESIAN_POINT('Ctrl Pts',(-0.000474269935258941,-0.0337984218882755,
-0.014676107920758));
#28467=CARTESIAN_POINT('Ctrl Pts',(-0.000951633769556664,-0.0337680693866886,
-0.0145363186693901));
#28468=CARTESIAN_POINT('Ctrl Pts',(-0.00135267015008844,-0.0337377168851017,
-0.0142783003049297));
#28469=CARTESIAN_POINT('Ctrl Pts',(-0.00150216002983868,-0.0337264027200219,
-0.0141821216634175));
#28470=CARTESIAN_POINT('Ctrl Pts',(-0.00164118823616503,-0.0337150885549422,
-0.0140700299046978));
#28471=CARTESIAN_POINT('Ctrl Pts',(-0.00176657973183811,-0.0337037743898624,
-0.0139448066638574));
#28472=CARTESIAN_POINT('Ctrl Pts',(-0.00210928035767172,-0.0336728522652572,
-0.0136025658860874));
#28473=CARTESIAN_POINT('Ctrl Pts',(-0.00235027400587087,-0.033641930140652,
-0.0131569046615656));
#28474=CARTESIAN_POINT('Ctrl Pts',(-0.00244846038690231,-0.0336110080160469,
-0.0126808698543756));
#28475=CARTESIAN_POINT('Ctrl Pts',(-0.00248257730850229,-0.0336002634739854,
-0.0125154615561457));
#28476=CARTESIAN_POINT('Ctrl Pts',(-0.00249986307686693,-0.0335895189319238,
-0.012346615537031));
#28477=CARTESIAN_POINT('Ctrl Pts',(-0.00249999918675125,-0.0335787743898623,
-0.0121778697793265));
#28478=CARTESIAN_POINT('',(-0.00249999968131482,-0.032578830244044,-0.0121749483697152));
#28479=CARTESIAN_POINT('Ctrl Pts',(-0.00249999999989964,-0.0335786477078032,
-0.0121758756868695));
#28480=CARTESIAN_POINT('Ctrl Pts',(-0.00250000435121429,-0.03354777589403,
-0.011690244642358));
#28481=CARTESIAN_POINT('Ctrl Pts',(-0.00235422169308874,-0.0335168994267022,
-0.0112046356695078));
#28482=CARTESIAN_POINT('Ctrl Pts',(-0.00199404053235062,-0.0334752737185985,
-0.0106585233900779));
#28483=CARTESIAN_POINT('Ctrl Pts',(-0.00188687582372486,-0.0334645330462428,
-0.0105271995947348));
#28484=CARTESIAN_POINT('Ctrl Pts',(-0.00143164247358771,-0.033423465707693,
-0.0100719494622799));
#28485=CARTESIAN_POINT('Ctrl Pts',(-0.000995226297729509,-0.0333931293360795,
-0.00983341399802515));
#28486=CARTESIAN_POINT('Ctrl Pts',(-0.00035519762743697,-0.033351483030854,
-0.00969482912049473));
#28487=CARTESIAN_POINT('Ctrl Pts',(-0.000177459478791954,-0.0333401702097692,
-0.00967585823750568));
#28488=CARTESIAN_POINT('Ctrl Pts',(0.000477316285896267,-0.0332984171435253,
-0.00967583996630468));
#28489=CARTESIAN_POINT('Ctrl Pts',(0.000956234436266438,-0.0332679844914464,
-0.00981688305921691));
#28490=CARTESIAN_POINT('Ctrl Pts',(0.00150595431923458,-0.0332262951843495,
-0.010172578594861));
#28491=CARTESIAN_POINT('Ctrl Pts',(0.00164351146432768,-0.0332150772452965,
-0.0102838401306641));
#28492=CARTESIAN_POINT('Ctrl Pts',(0.00210504588375627,-0.0331733547444291,
-0.0107453400500872));
#28493=CARTESIAN_POINT('Ctrl Pts',(0.00234387620624605,-0.0331427945138748,
-0.011183365842278));
#28494=CARTESIAN_POINT('Ctrl Pts',(0.00248132798507893,-0.0331011467372314,
-0.0118235205721592));
#28495=CARTESIAN_POINT('Ctrl Pts',(0.00249999175449094,-0.033089942642566,
-0.0119997927455534));
#28496=CARTESIAN_POINT('Ctrl Pts',(0.00250002238124961,-0.0330484181473094,
-0.0126535268110293));
#28497=CARTESIAN_POINT('Ctrl Pts',(0.0023587575513812,-0.0330182784947822,
-0.0131328112098241));
#28498=CARTESIAN_POINT('Ctrl Pts',(0.00200285349422997,-0.0329770278050595,
-0.0136823131940857));
#28499=CARTESIAN_POINT('Ctrl Pts',(0.001891864930695,-0.0329659560479124,
-0.0138194872129651));
#28500=CARTESIAN_POINT('Ctrl Pts',(0.00143078271491195,-0.0329246669105755,
-0.0142806997828226));
#28501=CARTESIAN_POINT('Ctrl Pts',(0.000992831074572435,-0.0328943299887714,
-0.0145195833260247));
#28502=CARTESIAN_POINT('Ctrl Pts',(0.000352619070780477,-0.0328527049860756,
-0.0146571464594452));
#28503=CARTESIAN_POINT('Ctrl Pts',(0.000176261132541491,-0.0328414755467602,
-0.0146758372723657));
#28504=CARTESIAN_POINT('Ctrl Pts',(-0.000475416776196498,-0.0327998829768102,
-0.0146758965187131));
#28505=CARTESIAN_POINT('Ctrl Pts',(-0.000952748003858568,-0.0327694838534468,
-0.0145358755492953));
#28506=CARTESIAN_POINT('Ctrl Pts',(-0.00150323296627836,-0.0327276627470969,
-0.0141813287735633));
#28507=CARTESIAN_POINT('Ctrl Pts',(-0.00164229600481632,-0.0327162930278274,
-0.0140690810302145));
#28508=CARTESIAN_POINT('Ctrl Pts',(-0.00211018950912318,-0.0326738348307577,
-0.0136012254148823));
#28509=CARTESIAN_POINT('Ctrl Pts',(-0.00235090480190234,-0.0326426854238918,
-0.0131553983571458));
#28510=CARTESIAN_POINT('Ctrl Pts',(-0.002482824807499,-0.0326006178733433,
-0.0125137184272263));
#28511=CARTESIAN_POINT('Ctrl Pts',(-0.00250000167733419,-0.0325897556944878,
-0.0123447162660254));
#28512=CARTESIAN_POINT('Ctrl Pts',(-0.00249999999987668,-0.0325788860982257,
-0.0121758284556141));
#28513=CARTESIAN_POINT('',(-0.00249999999999741,-0.0315787642283226,-0.0121758496907437));
#28514=CARTESIAN_POINT('Ctrl Pts',(-0.00249999936275296,-0.0325787743898623,
-0.0121740682838162));
#28515=CARTESIAN_POINT('Ctrl Pts',(-0.00249965261591296,-0.032547853826465,
-0.0116884293216484));
#28516=CARTESIAN_POINT('Ctrl Pts',(-0.00235351427316652,-0.0325169332630677,
-0.0112029186931701));
#28517=CARTESIAN_POINT('Ctrl Pts',(-0.00208595935539751,-0.0324860126996704,
-0.0107978933569413));
#28518=CARTESIAN_POINT('Ctrl Pts',(-0.00199297357310003,-0.032475266596401,
-0.0106571312358277));
#28519=CARTESIAN_POINT('Ctrl Pts',(-0.00188577101279796,-0.0324645204931317,
-0.0105259441942091));
#28520=CARTESIAN_POINT('Ctrl Pts',(-0.00176667590864148,-0.0324537743898623,
-0.0104069959622309));
#28521=CARTESIAN_POINT('Ctrl Pts',(-0.0014303078820767,-0.0324234234734616,
-0.0100710427562847));
#28522=CARTESIAN_POINT('Ctrl Pts',(-0.000993744870917422,-0.032393072557061,
-0.00983278630991865));
#28523=CARTESIAN_POINT('Ctrl Pts',(-0.000527523167523132,-0.0323627216406603,
-0.00973214313440699));
#28524=CARTESIAN_POINT('Ctrl Pts',(-0.000353701451745077,-0.0323514058903943,
-0.00969462027924725));
#28525=CARTESIAN_POINT('Ctrl Pts',(-0.000176021369284442,-0.0323400901401283,
-0.00967576141850525));
#28526=CARTESIAN_POINT('Ctrl Pts',(1.29998489136426E-6,-0.0323287743898623,
-0.00967585362455026));
#28527=CARTESIAN_POINT('Ctrl Pts',(0.000478667387052929,-0.032298311221266,
-0.00967610185274799));
#28528=CARTESIAN_POINT('Ctrl Pts',(0.000957492025298925,-0.0322678480526696,
-0.00981739670095818));
#28529=CARTESIAN_POINT('Ctrl Pts',(0.00135921932706133,-0.0322373848840733,
-0.0100776343225453));
#28530=CARTESIAN_POINT('Ctrl Pts',(0.00150696334902196,-0.032226181386003,
-0.0101733424128595));
#28531=CARTESIAN_POINT('Ctrl Pts',(0.0016444216184737,-0.0322149778879326,
-0.0102846362907292));
#28532=CARTESIAN_POINT('Ctrl Pts',(0.00176851454323397,-0.0322037743898623,
-0.0104088342401497));
#28533=CARTESIAN_POINT('Ctrl Pts',(0.00210586927790242,-0.0321733169473757,
-0.0107464744912283));
#28534=CARTESIAN_POINT('Ctrl Pts',(0.00234455494301116,-0.0321428595048892,
-0.0111848556501687));
#28535=CARTESIAN_POINT('Ctrl Pts',(0.0024446749625898,-0.0321124020624027,
-0.011652819513952));
#28536=CARTESIAN_POINT('Ctrl Pts',(0.00248152204011029,-0.0321011928382226,
-0.0118250438187232));
#28537=CARTESIAN_POINT('Ctrl Pts',(0.00250005712607798,-0.0320899836140425,
-0.012001020313999));
#28538=CARTESIAN_POINT('Ctrl Pts',(0.00249999986716576,-0.0320787743898623,
-0.01217666825355));
#28539=CARTESIAN_POINT('Ctrl Pts',(0.00249984428458505,-0.0320483169473756,
-0.0126539347379028));
#28540=CARTESIAN_POINT('Ctrl Pts',(0.00235869983460178,-0.0320178595048889,
-0.0131327029367118));
#28541=CARTESIAN_POINT('Ctrl Pts',(0.00209863064063772,-0.0319874020624023,
-0.0135344368998026));
#28542=CARTESIAN_POINT('Ctrl Pts',(0.00200291761749952,-0.0319761928382223,
-0.0136822866759281));
#28543=CARTESIAN_POINT('Ctrl Pts',(0.00189159945511839,-0.0319649836140423,
-0.0138198445281878));
#28544=CARTESIAN_POINT('Ctrl Pts',(0.00176736211766683,-0.0319537743898623,
-0.0139440249821341));
#28545=CARTESIAN_POINT('Ctrl Pts',(0.00142972385689433,-0.031923311221266,
-0.0142815086513147));
#28546=CARTESIAN_POINT('Ctrl Pts',(0.000991294697778186,-0.0318928480526697,
-0.0145203012508883));
#28547=CARTESIAN_POINT('Ctrl Pts',(0.00052325059434184,-0.0318623848840733,
-0.0146204818504755));
#28548=CARTESIAN_POINT('Ctrl Pts',(0.000351117114756464,-0.031851181386003,
-0.0146573254621507));
#28549=CARTESIAN_POINT('Ctrl Pts',(0.000175232400223226,-0.0318399778879326,
-0.014675876435438));
#28550=CARTESIAN_POINT('Ctrl Pts',(-3.2994906170825E-7,-0.0318287743898623,
-0.0146758532647848));
#28551=CARTESIAN_POINT('Ctrl Pts',(-0.000475938384284838,-0.0317984234734617,
-0.0146757904941615));
#28552=CARTESIAN_POINT('Ctrl Pts',(-0.000953207210028182,-0.0317680725570609,
-0.0145356834111494));
#28553=CARTESIAN_POINT('Ctrl Pts',(-0.00135407034799732,-0.0317377216406602,
-0.0142773987875346));
#28554=CARTESIAN_POINT('Ctrl Pts',(-0.00150352439084073,-0.0317264058903942,
-0.0141811023772458));
#28555=CARTESIAN_POINT('Ctrl Pts',(-0.00164250217809006,-0.0317150901401283,
-0.0140688937794005));
#28556=CARTESIAN_POINT('Ctrl Pts',(-0.00176782878136625,-0.0317037743898623,
-0.013943558408962));
#28557=CARTESIAN_POINT('Ctrl Pts',(-0.00211028677936814,-0.031672853826465,
-0.0136010764544755));
#28558=CARTESIAN_POINT('Ctrl Pts',(-0.002350965451897,-0.0316419332630677,
-0.0131552461552842));
#28559=CARTESIAN_POINT('Ctrl Pts',(-0.00244881593451928,-0.0316110126996704,
-0.0126791429832979));
#28560=CARTESIAN_POINT('Ctrl Pts',(-0.00248282279842098,-0.0316002665964011,
-0.0125136785385756));
#28561=CARTESIAN_POINT('Ctrl Pts',(-0.00249998952627055,-0.0315895204931317,
-0.0123447869023314));
#28562=CARTESIAN_POINT('Ctrl Pts',(-0.00249999999519073,-0.0315787743898623,
-0.012176008355439));
#28563=CARTESIAN_POINT('',(-0.00249999796170874,-0.0305787743898623,-0.0121790456919423));
#28564=CARTESIAN_POINT('Ctrl Pts',(-0.00249999999999741,-0.0315787642283226,
-0.0121758496907437));
#28565=CARTESIAN_POINT('Ctrl Pts',(-0.00249999930148813,-0.0315478414143166,
-0.0116902091587184));
#28566=CARTESIAN_POINT('Ctrl Pts',(-0.00235420613190631,-0.0315169186003106,
-0.0112045933187037));
#28567=CARTESIAN_POINT('Ctrl Pts',(-0.00208693851711527,-0.0314859957863047,
-0.0107993767608662));
#28568=CARTESIAN_POINT('Ctrl Pts',(-0.00199408245578486,-0.0314752523570415,
-0.0106585934730142));
#28569=CARTESIAN_POINT('Ctrl Pts',(-0.00188701190510759,-0.0314645089277783,
-0.0105273690150605));
#28570=CARTESIAN_POINT('Ctrl Pts',(-0.00176804687751574,-0.0314537654985151,
-0.010408366302474));
#28571=CARTESIAN_POINT('Ctrl Pts',(-0.00143193718319067,-0.0314234122863254,
-0.0100721501374298));
#28572=CARTESIAN_POINT('Ctrl Pts',(-0.000995556008603784,-0.0313930590741356,
-0.00983355476771765));
#28573=CARTESIAN_POINT('Ctrl Pts',(-0.000529409695698544,-0.0313627058619459,
-0.00973255114107948));
#28574=CARTESIAN_POINT('Ctrl Pts',(-0.000355670992443751,-0.0313513928308664,
-0.00969490579533647));
#28575=CARTESIAN_POINT('Ctrl Pts',(-0.000178061926068187,-0.031340079799787,
-0.00967590981254358));
#28576=CARTESIAN_POINT('Ctrl Pts',(-7.95404688749067E-7,-0.0313287667687076,
-0.00967585341309182));
#28577=CARTESIAN_POINT('Ctrl Pts',(0.000476575028159227,-0.0312983013062999,
-0.00967570153201191));
#28578=CARTESIAN_POINT('Ctrl Pts',(0.000955520274846601,-0.0312678358438924,
-0.00981659668333524));
#28579=CARTESIAN_POINT('Ctrl Pts',(0.00135746673941968,-0.0312373703814847,
-0.010076500040587));
#28580=CARTESIAN_POINT('Ctrl Pts',(0.00150524438374116,-0.0312261696006231,
-0.0101720548203179));
#28581=CARTESIAN_POINT('Ctrl Pts',(0.00164275575461887,-0.0312149688197616,
-0.010283194175715));
#28582=CARTESIAN_POINT('Ctrl Pts',(0.00176692182567706,-0.0312037680389,
-0.0104072416101446));
#28583=CARTESIAN_POINT('Ctrl Pts',(0.00210458267841763,-0.0311733083071484,
-0.0107445798389603));
#28584=CARTESIAN_POINT('Ctrl Pts',(0.002343663667394,-0.031142848575397,
-0.0111827485478995));
#28585=CARTESIAN_POINT('Ctrl Pts',(0.00244420433014957,-0.0311123888436454,
-0.0116506245816322));
#28586=CARTESIAN_POINT('Ctrl Pts',(0.0024811944817488,-0.0311011823321278,
-0.0118227619531502));
#28587=CARTESIAN_POINT('Ctrl Pts',(0.0024998875048212,-0.0310899758206101,
-0.0119986655995088));
#28588=CARTESIAN_POINT('Ctrl Pts',(0.00249999949157442,-0.0310787693090925,
-0.0121742588814475));
#28589=CARTESIAN_POINT('Ctrl Pts',(0.0025003038759011,-0.031048309577341,
-0.0126515282133713));
#28590=CARTESIAN_POINT('Ctrl Pts',(0.00235961926287144,-0.0310178498455895,
-0.0131304345073108));
#28591=CARTESIAN_POINT('Ctrl Pts',(0.00209993488958646,-0.0309873901138379,
-0.0135324200779464));
#28592=CARTESIAN_POINT('Ctrl Pts',(0.00200439380130905,-0.0309761836023203,
-0.0136803155342825));
#28593=CARTESIAN_POINT('Ctrl Pts',(0.00189324748533952,-0.0309649770908026,
-0.0138179405156711));
#28594=CARTESIAN_POINT('Ctrl Pts',(0.00176917629465765,-0.0309537705792849,
-0.0139422097733471));
#28595=CARTESIAN_POINT('Ctrl Pts',(0.00143188255345838,-0.0309233051168773,
-0.0142800419695822));
#28596=CARTESIAN_POINT('Ctrl Pts',(0.000993695915477766,-0.0308928396544697,
-0.0145192849880158));
#28597=CARTESIAN_POINT('Ctrl Pts',(0.00052575226151233,-0.0308623741920621,
-0.0146199450523301));
#28598=CARTESIAN_POINT('Ctrl Pts',(0.000353710417751829,-0.0308511734112005,
-0.0146569532325051));
#28599=CARTESIAN_POINT('Ctrl Pts',(0.000177900980369277,-0.0308399726303389,
-0.014675684116494));
#28600=CARTESIAN_POINT('Ctrl Pts',(2.39340536966486E-6,-0.0308287718494774,
-0.01467585214088));
#28601=CARTESIAN_POINT('Ctrl Pts',(-0.000473217958759423,-0.0307984186372876,
-0.0146763074734057));
#28602=CARTESIAN_POINT('Ctrl Pts',(-0.000950641601993971,-0.0307680654250979,
-0.0145367186222503));
#28603=CARTESIAN_POINT('Ctrl Pts',(-0.00135178712369863,-0.0307377122129081,
-0.0142788681633962));
#28604=CARTESIAN_POINT('Ctrl Pts',(-0.00150129919925867,-0.0307263991818287,
-0.0141827639937085));
#28605=CARTESIAN_POINT('Ctrl Pts',(-0.00164035884141642,-0.0307150861507493,
-0.0140707462013264));
#28606=CARTESIAN_POINT('Ctrl Pts',(-0.00176579096747762,-0.0307037731196699,
-0.0139455940187487));
#28607=CARTESIAN_POINT('Ctrl Pts',(-0.00210864464456624,-0.0306728503056636,
-0.0136035055336064));
#28608=CARTESIAN_POINT('Ctrl Pts',(-0.00234983702321265,-0.0306419274916575,
-0.0131579511193642));
#28609=CARTESIAN_POINT('Ctrl Pts',(-0.00244823537039844,-0.0306110046776513,
-0.0126819595709787));
#28610=CARTESIAN_POINT('Ctrl Pts',(-0.00248242164084506,-0.0306002612483883,
-0.0125165871204365));
#28611=CARTESIAN_POINT('Ctrl Pts',(-0.00249978250656215,-0.0305895178191253,
-0.0123477703250945));
#28612=CARTESIAN_POINT('Ctrl Pts',(-0.00249999796170874,-0.0305787743898623,
-0.0121790456919423));
#28613=CARTESIAN_POINT('',(-0.0020225424859345,-0.0304787743898643,-0.0107063901558304));
#28614=CARTESIAN_POINT('Ctrl Pts',(-0.00249999827498751,-0.0305768133462266,
-0.0121787901317142));
#28615=CARTESIAN_POINT('Ctrl Pts',(-0.00250007190193453,-0.0305725335791676,
-0.0121161149715434));
#28616=CARTESIAN_POINT('Ctrl Pts',(-0.002497788617112,-0.0305683056341438,
-0.0120534556549794));
#28617=CARTESIAN_POINT('Ctrl Pts',(-0.0024931523602667,-0.0305641400813256,
-0.0119909443670962));
#28618=CARTESIAN_POINT('Ctrl Pts',(-0.00249014764196586,-0.030561440422268,
-0.0119504313375166));
#28619=CARTESIAN_POINT('Ctrl Pts',(-0.00248615576125712,-0.0305587677962322,
-0.0119099958863706));
#28620=CARTESIAN_POINT('Ctrl Pts',(-0.00248117998961982,-0.0305561228206165,
-0.0118696738308296));
#28621=CARTESIAN_POINT('Ctrl Pts',(-0.00247831465547303,-0.0305545996922453,
-0.0118464540830132));
#28622=CARTESIAN_POINT('Ctrl Pts',(-0.00247512344458627,-0.0305530859103769,
-0.0118232751292318));
#28623=CARTESIAN_POINT('Ctrl Pts',(-0.0024716072436851,-0.0305515813272362,
-0.0118001437804721));
#28624=CARTESIAN_POINT('Ctrl Pts',(-0.00246856976557504,-0.0305502815896833,
-0.0117801617124708));
#28625=CARTESIAN_POINT('Ctrl Pts',(-0.00246529001379808,-0.0305489888193277,
-0.0117602167955565));
#28626=CARTESIAN_POINT('Ctrl Pts',(-0.00246176867545611,-0.0305477028057356,
-0.0117403134048675));
#28627=CARTESIAN_POINT('Ctrl Pts',(-0.00245794692801323,-0.0305463070809629,
-0.0117187120348532));
#28628=CARTESIAN_POINT('Ctrl Pts',(-0.00245384094344368,-0.0305449194362869,
-0.0116971614306637));
#28629=CARTESIAN_POINT('Ctrl Pts',(-0.00244945174311329,-0.0305435394624721,
-0.0116756671630408));
#28630=CARTESIAN_POINT('Ctrl Pts',(-0.00244368591563245,-0.030541726674186,
-0.0116474314413576));
#28631=CARTESIAN_POINT('Ctrl Pts',(-0.00243743214261921,-0.0305399273839073,
-0.0116192967816556));
#28632=CARTESIAN_POINT('Ctrl Pts',(-0.00243069313014558,-0.0305381402891356,
-0.0115912757407499));
#28633=CARTESIAN_POINT('Ctrl Pts',(-0.00241542092603212,-0.0305340903075945,
-0.0115277734015189));
#28634=CARTESIAN_POINT('Ctrl Pts',(-0.00239766542416501,-0.0305301059677435,
-0.0114648911574963));
#28635=CARTESIAN_POINT('Ctrl Pts',(-0.00237746654675865,-0.0305261643904438,
-0.0114027732007691));
#28636=CARTESIAN_POINT('Ctrl Pts',(-0.00234285388810228,-0.0305194101304471,
-0.0112963282934916));
#28637=CARTESIAN_POINT('Ctrl Pts',(-0.00230113128439389,-0.0305127976518697,
-0.0111923267536372));
#28638=CARTESIAN_POINT('Ctrl Pts',(-0.0022525787066754,-0.0305061482064187,
-0.0110914690510435));
#28639=CARTESIAN_POINT('Ctrl Pts',(-0.0022055666684243,-0.0304997097432396,
-0.0109938114930916));
#28640=CARTESIAN_POINT('Ctrl Pts',(-0.00215225704739796,-0.0304932486502635,
-0.0108993215649116));
#28641=CARTESIAN_POINT('Ctrl Pts',(-0.00209299025559816,-0.03048655461756,
-0.0108085962551367));
#28642=CARTESIAN_POINT('Ctrl Pts',(-0.0020793513660387,-0.0304850141398324,
-0.0107877179109124));
#28643=CARTESIAN_POINT('Ctrl Pts',(-0.00206540128873714,-0.0304834616888587,
-0.0107670455075156));
#28644=CARTESIAN_POINT('Ctrl Pts',(-0.00205114477230131,-0.0304818945665418,
-0.0107465859487024));
#28645=CARTESIAN_POINT('Ctrl Pts',(-0.00204615281254276,-0.0304813458342075,
-0.0107394219760214));
#28646=CARTESIAN_POINT('Ctrl Pts',(-0.00204112342134774,-0.0304807953183517,
-0.0107322843006978));
#28647=CARTESIAN_POINT('Ctrl Pts',(-0.0020360568086995,-0.0304802429033023,
-0.0107251732144028));
#28648=CARTESIAN_POINT('Ctrl Pts',(-0.00203158097889193,-0.030479754901571,
-0.0107188913029537));
#28649=CARTESIAN_POINT('Ctrl Pts',(-0.00202707615544529,-0.0304792654235685,
-0.010712630216571));
#28650=CARTESIAN_POINT('Ctrl Pts',(-0.0020225424859383,-0.0304787743898724,
-0.0107063901558282));
#28651=CARTESIAN_POINT('',(-0.000393037172625865,-0.0304787744837451,-0.0097069422349132));
#28652=CARTESIAN_POINT('Origin',(1.00024155624823E-14,-0.0304787743898623,
-0.0121758532865681));
#28653=CARTESIAN_POINT('',(-0.00249999960057212,-0.0307038306106531,-0.012174809678307));
#28654=CARTESIAN_POINT('Ctrl Pts',(-0.000393037172625865,-0.0304787744837451,
-0.0097069422349132));
#28655=CARTESIAN_POINT('Ctrl Pts',(-0.000873042018136126,-0.0305097515278591,
-0.00978335638810855));
#28656=CARTESIAN_POINT('Ctrl Pts',(-0.00132989543511568,-0.0305407285719731,
-0.0100039314220522));
#28657=CARTESIAN_POINT('Ctrl Pts',(-0.00168811523538598,-0.0305717056160869,
-0.0103318720089802));
#28658=CARTESIAN_POINT('Ctrl Pts',(-0.00176354660113698,-0.0305782285406787,
-0.0104009273943567));
#28659=CARTESIAN_POINT('Ctrl Pts',(-0.00183469500662704,-0.0305847514652705,
-0.0104745810657172));
#28660=CARTESIAN_POINT('Ctrl Pts',(-0.00190103004203007,-0.0305912743898623,
-0.0105522508785471));
#28661=CARTESIAN_POINT('Ctrl Pts',(-0.00221605182441028,-0.030622251434176,
-0.0109211009549228));
#28662=CARTESIAN_POINT('Ctrl Pts',(-0.00242095374775302,-0.0306532284784897,
-0.0113849850894544));
#28663=CARTESIAN_POINT('Ctrl Pts',(-0.00248092016327206,-0.0306842055228035,
-0.0118675755814445));
#28664=CARTESIAN_POINT('Ctrl Pts',(-0.00249354752265257,-0.0306907284784897,
-0.0119691965224867));
#28665=CARTESIAN_POINT('Ctrl Pts',(-0.00249992035016284,-0.030697251434176,
-0.0120715766804667));
#28666=CARTESIAN_POINT('Ctrl Pts',(-0.00249999925703147,-0.0307037743898623,
-0.0121739258939954));
#28667=CARTESIAN_POINT('',(-0.00249999980101701,-0.0317037304164077,-0.0121765701516269));
#28668=CARTESIAN_POINT('Ctrl Pts',(-0.00249999999994761,-0.0307038959688732,
-0.0121758371019472));
#28669=CARTESIAN_POINT('Ctrl Pts',(-0.00250000314392324,-0.0307348003099762,
-0.012661479860859));
#28670=CARTESIAN_POINT('Ctrl Pts',(-0.00235421249077242,-0.0307657055154774,
-0.0131470991042038));
#28671=CARTESIAN_POINT('Ctrl Pts',(-0.00208694555713805,-0.0307966129601098,
-0.0135523191384926));
#28672=CARTESIAN_POINT('Ctrl Pts',(-0.00199403940976012,-0.0308073568690814,
-0.0136931799315364));
#28673=CARTESIAN_POINT('Ctrl Pts',(-0.00188690309448439,-0.030818101048622,
-0.0138244714868721));
#28674=CARTESIAN_POINT('Ctrl Pts',(-0.00176786054562226,-0.0308288455564767,
-0.0139435266419131));
#28675=CARTESIAN_POINT('Ctrl Pts',(-0.00143172188960472,-0.0308591846618166,
-0.0142797008938085));
#28676=CARTESIAN_POINT('Ctrl Pts',(-0.000995324916698483,-0.03088952638487,
-0.014518248219889));
#28677=CARTESIAN_POINT('Ctrl Pts',(-0.000529177622831193,-0.0309198668254454,
-0.0146192057055707));
#28678=CARTESIAN_POINT('Ctrl Pts',(-0.000355334125541598,-0.0309311818933828,
-0.014656856470939));
#28679=CARTESIAN_POINT('Ctrl Pts',(-0.000177617629157195,-0.0309424967829508,
-0.0146758356407072));
#28680=CARTESIAN_POINT('Ctrl Pts',(-2.48542410286077E-7,-0.0309538112918512,
-0.0146758532742034));
#28681=CARTESIAN_POINT('Ctrl Pts',(0.000477085134298968,-0.0309842607700137,
-0.0146759007292687));
#28682=CARTESIAN_POINT('Ctrl Pts',(0.000955967382520689,-0.0310147074911929,
-0.0145349217410522));
#28683=CARTESIAN_POINT('Ctrl Pts',(0.00135783874524607,-0.0310451659129698,
-0.0142749659423983));
#28684=CARTESIAN_POINT('Ctrl Pts',(0.00150570845889031,-0.0310563731760992,
-0.0141793144651534));
#28685=CARTESIAN_POINT('Ctrl Pts',(0.00164329361716952,-0.0310675820233643,
-0.0140680572997739));
#28686=CARTESIAN_POINT('Ctrl Pts',(0.00176750903723605,-0.0310787931749967,
-0.0139438781176306));
#28687=CARTESIAN_POINT('Ctrl Pts',(0.00210520254732306,-0.0311092719444186,
-0.0136062831243902));
#28688=CARTESIAN_POINT('Ctrl Pts',(0.00234418991460515,-0.0311397677450743,
-0.0131678179909039));
#28689=CARTESIAN_POINT('Ctrl Pts',(0.00244450605500945,-0.0311702266377108,
-0.0126996759159109));
#28690=CARTESIAN_POINT('Ctrl Pts',(0.00248137363267524,-0.0311814207046412,
-0.0125276271883695));
#28691=CARTESIAN_POINT('Ctrl Pts',(0.00249996619645104,-0.0311926097865355,
-0.0123518243035685));
#28692=CARTESIAN_POINT('Ctrl Pts',(0.00249999995374699,-0.0312037912059132,
-0.0121763341867927));
#28693=CARTESIAN_POINT('Ctrl Pts',(0.00250009171282573,-0.0312341845390259,
-0.0116993169676925));
#28694=CARTESIAN_POINT('Ctrl Pts',(0.00235933720099796,-0.0312645212567865,
-0.0112206806977134));
#28695=CARTESIAN_POINT('Ctrl Pts',(0.00209969662614369,-0.0312948701586445,
-0.0108189177397613));
#28696=CARTESIAN_POINT('Ctrl Pts',(0.00200391124991896,-0.0313060663323708,
-0.0106707012443148));
#28697=CARTESIAN_POINT('Ctrl Pts',(0.00189245071359453,-0.0313172641643344,
-0.0105328053465568));
#28698=CARTESIAN_POINT('Ctrl Pts',(0.00176801705468482,-0.0313284671088737,
-0.0104083364706993));
#28699=CARTESIAN_POINT('Ctrl Pts',(0.00143048434324852,-0.0313588556731862,
-0.0100707082314775));
#28700=CARTESIAN_POINT('Ctrl Pts',(0.000992115626683919,-0.0313892818555032,
-0.0098317474532645));
#28701=CARTESIAN_POINT('Ctrl Pts',(0.000524080923154784,-0.0314197271687171,
-0.00973140259448324));
#28702=CARTESIAN_POINT('Ctrl Pts',(0.000351865041266604,-0.031430929685165,
-0.00969448016497607));
#28703=CARTESIAN_POINT('Ctrl Pts',(0.000175887412909158,-0.0314421347917672,
-0.00967586932025064));
#28704=CARTESIAN_POINT('Ctrl Pts',(2.2804493397338E-7,-0.0314533415675346,
-0.00967585329695899));
#28705=CARTESIAN_POINT('Ctrl Pts',(-0.00047537783123628,-0.031483684432076,
-0.00967580991315456));
#28706=CARTESIAN_POINT('Ctrl Pts',(-0.000952675722152286,-0.0315140395329462,
-0.00981580905674417));
#28707=CARTESIAN_POINT('Ctrl Pts',(-0.00135359513164503,-0.0315444118556672,
-0.0100740016696291));
#28708=CARTESIAN_POINT('Ctrl Pts',(-0.00150317654237353,-0.0315557436464764,
-0.0101703322896005));
#28709=CARTESIAN_POINT('Ctrl Pts',(-0.001642270366962,-0.0315670778345774,
-0.0102826000216382));
#28710=CARTESIAN_POINT('Ctrl Pts',(-0.00176769456660348,-0.0315784146788944,
-0.0104080139501928));
#28711=CARTESIAN_POINT('Ctrl Pts',(-0.0021101716270565,-0.0316093705002396,
-0.0107504629649284));
#28712=CARTESIAN_POINT('Ctrl Pts',(-0.00235088267097563,-0.0316403461260748,
-0.0111962655494278));
#28713=CARTESIAN_POINT('Ctrl Pts',(-0.00244877259416916,-0.0316713397992797,
-0.0116723527582108));
#28714=CARTESIAN_POINT('Ctrl Pts',(-0.00248282015087859,-0.0316821198552002,
-0.0118379428997785));
#28715=CARTESIAN_POINT('Ctrl Pts',(-0.00250000157476981,-0.0316929020944027,
-0.0120069670480985));
#28716=CARTESIAN_POINT('Ctrl Pts',(-0.00249999999989133,-0.0317036864429531,
-0.0121758765960527));
#28717=CARTESIAN_POINT('',(-0.00249999998015666,-0.0327037598573404,-0.0121760717152833));
#28718=CARTESIAN_POINT('Ctrl Pts',(-0.00249999960214269,-0.0317037743898623,
-0.0121772637072012));
#28719=CARTESIAN_POINT('Ctrl Pts',(-0.00249972562032444,-0.0317346929904582,
-0.0126629021158245));
#28720=CARTESIAN_POINT('Ctrl Pts',(-0.00235366036551277,-0.031765611591054,
-0.0131484341365877));
#28721=CARTESIAN_POINT('Ctrl Pts',(-0.00208616670586763,-0.0317965301916499,
-0.0135534992771266));
#28722=CARTESIAN_POINT('Ctrl Pts',(-0.00199318980764039,-0.0318072770466772,
-0.0136942940174477));
#28723=CARTESIAN_POINT('Ctrl Pts',(-0.00188599091826558,-0.0318180239017046,
-0.013825513267719));
#28724=CARTESIAN_POINT('Ctrl Pts',(-0.00176689483772362,-0.0318287707567319,
-0.0139444919247275));
#28725=CARTESIAN_POINT('Ctrl Pts',(-0.00143056933241676,-0.0318591197105435,
-0.0142804858277763));
#28726=CARTESIAN_POINT('Ctrl Pts',(-0.000994037072133453,-0.0318894686643551,
-0.0145187961010783));
#28727=CARTESIAN_POINT('Ctrl Pts',(-0.000527828984604696,-0.0319198176181668,
-0.0146194974020158));
#28728=CARTESIAN_POINT('Ctrl Pts',(-0.000353989560030296,-0.0319311341199783,
-0.0146570468497349));
#28729=CARTESIAN_POINT('Ctrl Pts',(-0.000176288435109386,-0.0319424506217898,
-0.0146759279515235));
#28730=CARTESIAN_POINT('Ctrl Pts',(1.05568559110729E-6,-0.0319537671236013,
-0.0146758530636637));
#28731=CARTESIAN_POINT('Ctrl Pts',(0.000478421868862688,-0.0319842283266928,
-0.0146756514842052));
#28732=CARTESIAN_POINT('Ctrl Pts',(0.000957259337678074,-0.0320146895297843,
-0.0145344041261251));
#28733=CARTESIAN_POINT('Ctrl Pts',(0.00135901157724633,-0.0320451507328759,
-0.0142742068156162));
#28734=CARTESIAN_POINT('Ctrl Pts',(0.0015067842549624,-0.0320563549854075,
-0.014178500931438));
#28735=CARTESIAN_POINT('Ctrl Pts',(0.00164427003901416,-0.0320675592379392,
-0.0140672041779086));
#28736=CARTESIAN_POINT('Ctrl Pts',(0.0017683879085218,-0.0320787634904709,
-0.0139429990657721));
#28737=CARTESIAN_POINT('Ctrl Pts',(0.00210576598572575,-0.03210921896953,
-0.0136053838450328));
#28738=CARTESIAN_POINT('Ctrl Pts',(0.00234448287598003,-0.032139674448589,
-0.0131670209427273));
#28739=CARTESIAN_POINT('Ctrl Pts',(0.00244463681756341,-0.032170129927648,
-0.0126990653183515));
#28740=CARTESIAN_POINT('Ctrl Pts',(0.00248150122990054,-0.0321813399042121,
-0.012526821382469));
#28741=CARTESIAN_POINT('Ctrl Pts',(0.00250004915629776,-0.0321925498807762,
-0.0123508229465227));
#28742=CARTESIAN_POINT('Ctrl Pts',(0.00249999990173367,-0.0322037598573404,
-0.0121751523360403));
#28743=CARTESIAN_POINT('Ctrl Pts',(0.00249986608599048,-0.0322342153363994,
-0.011697887056473));
#28744=CARTESIAN_POINT('Ctrl Pts',(0.0023587441528943,-0.0322646708154585,
-0.0112191133705348));
#28745=CARTESIAN_POINT('Ctrl Pts',(0.0020986943065755,-0.0322951262945174,
-0.0108173680243828));
#28746=CARTESIAN_POINT('Ctrl Pts',(0.00200297580951634,-0.0323063362710816,
-0.0106694946021195));
#28747=CARTESIAN_POINT('Ctrl Pts',(0.00189164762937877,-0.0323175462476457,
-0.0105319150538955));
#28748=CARTESIAN_POINT('Ctrl Pts',(0.0017673966851248,-0.0323287562242099,
-0.0104077161432884));
#28749=CARTESIAN_POINT('Ctrl Pts',(0.00142976589476869,-0.0323592174273014,
-0.0100702267455101));
#28750=CARTESIAN_POINT('Ctrl Pts',(0.000991342583344342,-0.0323896786303929,
-0.00983142577155676));
#28751=CARTESIAN_POINT('Ctrl Pts',(0.00052330153238317,-0.0324201398334844,
-0.0097312356260219));
#28752=CARTESIAN_POINT('Ctrl Pts',(0.000351146476182227,-0.0324313440860161,
-0.00969438364455593));
#28753=CARTESIAN_POINT('Ctrl Pts',(0.00017523882882955,-0.0324425483385477,
-0.00967582899443021));
#28754=CARTESIAN_POINT('Ctrl Pts',(-3.46215430472113E-7,-0.0324537525910794,
-0.00967585331053111));
#28755=CARTESIAN_POINT('Ctrl Pts',(-0.000475953346134224,-0.0324841015448911,
-0.00967591917554274));
#28756=CARTESIAN_POINT('Ctrl Pts',(-0.000953220233558734,-0.0325144504987029,
-0.00981602863242962));
#28757=CARTESIAN_POINT('Ctrl Pts',(-0.00135408116879281,-0.0325447994525146,
-0.0100743147576891));
#28758=CARTESIAN_POINT('Ctrl Pts',(-0.00150355398185469,-0.0325561159543261,
-0.0101706243511766));
#28759=CARTESIAN_POINT('Ctrl Pts',(-0.00164254774097299,-0.0325674324561375,
-0.0102828501979924));
#28760=CARTESIAN_POINT('Ctrl Pts',(-0.00176788634241805,-0.032578748957949,
-0.0104082057311071));
#28761=CARTESIAN_POINT('Ctrl Pts',(-0.00211033264092056,-0.0326096675585449,
-0.0107506982898004));
#28762=CARTESIAN_POINT('Ctrl Pts',(-0.00235099671033441,-0.0326405861591409,
-0.0111965357179675));
#28763=CARTESIAN_POINT('Ctrl Pts',(-0.00244883194213856,-0.0326715047597367,
-0.0116726414830778));
#28764=CARTESIAN_POINT('Ctrl Pts',(-0.00248283804307749,-0.032682251614764,
-0.0118381289093085));
#28765=CARTESIAN_POINT('Ctrl Pts',(-0.00249999942473484,-0.0326929984697912,
-0.0120070439058234));
#28766=CARTESIAN_POINT('Ctrl Pts',(-0.00249999999998548,-0.0327037453248185,
-0.0121758447668942));
#28767=CARTESIAN_POINT('',(-0.00249999963235903,-0.0337038344979968,-0.0121748826709929));
#28768=CARTESIAN_POINT('Ctrl Pts',(-0.00249999996032784,-0.0327037743898623,
-0.0121762986636724));
#28769=CARTESIAN_POINT('Ctrl Pts',(-0.00249991344322729,-0.0327346958161416,
-0.0126619382284563));
#28770=CARTESIAN_POINT('Ctrl Pts',(-0.00235403500626082,-0.0327656172424207,
-0.0131475274998857));
#28771=CARTESIAN_POINT('Ctrl Pts',(-0.002086696698559,-0.0327965386686998,
-0.0135526963742856));
#28772=CARTESIAN_POINT('Ctrl Pts',(-0.00199379624968891,-0.0328072839090873,
-0.0136934931445783));
#28773=CARTESIAN_POINT('Ctrl Pts',(-0.00188667695832345,-0.0328180291494749,
-0.0138247245135547));
#28774=CARTESIAN_POINT('Ctrl Pts',(-0.00176766084901072,-0.0328287743898623,
-0.013943726337112));
#28775=CARTESIAN_POINT('Ctrl Pts',(-0.00143147923482751,-0.0328591261823979,
-0.0142798675987047));
#28776=CARTESIAN_POINT('Ctrl Pts',(-0.000995047975805245,-0.0328894779749335,
-0.0145183673326568));
#28777=CARTESIAN_POINT('Ctrl Pts',(-0.000528881464056954,-0.032919829767469,
-0.0146192698284062));
#28778=CARTESIAN_POINT('Ctrl Pts',(-0.000355098798720773,-0.0329311446416001,
-0.0146568853675075));
#28779=CARTESIAN_POINT('Ctrl Pts',(-0.000177448203374564,-0.0329424595157312,
-0.0146758429789933));
#28780=CARTESIAN_POINT('Ctrl Pts',(-1.4527881610982E-7,-0.0329537743898623,
-0.0146758532823369));
#28781=CARTESIAN_POINT('Ctrl Pts',(0.000477223193183005,-0.0329842384343121,
-0.0146758810229475));
#28782=CARTESIAN_POINT('Ctrl Pts',(0.000956130225102326,-0.0330147024787618,
-0.0145348624432454));
#28783=CARTESIAN_POINT('Ctrl Pts',(0.00135800830274932,-0.0330451665232116,
-0.0142748562521739));
#28784=CARTESIAN_POINT('Ctrl Pts',(0.00150579197239822,-0.0330563691454285,
-0.0141792434999856));
#28785=CARTESIAN_POINT('Ctrl Pts',(0.00164330105990532,-0.0330675717676454,
-0.0140680423228023));
#28786=CARTESIAN_POINT('Ctrl Pts',(0.00176745536946942,-0.0330787743898623,
-0.0139439317681119));
#28787=CARTESIAN_POINT('Ctrl Pts',(0.0021050130607344,-0.0331092327066532,
-0.0136064930400484));
#28788=CARTESIAN_POINT('Ctrl Pts',(0.00234396153004447,-0.0331396910234439,
-0.0131682540553602));
#28789=CARTESIAN_POINT('Ctrl Pts',(0.00244436163814869,-0.0331701493402348,
-0.0127003494085143));
#28790=CARTESIAN_POINT('Ctrl Pts',(0.00248130785375645,-0.0331813576901106,
-0.0125281652715381));
#28791=CARTESIAN_POINT('Ctrl Pts',(0.0024999481909198,-0.0331925660399865,
-0.0123522187821387));
#28792=CARTESIAN_POINT('Ctrl Pts',(0.00249999989168001,-0.0332037743898623,
-0.0121765892212965));
#28793=CARTESIAN_POINT('Ctrl Pts',(0.00250014038677074,-0.0332342327066532,
-0.01169932175006));
#28794=CARTESIAN_POINT('Ctrl Pts',(0.00235929242057106,-0.0332646910234441,
-0.0112204653127318));
#28795=CARTESIAN_POINT('Ctrl Pts',(0.00209947166519535,-0.0332951493402349,
-0.0108185697026885));
#28796=CARTESIAN_POINT('Ctrl Pts',(0.00200386027763117,-0.0333063576901107,
-0.0106706762179027));
#28797=CARTESIAN_POINT('Ctrl Pts',(0.00189264067368614,-0.0333175660399865,
-0.0105330628179937));
#28798=CARTESIAN_POINT('Ctrl Pts',(0.00176849601540297,-0.0333287743898623,
-0.0104088156968323));
#28799=CARTESIAN_POINT('Ctrl Pts',(0.00143107360888865,-0.0333592384343121,
-0.0100711147985052));
#28800=CARTESIAN_POINT('Ctrl Pts',(0.000992796766610591,-0.0333897024787619,
-0.00983204084068172));
#28801=CARTESIAN_POINT('Ctrl Pts',(0.000524816137036575,-0.0334201665232118,
-0.00973156033719502));
#28802=CARTESIAN_POINT('Ctrl Pts',(0.000352724404221588,-0.0334313691454286,
-0.00969461038058061));
#28803=CARTESIAN_POINT('Ctrl Pts',(0.000176870514703275,-0.0334425717676454,
-0.00967594678850897));
#28804=CARTESIAN_POINT('Ctrl Pts',(1.32659061961387E-6,-0.0334537743898623,
-0.00967585363852665));
#28805=CARTESIAN_POINT('Ctrl Pts',(-0.000474282839167653,-0.033484126182398,
-0.00967560126288786));
#28806=CARTESIAN_POINT('Ctrl Pts',(-0.000951645230172061,-0.0335144779749335,
-0.00981539266180371));
#28807=CARTESIAN_POINT('Ctrl Pts',(-0.00135267984762792,-0.0335448297674692,
-0.0100734125074108));
#28808=CARTESIAN_POINT('Ctrl Pts',(-0.00150218193101796,-0.0335561446416002,
-0.0101695999755126));
#28809=CARTESIAN_POINT('Ctrl Pts',(-0.00164122048733436,-0.0335674595157313,
-0.0102817032164137));
#28810=CARTESIAN_POINT('Ctrl Pts',(-0.00176661971134624,-0.0335787743898623,
-0.0104069398360233));
#28811=CARTESIAN_POINT('Ctrl Pts',(-0.00210931224294895,-0.0336096958161413,
-0.0107491880003286));
#28812=CARTESIAN_POINT('Ctrl Pts',(-0.00235029576238914,-0.0336406172424204,
-0.0111948542068774));
#28813=CARTESIAN_POINT('Ctrl Pts',(-0.00244847155006307,-0.0336715386686993,
-0.0116708908438639));
#28814=CARTESIAN_POINT('Ctrl Pts',(-0.00248258777837945,-0.033682283909087,
-0.0118363142642324));
#28815=CARTESIAN_POINT('Ctrl Pts',(-0.00249986984268188,-0.0336930291494747,
-0.0120051756354036));
#28816=CARTESIAN_POINT('Ctrl Pts',(-0.00249999926483312,-0.0337037743898623,
-0.0121739360401313));
#28817=CARTESIAN_POINT('',(-0.00250011285302282,-0.03470351490128,-0.0121767698938277));
#28818=CARTESIAN_POINT('Ctrl Pts',(-0.00249999999988495,-0.0337038946061314,
-0.0121758293018544));
#28819=CARTESIAN_POINT('Ctrl Pts',(-0.00250000466247185,-0.033734778565668,
-0.0126618251857962));
#28820=CARTESIAN_POINT('Ctrl Pts',(-0.00235401049354569,-0.0337656732166077,
-0.0131477676332546));
#28821=CARTESIAN_POINT('Ctrl Pts',(-0.00208637960977751,-0.0337965745867032,
-0.013553176822952));
#28822=CARTESIAN_POINT('Ctrl Pts',(-0.00199358657942657,-0.0338072887155541,
-0.0136937403734454));
#28823=CARTESIAN_POINT('Ctrl Pts',(-0.00188661745613048,-0.0338180036521474,
-0.0138247680260886));
#28824=CARTESIAN_POINT('Ctrl Pts',(-0.00176777967268957,-0.0338287192309164,
-0.0139436075197097));
#28825=CARTESIAN_POINT('Ctrl Pts',(-0.00143185883991029,-0.0338590091441037,
-0.0142795331866852));
#28826=CARTESIAN_POINT('Ctrl Pts',(-0.000995819000972656,-0.0338893041884867,
-0.0145179579746008));
#28827=CARTESIAN_POINT('Ctrl Pts',(-0.00053009486265646,-0.033919615582755,
-0.01461900687088));
#28828=CARTESIAN_POINT('Ctrl Pts',(-0.000355871137815989,-0.0339309548361457,
-0.0146568084655417));
#28829=CARTESIAN_POINT('Ctrl Pts',(-0.000177759162184081,-0.0339422963776195,
-0.0146758524338922));
#28830=CARTESIAN_POINT('Ctrl Pts',(-1.19922745325362E-8,-0.0339536407945005,
-0.0146758532865293));
#28831=CARTESIAN_POINT('Ctrl Pts',(0.000475378078808354,-0.0339839817734889,
-0.0146758555669326));
#28832=CARTESIAN_POINT('Ctrl Pts',(0.000952534340723019,-0.0340143433205773,
-0.014535936885229));
#28833=CARTESIAN_POINT('Ctrl Pts',(0.00135340362296399,-0.0340446842363143,
-0.0142778282229805));
#28834=CARTESIAN_POINT('Ctrl Pts',(0.00150307914058896,-0.0340560128475831,
-0.0141814562899414));
#28835=CARTESIAN_POINT('Ctrl Pts',(0.00164226268650892,-0.0340673385826217,
-0.0140691239039628));
#28836=CARTESIAN_POINT('Ctrl Pts',(0.00176776271306561,-0.0340786592968838,
-0.013943624479415));
#28837=CARTESIAN_POINT('Ctrl Pts',(0.00211667616122357,-0.0341101329910108,
-0.013594712704954));
#28838=CARTESIAN_POINT('Ctrl Pts',(0.0023594874416597,-0.0341415678773693,
-0.0131392469395127));
#28839=CARTESIAN_POINT('Ctrl Pts',(0.00245403057651737,-0.0341731357263291,
-0.0126530680490265));
#28840=CARTESIAN_POINT('Ctrl Pts',(0.0024845703595109,-0.0341833329263505,
-0.0124960201805183));
#28841=CARTESIAN_POINT('Ctrl Pts',(0.0025,-0.0341935440003627,-0.0123359654368259));
#28842=CARTESIAN_POINT('Ctrl Pts',(0.0025,-0.0342037747380661,-0.0121758532865581));
#28843=CARTESIAN_POINT('Ctrl Pts',(0.00250000000000001,-0.034232937675464,
-0.0117194501658555));
#28844=CARTESIAN_POINT('Ctrl Pts',(0.00237063675736665,-0.0342622603896458,
-0.0112584460522841));
#28845=CARTESIAN_POINT('Ctrl Pts',(0.00212976212905734,-0.0342915473991,
-0.0108666117986602));
#28846=CARTESIAN_POINT('Ctrl Pts',(0.00202453898889524,-0.0343043410715692,
-0.0106954437894814));
#28847=CARTESIAN_POINT('Ctrl Pts',(0.00189872674918113,-0.0343171279306032,
-0.0105373403262591));
#28848=CARTESIAN_POINT('Ctrl Pts',(0.00175661849558318,-0.0343298916807547,
-0.0103970077449286));
#28849=CARTESIAN_POINT('Ctrl Pts',(0.0014136044427166,-0.0343607002056529,
-0.0100582797241931));
#28850=CARTESIAN_POINT('Ctrl Pts',(0.000969667592712359,-0.0343913740936313,
-0.00982187960567954));
#28851=CARTESIAN_POINT('Ctrl Pts',(0.000498228384675477,-0.0344219748273925,
-0.00972600258157551));
#28852=CARTESIAN_POINT('Ctrl Pts',(0.000327245261845305,-0.034433073202178,
-0.00969122958707377));
#28853=CARTESIAN_POINT('Ctrl Pts',(0.000152869457994301,-0.0344441619543187,
-0.00967448373110126));
#28854=CARTESIAN_POINT('Ctrl Pts',(-2.09597687845891E-5,-0.0344552440169733,
-0.00967594115048361));
#28855=CARTESIAN_POINT('Ctrl Pts',(-0.000498417069704019,-0.0344856831544058,
-0.0096799442490275));
#28856=CARTESIAN_POINT('Ctrl Pts',(-0.00097515733266665,-0.0345160718238225,
-0.00982503436728499));
#28857=CARTESIAN_POINT('Ctrl Pts',(-0.00137350204111084,-0.0345463934484738,
-0.0100869559355462));
#28858=CARTESIAN_POINT('Ctrl Pts',(-0.00152005468315037,-0.0345575488977853,
-0.0101833179482004));
#28859=CARTESIAN_POINT('Ctrl Pts',(-0.00165616134946322,-0.0345686952723593,
-0.0102949970394808));
#28860=CARTESIAN_POINT('Ctrl Pts',(-0.00177885400776298,-0.034579831746722,
-0.0104192433642744));
#28861=CARTESIAN_POINT('Ctrl Pts',(-0.00211985554664619,-0.0346107835163558,
-0.0107645630316637));
#28862=CARTESIAN_POINT('Ctrl Pts',(-0.0023572611775204,-0.0346416588109018,
-0.0112121927339843));
#28863=CARTESIAN_POINT('Ctrl Pts',(-0.00245193093994344,-0.0346724635377442,
-0.0116879653222178));
#28864=CARTESIAN_POINT('Ctrl Pts',(-0.00248390807885714,-0.034682868623848,
-0.0118486697092986));
#28865=CARTESIAN_POINT('Ctrl Pts',(-0.00250000157580861,-0.0346932656587147,
-0.012012385288373));
#28866=CARTESIAN_POINT('Ctrl Pts',(-0.00249999999988386,-0.0347036548700008,
-0.0121758773844318));
#28867=CARTESIAN_POINT('',(-0.00249999998223552,-0.0357037881422828,-0.0121756466480986));
#28868=CARTESIAN_POINT('Ctrl Pts',(-0.00249999927306645,-0.0347037743898623,
-0.0121777597668807));
#28869=CARTESIAN_POINT('Ctrl Pts',(-0.00249962892818142,-0.0347346957451935,
-0.0126633991581566));
#28870=CARTESIAN_POINT('Ctrl Pts',(-0.00235346674042249,-0.0347656171005246,
-0.0131489030560318));
#28871=CARTESIAN_POINT('Ctrl Pts',(-0.00208589171888402,-0.0347965384558557,
-0.0135539155990429));
#28872=CARTESIAN_POINT('Ctrl Pts',(-0.001992908184325,-0.0348072837671912,
-0.013694659296169));
#28873=CARTESIAN_POINT('Ctrl Pts',(-0.00188571114828099,-0.0348180290785268,
-0.0138258291141247));
#28874=CARTESIAN_POINT('Ctrl Pts',(-0.00176662425626108,-0.0348287743898623,
-0.0139447621980598));
#28875=CARTESIAN_POINT('Ctrl Pts',(-0.00143024572345875,-0.0348591261103602,
-0.0142807062771868));
#28876=CARTESIAN_POINT('Ctrl Pts',(-0.000993674819817364,-0.0348894778308581,
-0.0145189501297577));
#28877=CARTESIAN_POINT('Ctrl Pts',(-0.000527449318288785,-0.034919829551356,
-0.0146195793793591));
#28878=CARTESIAN_POINT('Ctrl Pts',(-0.000353643143028753,-0.0349311444975248,
-0.0146570933826369));
#28879=CARTESIAN_POINT('Ctrl Pts',(-0.000175979907123819,-0.0349424594436935,
-0.0146759468723011));
#28880=CARTESIAN_POINT('Ctrl Pts',(1.32451008204644E-6,-0.0349537743898623,
-0.0146758529356927));
#28881=CARTESIAN_POINT('Ctrl Pts',(0.000478692833169598,-0.0349842383622976,
-0.0146756000239945));
#28882=CARTESIAN_POINT('Ctrl Pts',(0.000957516810351806,-0.0350147023347329,
-0.0145342999583668));
#28883=CARTESIAN_POINT('Ctrl Pts',(0.00135924192416223,-0.0350451663071681,
-0.0142740576120707));
#28884=CARTESIAN_POINT('Ctrl Pts',(0.00150697064288591,-0.0350563690013995,
-0.0141783571764885));
#28885=CARTESIAN_POINT('Ctrl Pts',(0.00164441543894939,-0.0350675716956309,
-0.0140670740874734));
#28886=CARTESIAN_POINT('Ctrl Pts',(0.00176849761439238,-0.0350787743898623,
-0.0139428892759733));
#28887=CARTESIAN_POINT('Ctrl Pts',(0.0021058562184701,-0.0351092326347659,
-0.0136052516216866));
#28888=CARTESIAN_POINT('Ctrl Pts',(0.00234454622479179,-0.0351396908796696,
-0.0131668718932853));
#28889=CARTESIAN_POINT('Ctrl Pts',(0.00244467043999084,-0.0351701491245732,
-0.0126989081974757));
#28890=CARTESIAN_POINT('Ctrl Pts',(0.00248151545309635,-0.0351813575463362,
-0.0125267008201621));
#28891=CARTESIAN_POINT('Ctrl Pts',(0.00250005205495153,-0.0351925659680993,
-0.0123507418187357));
#28892=CARTESIAN_POINT('Ctrl Pts',(0.00249999988972694,-0.0352037743898623,
-0.0121751107467884));
#28893=CARTESIAN_POINT('Ctrl Pts',(0.00249985813371351,-0.0352342326347659,
-0.011697843356682));
#28894=CARTESIAN_POINT('Ctrl Pts',(0.0023587270467928,-0.0352646908796697,
-0.0112190703624375));
#28895=CARTESIAN_POINT('Ctrl Pts',(0.00209866872827452,-0.0352951491245732,
-0.0108173285098379));
#28896=CARTESIAN_POINT('Ctrl Pts',(0.00200296908024305,-0.0353063575463362,
-0.010669490309113));
#28897=CARTESIAN_POINT('Ctrl Pts',(0.00189166702651383,-0.0353175659680993,
-0.0105319415994415));
#28898=CARTESIAN_POINT('Ctrl Pts',(0.00176744762681308,-0.0353287743898623,
-0.0104077670651105));
#28899=CARTESIAN_POINT('Ctrl Pts',(0.00142982503833262,-0.0353592383622976,
-0.010070266418632));
#28900=CARTESIAN_POINT('Ctrl Pts',(0.000991406550564997,-0.0353897023347329,
-0.00983145246976956));
#28901=CARTESIAN_POINT('Ctrl Pts',(0.000523366478542818,-0.0354201663071682,
-0.00973124952947645));
#28902=CARTESIAN_POINT('Ctrl Pts',(0.00035125137352712,-0.0354313690013995,
-0.00969440131791859));
#28903=CARTESIAN_POINT('Ctrl Pts',(0.000175384892034823,-0.0354425716956309,
-0.00967584201682161));
#28904=CARTESIAN_POINT('Ctrl Pts',(-1.60569417170369E-7,-0.0354537743898623,
-0.0096758532917146));
#28905=CARTESIAN_POINT('Ctrl Pts',(-0.000475769978245463,-0.0354841261103602,
-0.0096758838390449));
#28906=CARTESIAN_POINT('Ctrl Pts',(-0.000953049059468749,-0.0355144778308581,
-0.00981595913017058));
#28907=CARTESIAN_POINT('Ctrl Pts',(-0.00135393008443228,-0.0355448295513561,
-0.0100742174174149));
#28908=CARTESIAN_POINT('Ctrl Pts',(-0.00150337621608888,-0.0355561444975248,
-0.0101704946158691));
#28909=CARTESIAN_POINT('Ctrl Pts',(-0.00164234917519774,-0.0355674594436935,
-0.0102826816354944));
#28910=CARTESIAN_POINT('Ctrl Pts',(-0.00176767473268967,-0.0355787743898623,
-0.0104079941181257));
#28911=CARTESIAN_POINT('Ctrl Pts',(-0.00211016298119799,-0.0356096957451935,
-0.0107504466358045));
#28912=CARTESIAN_POINT('Ctrl Pts',(-0.0023508805670986,-0.0356406171005249,
-0.0111962564868814));
#28913=CARTESIAN_POINT('Ctrl Pts',(-0.00244877235014627,-0.0356715384558562,
-0.011672351571408));
#28914=CARTESIAN_POINT('Ctrl Pts',(-0.00248279018910421,-0.0356822837671916,
-0.0118377967743644));
#28915=CARTESIAN_POINT('Ctrl Pts',(-0.00249997151790758,-0.0356930290785269,
-0.0120066699460638));
#28916=CARTESIAN_POINT('Ctrl Pts',(-0.00249999996448425,-0.0357037743898623,
-0.012175431885614));
#28917=CARTESIAN_POINT('',(-0.00249972264876189,-0.0367042860702267,-0.0121749056154874));
#28918=CARTESIAN_POINT('Ctrl Pts',(-0.0024999999999868,-0.0357038018947033,
-0.0121758614105833));
#28919=CARTESIAN_POINT('Ctrl Pts',(-0.00249999842185102,-0.0357347205736624,
-0.0126614999134783));
#28920=CARTESIAN_POINT('Ctrl Pts',(-0.00235420552434013,-0.0357656392526216,
-0.0131471138027068));
#28921=CARTESIAN_POINT('Ctrl Pts',(-0.00208693909926123,-0.0357965579315808,
-0.0135523289296316));
#28922=CARTESIAN_POINT('Ctrl Pts',(-0.00199404153534899,-0.0358073047732533,
-0.0136931752710327));
#28923=CARTESIAN_POINT('Ctrl Pts',(-0.00188691671847274,-0.0358180516149257,
-0.0138244541731427));
#28924=CARTESIAN_POINT('Ctrl Pts',(-0.00176788792603608,-0.0358287984565982,
-0.0139434992581757));
#28925=CARTESIAN_POINT('Ctrl Pts',(-0.00143175116039164,-0.035859147488347,
-0.0142796820340376));
#28926=CARTESIAN_POINT('Ctrl Pts',(-0.000995352781842014,-0.0358894965200957,
-0.0145182374567289));
#28927=CARTESIAN_POINT('Ctrl Pts',(-0.00052920129466083,-0.0359198455518445,
-0.0146192005786411));
#28928=CARTESIAN_POINT('Ctrl Pts',(-0.000355383620143761,-0.0359311620407274,
-0.0146568475143376));
#28929=CARTESIAN_POINT('Ctrl Pts',(-0.000177693789749482,-0.0359424785296102,
-0.0146758284126996));
#28930=CARTESIAN_POINT('Ctrl Pts',(-3.50299244509837E-7,-0.0359537950184931,
-0.0146758532620162));
#28931=CARTESIAN_POINT('Ctrl Pts',(0.000477015957030029,-0.035984256299687,
-0.0146759201504324));
#28932=CARTESIAN_POINT('Ctrl Pts',(0.000955932814372235,-0.0360147175808809,
-0.0145349420902015));
#28933=CARTESIAN_POINT('Ctrl Pts',(0.0013578313376968,-0.0360451788620748,
-0.0142749707340509));
#28934=CARTESIAN_POINT('Ctrl Pts',(0.00150565726978155,-0.0360563831015125,
-0.0141793483174259));
#28935=CARTESIAN_POINT('Ctrl Pts',(0.0016432051534008,-0.0360675873409502,
-0.0140681293640874));
#28936=CARTESIAN_POINT('Ctrl Pts',(0.00176739249258247,-0.0360787915803879,
-0.0139439946206044));
#28937=CARTESIAN_POINT('Ctrl Pts',(0.00210496066223601,-0.0361092471374863,
-0.0136065694174872));
#28938=CARTESIAN_POINT('Ctrl Pts',(0.00234392437601904,-0.0361397026945847,
-0.0131683409811333));
#28939=CARTESIAN_POINT('Ctrl Pts',(0.00244434181137516,-0.0361701582516831,
-0.0127004418006939));
#28940=CARTESIAN_POINT('Ctrl Pts',(0.00248130307216595,-0.0361813682152163,
-0.0125282192820577));
#28941=CARTESIAN_POINT('Ctrl Pts',(0.00249995009903626,-0.0361925781787496,
-0.0123522319776715));
#28942=CARTESIAN_POINT('Ctrl Pts',(0.00249999989954248,-0.0362037881422828,
-0.0121765620090651));
#28943=CARTESIAN_POINT('Ctrl Pts',(0.0025001351990157,-0.0362342436993812,
-0.0116992966956233));
#28944=CARTESIAN_POINT('Ctrl Pts',(0.00235928323479914,-0.0362646992564795,
-0.0112204434845985));
#28945=CARTESIAN_POINT('Ctrl Pts',(0.00209945993261631,-0.0362951548135779,
-0.0108185515546876));
#28946=CARTESIAN_POINT('Ctrl Pts',(0.00200382517758116,-0.0363063647771112,
-0.0106706247292461));
#28947=CARTESIAN_POINT('Ctrl Pts',(0.00189257505294478,-0.0363175747406445,
-0.0105329828990932));
#28948=CARTESIAN_POINT('Ctrl Pts',(0.00176839470571282,-0.0363287847041777,
-0.010408714309339));
#28949=CARTESIAN_POINT('Ctrl Pts',(0.0014309544933013,-0.0363592459853716,
-0.0100710343120011));
#28950=CARTESIAN_POINT('Ctrl Pts',(0.000992666047037264,-0.0363897072665655,
-0.00983198583372535));
#28951=CARTESIAN_POINT('Ctrl Pts',(0.000524681607744771,-0.0364201685477594,
-0.00973153145617357));
#28952=CARTESIAN_POINT('Ctrl Pts',(0.000352548016987815,-0.0364313727871972,
-0.0096945824226942));
#28953=CARTESIAN_POINT('Ctrl Pts',(0.00017665153322615,-0.0364425770266349,
-0.00967592846397843));
#28954=CARTESIAN_POINT('Ctrl Pts',(1.06714575491062E-6,-0.0364537812660726,
-0.00967585351431812));
#28955=CARTESIAN_POINT('Ctrl Pts',(-0.000474539983097998,-0.0364841302978213,
-0.0096756504974482));
#28956=CARTESIAN_POINT('Ctrl Pts',(-0.000951886033433265,-0.0365144793295702,
-0.00981549013244667));
#28957=CARTESIAN_POINT('Ctrl Pts',(-0.00135289294003649,-0.0365448283613189,
-0.0100735496232403));
#28958=CARTESIAN_POINT('Ctrl Pts',(-0.00150241962800714,-0.0365561448502018,
-0.0101697743523469));
#28959=CARTESIAN_POINT('Ctrl Pts',(-0.00164147633810056,-0.0365674613390846,
-0.0102819211394351));
#28960=CARTESIAN_POINT('Ctrl Pts',(-0.00176688542553261,-0.0365787778279675,
-0.0104072052455278));
#28961=CARTESIAN_POINT('Ctrl Pts',(-0.00210952556356602,-0.0366096965069265,
-0.0107495039121076));
#28962=CARTESIAN_POINT('Ctrl Pts',(-0.00235044197743157,-0.0366406151858856,
-0.011195205053263));
#28963=CARTESIAN_POINT('Ctrl Pts',(-0.00244854670136544,-0.0366715338648448,
-0.0116712553761062));
#28964=CARTESIAN_POINT('Ctrl Pts',(-0.0024826463450416,-0.0366822807065173,
-0.0118367229064141));
#28965=CARTESIAN_POINT('Ctrl Pts',(-0.00249990333900219,-0.0366930275481898,
-0.0120056275156314));
#28966=CARTESIAN_POINT('Ctrl Pts',(-0.00249999959355058,-0.0367037743898623,
-0.0121744277175772));
#28967=CARTESIAN_POINT('',(-0.00249992752834032,-0.037703848024675,-0.0121772085200007));
#28968=CARTESIAN_POINT('Ctrl Pts',(-0.00249923804932589,-0.0367051814111975,
-0.0121757418437438));
#28969=CARTESIAN_POINT('Ctrl Pts',(-0.00249855972559852,-0.0367376271573855,
-0.0126675611060721));
#28970=CARTESIAN_POINT('Ctrl Pts',(-0.00235152199160866,-0.0367651264597615,
-0.0131596652408496));
#28971=CARTESIAN_POINT('Ctrl Pts',(-0.00207812613851097,-0.0367966312627343,
-0.0135691277197265));
#28972=CARTESIAN_POINT('Ctrl Pts',(-0.0020685210477245,-0.0367977381064897,
-0.0135835131767066));
#28973=CARTESIAN_POINT('Ctrl Pts',(-0.00205875490051772,-0.0367988448921768,
-0.013597788859014));
#28974=CARTESIAN_POINT('Ctrl Pts',(-0.00204882967407331,-0.0367999522846867,
-0.0136119509893344));
#28975=CARTESIAN_POINT('Ctrl Pts',(-0.00196547955788986,-0.0368092519510344,
-0.0137308817980391));
#28976=CARTESIAN_POINT('Ctrl Pts',(-0.0018709240015511,-0.0368185944124242,
-0.0138417564093648));
#28977=CARTESIAN_POINT('Ctrl Pts',(-0.00176808080539617,-0.0368283734436502,
-0.0139439442940955));
#28978=CARTESIAN_POINT('Ctrl Pts',(-0.00153624688627666,-0.0368504177909582,
-0.0141743009797042));
#28979=CARTESIAN_POINT('Ctrl Pts',(-0.00125868197897531,-0.0368724829537764,
-0.0143590236955169));
#28980=CARTESIAN_POINT('Ctrl Pts',(-0.000956441897266579,-0.0368927141725844,
-0.0144845980144631));
#28981=CARTESIAN_POINT('Ctrl Pts',(-0.000654201815557846,-0.0369129453913923,
-0.0146101723334094));
#28982=CARTESIAN_POINT('Ctrl Pts',(-0.00032735114465414,-0.0369316777830255,
-0.0146769121014811));
#28983=CARTESIAN_POINT('Ctrl Pts',(7.98294045574838E-8,-0.0369526287167429,
-0.0146777668731382));
#28984=CARTESIAN_POINT('Ctrl Pts',(2.47087250033536E-5,-0.0369542046163984,
-0.0146778311678555));
#28985=CARTESIAN_POINT('Ctrl Pts',(4.93327602190462E-5,-0.0369557877516931,
-0.014677514822621));
#28986=CARTESIAN_POINT('Ctrl Pts',(7.39420047343854E-5,-0.0369573773469808,
-0.0146768118236171));
#28987=CARTESIAN_POINT('Ctrl Pts',(0.000376502481255991,-0.0369769207631717,
-0.0146681687418079));
#28988=CARTESIAN_POINT('Ctrl Pts',(0.00067701295653365,-0.0369974406515327,
-0.0146009312101924));
#28989=CARTESIAN_POINT('Ctrl Pts',(0.000956270931532571,-0.0370174955425343,
-0.0144847845969389));
#28990=CARTESIAN_POINT('Ctrl Pts',(0.00125824280448874,-0.0370391816304525,
-0.014359191011503));
#28991=CARTESIAN_POINT('Ctrl Pts',(0.00153575432463791,-0.0370591854105042,
-0.0141743965678716));
#28992=CARTESIAN_POINT('Ctrl Pts',(0.00176771012644472,-0.0370786390032289,
-0.0139435813207743));
#28993=CARTESIAN_POINT('Ctrl Pts',(0.00188368802734813,-0.0370883657995912,
-0.0138281736972256));
#28994=CARTESIAN_POINT('Ctrl Pts',(0.00198878162811406,-0.037098386354272,
-0.0137017201996478));
#28995=CARTESIAN_POINT('Ctrl Pts',(0.00208027048894701,-0.0371088726100384,
-0.013565738145873));
#28996=CARTESIAN_POINT('Ctrl Pts',(0.00209738775771892,-0.0371108345544405,
-0.0135402963451836));
#28997=CARTESIAN_POINT('Ctrl Pts',(0.00211400414750772,-0.0371127972484263,
-0.013514509538353));
#28998=CARTESIAN_POINT('Ctrl Pts',(0.00213009819447958,-0.0371147630535618,
-0.0134884013575589));
#28999=CARTESIAN_POINT('Ctrl Pts',(0.00220002406360927,-0.0371233041391496,
-0.0133749657974033));
#29000=CARTESIAN_POINT('Ctrl Pts',(0.00226003460348998,-0.0371319039555668,
-0.0132554650136785));
#29001=CARTESIAN_POINT('Ctrl Pts',(0.00231026196285467,-0.0371407561975987,
-0.0131327594162781));
#29002=CARTESIAN_POINT('Ctrl Pts',(0.00237204958583781,-0.037151645860128,
-0.012981812058384));
#29003=CARTESIAN_POINT('Ctrl Pts',(0.00241912822389077,-0.0371627376694534,
-0.0128259652542995));
#29004=CARTESIAN_POINT('Ctrl Pts',(0.00245118988178313,-0.0371737434262344,
-0.0126635182536309));
#29005=CARTESIAN_POINT('Ctrl Pts',(0.00246722071072931,-0.0371792463046249,
-0.0125822947532966));
#29006=CARTESIAN_POINT('Ctrl Pts',(0.00247924886171843,-0.037184729174554,
-0.0124993501380759));
#29007=CARTESIAN_POINT('Ctrl Pts',(0.00248695105986065,-0.0371898047233834,
-0.0124209100338158));
#29008=CARTESIAN_POINT('Ctrl Pts',(0.00249080215893176,-0.0371923424977981,
-0.0123816899816858));
#29009=CARTESIAN_POINT('Ctrl Pts',(0.00249374966613724,-0.0371947823017465,
-0.0123436223993365));
#29010=CARTESIAN_POINT('Ctrl Pts',(0.00249597895609703,-0.0371976356976271,
-0.012298583023874));
#29011=CARTESIAN_POINT('Ctrl Pts',(0.00249820824605681,-0.0372004890935078,
-0.0122535436484114));
#29012=CARTESIAN_POINT('Ctrl Pts',(0.00249904761869242,-0.0372037421797348,
-0.0122014924554208));
#29013=CARTESIAN_POINT('Ctrl Pts',(0.00249907294475291,-0.0372053301768058,
-0.0121759520549198));
#29014=CARTESIAN_POINT('Ctrl Pts',(0.00249908560778316,-0.0372061241753414,
-0.0121631818546693));
#29015=CARTESIAN_POINT('Ctrl Pts',(0.00249902385857616,-0.0372065047276103,
-0.0121570379698692));
#29016=CARTESIAN_POINT('Ctrl Pts',(0.00249899372733659,-0.0372067387506886,
-0.0121532622930291));
#29017=CARTESIAN_POINT('Ctrl Pts',(0.00249896359609703,-0.0372069727737668,
-0.0121494866161891));
#29018=CARTESIAN_POINT('Ctrl Pts',(0.00249894915827925,-0.0372070598936226,
-0.012148079571669));
#29019=CARTESIAN_POINT('Ctrl Pts',(0.00249891180836883,-0.0372072637224387,
-0.0121447869733562));
#29020=CARTESIAN_POINT('Ctrl Pts',(0.00249883710854799,-0.037207671380071,
-0.0121382017767306));
#29021=CARTESIAN_POINT('Ctrl Pts',(0.00249862743784474,-0.037208544928947,
-0.0121240749706626));
#29022=CARTESIAN_POINT('Ctrl Pts',(0.00249829606817123,-0.03720936813279,
-0.0121107206095793));
#29023=CARTESIAN_POINT('Ctrl Pts',(0.0024976333288242,-0.0372110145404761,
-0.0120840118874126));
#29024=CARTESIAN_POINT('Ctrl Pts',(0.00249668406465387,-0.0372124639781498,
-0.0120603837583854));
#29025=CARTESIAN_POINT('Ctrl Pts',(0.0024952206104089,-0.0372140812858203,
-0.0120339199927811));
#29026=CARTESIAN_POINT('Ctrl Pts',(0.00249229370191897,-0.0372173159011614,
-0.0119809924615723));
#29027=CARTESIAN_POINT('Ctrl Pts',(0.002487012242735,-0.0372212121210945,
-0.0119167482118306));
#29028=CARTESIAN_POINT('Ctrl Pts',(0.00247777616113699,-0.0372254769490124,
-0.0118461480055289));
#29029=CARTESIAN_POINT('Ctrl Pts',(0.00246854007953898,-0.0372297417769303,
-0.0117755477992272));
#29030=CARTESIAN_POINT('Ctrl Pts',(0.00245548734276733,-0.0372343746526518,
-0.0116985653847269));
#29031=CARTESIAN_POINT('Ctrl Pts',(0.002436394845427,-0.0372394863755516,
-0.0116147295254093));
#29032=CARTESIAN_POINT('Ctrl Pts',(0.00241730234808667,-0.0372445980984513,
-0.0115308936660916));
#29033=CARTESIAN_POINT('Ctrl Pts',(0.00239213549960774,-0.0372501832347442,
-0.01144023087194));
#29034=CARTESIAN_POINT('Ctrl Pts',(0.00235885979455609,-0.0372566368387057,
-0.0113439889242858));
#29035=CARTESIAN_POINT('Ctrl Pts',(0.00233366528118125,-0.037261523148735,
-0.0112711198736187));
#29036=CARTESIAN_POINT('Ctrl Pts',(0.0023035388911288,-0.0372667114623,
-0.011195276533937));
#29037=CARTESIAN_POINT('Ctrl Pts',(0.00226725689186798,-0.0372722367914396,
-0.0111174342408781));
#29038=CARTESIAN_POINT('Ctrl Pts',(0.00220769984171952,-0.037281306641816,
-0.0109896557985147));
#29039=CARTESIAN_POINT('Ctrl Pts',(0.00213143837634023,-0.0372912845926809,
-0.0108564220403585));
#29040=CARTESIAN_POINT('Ctrl Pts',(0.00203506830126738,-0.0373023255054793,
-0.010722635940189));
#29041=CARTESIAN_POINT('Ctrl Pts',(0.00187998982838368,-0.037320092513492,
-0.0105073476975298));
#29042=CARTESIAN_POINT('Ctrl Pts',(0.00167209784656463,-0.0373402307396795,
-0.0102902804756762));
#29043=CARTESIAN_POINT('Ctrl Pts',(0.00140122162816635,-0.0373606613334278,
-0.0101065759256013));
#29044=CARTESIAN_POINT('Ctrl Pts',(0.00113034540976807,-0.0373810919271762,
-0.00992287137552641));
#29045=CARTESIAN_POINT('Ctrl Pts',(0.000795801869857682,-0.0374013980344111,
-0.00977278122525912));
#29046=CARTESIAN_POINT('Ctrl Pts',(0.000411562655167207,-0.0374263325491636,
-0.00970796947441034));
#29047=CARTESIAN_POINT('Ctrl Pts',(0.000394994239586353,-0.0374274077267794,
-0.0097051747882317));
#29048=CARTESIAN_POINT('Ctrl Pts',(0.00037834529328193,-0.0374284912538621,
-0.00970254432404357));
#29049=CARTESIAN_POINT('Ctrl Pts',(0.000361617587882895,-0.0374295827143858,
-0.00970008436041701));
#29050=CARTESIAN_POINT('Ctrl Pts',(-9.58802205126288E-6,-0.0374538033866029,
-0.00964549514589953));
#29051=CARTESIAN_POINT('Ctrl Pts',(-0.000423761120905089,-0.0374819308294292,
-0.00967548372821087));
#29052=CARTESIAN_POINT('Ctrl Pts',(-0.000830943860492442,-0.0375094187748174,
-0.00981905156170969));
#29053=CARTESIAN_POINT('Ctrl Pts',(-0.00120508340729675,-0.0375346760522761,
-0.00995096875499584));
#29054=CARTESIAN_POINT('Ctrl Pts',(-0.00157461097999646,-0.0375587613643777,
-0.0101807716301553));
#29055=CARTESIAN_POINT('Ctrl Pts',(-0.00186972884662011,-0.0375869868999544,
-0.0105132308823403));
#29056=CARTESIAN_POINT('Ctrl Pts',(-0.00188237997769656,-0.0375881968739704,
-0.0105274827662574));
#29057=CARTESIAN_POINT('Ctrl Pts',(-0.00189489004442169,-0.037589414456354,
-0.0105419235332971));
#29058=CARTESIAN_POINT('Ctrl Pts',(-0.00190725605658699,-0.0375906400655857,
-0.0105565503326961));
#29059=CARTESIAN_POINT('Ctrl Pts',(-0.00193451409969029,-0.0375933416405815,
-0.0105887917637372));
#29060=CARTESIAN_POINT('Ctrl Pts',(-0.00196101730123458,-0.037596055918673,
-0.0106219374042091));
#29061=CARTESIAN_POINT('Ctrl Pts',(-0.00198680450692279,-0.0375988418278651,
-0.010655880158455));
#29062=CARTESIAN_POINT('Ctrl Pts',(-0.00224671291071142,-0.0376269209156098,
-0.0109979880697548));
#29063=CARTESIAN_POINT('Ctrl Pts',(-0.00243044774190981,-0.0376584425706656,
-0.0114279639088363));
#29064=CARTESIAN_POINT('Ctrl Pts',(-0.00248377020356829,-0.0376872536324111,
-0.0118982228572852));
#29065=CARTESIAN_POINT('Ctrl Pts',(-0.00249412635367718,-0.0376928492420463,
-0.0119895553297315));
#29066=CARTESIAN_POINT('Ctrl Pts',(-0.00249958564975923,-0.0376984023199869,
-0.0120822814837863));
#29067=CARTESIAN_POINT('Ctrl Pts',(-0.00249980699897089,-0.037703972088345,
-0.0121758498398408));
#29068=CARTESIAN_POINT('',(-0.00249999985275848,-0.0387038137045467,-0.0121752545238663));
#29069=CARTESIAN_POINT('Ctrl Pts',(-0.00249999906545952,-0.0377037743898623,
-0.0121780149297994));
#29070=CARTESIAN_POINT('Ctrl Pts',(-0.00249957915265185,-0.0377346978836163,
-0.012663655486345));
#29071=CARTESIAN_POINT('Ctrl Pts',(-0.00235336672748243,-0.0377656213773703,
-0.0131491454651922));
#29072=CARTESIAN_POINT('Ctrl Pts',(-0.00208574922620988,-0.0377965448711243,
-0.0135541312575657));
#29073=CARTESIAN_POINT('Ctrl Pts',(-0.00199277586707078,-0.037807288044037,
-0.0136948279210557));
#29074=CARTESIAN_POINT('Ctrl Pts',(-0.00188559757212201,-0.0378180312169497,
-0.0138259543605948));
#29075=CARTESIAN_POINT('Ctrl Pts',(-0.00176653632040396,-0.0378287743898624,
-0.0139448500159767));
#29076=CARTESIAN_POINT('Ctrl Pts',(-0.00143013920781834,-0.0378591282816254,
-0.0142807792506547));
#29077=CARTESIAN_POINT('Ctrl Pts',(-0.00099355393580092,-0.0378894821733885,
-0.0145190018168816));
#29078=CARTESIAN_POINT('Ctrl Pts',(-0.000527321111942944,-0.0379198360651516,
-0.0146196070476599));
#29079=CARTESIAN_POINT('Ctrl Pts',(-0.000353557990227819,-0.0379311488400552,
-0.0146571022175972));
#29080=CARTESIAN_POINT('Ctrl Pts',(-0.000175940789421143,-0.0379424616149587,
-0.0146759463829256));
#29081=CARTESIAN_POINT('Ctrl Pts',(1.31790050661161E-6,-0.0379537743898623,
-0.0146758529391857));
#29082=CARTESIAN_POINT('Ctrl Pts',(0.000478688717282434,-0.0379842405328645,
-0.0146756012882542));
#29083=CARTESIAN_POINT('Ctrl Pts',(0.000957515025671042,-0.0380147066758667,
-0.0145343010843038));
#29084=CARTESIAN_POINT('Ctrl Pts',(0.00135924181305373,-0.0380451728188689,
-0.0142740576840481));
#29085=CARTESIAN_POINT('Ctrl Pts',(0.00150693200109036,-0.0380563733425334,
-0.0141783822202099));
#29086=CARTESIAN_POINT('Ctrl Pts',(0.00164434366011201,-0.0380675738661978,
-0.0140671322639597));
#29087=CARTESIAN_POINT('Ctrl Pts',(0.00176840042766013,-0.0380787743898623,
-0.0139429865377453));
#29088=CARTESIAN_POINT('Ctrl Pts',(0.00210577931443683,-0.0381092348014942,
-0.0136053657232093));
#29089=CARTESIAN_POINT('Ctrl Pts',(0.00234449381233911,-0.0381396952131261,
-0.0131669968114185));
#29090=CARTESIAN_POINT('Ctrl Pts',(0.0024446429880769,-0.0381701556247581,
-0.0126990364866386));
#29091=CARTESIAN_POINT('Ctrl Pts',(0.00248148744108023,-0.0381813618797928,
-0.0125268758865462));
#29092=CARTESIAN_POINT('Ctrl Pts',(0.00250003325712235,-0.0381925681348276,
-0.012350964658492));
#29093=CARTESIAN_POINT('Ctrl Pts',(0.00249999995503491,-0.0382037743898623,
-0.0121753791289363));
#29094=CARTESIAN_POINT('Ctrl Pts',(0.00249990943458105,-0.0382342348014941,
-0.0116981092925555));
#29095=CARTESIAN_POINT('Ctrl Pts',(0.00235882837656811,-0.038264695213126,
-0.0112193192424479));
#29096=CARTESIAN_POINT('Ctrl Pts',(0.00209881112704663,-0.0382951556247579,
-0.0108175485147984));
#29097=CARTESIAN_POINT('Ctrl Pts',(0.00200315189411168,-0.0383063618797927,
-0.0106697387841232));
#29098=CARTESIAN_POINT('Ctrl Pts',(0.0018918973356533,-0.0383175681348275,
-0.0105322115233738));
#29099=CARTESIAN_POINT('Ctrl Pts',(0.00176772998068626,-0.0383287743898623,
-0.0104080493620849));
#29100=CARTESIAN_POINT('Ctrl Pts',(0.00143015954516786,-0.0383592405328645,
-0.0100704930464788));
#29101=CARTESIAN_POINT('Ctrl Pts',(0.000991776834235544,-0.0383897066758667,
-0.00983160868598701));
#29102=CARTESIAN_POINT('Ctrl Pts',(0.000523750573447141,-0.0384201728188689,
-0.00973133179211101));
#29103=CARTESIAN_POINT('Ctrl Pts',(0.000351686153964219,-0.0384313733425333,
-0.00969446615661599));
#29104=CARTESIAN_POINT('Ctrl Pts',(0.000175869444756074,-0.0384425738661978,
-0.00967587925874551));
#29105=CARTESIAN_POINT('Ctrl Pts',(3.69585316966004E-7,-0.0384537743898623,
-0.00967585331387676));
#29106=CARTESIAN_POINT('Ctrl Pts',(-0.000475242439390424,-0.0384841282816254,
-0.00967578300218763));
#29107=CARTESIAN_POINT('Ctrl Pts',(-0.000952553277734538,-0.0385144821733884,
-0.00981575854653882));
#29108=CARTESIAN_POINT('Ctrl Pts',(-0.00135349011024409,-0.0385448360651514,
-0.0100739340394243));
#29109=CARTESIAN_POINT('Ctrl Pts',(-0.0015029176753208,-0.038556148840055,
-0.0101701550202279));
#29110=CARTESIAN_POINT('Ctrl Pts',(-0.00164188085258634,-0.0385674616149587,
-0.010282279737598));
#29111=CARTESIAN_POINT('Ctrl Pts',(-0.00176720721992576,-0.0385787743898623,
-0.0104075267777249));
#29112=CARTESIAN_POINT('Ctrl Pts',(-0.00210978710599715,-0.0386096978836163,
-0.0107498898226957));
#29113=CARTESIAN_POINT('Ctrl Pts',(-0.00235062273498652,-0.0386406213773703,
-0.0111956374309725));
#29114=CARTESIAN_POINT('Ctrl Pts',(-0.00244863989484262,-0.0386715448711244,
-0.0116717078061805));
#29115=CARTESIAN_POINT('Ctrl Pts',(-0.00248269216930797,-0.038682288044037,
-0.0118371000610185));
#29116=CARTESIAN_POINT('Ctrl Pts',(-0.00249991782187621,-0.0386930312169497,
-0.0120059228706272));
#29117=CARTESIAN_POINT('Ctrl Pts',(-0.00249999970556691,-0.0387037743898623,
-0.0121746399583445));
#29118=CARTESIAN_POINT('',(-0.00249999994305708,-0.0397037978472385,-0.0121754691093855));
#29119=CARTESIAN_POINT('Ctrl Pts',(-0.00249999999995005,-0.0387038530192311,
-0.0121758690893881));
#29120=CARTESIAN_POINT('Ctrl Pts',(-0.0024999969301698,-0.0387347687629928,
-0.012661506828381));
#29121=CARTESIAN_POINT('Ctrl Pts',(-0.00235420297464426,-0.0387656845067545,
-0.0131471196348283));
#29122=CARTESIAN_POINT('Ctrl Pts',(-0.00208693602911737,-0.0387966002505162,
-0.013552333584409));
#29123=CARTESIAN_POINT('Ctrl Pts',(-0.00199402250511303,-0.0388073478971975,
-0.0136932034400399));
#29124=CARTESIAN_POINT('Ctrl Pts',(-0.00188687694470658,-0.0388180955438787,
-0.0138245025803785));
#29125=CARTESIAN_POINT('Ctrl Pts',(-0.00176782386158655,-0.03882884319056,
-0.0139435633290722));
#29126=CARTESIAN_POINT('Ctrl Pts',(-0.00143167610268005,-0.0388591892954298,
-0.0142797327318146));
#29127=CARTESIAN_POINT('Ctrl Pts',(-0.000995270678790388,-0.0388895354002997,
-0.0145182720734748));
#29128=CARTESIAN_POINT('Ctrl Pts',(-0.000529117003512208,-0.0389198815051695,
-0.0146192188336251));
#29129=CARTESIAN_POINT('Ctrl Pts',(-0.000355269510177465,-0.0389311987907426,
-0.014656865949036));
#29130=CARTESIAN_POINT('Ctrl Pts',(-0.000177549231046672,-0.0389425160763158,
-0.0146758407388477));
#29131=CARTESIAN_POINT('Ctrl Pts',(-1.76767305915852E-7,-0.0389538333618889,
-0.0146758532803088));
#29132=CARTESIAN_POINT('Ctrl Pts',(0.000477187912742321,-0.038984291710906,
-0.0146758870332962));
#29133=CARTESIAN_POINT('Ctrl Pts',(0.000956093742291461,-0.0390147500599231,
-0.0145348766195195));
#29134=CARTESIAN_POINT('Ctrl Pts',(0.00135797359406222,-0.0390452084089402,
-0.0142748787075165));
#29135=CARTESIAN_POINT('Ctrl Pts',(0.00150581747045849,-0.039056413450366,
-0.0141792304708705));
#29136=CARTESIAN_POINT('Ctrl Pts',(0.00164337882623664,-0.039067618491792,
-0.0140679812187286));
#29137=CARTESIAN_POINT('Ctrl Pts',(0.00176757386523736,-0.0390788235332179,
-0.0139438133061654));
#29138=CARTESIAN_POINT('Ctrl Pts',(0.00210510633250146,-0.0391092761608647,
-0.0136063545620827));
#29139=CARTESIAN_POINT('Ctrl Pts',(0.00234402484748426,-0.0391397287885115,
-0.0131681030789221));
#29140=CARTESIAN_POINT('Ctrl Pts',(0.00244439477502579,-0.0391701814161583,
-0.0127001949536289));
#29141=CARTESIAN_POINT('Ctrl Pts',(0.00248134473752436,-0.0391813921789545,
-0.012527940294232));
#29142=CARTESIAN_POINT('Ctrl Pts',(0.00249997401585501,-0.0391926029417506,
-0.012351921455295));
#29143=CARTESIAN_POINT('Ctrl Pts',(0.00249999997271797,-0.0392038137045467,
-0.0121762226239989));
#29144=CARTESIAN_POINT('Ctrl Pts',(0.00250007048127274,-0.0392342663321936,
-0.0116989588387642));
#29145=CARTESIAN_POINT('Ctrl Pts',(0.00235915437950149,-0.0392647189598404,
-0.0112201259624989));
#29146=CARTESIAN_POINT('Ctrl Pts',(0.00209927782671647,-0.0392951715874873,
-0.010818269916648));
#29147=CARTESIAN_POINT('Ctrl Pts',(0.00200360744899664,-0.0393063823502834,
-0.0106703315232702));
#29148=CARTESIAN_POINT('Ctrl Pts',(0.00189231790892485,-0.0393175931130795,
-0.0105326836318434));
#29149=CARTESIAN_POINT('Ctrl Pts',(0.00176809616713814,-0.0393288038758756,
-0.010408415609085));
#29150=CARTESIAN_POINT('Ctrl Pts',(0.00143060002743081,-0.0393592622248927,
-0.0100707937293175));
#29151=CARTESIAN_POINT('Ctrl Pts',(0.000992272707346792,-0.0393897205739098,
-0.00983181954340048));
#29152=CARTESIAN_POINT('Ctrl Pts',(0.000524272698241825,-0.039420178922927,
-0.00973144371820049));
#29153=CARTESIAN_POINT('Ctrl Pts',(0.000352104486288874,-0.0394313839643528,
-0.0096945173805685));
#29154=CARTESIAN_POINT('Ctrl Pts',(0.000176175198052129,-0.0394425890057786,
-0.00967589282108229));
#29155=CARTESIAN_POINT('Ctrl Pts',(5.61907573495769E-7,-0.0394537940472045,
-0.00967585334970612));
#29156=CARTESIAN_POINT('Ctrl Pts',(-0.000475043592385584,-0.0394841401520743,
-0.00967574645117045));
#29157=CARTESIAN_POINT('Ctrl Pts',(-0.000952360064664738,-0.0395144862569442,
-0.00981568162193327));
#29158=CARTESIAN_POINT('Ctrl Pts',(-0.00135331414519892,-0.039544832361814,
-0.0100738207405673));
#29159=CARTESIAN_POINT('Ctrl Pts',(-0.00150284608185382,-0.0395561496473871,
-0.010170091221926));
#29160=CARTESIAN_POINT('Ctrl Pts',(-0.00164190139392532,-0.0395674669329603,
-0.0102822869096362));
#29161=CARTESIAN_POINT('Ctrl Pts',(-0.00176730147922207,-0.0395787842185334,
-0.0104076209823799));
#29162=CARTESIAN_POINT('Ctrl Pts',(-0.00210986037991485,-0.0396096999622953,
-0.0107499995547453));
#29163=CARTESIAN_POINT('Ctrl Pts',(-0.00235067181986224,-0.0396406157060572,
-0.0111957564616439));
#29164=CARTESIAN_POINT('Ctrl Pts',(-0.00244866486404371,-0.0396715314498192,
-0.0116718290970614));
#29165=CARTESIAN_POINT('Ctrl Pts',(-0.00248273147502909,-0.0396822790965002,
-0.0118373324897463));
#29166=CARTESIAN_POINT('Ctrl Pts',(-0.00249994893517625,-0.0396930267431813,
-0.0120062701810751));
#29167=CARTESIAN_POINT('Ctrl Pts',(-0.00249999988615268,-0.0397037743898623,
-0.0121750988088553));
#29168=CARTESIAN_POINT('Ctrl Pts',(-0.00249999999996149,-0.0397038213046146,
-0.0121758394099156));
#29169=CARTESIAN_POINT('Ctrl Pts',(-0.00250000270759189,-0.0397348741491189,
-0.0126636429977115));
#29170=CARTESIAN_POINT('Ctrl Pts',(-0.00235297981442275,-0.0397659269936232,
-0.0131510877618962));
#29171=CARTESIAN_POINT('Ctrl Pts',(-0.00208362329733661,-0.0397969798381275,
-0.0135573430457659));
#29172=CARTESIAN_POINT('Ctrl Pts',(-0.00203675232193105,-0.0398023833721752,
-0.0136280359015566));
#29173=CARTESIAN_POINT('Ctrl Pts',(-0.00198629761776183,-0.0398077869062229,
-0.0136963151048329));
#29174=CARTESIAN_POINT('Ctrl Pts',(-0.00193253383622679,-0.0398131904402706,
-0.0137618271110075));
#29175=CARTESIAN_POINT('Ctrl Pts',(-0.00162797270880739,-0.0398438003857508,
-0.0141329395939904));
#29176=CARTESIAN_POINT('Ctrl Pts',(-0.00121263146935118,-0.0398744103312313,
-0.0144143026950736));
#29177=CARTESIAN_POINT('Ctrl Pts',(-0.000754274313859049,-0.0399050202767117,
-0.0145593528689899));
#29178=CARTESIAN_POINT('Ctrl Pts',(-0.000666729093165872,-0.0399108667097833,
-0.0145870571370152));
#29179=CARTESIAN_POINT('Ctrl Pts',(-0.000577695385311776,-0.0399167131428548,
-0.0146099200360221));
#29180=CARTESIAN_POINT('Ctrl Pts',(-0.000487736012541149,-0.0399225595759265,
-0.0146278144571459));
#29181=CARTESIAN_POINT('Ctrl Pts',(-1.52759145852082E-5,-0.0399532646181766,
-0.014721794658393));
#29182=CARTESIAN_POINT('Ctrl Pts',(0.000485825779097723,-0.0399839696604266,
-0.0146751536575047));
#29183=CARTESIAN_POINT('Ctrl Pts',(0.000933184668445214,-0.0400146747026767,
-0.0144951562798254));
#29184=CARTESIAN_POINT('Ctrl Pts',(0.00101697909541043,-0.0400204260389786,
-0.0144614411185153));
#29185=CARTESIAN_POINT('Ctrl Pts',(0.00109890870822176,-0.0400261773752806,
-0.0144231941637545));
#29186=CARTESIAN_POINT('Ctrl Pts',(0.00117848419324155,-0.0400319287115825,
-0.0143806605357932));
#29187=CARTESIAN_POINT('Ctrl Pts',(0.00160317707498042,-0.0400626234863275,
-0.014153659355402));
#29188=CARTESIAN_POINT('Ctrl Pts',(0.0019608573886363,-0.0400933182610726,
-0.0137998630381147));
#29189=CARTESIAN_POINT('Ctrl Pts',(0.00219248251600564,-0.0401240130358175,
-0.0133771111344033));
#29190=CARTESIAN_POINT('Ctrl Pts',(0.00223596002078373,-0.0401297746396245,
-0.0132977579220713));
#29191=CARTESIAN_POINT('Ctrl Pts',(0.00227510586067259,-0.0401355362434315,
-0.0132160760307234));
#29192=CARTESIAN_POINT('Ctrl Pts',(0.0023096961760887,-0.0401412978472384,
-0.0131325682776402));
#29193=CARTESIAN_POINT('Ctrl Pts',(0.00249397506363996,-0.0401719926219835,
-0.0126876831803244));
#29194=CARTESIAN_POINT('Ctrl Pts',(0.00254602571120722,-0.0402026873967285,
-0.0121872878122934));
#29195=CARTESIAN_POINT('Ctrl Pts',(0.00245688259764042,-0.0402333821714736,
-0.0117135461360492));
#29196=CARTESIAN_POINT('Ctrl Pts',(0.00244014987010768,-0.0402391437752805,
-0.0116246218201674));
#29197=CARTESIAN_POINT('Ctrl Pts',(0.00241859117801914,-0.0402449053790875,
-0.0115366450454989));
#29198=CARTESIAN_POINT('Ctrl Pts',(0.00239235234989162,-0.0402506669828944,
-0.0114501465730932));
#29199=CARTESIAN_POINT('Ctrl Pts',(0.002252519006042,-0.040281372025145,
-0.0109891743613927));
#29200=CARTESIAN_POINT('Ctrl Pts',(0.00197516790000548,-0.0403120770673955,
-0.0105692288056267));
#29201=CARTESIAN_POINT('Ctrl Pts',(0.00160553921447455,-0.040342782109646,
-0.0102595433349103));
#29202=CARTESIAN_POINT('Ctrl Pts',(0.00153630436829489,-0.0403485334459475,
-0.0102015364031747));
#29203=CARTESIAN_POINT('Ctrl Pts',(0.0014639518422826,-0.040354284782249,
-0.010147310350429));
#29204=CARTESIAN_POINT('Ctrl Pts',(0.00138892846704934,-0.0403600361185504,
-0.0100971811831661));
#29205=CARTESIAN_POINT('Ctrl Pts',(0.000989636666800498,-0.0403906460640308,
-0.00983038213048244));
#29206=CARTESIAN_POINT('Ctrl Pts',(0.000510458335853878,-0.0404212560095112,
-0.00968176584124858));
#29207=CARTESIAN_POINT('Ctrl Pts',(2.98264480542069E-5,-0.0404518659549916,
-0.0096760312162906));
#29208=CARTESIAN_POINT('Ctrl Pts',(-6.1973198106119E-5,-0.0404577123880632,
-0.00967493591538493));
#29209=CARTESIAN_POINT('Ctrl Pts',(-0.000153787395074284,-0.0404635588211348,
-0.00967890365590639));
#29210=CARTESIAN_POINT('Ctrl Pts',(-0.000245041124596022,-0.0404694052542064,
-0.0096878912998596));
#29211=CARTESIAN_POINT('Ctrl Pts',(-0.000729727742681694,-0.0405004580987112,
-0.00973562842550997));
#29212=CARTESIAN_POINT('Ctrl Pts',(-0.0012004523423602,-0.0405315109432161,
-0.00992929143953727));
#29213=CARTESIAN_POINT('Ctrl Pts',(-0.0015788116380206,-0.040562563787721,
-0.0102374637974072));
#29214=CARTESIAN_POINT('Ctrl Pts',(-0.00164465028722456,-0.0405679673217681,
-0.0102910891529802));
#29215=CARTESIAN_POINT('Ctrl Pts',(-0.00170774550115013,-0.0405733708558151,
-0.0103480648817755));
#29216=CARTESIAN_POINT('Ctrl Pts',(-0.00176776695296642,-0.0405787743898623,
-0.0104080863335918));
#29217=CARTESIAN_POINT('Ctrl Pts',(-0.00249999922097496,-0.0405787743898623,
-0.012173879679554));
#29218=CARTESIAN_POINT('Ctrl Pts',(-0.00249961583479718,-0.0405478495637463,
-0.0116882383417466));
#29219=CARTESIAN_POINT('Ctrl Pts',(-0.00235343949917405,-0.0405169247376302,
-0.0112027367429832));
#29220=CARTESIAN_POINT('Ctrl Pts',(-0.00208585174715449,-0.0404859999115143,
-0.0107977304731294));
#29221=CARTESIAN_POINT('Ctrl Pts',(-0.00199290425717607,-0.0404752580709636,
-0.0106570502068455));
#29222=CARTESIAN_POINT('Ctrl Pts',(-0.00188575583833928,-0.0404645162304129,
-0.0105259359162076));
#29223=CARTESIAN_POINT('Ctrl Pts',(-0.00176672706272141,-0.0404537743898623,
-0.0104070470547035));
#29224=CARTESIAN_POINT('Ctrl Pts',(-0.00143036500450258,-0.0404234191452761,
-0.0100710803781813));
#29225=CARTESIAN_POINT('Ctrl Pts',(-0.000993803849420159,-0.0403930639006899,
-0.0098328104764883));
#29226=CARTESIAN_POINT('Ctrl Pts',(-0.000527580430923165,-0.0403627086561037,
-0.00973215549654663));
#29227=CARTESIAN_POINT('Ctrl Pts',(-0.000353849336270321,-0.0403513972340232,
-0.00969464794297092));
#29228=CARTESIAN_POINT('Ctrl Pts',(-0.000176263431322318,-0.0403400858119428,
-0.00967578493628572));
#29229=CARTESIAN_POINT('Ctrl Pts',(9.66782122917552E-7,-0.0403287743898623,
-0.00967585347349164));
#29230=CARTESIAN_POINT('Ctrl Pts',(0.000478339182571104,-0.0402983068944727,
-0.00967603807954653));
#29231=CARTESIAN_POINT('Ctrl Pts',(0.000957186551135902,-0.0402678393990832,
-0.00981727190682606));
#29232=CARTESIAN_POINT('Ctrl Pts',(0.00135895049920568,-0.0402373719036936,
-0.0100774602011929));
#29233=CARTESIAN_POINT('Ctrl Pts',(0.00150662995922923,-0.0402261727324165,
-0.010173099610854));
#29234=CARTESIAN_POINT('Ctrl Pts',(0.00164403641083569,-0.0402149735611394,
-0.0102843098558379));
#29235=CARTESIAN_POINT('Ctrl Pts',(0.00176809457439739,-0.0402037743898623,
-0.0104084140157523));
#29236=CARTESIAN_POINT('Ctrl Pts',(0.00210553295380404,-0.0401733126282341,
-0.0107459775053031));
#29237=CARTESIAN_POINT('Ctrl Pts',(0.00234432355200967,-0.0401428508666059,
-0.0111843065377002));
#29238=CARTESIAN_POINT('Ctrl Pts',(0.00244455322970797,-0.0401123891049778,
-0.0116522508542449));
#29239=CARTESIAN_POINT('Ctrl Pts',(0.00248142122291065,-0.0401011841999393,
-0.0118243771972382));
#29240=CARTESIAN_POINT('Ctrl Pts',(0.00249999718775118,-0.0400899792949008,
-0.0120002560863263));
#29241=CARTESIAN_POINT('Ctrl Pts',(0.00249999999967931,-0.0400787743898623,
-0.012175813243643));
#29242=CARTESIAN_POINT('Ctrl Pts',(0.00250000764421395,-0.0400483126282342,
-0.0126530846047037));
#29243=CARTESIAN_POINT('Ctrl Pts',(0.0023590242138907,-0.0400178508666063,
-0.0131319048509345));
#29244=CARTESIAN_POINT('Ctrl Pts',(0.0020990883225621,-0.0399873891049782,
-0.0135337296484127));
#29245=CARTESIAN_POINT('Ctrl Pts',(0.00200347477880099,-0.0399761841999396,
-0.013681534911709));
#29246=CARTESIAN_POINT('Ctrl Pts',(0.00189226889350245,-0.0399649792949009,
-0.0138190642417662));
#29247=CARTESIAN_POINT('Ctrl Pts',(0.00176815119222662,-0.0399537743898623,
-0.0139432359167284));
#29248=CARTESIAN_POINT('Ctrl Pts',(0.00143066011324305,-0.0399233068944727,
-0.0142808737567094));
#29249=CARTESIAN_POINT('Ctrl Pts',(0.000992332864294848,-0.0398928393990831,
-0.0145198628226008));
#29250=CARTESIAN_POINT('Ctrl Pts',(0.000524329143107271,-0.0398623719036935,
-0.0146202507480378));
#29251=CARTESIAN_POINT('Ctrl Pts',(0.000352301420944516,-0.0398511727324164,
-0.0146571511087908));
#29252=CARTESIAN_POINT('Ctrl Pts',(0.000176518305235053,-0.0398399735611394,
-0.0146757795891959));
#29253=CARTESIAN_POINT('Ctrl Pts',(1.04686794656891E-6,-0.0398287743898623,
-0.0146758530673716));
#29254=CARTESIAN_POINT('Ctrl Pts',(-0.000474566752473521,-0.0397984191452761,
-0.0146760522292507));
#29255=CARTESIAN_POINT('Ctrl Pts',(-0.000951916780078385,-0.0397680639006899,
-0.0145362050849411));
#29256=CARTESIAN_POINT('Ctrl Pts',(-0.00135292419538027,-0.0397377086561037,
-0.0142781368358337));
#29257=CARTESIAN_POINT('Ctrl Pts',(-0.00150235353432011,-0.0397263972340233,
-0.014181971611965));
#29258=CARTESIAN_POINT('Ctrl Pts',(-0.00164132616302582,-0.0397150858119428,
-0.0140699049910283));
#29259=CARTESIAN_POINT('Ctrl Pts',(-0.00176667039928876,-0.0397037743898623,
-0.0139447161134265));
#29260=CARTESIAN_POINT('Ctrl Pts',(-0.00210935487198405,-0.0396728495637463,
-0.0136024563830445));
#29261=CARTESIAN_POINT('Ctrl Pts',(-0.00235032589488465,-0.0396419247376303,
-0.01315678100991));
#29262=CARTESIAN_POINT('Ctrl Pts',(-0.00244848723592954,-0.0396109999115143,
-0.0126807396653505));
#29263=CARTESIAN_POINT('Ctrl Pts',(-0.00248258390214153,-0.0396002580709636,
-0.0125153851311136));
#29264=CARTESIAN_POINT('Ctrl Pts',(-0.00249986058216984,-0.039589516230413,
-0.0123465960986312));
#29265=CARTESIAN_POINT('Ctrl Pts',(-0.00249999915646903,-0.0395787743898623,
-0.0121779069793664));
#29266=CARTESIAN_POINT('Origin',(0.,-0.0405787743898723,-0.0121758532865581));
#29267=CARTESIAN_POINT('',(0.00257042566803073,-0.0405782384986467,-0.0106271515585321));
#29268=CARTESIAN_POINT('',(0.0007218555435634,-0.0405787743898678,-0.0150877125850593));
#29269=CARTESIAN_POINT('Origin',(1.00006808390063E-14,-0.0405787743898623,
-0.0121758532865681));
#29270=CARTESIAN_POINT('Ctrl Pts',(0.000721855543558197,-0.0405787743898723,
-0.0150877125850536));
#29271=CARTESIAN_POINT('Ctrl Pts',(0.00012268413029149,-0.0405787743898723,
-0.0151791096272557));
#29272=CARTESIAN_POINT('Ctrl Pts',(-0.000503677158141744,-0.0405787743898723,
-0.0150739619320304));
#29273=CARTESIAN_POINT('Ctrl Pts',(-0.00104449598105803,-0.0405787743898723,
-0.0148006456629191));
#29274=CARTESIAN_POINT('Ctrl Pts',(-0.00134936358119689,-0.0405787743898723,
-0.0146465732240318));
#29275=CARTESIAN_POINT('Ctrl Pts',(-0.001626067145542,-0.0405787743898723,
-0.0144398053336723));
#29276=CARTESIAN_POINT('Ctrl Pts',(-0.0018533658809598,-0.0405787743898723,
-0.014182243962393));
#29277=CARTESIAN_POINT('Ctrl Pts',(-0.0019941234239128,-0.0405787743898723,
-0.0140227459092506));
#29278=CARTESIAN_POINT('Ctrl Pts',(-0.00211781727968312,-0.0405787743898723,
-0.0138421912823585));
#29279=CARTESIAN_POINT('Ctrl Pts',(-0.00222177552425318,-0.0405787743898723,
-0.0136368054667619));
#29280=CARTESIAN_POINT('Ctrl Pts',(-0.00231573504664697,-0.0405787743898723,
-0.013451173694893));
#29281=CARTESIAN_POINT('Ctrl Pts',(-0.00238865409568575,-0.0405787743898723,
-0.013253473685689));
#29282=CARTESIAN_POINT('Ctrl Pts',(-0.00243804199053378,-0.0405787743898723,
-0.0130507592809956));
#29283=CARTESIAN_POINT('Ctrl Pts',(-0.00250778716150712,-0.0405787743898723,
-0.0127644876985035));
#29284=CARTESIAN_POINT('Ctrl Pts',(-0.00253129823554409,-0.0405787743898723,
-0.0124667360306207));
#29285=CARTESIAN_POINT('Ctrl Pts',(-0.00250173218769294,-0.0405787743898723,
-0.0121740091469983));
#29286=CARTESIAN_POINT('Ctrl Pts',(-0.00176776695296641,-0.0405787743898723,
-0.0104080863335918));
#29287=CARTESIAN_POINT('Ctrl Pts',(-0.00149473584801468,-0.0405787743898723,
-0.0100673811147438));
#29288=CARTESIAN_POINT('Ctrl Pts',(-0.00112754673188857,-0.0405787743898723,
-0.00980644043751801));
#29289=CARTESIAN_POINT('Ctrl Pts',(-0.000722280104342335,-0.0405787743898723,
-0.00964250969240816));
#29290=CARTESIAN_POINT('Ctrl Pts',(-0.000462635152748786,-0.0405787743898723,
-0.00953748305689057));
#29291=CARTESIAN_POINT('Ctrl Pts',(-0.000187046045747263,-0.0405787743898723,
-0.00947201344856637));
#29292=CARTESIAN_POINT('Ctrl Pts',(9.20188708201852E-5,-0.0405787743898723,
-0.00945044526887669));
#29293=CARTESIAN_POINT('Ctrl Pts',(0.000248532219532483,-0.0405787743898723,
-0.00943834877150833));
#29294=CARTESIAN_POINT('Ctrl Pts',(0.00040854209693118,-0.0405787743898723,
-0.00944044634427772));
#29295=CARTESIAN_POINT('Ctrl Pts',(0.000560837419894266,-0.0405787743898723,
-0.00945634420536109));
#29296=CARTESIAN_POINT('Ctrl Pts',(0.000864786366481517,-0.0405787743898723,
-0.00948807294157746));
#29297=CARTESIAN_POINT('Ctrl Pts',(0.00113113360580538,-0.0405787743898723,
-0.00957065365736988));
#29298=CARTESIAN_POINT('Ctrl Pts',(0.00135440211750958,-0.0405787743898723,
-0.00966712856289749));
#29299=CARTESIAN_POINT('Ctrl Pts',(0.00147242656286442,-0.0405787743898723,
-0.00971812723319204));
#29300=CARTESIAN_POINT('Ctrl Pts',(0.00158170838481421,-0.0405787743898723,
-0.00977423237411966));
#29301=CARTESIAN_POINT('Ctrl Pts',(0.0016894090238867,-0.0405787743898723,
-0.00983801248702863));
#29302=CARTESIAN_POINT('Ctrl Pts',(0.00203095285777748,-0.0405787743898723,
-0.0100402740936126));
#29303=CARTESIAN_POINT('Ctrl Pts',(0.00233296277669372,-0.0405787743898723,
-0.0103094920811301));
#29304=CARTESIAN_POINT('Ctrl Pts',(0.00257120062921594,-0.0405787743898723,
-0.0106266352500323));
#29305=CARTESIAN_POINT('Origin',(0.006,-0.0408432743898723,-0.0121758532865581));
#29306=CARTESIAN_POINT('Ctrl Pts',(0.0066708408081868,-0.0408432743898723,
-0.0135653933579743));
#29307=CARTESIAN_POINT('Ctrl Pts',(0.00644291256165282,-0.0408432743898723,
-0.0136513645485826));
#29308=CARTESIAN_POINT('Ctrl Pts',(0.0061939241669469,-0.0408432743898723,
-0.0136786575412909));
#29309=CARTESIAN_POINT('Ctrl Pts',(0.00595206629017699,-0.0408432743898723,
-0.0136486405340303));
#29310=CARTESIAN_POINT('Ctrl Pts',(0.0057959164633947,-0.0408432743898723,
-0.0136292607621292));
#29311=CARTESIAN_POINT('Ctrl Pts',(0.00564276939617046,-0.0408432743898723,
-0.0135859598764373));
#29312=CARTESIAN_POINT('Ctrl Pts',(0.00550095178366503,-0.0408432743898723,
-0.0135187810726581));
#29313=CARTESIAN_POINT('Ctrl Pts',(0.00542311044837692,-0.0408432743898723,
-0.0134819077415052));
#29314=CARTESIAN_POINT('Ctrl Pts',(0.00534758693333899,-0.0408432743898723,
-0.0134369783461034));
#29315=CARTESIAN_POINT('Ctrl Pts',(0.00527959366954842,-0.0408432743898723,
-0.0133868303201724));
#29316=CARTESIAN_POINT('Ctrl Pts',(0.00518003238464839,-0.0408432743898723,
-0.0133133994886672));
#29317=CARTESIAN_POINT('Ctrl Pts',(0.0051027042655517,-0.0408432743898723,
-0.0132342662983514));
#29318=CARTESIAN_POINT('Ctrl Pts',(0.00504408437945305,-0.0408432743898723,
-0.0131635163957752));
#29319=CARTESIAN_POINT('Ctrl Pts',(0.00500661674994715,-0.0408432743898723,
-0.0131182957153248));
#29320=CARTESIAN_POINT('Ctrl Pts',(0.00497754696327898,-0.0408432743898723,
-0.0130777006059599));
#29321=CARTESIAN_POINT('Ctrl Pts',(0.00495287577896128,-0.0408432743898723,
-0.0130402400194263));
#29322=CARTESIAN_POINT('Ctrl Pts',(0.0048661367091343,-0.0408432743898723,
-0.0129085359070798));
#29323=CARTESIAN_POINT('Ctrl Pts',(0.00480112740676211,-0.0408432743898723,
-0.0127617780100069));
#29324=CARTESIAN_POINT('Ctrl Pts',(0.00476339054481838,-0.0408432743898723,
-0.012608747868102));
#29325=CARTESIAN_POINT('Ctrl Pts',(0.00473186775269151,-0.0408432743898723,
-0.0124809169594376));
#29326=CARTESIAN_POINT('Ctrl Pts',(0.00472093115928062,-0.0408432743898723,
-0.0123552969347836));
#29327=CARTESIAN_POINT('Ctrl Pts',(0.00472819748833167,-0.0408432743898723,
-0.0122359809577845));
#29328=CARTESIAN_POINT('Ctrl Pts',(0.00472941863046114,-0.0408432743898723,
-0.0122159293243933));
#29329=CARTESIAN_POINT('Ctrl Pts',(0.00473115808435559,-0.0408432743898723,
-0.0121959887117323));
#29330=CARTESIAN_POINT('Ctrl Pts',(0.00473339895604038,-0.0408432743898723,
-0.0121761426976128));
#29331=CARTESIAN_POINT('Ctrl Pts',(0.00510586347518963,-0.0408432743898723,
-0.0112817167617477));
#29332=CARTESIAN_POINT('Ctrl Pts',(0.00523985302939051,-0.0408432743898723,
-0.0111149436690097));
#29333=CARTESIAN_POINT('Ctrl Pts',(0.00541836403085339,-0.0408432743898723,
-0.010986190403829));
#29334=CARTESIAN_POINT('Ctrl Pts',(0.00561597474088275,-0.0408432743898723,
-0.0109031332635979));
#29335=CARTESIAN_POINT('Ctrl Pts',(0.0057127184838363,-0.0408432743898723,
-0.0108624712032076));
#29336=CARTESIAN_POINT('Ctrl Pts',(0.00581188031817111,-0.0408432743898723,
-0.010833090617441));
#29337=CARTESIAN_POINT('Ctrl Pts',(0.00591786028704338,-0.0408432743898723,
-0.0108147439575407));
#29338=CARTESIAN_POINT('Ctrl Pts',(0.00602835712854006,-0.0408432743898723,
-0.0107956153618959));
#29339=CARTESIAN_POINT('Ctrl Pts',(0.00615352503003078,-0.0408432743898723,
-0.0107875324977288));
#29340=CARTESIAN_POINT('Ctrl Pts',(0.00628985470781804,-0.0408432743898723,
-0.0108025493456774));
#29341=CARTESIAN_POINT('Ctrl Pts',(0.00640764562415654,-0.0408432743898723,
-0.0108155241308385));
#29342=CARTESIAN_POINT('Ctrl Pts',(0.00653154785488207,-0.0408432743898723,
-0.0108469563098139));
#29343=CARTESIAN_POINT('Ctrl Pts',(0.00664639836621562,-0.0408432743898723,
-0.0108929699340679));
#29344=CARTESIAN_POINT('Ctrl Pts',(0.00684726066682443,-0.0408432743898723,
-0.0109734432582151));
#29345=CARTESIAN_POINT('Ctrl Pts',(0.00703025890384745,-0.0408432743898723,
-0.011098646305903));
#29346=CARTESIAN_POINT('Ctrl Pts',(0.00718006637589825,-0.0408432743898723,
-0.0112550411609207));
#29347=CARTESIAN_POINT('Ctrl Pts',(0.00728593172218851,-0.0408432743898723,
-0.011365561652708));
#29348=CARTESIAN_POINT('Ctrl Pts',(0.00737184727087407,-0.0408432743898723,
-0.0114874543259832));
#29349=CARTESIAN_POINT('Ctrl Pts',(0.00743748127739367,-0.0408432743898723,
-0.0116201260411841));
#29350=CARTESIAN_POINT('Ctrl Pts',(0.00744482695207721,-0.0408432743898723,
-0.0116349744911151));
#29351=CARTESIAN_POINT('Ctrl Pts',(0.00745192010089368,-0.0408432743898723,
-0.0116499769291171));
#29352=CARTESIAN_POINT('Ctrl Pts',(0.0074587645768567,-0.0408432743898723,
-0.0116651389210321));
#29353=CARTESIAN_POINT('Origin',(0.0076,-0.0412787743898723,-0.00457585328655813));
#29354=CARTESIAN_POINT('Origin',(0.008,-0.0412787743898723,-0.00417585328655813));
#29355=CARTESIAN_POINT('',(0.00800000000001,-0.0301787743898623,-0.00817585328656812));
#29356=CARTESIAN_POINT('Origin',(0.0076,-0.0412787743898723,-0.0197758532865581));
#29357=CARTESIAN_POINT('Origin',(0.0076,-0.0301787743898723,-0.0201758532865581));
#29358=CARTESIAN_POINT('',(0.00800000000001,-0.0301787743898623,-0.0197758532865681));
#29359=CARTESIAN_POINT('Origin',(-0.0035,-0.0297787743898723,-0.0121758532865581));
#29360=CARTESIAN_POINT('',(0.00760000000001,-0.0297787743898623,-0.00817585328656812));
#29361=CARTESIAN_POINT('',(-0.01459999999999,-0.0297787743898623,-0.0161758532865681));
#29362=CARTESIAN_POINT('',(-0.00320000000001762,-0.0297787743898547,-0.0121758532865581));
#29363=CARTESIAN_POINT('Origin',(1.00024155624823E-14,-0.0297787743898623,
-0.0121758532865681));
#29364=CARTESIAN_POINT('',(-0.0142000000000176,-0.0297787743898547,-0.0121758532865581));
#29365=CARTESIAN_POINT('Origin',(-0.01249999999999,-0.0297787743898623,
-0.0121758532865681));
#29366=CARTESIAN_POINT('Origin',(-0.015,-0.0301787743898723,-0.0197758532865581));
#29367=CARTESIAN_POINT('',(-0.01459999999999,-0.0297787743898623,-0.0197758532865681));
#29368=CARTESIAN_POINT('Origin',(-0.015,-0.0412787743898723,-0.0201758532865581));
#29369=CARTESIAN_POINT('',(-0.015,-0.0301787743898623,-0.0161758532865681));
#29370=CARTESIAN_POINT('Origin',(-0.0125,-0.0375520664398416,-0.0121758532865581));
#29371=CARTESIAN_POINT('',(-0.0140429999982064,-0.0363035190698315,-0.0121757788889842));
#29372=CARTESIAN_POINT('Ctrl Pts',(-0.014043,-0.0363035228772662,-0.012175853286558));
#29373=CARTESIAN_POINT('Ctrl Pts',(-0.014043,-0.0363035216081401,-0.0121758284873666));
#29374=CARTESIAN_POINT('Ctrl Pts',(-0.0140429999994021,-0.0363035203389952,
-0.0121758036881753));
#29375=CARTESIAN_POINT('Ctrl Pts',(-0.0140429999982064,-0.0363035190698315,
-0.0121757788889841));
#29376=CARTESIAN_POINT('Ctrl Pts',(-0.0140429999982064,-0.0363035190698315,
-0.0121757788889842));
#29377=CARTESIAN_POINT('Ctrl Pts',(-0.0140429995987208,-0.03630309504786,
-0.0121674935888125));
#29378=CARTESIAN_POINT('Ctrl Pts',(-0.0140429325737997,-0.0363026694551463,
-0.0121592185236324));
#29379=CARTESIAN_POINT('Ctrl Pts',(-0.0140426306945938,-0.0363017033307592,
-0.0121405282383409));
#29380=CARTESIAN_POINT('Ctrl Pts',(-0.0140423573365181,-0.0363011621194678,
-0.0121301241024859));
#29381=CARTESIAN_POINT('Ctrl Pts',(-0.0140411875071023,-0.0362994795614532,
-0.0120979868273761));
#29382=CARTESIAN_POINT('Ctrl Pts',(-0.0140399367540347,-0.036298327231832,
-0.0120762699238923));
#29383=CARTESIAN_POINT('Ctrl Pts',(-0.0140299305721976,-0.0362915005031093,
-0.0119493439846875));
#29384=CARTESIAN_POINT('Ctrl Pts',(-0.0140108559444092,-0.0362855032348445,
-0.011845244152624));
#29385=CARTESIAN_POINT('Ctrl Pts',(-0.0139628756321997,-0.0362756526337917,
-0.0116806953806947));
#29386=CARTESIAN_POINT('Ctrl Pts',(-0.0139404098438068,-0.0362718583152341,
-0.0116187118331264));
#29387=CARTESIAN_POINT('Ctrl Pts',(-0.0139013033997271,-0.036266405575857,
-0.0115291598057157));
#29388=CARTESIAN_POINT('Ctrl Pts',(-0.0138876538029265,-0.0362646578194073,
-0.0115003676365055));
#29389=CARTESIAN_POINT('Ctrl Pts',(-0.0138691932555083,-0.036262497376662,
-0.0114643527577709));
#29390=CARTESIAN_POINT('Ctrl Pts',(-0.0138652005395636,-0.03626204110314,
-0.0114567214023763));
#29391=CARTESIAN_POINT('Ctrl Pts',(-0.0138586660477047,-0.0362613122907672,
-0.011444482483014));
#29392=CARTESIAN_POINT('Ctrl Pts',(-0.0138561642881782,-0.0362610373492196,
-0.0114398538935162));
#29393=CARTESIAN_POINT('Ctrl Pts',(-0.0138512935016634,-0.0362605100001696,
-0.0114309514482718));
#29394=CARTESIAN_POINT('Ctrl Pts',(-0.0138489277927363,-0.0362602574052702,
-0.0114266759466823));
#29395=CARTESIAN_POINT('Ctrl Pts',(-0.0138430736484742,-0.0362596407828723,
-0.0114162134897503));
#29396=CARTESIAN_POINT('Ctrl Pts',(-0.0138395626813316,-0.0362592781736722,
-0.0114100391624586));
#29397=CARTESIAN_POINT('Ctrl Pts',(-0.0138273285772317,-0.0362580383913607,
-0.0113888660601725));
#29398=CARTESIAN_POINT('Ctrl Pts',(-0.0138183948907351,-0.0362571737259045,
-0.0113739898283539));
#29399=CARTESIAN_POINT('Ctrl Pts',(-0.0137322308887414,-0.036249174949193,
-0.0112358453145593));
#29400=CARTESIAN_POINT('Ctrl Pts',(-0.0136381774313634,-0.0362428638621241,
-0.0111239166007904));
#29401=CARTESIAN_POINT('Ctrl Pts',(-0.0135017800160587,-0.0362342750410312,
-0.0110016708600523));
#29402=CARTESIAN_POINT('Ctrl Pts',(-0.0134728226373155,-0.0362324821888421,
-0.0109775697401679));
#29403=CARTESIAN_POINT('Ctrl Pts',(-0.0134218449267673,-0.0362293496275276,
-0.0109382078555016));
#29404=CARTESIAN_POINT('Ctrl Pts',(-0.0134002556650593,-0.0362280298575219,
-0.0109224164460669));
#29405=CARTESIAN_POINT('Ctrl Pts',(-0.0133687119399263,-0.0362261055605039,
-0.0109005793397179));
#29406=CARTESIAN_POINT('Ctrl Pts',(-0.0133590819284627,-0.036225518625291,
-0.0108940723751991));
#29407=CARTESIAN_POINT('Ctrl Pts',(-0.0133421521230947,-0.0362244872862137,
-0.0108829094570772));
#29408=CARTESIAN_POINT('Ctrl Pts',(-0.0133348848759541,-0.0362240447375029,
-0.0108782049580479));
#29409=CARTESIAN_POINT('Ctrl Pts',(-0.0133197761820495,-0.0362231248393869,
-0.0108686037037348));
#29410=CARTESIAN_POINT('Ctrl Pts',(-0.0133119295597613,-0.0362226471858507,
-0.0108637157764484));
#29411=CARTESIAN_POINT('Ctrl Pts',(-0.0132915687334052,-0.0362214077789512,
-0.0108512848914695));
#29412=CARTESIAN_POINT('Ctrl Pts',(-0.0132789906524162,-0.0362206421499758,
-0.0108438487683383));
#29413=CARTESIAN_POINT('Ctrl Pts',(-0.0132261471095531,-0.0362174248421312,
-0.0108136123180992));
#29414=CARTESIAN_POINT('Ctrl Pts',(-0.013184974933425,-0.0362149154202119,
-0.0107924521084515));
#29415=CARTESIAN_POINT('Ctrl Pts',(-0.0130495141989045,-0.0362066586971812,
-0.0107303637406961));
#29416=CARTESIAN_POINT('Ctrl Pts',(-0.0129520745200486,-0.0362006991898911,
-0.0106969919173001));
#29417=CARTESIAN_POINT('Ctrl Pts',(-0.0127936055887318,-0.036191375902033,
-0.0106598556981046));
#29418=CARTESIAN_POINT('Ctrl Pts',(-0.0127344017609904,-0.0361879763827394,
-0.0106495800797282));
#29419=CARTESIAN_POINT('Ctrl Pts',(-0.0126611378304009,-0.036183982981313,
-0.0106412291701596));
#29420=CARTESIAN_POINT('Ctrl Pts',(-0.0126475094785747,-0.0361832492079286,
-0.010639859289788));
#29421=CARTESIAN_POINT('Ctrl Pts',(-0.0126276017009878,-0.0361821923412473,
-0.0106381256374585));
#29422=CARTESIAN_POINT('Ctrl Pts',(-0.012621335773148,-0.0361818618585971,
-0.0106376185353679));
#29423=CARTESIAN_POINT('Ctrl Pts',(-0.0126102740648317,-0.0361812824627403,
-0.0106367913223943));
#29424=CARTESIAN_POINT('Ctrl Pts',(-0.0126054796538431,-0.0361810326829888,
-0.0106364553056877));
#29425=CARTESIAN_POINT('Ctrl Pts',(-0.0125950543010995,-0.036180492503163,
-0.0106357735795657));
#29426=CARTESIAN_POINT('Ctrl Pts',(-0.01258942297963,-0.0361802025727367,
-0.0106354363440624));
#29427=CARTESIAN_POINT('Ctrl Pts',(-0.0125736493454721,-0.0361793953341253,
-0.0106345785194115));
#29428=CARTESIAN_POINT('Ctrl Pts',(-0.012563503387812,-0.0361788817364137,
-0.0106341271552065));
#29429=CARTESIAN_POINT('Ctrl Pts',(-0.0124975830130454,-0.0361755771902464,
-0.0106318464134615));
#29430=CARTESIAN_POINT('Ctrl Pts',(-0.0124417436970142,-0.03617292787673,
-0.0106329435746703));
#29431=CARTESIAN_POINT('Ctrl Pts',(-0.0123603292422337,-0.0361691335567524,
-0.010638970749754));
#29432=CARTESIAN_POINT('Ctrl Pts',(-0.0123346277314895,-0.0361679459048419,
-0.010641523495776));
#29433=CARTESIAN_POINT('Ctrl Pts',(-0.0122451012455231,-0.0361638121181602,
-0.0106526912869685));
#29434=CARTESIAN_POINT('Ctrl Pts',(-0.0121817623607875,-0.0361608904467523,
-0.0106646549167043));
#29435=CARTESIAN_POINT('Ctrl Pts',(-0.012076874194689,-0.0361558565449464,
-0.0106913549392201));
#29436=CARTESIAN_POINT('Ctrl Pts',(-0.0120348730263031,-0.0361537867317166,
-0.0107039744334159));
#29437=CARTESIAN_POINT('Ctrl Pts',(-0.0119652722616709,-0.0361502203473588,
-0.0107281633143499));
#29438=CARTESIAN_POINT('Ctrl Pts',(-0.0119373682843611,-0.0361487525382031,
-0.0107387779869717));
#29439=CARTESIAN_POINT('Ctrl Pts',(-0.0118986011461219,-0.036146651323729,
-0.010754827218869));
#29440=CARTESIAN_POINT('Ctrl Pts',(-0.0118874666740248,-0.0361460405059185,
-0.0107595911002697));
#29441=CARTESIAN_POINT('Ctrl Pts',(-0.0118684049991676,-0.0361449816844189,
-0.0107680134675328));
#29442=CARTESIAN_POINT('Ctrl Pts',(-0.0118604505613438,-0.0361445358540261,
-0.0107716091081905));
#29443=CARTESIAN_POINT('Ctrl Pts',(-0.0118443022031949,-0.0361436224505098,
-0.0107790743108959));
#29444=CARTESIAN_POINT('Ctrl Pts',(-0.0118361110137875,-0.0361431547138178,
-0.0107829489406442));
#29445=CARTESIAN_POINT('Ctrl Pts',(-0.011815539604574,-0.0361419686657032,
-0.010792902390383));
#29446=CARTESIAN_POINT('Ctrl Pts',(-0.011803206049612,-0.0361412470777422,
-0.0107990753857635));
#29447=CARTESIAN_POINT('Ctrl Pts',(-0.0117562952369704,-0.0361384613876635,
-0.0108233462496241));
#29448=CARTESIAN_POINT('Ctrl Pts',(-0.0117223285073193,-0.0361363572825881,
-0.0108425870932123));
#29449=CARTESIAN_POINT('Ctrl Pts',(-0.0115868358228125,-0.0361276040364828,
-0.0109262787436451));
#29450=CARTESIAN_POINT('Ctrl Pts',(-0.0114922853091864,-0.0361205972335303,
-0.0110012000843454));
#29451=CARTESIAN_POINT('Ctrl Pts',(-0.0113702319632128,-0.0361107339349849,
-0.0111235963987869));
#29452=CARTESIAN_POINT('Ctrl Pts',(-0.0113349883521476,-0.0361077717449535,
-0.0111627545188793));
#29453=CARTESIAN_POINT('Ctrl Pts',(-0.0112937047977956,-0.0361042303693944,
-0.0112136337190421));
#29454=CARTESIAN_POINT('Ctrl Pts',(-0.0112857213799507,-0.036103541949859,
-0.0112237282605686));
#29455=CARTESIAN_POINT('Ctrl Pts',(-0.0112741240199205,-0.0361025380222728,
-0.0112387755763679));
#29456=CARTESIAN_POINT('Ctrl Pts',(-0.011270411985179,-0.036102216085183,
-0.0112436516614767));
#29457=CARTESIAN_POINT('Ctrl Pts',(-0.011264124086186,-0.0361016699009137,
-0.0112520142778883));
#29458=CARTESIAN_POINT('Ctrl Pts',(-0.0112615337433139,-0.0361014446541618,
-0.0112554897058278));
#29459=CARTESIAN_POINT('Ctrl Pts',(-0.0112556520156969,-0.036100932670152,
-0.0112634509371026));
#29460=CARTESIAN_POINT('Ctrl Pts',(-0.0112523702214137,-0.0361006465946965,
-0.0112679436595548));
#29461=CARTESIAN_POINT('Ctrl Pts',(-0.0112433780333029,-0.0360998613178757,
-0.011280394648733));
#29462=CARTESIAN_POINT('Ctrl Pts',(-0.0112377189156356,-0.0360993655033892,
-0.0112883898153702));
#29463=CARTESIAN_POINT('Ctrl Pts',(-0.0112056838884276,-0.0360965461215234,
-0.0113345751350492));
#29464=CARTESIAN_POINT('Ctrl Pts',(-0.0111809635622188,-0.0360943198979953,
-0.0113738890186394));
#29465=CARTESIAN_POINT('Ctrl Pts',(-0.0111186096703849,-0.0360883944281096,
-0.0114837583639859));
#29466=CARTESIAN_POINT('Ctrl Pts',(-0.011084624935768,-0.0360847953911461,
-0.0115562171575177));
#29467=CARTESIAN_POINT('Ctrl Pts',(-0.0110290236848174,-0.0360775554291241,
-0.0117035290877667));
#29468=CARTESIAN_POINT('Ctrl Pts',(-0.0110071517273209,-0.0360739282113978,
-0.0117780292647345));
#29469=CARTESIAN_POINT('Ctrl Pts',(-0.0109866243092998,-0.0360690960564971,
-0.0118742291234214));
#29470=CARTESIAN_POINT('Ctrl Pts',(-0.0109826895721706,-0.0360680604689365,
-0.0118946911793152));
#29471=CARTESIAN_POINT('Ctrl Pts',(-0.0109773892129962,-0.03606648090869,
-0.0119256201905137));
#29472=CARTESIAN_POINT('Ctrl Pts',(-0.0109757145858098,-0.0360659467598764,
-0.0119360321449306));
#29473=CARTESIAN_POINT('Ctrl Pts',(-0.0109728790368387,-0.036064974501252,
-0.0119548933625149));
#29474=CARTESIAN_POINT('Ctrl Pts',(-0.0109716811795748,-0.0360645375862603,
-0.0119633366909382));
#29475=CARTESIAN_POINT('Ctrl Pts',(-0.0109692547598527,-0.0360635927634442,
-0.011981522561878));
#29476=CARTESIAN_POINT('Ctrl Pts',(-0.0109680490903508,-0.0360630841489514,
-0.0119912677367114));
#29477=CARTESIAN_POINT('Ctrl Pts',(-0.0109650285093156,-0.0360616952299219,
-0.0120177549009252));
#29478=CARTESIAN_POINT('Ctrl Pts',(-0.0109633945624542,-0.0360608092650984,
-0.0120345158333276));
#29479=CARTESIAN_POINT('Ctrl Pts',(-0.0109545266090645,-0.0360549735842397,
-0.0121440157010463));
#29480=CARTESIAN_POINT('Ctrl Pts',(-0.0109554182214037,-0.0360497672504841,
-0.0122372073786588));
#29481=CARTESIAN_POINT('Ctrl Pts',(-0.0109713658684127,-0.0360406147123997,
-0.0123963155300473));
#29482=CARTESIAN_POINT('Ctrl Pts',(-0.0109823622024224,-0.0360367391193339,
-0.0124623868104888));
#29483=CARTESIAN_POINT('Ctrl Pts',(-0.0110091177740337,-0.0360300702925261,
-0.0125766866408892));
#29484=CARTESIAN_POINT('Ctrl Pts',(-0.011023029248533,-0.0360272500713398,
-0.0126252478299691));
#29485=CARTESIAN_POINT('Ctrl Pts',(-0.0110424454972302,-0.0360240207758172,
-0.0126822911458022));
#29486=CARTESIAN_POINT('Ctrl Pts',(-0.0110456811354356,-0.0360235016189537,
-0.0126915092606584));
#29487=CARTESIAN_POINT('Ctrl Pts',(-0.0110508756971738,-0.0360226977427472,
-0.0127058702940551));
#29488=CARTESIAN_POINT('Ctrl Pts',(-0.0110527749018212,-0.0360224096804733,
-0.0127110343683717));
#29489=CARTESIAN_POINT('Ctrl Pts',(-0.0110563954798538,-0.0360218715075487,
-0.0127207187596324));
#29490=CARTESIAN_POINT('Ctrl Pts',(-0.01105811048303,-0.0360216210530846,
-0.0127252411418428));
#29491=CARTESIAN_POINT('Ctrl Pts',(-0.0110621502130185,-0.0360210412683744,
-0.0127357444931532));
#29492=CARTESIAN_POINT('Ctrl Pts',(-0.0110644910138327,-0.03602071289796,
-0.0127417191068715));
#29493=CARTESIAN_POINT('Ctrl Pts',(-0.0110721430617942,-0.0360196629484713,
-0.0127608969534907));
#29494=CARTESIAN_POINT('Ctrl Pts',(-0.0110775998570417,-0.0360189495545451,
-0.0127740417088676));
#29495=CARTESIAN_POINT('Ctrl Pts',(-0.0111138261826433,-0.0360144216590649,
-0.0128580066357587));
#29496=CARTESIAN_POINT('Ctrl Pts',(-0.011149696181361,-0.0360108577377136,
-0.0129265149499834));
#29497=CARTESIAN_POINT('Ctrl Pts',(-0.0112271598202884,-0.0360041510072435,
-0.0130507917643758));
#29498=CARTESIAN_POINT('Ctrl Pts',(-0.0112676818787368,-0.0360010098393769,
-0.0131069984197846));
#29499=CARTESIAN_POINT('Ctrl Pts',(-0.0113500409910983,-0.0359949745492503,
-0.0132064009933315));
#29500=CARTESIAN_POINT('Ctrl Pts',(-0.0113908911369384,-0.0359921099933848,
-0.0132502418920114));
#29501=CARTESIAN_POINT('Ctrl Pts',(-0.0114452528738829,-0.0359883753994694,
-0.0133021711261851));
#29502=CARTESIAN_POINT('Ctrl Pts',(-0.0114564795577272,-0.0359876081218057,
-0.0133125803607398));
#29503=CARTESIAN_POINT('Ctrl Pts',(-0.01147484010386,-0.0359863586370829,
-0.0133291027776311));
#29504=CARTESIAN_POINT('Ctrl Pts',(-0.0114818782892177,-0.0359858809038878,
-0.013335320999878));
#29505=CARTESIAN_POINT('Ctrl Pts',(-0.0114954693582739,-0.0359849605092637,
-0.0133471095137818));
#29506=CARTESIAN_POINT('Ctrl Pts',(-0.0115020129210706,-0.0359845183011864,
-0.0133526900408555));
#29507=CARTESIAN_POINT('Ctrl Pts',(-0.0115170844901004,-0.0359835017207827,
-0.0133653273803864));
#29508=CARTESIAN_POINT('Ctrl Pts',(-0.0115256423996949,-0.0359829258838647,
-0.0133723476566219));
#29509=CARTESIAN_POINT('Ctrl Pts',(-0.0115487225954577,-0.0359813762900012,
-0.0133908691113019));
#29510=CARTESIAN_POINT('Ctrl Pts',(-0.0115633774001219,-0.0359803958916534,
-0.0134022016138494));
#29511=CARTESIAN_POINT('Ctrl Pts',(-0.0116750923253533,-0.0359729465043413,
-0.0134854196959764));
#29512=CARTESIAN_POINT('Ctrl Pts',(-0.0117800754417224,-0.0359660328372556,
-0.0135459396171147));
#29513=CARTESIAN_POINT('Ctrl Pts',(-0.0119435297002618,-0.0359558018743863,
-0.0136161505507782));
#29514=CARTESIAN_POINT('Ctrl Pts',(-0.0119972577903227,-0.0359525246206751,
-0.0136357732434587));
#29515=CARTESIAN_POINT('Ctrl Pts',(-0.01208002868533,-0.0359477114662054,
-0.0136608899638922));
#29516=CARTESIAN_POINT('Ctrl Pts',(-0.0121083436564838,-0.0359461056270923,
-0.0136686075730028));
#29517=CARTESIAN_POINT('Ctrl Pts',(-0.0121449907778423,-0.0359440940928235,
-0.0136774815309303));
#29518=CARTESIAN_POINT('Ctrl Pts',(-0.012153134478864,-0.0359436512919703,
-0.013679383548484));
#29519=CARTESIAN_POINT('Ctrl Pts',(-0.0121663586259715,-0.0359429395053464,
-0.0136823589748054));
#29520=CARTESIAN_POINT('Ctrl Pts',(-0.0121714296287183,-0.0359426682819566,
-0.0136834730887209));
#29521=CARTESIAN_POINT('Ctrl Pts',(-0.0121812992090917,-0.0359421438836818,
-0.0136855893014541));
#29522=CARTESIAN_POINT('Ctrl Pts',(-0.0121860970720809,-0.0359418905632593,
-0.0136865941581665));
#29523=CARTESIAN_POINT('Ctrl Pts',(-0.0121968466705296,-0.0359413264305017,
-0.0136887921168352));
#29524=CARTESIAN_POINT('Ctrl Pts',(-0.0122028008832575,-0.0359410163031011,
-0.0136899730086087));
#29525=CARTESIAN_POINT('Ctrl Pts',(-0.0122235754086168,-0.0359399419415139,
-0.0136939659268531));
#29526=CARTESIAN_POINT('Ctrl Pts',(-0.0122384302894439,-0.0359391873207996,
-0.013696595822847));
#29527=CARTESIAN_POINT('Ctrl Pts',(-0.0123998461531614,-0.0359311117314028,
-0.0137227374729462));
#29528=CARTESIAN_POINT('Ctrl Pts',(-0.0125490438585983,-0.035924687387436,
-0.0137252042013086));
#29529=CARTESIAN_POINT('Ctrl Pts',(-0.0127338478242501,-0.0359159540341034,
-0.013701499497371));
#29530=CARTESIAN_POINT('Ctrl Pts',(-0.0127711927113669,-0.035914153245928,
-0.0136953056371316));
#29531=CARTESIAN_POINT('Ctrl Pts',(-0.0128345677915181,-0.0359110081064292,
-0.0136823836313994));
#29532=CARTESIAN_POINT('Ctrl Pts',(-0.0128607194264732,-0.0359096839505254,
-0.0136763367669058));
#29533=CARTESIAN_POINT('Ctrl Pts',(-0.0128979612624479,-0.0359077545917146,
-0.0136666957224692));
#29534=CARTESIAN_POINT('Ctrl Pts',(-0.0129091898275224,-0.0359071671388194,
-0.0136636530078299));
#29535=CARTESIAN_POINT('Ctrl Pts',(-0.0129287096730245,-0.0359061354412712,
-0.0136581258369899));
#29536=CARTESIAN_POINT('Ctrl Pts',(-0.0129370165256779,-0.03590569306243,
-0.0136556980249516));
#29537=CARTESIAN_POINT('Ctrl Pts',(-0.0129530712650107,-0.0359048314494076,
-0.013650858800963));
#29538=CARTESIAN_POINT('Ctrl Pts',(-0.012960821430074,-0.0359044125073906,
-0.0136484558958556));
#29539=CARTESIAN_POINT('Ctrl Pts',(-0.0129814569729196,-0.0359032888339924,
-0.0136418790820071));
#29540=CARTESIAN_POINT('Ctrl Pts',(-0.0129943067553862,-0.0359025805331877,
-0.0136375965148469));
#29541=CARTESIAN_POINT('Ctrl Pts',(-0.0130421280175331,-0.0358999116794568,
-0.0136209560098568));
#29542=CARTESIAN_POINT('Ctrl Pts',(-0.0130767046633142,-0.0358979153612362,
-0.0136075083022656));
#29543=CARTESIAN_POINT('Ctrl Pts',(-0.0132230101712836,-0.0358891796574392,
-0.0135444459813325));
#29544=CARTESIAN_POINT('Ctrl Pts',(-0.013329103801223,-0.0358820586361552,
-0.0134828994582018));
#29545=CARTESIAN_POINT('Ctrl Pts',(-0.013469156271715,-0.0358720619017414,
-0.0133776814048846));
#29546=CARTESIAN_POINT('Ctrl Pts',(-0.0135098426280364,-0.0358690807626917,
-0.0133437032170579));
#29547=CARTESIAN_POINT('Ctrl Pts',(-0.0135581741855435,-0.0358655192881218,
-0.013298921892953));
#29548=CARTESIAN_POINT('Ctrl Pts',(-0.013567534863224,-0.0358648285682008,
-0.0132900278863636));
#29549=CARTESIAN_POINT('Ctrl Pts',(-0.0135811805094935,-0.0358638217688148,
-0.0132767326623448));
#29550=CARTESIAN_POINT('Ctrl Pts',(-0.0135855523902188,-0.0358634992208278,
-0.013272421891237));
#29551=CARTESIAN_POINT('Ctrl Pts',(-0.0135929690097306,-0.0358629522602076,
-0.01326502111551));
#29552=CARTESIAN_POINT('Ctrl Pts',(-0.0135960265954076,-0.0358627268422441,
-0.0132619442217293));
#29553=CARTESIAN_POINT('Ctrl Pts',(-0.0136029734890203,-0.0358622148854447,
-0.013254894246076));
#29554=CARTESIAN_POINT('Ctrl Pts',(-0.0136068543304453,-0.0358619290044352,
-0.0132509130071594));
#29555=CARTESIAN_POINT('Ctrl Pts',(-0.0136175014635884,-0.0358611447291482,
-0.0132398716620225));
#29556=CARTESIAN_POINT('Ctrl Pts',(-0.0136242223966772,-0.0358606497083555,
-0.0132327679645763));
#29557=CARTESIAN_POINT('Ctrl Pts',(-0.0136622344212292,-0.0358578469754445,
-0.0131918182392619));
#29558=CARTESIAN_POINT('Ctrl Pts',(-0.0136920664185269,-0.0358556352636389,
-0.0131566447847472));
#29559=CARTESIAN_POINT('Ctrl Pts',(-0.0137693193746737,-0.0358497125445119,
-0.0130568173425352));
#29560=CARTESIAN_POINT('Ctrl Pts',(-0.0138133489278706,-0.035846103934367,
-0.0129897235680702));
#29561=CARTESIAN_POINT('Ctrl Pts',(-0.0138929012330122,-0.035838514677895,
-0.0128450976560723));
#29562=CARTESIAN_POINT('Ctrl Pts',(-0.013927616219135,-0.0358345345281592,
-0.0127674373678192));
#29563=CARTESIAN_POINT('Ctrl Pts',(-0.0139612583895272,-0.0358295068755572,
-0.0126716835632191));
#29564=CARTESIAN_POINT('Ctrl Pts',(-0.0139665002655861,-0.0358286779049506,
-0.0126559581588717));
#29565=CARTESIAN_POINT('Ctrl Pts',(-0.0139743956968318,-0.0358273523746311,
-0.0126309353962905));
#29566=CARTESIAN_POINT('Ctrl Pts',(-0.013977217030481,-0.0358268613558079,
-0.0126216920878426));
#29567=CARTESIAN_POINT('Ctrl Pts',(-0.0139823682783781,-0.0358259309073835,
-0.012604229594541));
#29568=CARTESIAN_POINT('Ctrl Pts',(-0.0139847171341991,-0.035825492120375,
-0.0125960163519055));
#29569=CARTESIAN_POINT('Ctrl Pts',(-0.0139898706629757,-0.0358244954699947,
-0.0125774130229305));
#29570=CARTESIAN_POINT('Ctrl Pts',(-0.0139926350580568,-0.03582393631605,
-0.0125670123204707));
#29571=CARTESIAN_POINT('Ctrl Pts',(-0.0140005286689846,-0.0358222635479209,
-0.0125360107526621));
#29572=CARTESIAN_POINT('Ctrl Pts',(-0.0140053416275327,-0.0358211398215695,
-0.0125153326093378));
#29573=CARTESIAN_POINT('Ctrl Pts',(-0.0140318429248073,-0.0358142675351953,
-0.012389795869212));
#29574=CARTESIAN_POINT('Ctrl Pts',(-0.014042991191137,-0.0358081827035411,
-0.0122830263609671));
#29575=CARTESIAN_POINT('Ctrl Pts',(-0.014043,-0.035802018678757,-0.012175853286457));
#29576=CARTESIAN_POINT('Ctrl Pts',(-0.014043,-0.0359172995678105,-0.0121758532865631));
#29577=CARTESIAN_POINT('Ctrl Pts',(-0.014043,-0.0359173084265614,-0.0121760097131553));
#29578=CARTESIAN_POINT('Ctrl Pts',(-0.0140429999762123,-0.0359173172857548,
-0.0121761661401342));
#29579=CARTESIAN_POINT('Ctrl Pts',(-0.0140429684641662,-0.0359231855911133,
-0.0122797780343122));
#29580=CARTESIAN_POINT('Ctrl Pts',(-0.0140325327356852,-0.0359292371515285,
-0.0123829630213215));
#29581=CARTESIAN_POINT('Ctrl Pts',(-0.0140045001279798,-0.0359371137793574,
-0.0125203535658078));
#29582=CARTESIAN_POINT('Ctrl Pts',(-0.0139958629864661,-0.0359391439549073,
-0.0125561102895848));
#29583=CARTESIAN_POINT('Ctrl Pts',(-0.0139834355650421,-0.0359416130535868,
-0.0126005360473383));
#29584=CARTESIAN_POINT('Ctrl Pts',(-0.0139808333466751,-0.0359421097241874,
-0.0126095226661828));
#29585=CARTESIAN_POINT('Ctrl Pts',(-0.0139765932965655,-0.0359428872444756,
-0.0126236821215912));
#29586=CARTESIAN_POINT('Ctrl Pts',(-0.013975009681435,-0.0359431710880598,
-0.0126288708032211));
#29587=CARTESIAN_POINT('Ctrl Pts',(-0.0139719495018691,-0.0359437072071874,
-0.0126387112355998));
#29588=CARTESIAN_POINT('Ctrl Pts',(-0.0139704782037362,-0.0359439597641907,
-0.0126433644304188));
#29589=CARTESIAN_POINT('Ctrl Pts',(-0.0139669203884198,-0.0359445583993516,
-0.0126544335726152));
#29590=CARTESIAN_POINT('Ctrl Pts',(-0.0139648138017627,-0.0359449033124146,
-0.012660843024175));
#29591=CARTESIAN_POINT('Ctrl Pts',(-0.0139574804935722,-0.0359460727355704,
-0.0126826714654573));
#29592=CARTESIAN_POINT('Ctrl Pts',(-0.0139520516555066,-0.0359468861625328,
-0.0126980219231832));
#29593=CARTESIAN_POINT('Ctrl Pts',(-0.0139380598086627,-0.0359488659028139,
-0.0127356779987292));
#29594=CARTESIAN_POINT('Ctrl Pts',(-0.0139292196291492,-0.0359500192383533,
-0.0127578765402717));
#29595=CARTESIAN_POINT('Ctrl Pts',(-0.0138881927526948,-0.0359550051373991,
-0.0128543200874838));
#29596=CARTESIAN_POINT('Ctrl Pts',(-0.0138507088334025,-0.0359586598786273,
-0.0129261754747037));
#29597=CARTESIAN_POINT('Ctrl Pts',(-0.0137568784338933,-0.0359667549029487,
-0.0130760183253592));
#29598=CARTESIAN_POINT('Ctrl Pts',(-0.013698538097385,-0.035971206151278,
-0.0131523492646557));
#29599=CARTESIAN_POINT('Ctrl Pts',(-0.0136221214083504,-0.0359767804573778,
-0.0132350858910033));
#29600=CARTESIAN_POINT('Ctrl Pts',(-0.0136105447111052,-0.0359776184010784,
-0.0132472171753907));
#29601=CARTESIAN_POINT('Ctrl Pts',(-0.0135918779662547,-0.0359789606820361,
-0.0132661504726461));
#29602=CARTESIAN_POINT('Ctrl Pts',(-0.013584916547098,-0.0359794593730415,
-0.0132730777518259));
#29603=CARTESIAN_POINT('Ctrl Pts',(-0.013571767802077,-0.0359803980496948,
-0.0132859145341878));
#29604=CARTESIAN_POINT('Ctrl Pts',(-0.0135655965113048,-0.0359808373052295,
-0.0132918399648914));
#29605=CARTESIAN_POINT('Ctrl Pts',(-0.0135516589585818,-0.0359818265948423,
-0.0133050012402238));
#29606=CARTESIAN_POINT('Ctrl Pts',(-0.0135438667168005,-0.0359823778180092,
-0.0133122088367204));
#29607=CARTESIAN_POINT('Ctrl Pts',(-0.0135203697653379,-0.0359840347598457,
-0.0133334972003947));
#29608=CARTESIAN_POINT('Ctrl Pts',(-0.0135044504946735,-0.0359851505275389,
-0.0133473365486772));
#29609=CARTESIAN_POINT('Ctrl Pts',(-0.0134272610448144,-0.0359905305136053,
-0.0134117106047961));
#29610=CARTESIAN_POINT('Ctrl Pts',(-0.0133624404701795,-0.0359949690584087,
-0.0134577854510251));
#29611=CARTESIAN_POINT('Ctrl Pts',(-0.0132223108652746,-0.0360043012555447,
-0.013541935631443));
#29612=CARTESIAN_POINT('Ctrl Pts',(-0.0131468377728911,-0.0360091907997271,
-0.0135792473344017));
#29613=CARTESIAN_POINT('Ctrl Pts',(-0.0130310415736704,-0.0360162145157066,
-0.0136251583234202));
#29614=CARTESIAN_POINT('Ctrl Pts',(-0.0129928049128773,-0.0360184595105425,
-0.0136386020881521));
#29615=CARTESIAN_POINT('Ctrl Pts',(-0.0129449067758753,-0.0360211441686762,
-0.0136533508679007));
#29616=CARTESIAN_POINT('Ctrl Pts',(-0.0129357063838397,-0.0360216541102725,
-0.0136560901251581));
#29617=CARTESIAN_POINT('Ctrl Pts',(-0.012921219468802,-0.0360224474124532,
-0.0136602565775855));
#29618=CARTESIAN_POINT('Ctrl Pts',(-0.0129159500376674,-0.0360227339724926,
-0.0136617417545478));
#29619=CARTESIAN_POINT('Ctrl Pts',(-0.0129059823901048,-0.0360232721173483,
-0.0136644939333971));
#29620=CARTESIAN_POINT('Ctrl Pts',(-0.0129012859861638,-0.0360235240205948,
-0.0136657667854144));
#29621=CARTESIAN_POINT('Ctrl Pts',(-0.0128901669822468,-0.0360241166336277,
-0.0136687239476847));
#29622=CARTESIAN_POINT('Ctrl Pts',(-0.0128837393290513,-0.036024456247394,
-0.0136703890724609));
#29623=CARTESIAN_POINT('Ctrl Pts',(-0.0128621621749092,-0.0360255869958932,
-0.013675830392529));
#29624=CARTESIAN_POINT('Ctrl Pts',(-0.0128469657106298,-0.0360263680332772,
-0.0136794182470108));
#29625=CARTESIAN_POINT('Ctrl Pts',(-0.0128096772733231,-0.0360282528572942,
-0.0136876265062317));
#29626=CARTESIAN_POINT('Ctrl Pts',(-0.0127875329909992,-0.0360293452530651,
-0.0136919941579886));
#29627=CARTESIAN_POINT('Ctrl Pts',(-0.0126939422214461,-0.0360338783876603,
-0.0137083292136836));
#29628=CARTESIAN_POINT('Ctrl Pts',(-0.0126217919625651,-0.0360371722565894,
-0.0137157441696818));
#29629=CARTESIAN_POINT('Ctrl Pts',(-0.0124507582954497,-0.0360449942503845,
-0.0137212209970137));
#29630=CARTESIAN_POINT('Ctrl Pts',(-0.012352061981371,-0.0360495310743024,
-0.0137149108726152));
#29631=CARTESIAN_POINT('Ctrl Pts',(-0.0122331556746266,-0.0360554375865097,
-0.0136957602466473));
#29632=CARTESIAN_POINT('Ctrl Pts',(-0.012211736147531,-0.0360565184461448,
-0.013691843706578));
#29633=CARTESIAN_POINT('Ctrl Pts',(-0.0121798698374775,-0.0360581547263099,
-0.0136853172227601));
#29634=CARTESIAN_POINT('Ctrl Pts',(-0.0121693554150916,-0.0360586992507125,
-0.0136830489760829));
#29635=CARTESIAN_POINT('Ctrl Pts',(-0.0121504996779944,-0.0360596844194159,
-0.0136787744796693));
#29636=CARTESIAN_POINT('Ctrl Pts',(-0.0121421496976041,-0.0360601237580958,
-0.0136768082308897));
#29637=CARTESIAN_POINT('Ctrl Pts',(-0.0121243464727108,-0.0360610672182272,
-0.0136724589341255));
#29638=CARTESIAN_POINT('Ctrl Pts',(-0.0121148985784008,-0.0360615719774445,
-0.0136700557246864));
#29639=CARTESIAN_POINT('Ctrl Pts',(-0.0120891986319751,-0.0360629563944502,
-0.0136632586315875));
#29640=CARTESIAN_POINT('Ctrl Pts',(-0.0120729950306185,-0.0360638417506793,
-0.0136586881223282));
#29641=CARTESIAN_POINT('Ctrl Pts',(-0.011968443115175,-0.0360696374109848,
-0.0136273416432165));
#29642=CARTESIAN_POINT('Ctrl Pts',(-0.0118825866640175,-0.0360748002806229,
-0.0135929515872037));
#29643=CARTESIAN_POINT('Ctrl Pts',(-0.0117171428438136,-0.0360854202819952,
-0.0135087803732864));
#29644=CARTESIAN_POINT('Ctrl Pts',(-0.0116379679362567,-0.0360908561655726,
-0.0134589983884585));
#29645=CARTESIAN_POINT('Ctrl Pts',(-0.0115418963141715,-0.0360975688297569,
-0.0133856648372971));
#29646=CARTESIAN_POINT('Ctrl Pts',(-0.0115204659908521,-0.0360990734352142,
-0.0133683800004309));
#29647=CARTESIAN_POINT('Ctrl Pts',(-0.0114930342625622,-0.0361009964526935,
-0.0133450159460462));
#29648=CARTESIAN_POINT('Ctrl Pts',(-0.0114866056476683,-0.0361014468862943,
-0.0133394482392113));
#29649=CARTESIAN_POINT('Ctrl Pts',(-0.01147628904584,-0.0361021688930658,
-0.0133303628639657));
#29650=CARTESIAN_POINT('Ctrl Pts',(-0.0114723724641684,-0.0361024427943175,
-0.0133268781043655));
#29651=CARTESIAN_POINT('Ctrl Pts',(-0.0114647613371767,-0.0361029745382788,
-0.0133200363262922));
#29652=CARTESIAN_POINT('Ctrl Pts',(-0.0114610652096871,-0.0361032325074985,
-0.01331668124008));
#29653=CARTESIAN_POINT('Ctrl Pts',(-0.0114520152452579,-0.0361038636917491,
-0.0133083858566633));
#29654=CARTESIAN_POINT('Ctrl Pts',(-0.011446679915248,-0.0361042354087775,
-0.0133034254002689));
#29655=CARTESIAN_POINT('Ctrl Pts',(-0.0114270579278263,-0.0361056019086352,
-0.0132849212904151));
#29656=CARTESIAN_POINT('Ctrl Pts',(-0.0114129951886707,-0.0361065801071223,
-0.0132711418945278));
#29657=CARTESIAN_POINT('Ctrl Pts',(-0.0113774380711826,-0.0361090624512274,
-0.0132349416272559));
#29658=CARTESIAN_POINT('Ctrl Pts',(-0.0113563494801813,-0.0361105436271254,
-0.013212133686451));
#29659=CARTESIAN_POINT('Ctrl Pts',(-0.0112900665192613,-0.0361152866218025,
-0.0131359567629314));
#29660=CARTESIAN_POINT('Ctrl Pts',(-0.0112478071716245,-0.0361184548574191,
-0.0130801494253951));
#29661=CARTESIAN_POINT('Ctrl Pts',(-0.0111579070747159,-0.0361259751813615,
-0.0129429819507985));
#29662=CARTESIAN_POINT('Ctrl Pts',(-0.0111136448225688,-0.0361303516688328,
-0.0128597514510496));
#29663=CARTESIAN_POINT('Ctrl Pts',(-0.0110707494608318,-0.0361358385312744,
-0.0127575517994717));
#29664=CARTESIAN_POINT('Ctrl Pts',(-0.0110645116010986,-0.0361366767583283,
-0.0127419833887681));
#29665=CARTESIAN_POINT('Ctrl Pts',(-0.0110550176752123,-0.036138020435348,
-0.0127171221209778));
#29666=CARTESIAN_POINT('Ctrl Pts',(-0.0110515945700138,-0.036138520272365,
-0.012707894238553));
#29667=CARTESIAN_POINT('Ctrl Pts',(-0.0110453506252458,-0.0361394617623763,
-0.0126905550800128));
#29668=CARTESIAN_POINT('Ctrl Pts',(-0.0110425087540463,-0.0361399026915109,
-0.0126824517504928));
#29669=CARTESIAN_POINT('Ctrl Pts',(-0.0110362871562949,-0.0361408966748177,
-0.0126642256829963));
#29670=CARTESIAN_POINT('Ctrl Pts',(-0.0110329445342361,-0.0361414509341665,
-0.0126540908207389));
#29671=CARTESIAN_POINT('Ctrl Pts',(-0.011023254600046,-0.0361431204423895,
-0.0126236529164242));
#29672=CARTESIAN_POINT('Ctrl Pts',(-0.0110172219038535,-0.0361442458995248,
-0.0126032530308853));
#29673=CARTESIAN_POINT('Ctrl Pts',(-0.0109903594074654,-0.0361496999765438,
-0.0125049892653878));
#29674=CARTESIAN_POINT('Ctrl Pts',(-0.0109752325960801,-0.0361542079032663,
-0.0124257067467117));
#29675=CARTESIAN_POINT('Ctrl Pts',(-0.010956872869965,-0.0361637402501552,
-0.0122598437510436));
#29676=CARTESIAN_POINT('Ctrl Pts',(-0.0109545906758734,-0.0361687620808592,
-0.012173428538151));
#29677=CARTESIAN_POINT('Ctrl Pts',(-0.0109616935662868,-0.0361757171680143,
-0.0120499020085666));
#29678=CARTESIAN_POINT('Ctrl Pts',(-0.0109652021514898,-0.0361777853871252,
-0.0120126161084856));
#29679=CARTESIAN_POINT('Ctrl Pts',(-0.0109712850658341,-0.036180293065164,
-0.0119661675885122));
#29680=CARTESIAN_POINT('Ctrl Pts',(-0.0109725914901125,-0.0361807923935559,
-0.0119568539841126));
#29681=CARTESIAN_POINT('Ctrl Pts',(-0.0109747873383674,-0.0361815731404391,
-0.0119421763981681));
#29682=CARTESIAN_POINT('Ctrl Pts',(-0.0109756200786809,-0.0361818575921791,
-0.0119368043195178));
#29683=CARTESIAN_POINT('Ctrl Pts',(-0.0109772496437129,-0.0361823928124027,
-0.0119266467736726));
#29684=CARTESIAN_POINT('Ctrl Pts',(-0.0109780406434466,-0.0361826438783202,
-0.0119218606663769));
#29685=CARTESIAN_POINT('Ctrl Pts',(-0.0109799727951164,-0.0361832370917533,
-0.0119105029883949));
#29686=CARTESIAN_POINT('Ctrl Pts',(-0.0109811339975104,-0.0361835781021954,
-0.0119039350010676));
#29687=CARTESIAN_POINT('Ctrl Pts',(-0.0109852226464653,-0.036184728706596,
-0.011881652546014));
#29688=CARTESIAN_POINT('Ctrl Pts',(-0.0109883517628177,-0.0361855275504684,
-0.0118659756468744));
#29689=CARTESIAN_POINT('Ctrl Pts',(-0.0109966474911758,-0.0361874661730907,
-0.0118275359933416));
#29690=CARTESIAN_POINT('Ctrl Pts',(-0.0110020881238203,-0.0361885935066934,
-0.0118048360314069));
#29691=CARTESIAN_POINT('Ctrl Pts',(-0.0110277809518416,-0.0361933875263122,
-0.0117074427553644));
#29692=CARTESIAN_POINT('Ctrl Pts',(-0.0110531220492531,-0.0361968875931943,
-0.0116342049881169));
#29693=CARTESIAN_POINT('Ctrl Pts',(-0.0111207497586246,-0.0362046666688781,
-0.0114778900941258));
#29694=CARTESIAN_POINT('Ctrl Pts',(-0.011165273332873,-0.0362089525329183,
-0.0113961183978989));
#29695=CARTESIAN_POINT('Ctrl Pts',(-0.0112290480928655,-0.0362145792624668,
-0.0113006330997497));
#29696=CARTESIAN_POINT('Ctrl Pts',(-0.0112416044612554,-0.0362156663512808,
-0.0112826737228367));
#29697=CARTESIAN_POINT('Ctrl Pts',(-0.011260875188243,-0.0362173078300366,
-0.0112563241015212));
#29698=CARTESIAN_POINT('Ctrl Pts',(-0.0112673018895231,-0.0362178510364836,
-0.0112477263652471));
#29699=CARTESIAN_POINT('Ctrl Pts',(-0.0112789882452256,-0.0362188316703332,
-0.0112324276951326));
#29700=CARTESIAN_POINT('Ctrl Pts',(-0.0112842147079078,-0.0362192677649649,
-0.0112257018925722));
#29701=CARTESIAN_POINT('Ctrl Pts',(-0.0112954697055776,-0.0362202018240542,
-0.0112114630370418));
#29702=CARTESIAN_POINT('Ctrl Pts',(-0.0113015134252252,-0.0362207003944266,
-0.0112039624964365));
#29703=CARTESIAN_POINT('Ctrl Pts',(-0.0113181050903677,-0.0362220612798321,
-0.0111837615714883));
#29704=CARTESIAN_POINT('Ctrl Pts',(-0.0113287870721487,-0.0362229290765472,
-0.0111711733388549));
#29705=CARTESIAN_POINT('Ctrl Pts',(-0.0113949512804052,-0.0362282558166161,
-0.0110956912317522));
#29706=CARTESIAN_POINT('Ctrl Pts',(-0.0114552760775991,-0.0362329222290524,
-0.011037243908343));
#29707=CARTESIAN_POINT('Ctrl Pts',(-0.0115615607828297,-0.0362407695512787,
-0.0109498557629705));
#29708=CARTESIAN_POINT('Ctrl Pts',(-0.0116048339847863,-0.0362438741970801,
-0.0109179122296245));
#29709=CARTESIAN_POINT('Ctrl Pts',(-0.0117101602480476,-0.036251124689397,
-0.0108483539185482));
#29710=CARTESIAN_POINT('Ctrl Pts',(-0.011773380539475,-0.0362552491934912,
-0.0108127217884991));
#29711=CARTESIAN_POINT('Ctrl Pts',(-0.0118482771097153,-0.0362597030087172,
-0.0107772058977001));
#29712=CARTESIAN_POINT('Ctrl Pts',(-0.0118577228629406,-0.0362602571113017,
-0.0107728431886333));
#29713=CARTESIAN_POINT('Ctrl Pts',(-0.0118724056986486,-0.0362611058785067,
-0.010766240993051));
#29714=CARTESIAN_POINT('Ctrl Pts',(-0.0118776120989624,-0.0362614044250356,
-0.0107639344759347));
#29715=CARTESIAN_POINT('Ctrl Pts',(-0.0118872463652017,-0.0362619522534782,
-0.0107597299907103));
#29716=CARTESIAN_POINT('Ctrl Pts',(-0.0118916703675122,-0.0362622020076609,
-0.0107578239269718));
#29717=CARTESIAN_POINT('Ctrl Pts',(-0.0119018501396967,-0.0362627726519869,
-0.0107534944206526));
#29718=CARTESIAN_POINT('Ctrl Pts',(-0.01190761176663,-0.0362630926873127,
-0.0107510851712563));
#29719=CARTESIAN_POINT('Ctrl Pts',(-0.0119257375343961,-0.0362640907588852,
-0.0107436347626959));
#29720=CARTESIAN_POINT('Ctrl Pts',(-0.011938152874298,-0.0362647616911954,
-0.010738718947152));
#29721=CARTESIAN_POINT('Ctrl Pts',(-0.0120034351687105,-0.0362682310749773,
-0.0107138459573434));
#29722=CARTESIAN_POINT('Ctrl Pts',(-0.0120573094421694,-0.0362708957164369,
-0.0106966412695876));
#29723=CARTESIAN_POINT('Ctrl Pts',(-0.0122073705300166,-0.036278072884494,
-0.0106576555457311));
#29724=CARTESIAN_POINT('Ctrl Pts',(-0.0123048831318662,-0.0362824830479426,
-0.0106420716389651));
#29725=CARTESIAN_POINT('Ctrl Pts',(-0.0124570484530169,-0.0362896466107501,
-0.0106325083995513));
#29726=CARTESIAN_POINT('Ctrl Pts',(-0.0125110161422331,-0.0362922379838347,
-0.010631950376522));
#29727=CARTESIAN_POINT('Ctrl Pts',(-0.0125803369323508,-0.0362956848547156,
-0.0106348686282824));
#29728=CARTESIAN_POINT('Ctrl Pts',(-0.0125957634583471,-0.036296459329547,
-0.010635750342602));
#29729=CARTESIAN_POINT('Ctrl Pts',(-0.0126206305493715,-0.0362977207308511,
-0.010637546695755));
#29730=CARTESIAN_POINT('Ctrl Pts',(-0.0126300806566654,-0.0362982031216088,
-0.0106383169734026));
#29731=CARTESIAN_POINT('Ctrl Pts',(-0.0126481729081534,-0.0362991326803021,
-0.0106399596612617));
#29732=CARTESIAN_POINT('Ctrl Pts',(-0.0126568159794567,-0.036299579390021,
-0.0106408180480625));
#29733=CARTESIAN_POINT('Ctrl Pts',(-0.012676762745127,-0.0363006165826884,
-0.0106429692822722));
#29734=CARTESIAN_POINT('Ctrl Pts',(-0.0126880602121421,-0.0363012086857701,
-0.0106443142612758));
#29735=CARTESIAN_POINT('Ctrl Pts',(-0.0127240947681315,-0.0363031125234025,
-0.0106490089410044));
#29736=CARTESIAN_POINT('Ctrl Pts',(-0.0127487650067397,-0.0363044390462012,
-0.0106528339187856));
#29737=CARTESIAN_POINT('Ctrl Pts',(-0.0128560992610033,-0.0363103133987427,
-0.0106721528892649));
#29738=CARTESIAN_POINT('Ctrl Pts',(-0.0129375016848264,-0.0363150478948562,
-0.0106937902533563));
#29739=CARTESIAN_POINT('Ctrl Pts',(-0.0131133414203478,-0.0363257331868827,
-0.0107562848289119));
#29740=CARTESIAN_POINT('Ctrl Pts',(-0.0132062956559183,-0.0363317003266798,
-0.0108001677884493));
#29741=CARTESIAN_POINT('Ctrl Pts',(-0.0133079152805953,-0.0363381526332863,
-0.0108611756241289));
#29742=CARTESIAN_POINT('Ctrl Pts',(-0.0133214903328683,-0.0363390125569821,
-0.0108696151274333));
#29743=CARTESIAN_POINT('Ctrl Pts',(-0.0133402175855677,-0.0363401933428642,
-0.0108816651593054));
#29744=CARTESIAN_POINT('Ctrl Pts',(-0.0133454821363869,-0.0363405246638285,
-0.0108850982906306));
#29745=CARTESIAN_POINT('Ctrl Pts',(-0.0133549177036505,-0.0363411171537095,
-0.0108913339335234));
#29746=CARTESIAN_POINT('Ctrl Pts',(-0.0133590962612432,-0.0363413790577134,
-0.0108941248188989));
#29747=CARTESIAN_POINT('Ctrl Pts',(-0.0133676818595878,-0.0363419161088174,
-0.0108999200454453));
#29748=CARTESIAN_POINT('Ctrl Pts',(-0.0133720870231281,-0.0363421910941396,
-0.010902926866466));
#29749=CARTESIAN_POINT('Ctrl Pts',(-0.0133834704633554,-0.0363429004487006,
-0.0109107836614822));
#29750=CARTESIAN_POINT('Ctrl Pts',(-0.0133904245067542,-0.0363433325704652,
-0.0109156686096983));
#29751=CARTESIAN_POINT('Ctrl Pts',(-0.0134209629100696,-0.0363452264748472,
-0.0109374996669656));
#29752=CARTESIAN_POINT('Ctrl Pts',(-0.013444107697458,-0.0363466519362665,
-0.0109550530511747));
#29753=CARTESIAN_POINT('Ctrl Pts',(-0.0135104271492173,-0.0363507502054419,
-0.0110083657052845));
#29754=CARTESIAN_POINT('Ctrl Pts',(-0.0135521665369769,-0.0363533483823784,
-0.0110458371295945));
#29755=CARTESIAN_POINT('Ctrl Pts',(-0.0136737002918405,-0.0363612738800246,
-0.0111675293003274));
#29756=CARTESIAN_POINT('Ctrl Pts',(-0.0137461116636287,-0.0363665559123479,
-0.0112585237994112));
#29757=CARTESIAN_POINT('Ctrl Pts',(-0.0138174488374334,-0.0363731688119264,
-0.0113724117269202));
#29758=CARTESIAN_POINT('Ctrl Pts',(-0.0138269664372651,-0.0363740864268147,
-0.0113882303957387));
#29759=CARTESIAN_POINT('Ctrl Pts',(-0.0138418413518704,-0.0363755811969191,
-0.011413988374745));
#29760=CARTESIAN_POINT('Ctrl Pts',(-0.0138473775129398,-0.036376152018528,
-0.0114238225780818));
#29761=CARTESIAN_POINT('Ctrl Pts',(-0.0138570156772217,-0.0363771724288197,
-0.0114413915201597));
#29762=CARTESIAN_POINT('Ctrl Pts',(-0.013861160693953,-0.0363776204767645,
-0.0114491021629619));
#29763=CARTESIAN_POINT('Ctrl Pts',(-0.0138697595828043,-0.0363785698534938,
-0.0114654296343553));
#29764=CARTESIAN_POINT('Ctrl Pts',(-0.0138741982534943,-0.0363790716882443,
-0.0114740540027902));
#29765=CARTESIAN_POINT('Ctrl Pts',(-0.0138858107905818,-0.0363804167990027,
-0.0114971498678827));
#29766=CARTESIAN_POINT('Ctrl Pts',(-0.0138928391087077,-0.0363812650498414,
-0.0115116928627213));
#29767=CARTESIAN_POINT('Ctrl Pts',(-0.013929096430443,-0.0363858303468814,
-0.0115898242272903));
#29768=CARTESIAN_POINT('Ctrl Pts',(-0.0139541988972364,-0.0363896858341416,
-0.0116552284130325));
#29769=CARTESIAN_POINT('Ctrl Pts',(-0.0140028366343276,-0.0363990330694428,
-0.0118133106121293));
#29770=CARTESIAN_POINT('Ctrl Pts',(-0.0140223757454965,-0.0364045969860129,
-0.0119069184214881));
#29771=CARTESIAN_POINT('Ctrl Pts',(-0.0140380045422238,-0.0364124568433655,
-0.0120445276131966));
#29772=CARTESIAN_POINT('Ctrl Pts',(-0.0140410714644329,-0.036414864931502,
-0.0120875148762122));
#29773=CARTESIAN_POINT('Ctrl Pts',(-0.0140426067239643,-0.0364176950862156,
-0.0121398133030783));
#29774=CARTESIAN_POINT('Ctrl Pts',(-0.0140427948970806,-0.0364181912692948,
-0.0121490521962625));
#29775=CARTESIAN_POINT('Ctrl Pts',(-0.014042966764963,-0.0364189954516571,
-0.0121641525360454));
#29776=CARTESIAN_POINT('Ctrl Pts',(-0.0140430000775132,-0.0364193058872427,
-0.0121700130663469));
#29777=CARTESIAN_POINT('Ctrl Pts',(-0.0140429999998646,-0.0364196145604726,
-0.0121758737299574));
#29778=CARTESIAN_POINT('Ctrl Pts',(-0.0133928340876084,-0.0365776381485745,
-0.0112832194050649));
#29779=CARTESIAN_POINT('Ctrl Pts',(-0.0130952609160143,-0.0365511095967742,
-0.0109855742143942));
#29780=CARTESIAN_POINT('Ctrl Pts',(-0.0121841523466751,-0.0364980554675351,
-0.010716645344559));
#29781=CARTESIAN_POINT('Ctrl Pts',(-0.0110992562595946,-0.036418475760857,
-0.0116550159846514));
#29782=CARTESIAN_POINT('Ctrl Pts',(-0.0113060193050241,-0.0363388990285403,
-0.013072272818964));
#29783=CARTESIAN_POINT('Ctrl Pts',(-0.0126086058506385,-0.0362593222962236,
-0.0136653243656934));
#29784=CARTESIAN_POINT('Ctrl Pts',(-0.0138123222557375,-0.0361797455639069,
-0.0128890170219797));
#29785=CARTESIAN_POINT('Ctrl Pts',(-0.0138090066083574,-0.0361001688315902,
-0.0114570252002803));
#29786=CARTESIAN_POINT('Ctrl Pts',(-0.0126024821547228,-0.0360205920992735,
-0.0106859178189944));
#29787=CARTESIAN_POINT('Ctrl Pts',(-0.0113015994342994,-0.0359410153669568,
-0.0112846225371221));
#29788=CARTESIAN_POINT('Ctrl Pts',(-0.0111025739600164,-0.0358614386346401,
-0.0127027090585796));
#29789=CARTESIAN_POINT('Ctrl Pts',(-0.0121882761682891,-0.0357818619023234,
-0.0136364138535612));
#29790=CARTESIAN_POINT('Ctrl Pts',(-0.0135605905087235,-0.0357022851700067,
-0.0132273094558074));
#29791=CARTESIAN_POINT('Ctrl Pts',(-0.0139578092204135,-0.03562270843769,
-0.0118515172183842));
#29792=CARTESIAN_POINT('Ctrl Pts',(-0.0130147529561138,-0.0355431317053733,
-0.0107739131649265));
#29793=CARTESIAN_POINT('Ctrl Pts',(-0.0115984404799773,-0.0354635549730566,
-0.0109852243885246));
#29794=CARTESIAN_POINT('Ctrl Pts',(-0.0110110050149965,-0.0353839782407399,
-0.0122911757623016));
#29795=CARTESIAN_POINT('Ctrl Pts',(-0.0117925206434878,-0.0353044015084232,
-0.0134911019626899));
#29796=CARTESIAN_POINT('Ctrl Pts',(-0.0132244788603522,-0.0352248247761065,
-0.0134818151702574));
#29797=CARTESIAN_POINT('Ctrl Pts',(-0.0139903656765037,-0.0351452480437898,
-0.0122718534549942));
#29798=CARTESIAN_POINT('Ctrl Pts',(-0.0133860405686823,-0.0350656713114731,
-0.0109736311318028));
#29799=CARTESIAN_POINT('Ctrl Pts',(-0.0119671076448217,-0.0349860945791564,
-0.0107807075166315));
#29800=CARTESIAN_POINT('Ctrl Pts',(-0.0110381051925874,-0.0349065178468397,
-0.0118704526781616));
#29801=CARTESIAN_POINT('Ctrl Pts',(-0.0114531392148339,-0.034826941114523,
-0.0132409769756585));
#29802=CARTESIAN_POINT('Ctrl Pts',(-0.0128306358568174,-0.0347473643822063,
-0.0136322481173509));
#29803=CARTESIAN_POINT('Ctrl Pts',(-0.0139041525817756,-0.0346677876498896,
-0.0126845393365732));
#29804=CARTESIAN_POINT('Ctrl Pts',(-0.0136867198526057,-0.0345882109175729,
-0.0112691548999602));
#29805=CARTESIAN_POINT('Ctrl Pts',(-0.0123782409152947,-0.0345086341852562,
-0.0106873706036063));
#29806=CARTESIAN_POINT('Ctrl Pts',(-0.0111817048159939,-0.0344290574529395,
-0.0114740671512591));
#29807=CARTESIAN_POINT('Ctrl Pts',(-0.0111971826193403,-0.0343494807206229,
-0.0129059716638541));
#29808=CARTESIAN_POINT('Ctrl Pts',(-0.0124104443467463,-0.0342699039883061,
-0.0136666201218039));
#29809=CARTESIAN_POINT('Ctrl Pts',(-0.0137060417285948,-0.0341903272559894,
-0.013056687732387));
#29810=CARTESIAN_POINT('Ctrl Pts',(-0.013892828761843,-0.0341107505236727,
-0.0116369339861979));
#29811=CARTESIAN_POINT('Ctrl Pts',(-0.0127990772296097,-0.034031173791356,
-0.0107126517341985));
#29812=CARTESIAN_POINT('Ctrl Pts',(-0.0114303601473809,-0.0339515970590393,
-0.0111336073665443));
#29813=CARTESIAN_POINT('Ctrl Pts',(-0.0110450482905081,-0.0338720203267226,
-0.0125127827972119));
#29814=CARTESIAN_POINT('Ctrl Pts',(-0.011997389579471,-0.0337924435944059,
-0.0135821920570098));
#29815=CARTESIAN_POINT('Ctrl Pts',(-0.0134118207135884,-0.0337128668620893,
-0.0133586419229471));
#29816=CARTESIAN_POINT('Ctrl Pts',(-0.0139879423436801,-0.0336332901297725,
-0.0120476598624509));
#29817=CARTESIAN_POINT('Ctrl Pts',(-0.0131960799067701,-0.0335537133974558,
-0.0108545362407697));
#29818=CARTESIAN_POINT('Ctrl Pts',(-0.011764255695894,-0.0334741366651392,
-0.0108762047605805));
#29819=CARTESIAN_POINT('Ctrl Pts',(-0.0110088599028788,-0.0333945599328224,
-0.012092743823454));
#29820=CARTESIAN_POINT('Ctrl Pts',(-0.0116243881266391,-0.0333149832005057,
-0.0133856920441328));
#29821=CARTESIAN_POINT('Ctrl Pts',(-0.0130449361797783,-0.0332354064681891,
-0.0135663390045967));
#29822=CARTESIAN_POINT('Ctrl Pts',(-0.0139644809416035,-0.0331558297358723,
-0.0124686015466394));
#29823=CARTESIAN_POINT('Ctrl Pts',(-0.0135376115745145,-0.0330762530035557,
-0.011101717265128));
#29824=CARTESIAN_POINT('Ctrl Pts',(-0.012156783132532,-0.0329966762712389,
-0.0107223718955571));
#29825=CARTESIAN_POINT('Ctrl Pts',(-0.0110915013299854,-0.0329170995389223,
-0.0116793278907656));
#29826=CARTESIAN_POINT('Ctrl Pts',(-0.0113211646892293,-0.0328375228066056,
-0.0130927792825796));
#29827=CARTESIAN_POINT('Ctrl Pts',(-0.01263462536737,-0.0327579460742888,
-0.0136632274770574));
#29828=CARTESIAN_POINT('Ctrl Pts',(-0.0138243142082752,-0.0326783693419721,
-0.012866213953063));
#29829=CARTESIAN_POINT('Ctrl Pts',(-0.0137964553771785,-0.0325987926096555,
-0.0114344968088202));
#29830=CARTESIAN_POINT('Ctrl Pts',(-0.0125766617193749,-0.0325192158773387,
-0.0106843678012449));
#29831=CARTESIAN_POINT('Ctrl Pts',(-0.0112863868288221,-0.032439639145022,
-0.0113054803533772));
#29832=CARTESIAN_POINT('Ctrl Pts',(-0.0111118833179225,-0.0323600624127054,
-0.0127267961593106));
#29833=CARTESIAN_POINT('Ctrl Pts',(-0.0122135861817712,-0.0322804856803887,
-0.0136415862420932));
#29834=CARTESIAN_POINT('Ctrl Pts',(-0.0135786121115237,-0.032200908948072,
-0.0132088111195533));
#29835=CARTESIAN_POINT('Ctrl Pts',(-0.0139519839028259,-0.0321213322157552,
-0.0118263554781389));
#29836=CARTESIAN_POINT('Ctrl Pts',(-0.0129904310894627,-0.0320417554834385,
-0.0107652210455696));
#29837=CARTESIAN_POINT('Ctrl Pts',(-0.0115779858617312,-0.0319621787511219,
-0.01100099333779));
#29838=CARTESIAN_POINT('Ctrl Pts',(-0.0110132217655809,-0.0318826020188051,
-0.0123169080795676));
#29839=CARTESIAN_POINT('Ctrl Pts',(-0.0118153714793421,-0.0318030252864884,
-0.0135031399041744));
#29840=CARTESIAN_POINT('Ctrl Pts',(-0.0132469547918328,-0.0317234485541717,
-0.0134690912764528));
#29841=CARTESIAN_POINT('Ctrl Pts',(-0.0139918029961525,-0.0316438718218551,
-0.0122460658368738));
#29842=CARTESIAN_POINT('Ctrl Pts',(-0.0133651177178693,-0.0315642950895384,
-0.0109584883729171));
#29843=CARTESIAN_POINT('Ctrl Pts',(-0.0119430607432697,-0.0314847183572217,
-0.0107901316166862));
#29844=CARTESIAN_POINT('Ctrl Pts',(-0.011033042409537,-0.0314051416249049,
-0.0118957792096504));
#29845=CARTESIAN_POINT('Ctrl Pts',(-0.0114717152553868,-0.0313255648925883,
-0.0132589214302837));
#29846=CARTESIAN_POINT('Ctrl Pts',(-0.0128557721434822,-0.0312459881602716,
-0.0136263123589553));
#29847=CARTESIAN_POINT('Ctrl Pts',(-0.0139127395828671,-0.0311664114279549,
-0.0126601812869636));
#29848=CARTESIAN_POINT('Ctrl Pts',(-0.013670862357182,-0.0310868346956382,
-0.0112487675025001));
#29849=CARTESIAN_POINT('Ctrl Pts',(-0.0123525189326018,-0.0310072579633215,
-0.0106897002180619));
#29850=CARTESIAN_POINT('Ctrl Pts',(-0.0111697647962804,-0.0309276812310048,
-0.011496966988396));
#29851=CARTESIAN_POINT('Ctrl Pts',(-0.0112100054671832,-0.0308481044986881,
-0.0129283976523225));
#29852=CARTESIAN_POINT('Ctrl Pts',(-0.0124362342931823,-0.0307685277663714,
-0.0136679358835917));
#29853=CARTESIAN_POINT('Ctrl Pts',(-0.0137211008826827,-0.0306889510340547,
-0.013035718856821));
#29854=CARTESIAN_POINT('Ctrl Pts',(-0.0138832873524999,-0.030609374301738,
-0.0116128911297885));
#29855=CARTESIAN_POINT('Ctrl Pts',(-0.01277375482353,-0.0305297975694213,
-0.0107077693601632));
#29856=CARTESIAN_POINT('Ctrl Pts',(-0.0114124466955457,-0.0304502208371046,
-0.0111521247940392));
#29857=CARTESIAN_POINT('Ctrl Pts',(-0.011051187659041,-0.0303706441047879,
-0.0125381544417569));
#29858=CARTESIAN_POINT('Ctrl Pts',(-0.0120216020104472,-0.0302910673724712,
-0.0135901705217094));
#29859=CARTESIAN_POINT('Ctrl Pts',(-0.0134324915261294,-0.0302114906401545,
-0.0133436777917981));
#29860=CARTESIAN_POINT('Ctrl Pts',(-0.0139848228738421,-0.0301319118250522,
-0.0120198866613579));
#29861=CARTESIAN_POINT('Ctrl Pts',(-0.013444661127689,-0.0300788585873889,
-0.011238463163598));
#29862=CARTESIAN_POINT('Ctrl Pts',(-0.0130689497297049,-0.0300523309271644,
-0.0110488021962071));
#29863=CARTESIAN_POINT('Ctrl Pts',(-0.0134596600795358,-0.0366321952253369,
-0.0112164083979732));
#29864=CARTESIAN_POINT('Ctrl Pts',(-0.0131398144357782,-0.0366056666735365,
-0.0108964853447243));
#29865=CARTESIAN_POINT('Ctrl Pts',(-0.0121605120835799,-0.0365526125442975,
-0.0106074279440297));
#29866=CARTESIAN_POINT('Ctrl Pts',(-0.0109944147317139,-0.0364730328376194,
-0.011616032852381));
#29867=CARTESIAN_POINT('Ctrl Pts',(-0.0112166533798299,-0.0363934561053027,
-0.0131393671708349));
#29868=CARTESIAN_POINT('Ctrl Pts',(-0.0126167346774819,-0.036313879372986,
-0.013776806872569));
#29869=CARTESIAN_POINT('Ctrl Pts',(-0.0139105456968955,-0.0362343026406694,
-0.0129423952192144));
#29870=CARTESIAN_POINT('Ctrl Pts',(-0.0139069818831113,-0.0361547259083527,
-0.0114032230431297));
#29871=CARTESIAN_POINT('Ctrl Pts',(-0.0126101526410306,-0.0360751491760359,
-0.010574400554018));
#29872=CARTESIAN_POINT('Ctrl Pts',(-0.0112119026948481,-0.0359955724437193,
-0.0112179165503167));
#29873=CARTESIAN_POINT('Ctrl Pts',(-0.0109979807522041,-0.0359159957114026,
-0.0127421426555453));
#29874=CARTESIAN_POINT('Ctrl Pts',(-0.0121649445610503,-0.0358364189790859,
-0.0137457324940732));
#29875=CARTESIAN_POINT('Ctrl Pts',(-0.0136399725728248,-0.0357568422467691,
-0.0133060078416033));
#29876=CARTESIAN_POINT('Ctrl Pts',(-0.0140669219307673,-0.0356772655144525,
-0.0118272416225322));
#29877=CARTESIAN_POINT('Ctrl Pts',(-0.0130532806930891,-0.0355976887821358,
-0.010668982091448));
#29878=CARTESIAN_POINT('Ctrl Pts',(-0.0115309614152291,-0.0355181120498191,
-0.0108961093354223));
#29879=CARTESIAN_POINT('Ctrl Pts',(-0.0108995581423592,-0.0354385353175024,
-0.0122998073086775));
#29880=CARTESIAN_POINT('Ctrl Pts',(-0.0117395679052095,-0.0353589585851857,
-0.013589544437763));
#29881=CARTESIAN_POINT('Ctrl Pts',(-0.0132787039612366,-0.035279381852869,
-0.0135795625563719));
#29882=CARTESIAN_POINT('Ctrl Pts',(-0.0141019151413475,-0.0351998051205523,
-0.0122790387837916));
#29883=CARTESIAN_POINT('Ctrl Pts',(-0.0134523580858022,-0.0351202283882355,
-0.0108836483577088));
#29884=CARTESIAN_POINT('Ctrl Pts',(-0.011927222227453,-0.0350406516559189,
-0.0106762849802916));
#29885=CARTESIAN_POINT('Ctrl Pts',(-0.0109286866881252,-0.0349610749236022,
-0.0118475943454942));
#29886=CARTESIAN_POINT('Ctrl Pts',(-0.0113747847799511,-0.0348814981912855,
-0.0133206983349094));
#29887=CARTESIAN_POINT('Ctrl Pts',(-0.0128553829732249,-0.0348019214589688,
-0.013741254964823));
#29888=CARTESIAN_POINT('Ctrl Pts',(-0.0140092492513551,-0.0347223447266521,
-0.0127226129835629));
#29889=CARTESIAN_POINT('Ctrl Pts',(-0.0137755423252142,-0.0346427679943354,
-0.0112012912062412));
#29890=CARTESIAN_POINT('Ctrl Pts',(-0.012369127607767,-0.0345631912620187,
-0.0105759620752631));
#29891=CARTESIAN_POINT('Ctrl Pts',(-0.0110830343188129,-0.034483614529702,
-0.0114215405337574));
#29892=CARTESIAN_POINT('Ctrl Pts',(-0.0110996705899822,-0.0344040377973853,
-0.0129606188659093));
#29893=CARTESIAN_POINT('Ctrl Pts',(-0.0124037413708582,-0.0343244610650686,
-0.0137781996121936));
#29894=CARTESIAN_POINT('Ctrl Pts',(-0.0137963103864987,-0.0342448843327519,
-0.0131226155866023));
#29895=CARTESIAN_POINT('Ctrl Pts',(-0.0139970778769776,-0.0341653076004352,
-0.0115965974698001));
#29896=CARTESIAN_POINT('Ctrl Pts',(-0.0128214622760691,-0.0340857308681185,
-0.0106031354237402));
#29897=CARTESIAN_POINT('Ctrl Pts',(-0.011350300766642,-0.0340061541358018,
-0.0110555983406749));
#29898=CARTESIAN_POINT('Ctrl Pts',(-0.010936149456399,-0.0339265774034851,
-0.0125380009750028));
#29899=CARTESIAN_POINT('Ctrl Pts',(-0.0119597706753867,-0.0338470006711684,
-0.0136874523563485));
#29900=CARTESIAN_POINT('Ctrl Pts',(-0.0134800677983394,-0.0337674239388517,
-0.0134471701556437));
#29901=CARTESIAN_POINT('Ctrl Pts',(-0.0140993104292263,-0.033687847206535,
-0.0120380649636411));
#29902=CARTESIAN_POINT('Ctrl Pts',(-0.0132481794299362,-0.0336082704742183,
-0.010755639566168));
#29903=CARTESIAN_POINT('Ctrl Pts',(-0.0117091874098493,-0.0335286937419016,
-0.0107789299106268));
#29904=CARTESIAN_POINT('Ctrl Pts',(-0.0108972524749411,-0.0334491170095849,
-0.0120865233258413));
#29905=CARTESIAN_POINT('Ctrl Pts',(-0.0115588511665332,-0.0333695402772682,
-0.0134762448984304));
#29906=CARTESIAN_POINT('Ctrl Pts',(-0.0130857230418127,-0.0332899635449515,
-0.0136704127498293));
#29907=CARTESIAN_POINT('Ctrl Pts',(-0.0140740930105643,-0.0332103868126348,
-0.0124905128884402));
#29908=CARTESIAN_POINT('Ctrl Pts',(-0.0136152737333239,-0.0331308100803181,
-0.011021321359446));
#29909=CARTESIAN_POINT('Ctrl Pts',(-0.0121310943646713,-0.0330512333480014,
-0.0106135831104403));
#29910=CARTESIAN_POINT('Ctrl Pts',(-0.0109860793685498,-0.0329716566156847,
-0.0116421644327933));
#29911=CARTESIAN_POINT('Ctrl Pts',(-0.0112329323512678,-0.032892079883368,
-0.0131614084826278));
#29912=CARTESIAN_POINT('Ctrl Pts',(-0.012644701678118,-0.0328125031510513,
-0.0137745530380177));
#29913=CARTESIAN_POINT('Ctrl Pts',(-0.0139234352116284,-0.0327329264187346,
-0.0129178854080032));
#29914=CARTESIAN_POINT('Ctrl Pts',(-0.0138934912293844,-0.0326533496864179,
-0.0113790084681708));
#29915=CARTESIAN_POINT('Ctrl Pts',(-0.0125823996224312,-0.0325737729541012,
-0.0105727345220222));
#29916=CARTESIAN_POINT('Ctrl Pts',(-0.0111955514708247,-0.0324941962217845,
-0.0112403355124556));
#29917=CARTESIAN_POINT('Ctrl Pts',(-0.0110079868880278,-0.0324146194894678,
-0.0127680326045561));
#29918=CARTESIAN_POINT('Ctrl Pts',(-0.0121921489542162,-0.0323350427571511,
-0.0137512920205955));
#29919=CARTESIAN_POINT('Ctrl Pts',(-0.0136593430393164,-0.0322554660248344,
-0.013286124959568));
#29920=CARTESIAN_POINT('Ctrl Pts',(-0.01406066060538,-0.0321758892925177,
-0.0118001966004165));
#29921=CARTESIAN_POINT('Ctrl Pts',(-0.0130271384066231,-0.0320963125602011,
-0.0106596393926541));
#29922=CARTESIAN_POINT('Ctrl Pts',(-0.0115089758292782,-0.0320167358278843,
-0.0109130585439219));
#29923=CARTESIAN_POINT('Ctrl Pts',(-0.0109019408101714,-0.0319371590955676,
-0.0123274656138171));
#29924=CARTESIAN_POINT('Ctrl Pts',(-0.0117641290585723,-0.0318575823632509,
-0.0136024833835792));
#29925=CARTESIAN_POINT('Ctrl Pts',(-0.0133028621497417,-0.0317780056309342,
-0.0135658863167324));
#29926=CARTESIAN_POINT('Ctrl Pts',(-0.0141034600401229,-0.0316984288986175,
-0.0122513210386921));
#29927=CARTESIAN_POINT('Ctrl Pts',(-0.0134298692214611,-0.0316188521663008,
-0.0108673722080879));
#29928=CARTESIAN_POINT('Ctrl Pts',(-0.0119013754864109,-0.0315392754339842,
-0.0106864144463745));
#29929=CARTESIAN_POINT('Ctrl Pts',(-0.0109232449707309,-0.0314596987016675,
-0.0118748164929907));
#29930=CARTESIAN_POINT('Ctrl Pts',(-0.0113947511822221,-0.0313801219693508,
-0.0133399858789131));
#29931=CARTESIAN_POINT('Ctrl Pts',(-0.0128824006366349,-0.031300545237034,
-0.0137348749324596));
#29932=CARTESIAN_POINT('Ctrl Pts',(-0.0140184789640921,-0.0312209685047174,
-0.0126964318059509));
#29933=CARTESIAN_POINT('Ctrl Pts',(-0.0137584979431382,-0.0311413917724006,
-0.0111793778723534));
#29934=CARTESIAN_POINT('Ctrl Pts',(-0.0123414804107126,-0.031061815040084,
-0.0105784660544736));
#29935=CARTESIAN_POINT('Ctrl Pts',(-0.0110702006239228,-0.0309822383077672,
-0.0114461543560042));
#29936=CARTESIAN_POINT('Ctrl Pts',(-0.0111134531900773,-0.0309026615754506,
-0.0129847233733154));
#29937=CARTESIAN_POINT('Ctrl Pts',(-0.0124314616185408,-0.0308230848431338,
-0.0137796138548614));
#29938=CARTESIAN_POINT('Ctrl Pts',(-0.0138124966737499,-0.0307435081108172,
-0.0131000772526917));
#29939=CARTESIAN_POINT('Ctrl Pts',(-0.013986822321353,-0.0306639313785005,
-0.0115707550766674));
#29940=CARTESIAN_POINT('Ctrl Pts',(-0.0127942445627561,-0.0305843546461837,
-0.0105978876184423));
#29941=CARTESIAN_POINT('Ctrl Pts',(-0.0113310465458955,-0.0305047779138671,
-0.011075501742874));
#29942=CARTESIAN_POINT('Ctrl Pts',(-0.0109427483385165,-0.0304252011815503,
-0.0125652716121345));
#29943=CARTESIAN_POINT('Ctrl Pts',(-0.0119857953352411,-0.0303456244492337,
-0.0136960279855438));
#29944=CARTESIAN_POINT('Ctrl Pts',(-0.013502285760089,-0.0302660477169169,
-0.0134310860035175));
#29945=CARTESIAN_POINT('Ctrl Pts',(-0.014095957476293,-0.0301864689018147,
-0.0120082130205535));
#29946=CARTESIAN_POINT('Ctrl Pts',(-0.0135153662203476,-0.0301334156641513,
-0.0111683022841477));
#29947=CARTESIAN_POINT('Ctrl Pts',(-0.0131115339349587,-0.0301068880039268,
-0.0109644457540518));
#29948=CARTESIAN_POINT('Ctrl Pts',(-0.0135264860714633,-0.0366867523020992,
-0.0111495973908816));
#29949=CARTESIAN_POINT('Ctrl Pts',(-0.0131843679555423,-0.0366602237502991,
-0.0108073964750543));
#29950=CARTESIAN_POINT('Ctrl Pts',(-0.0121368718204848,-0.0366071696210597,
-0.0104982105435003));
#29951=CARTESIAN_POINT('Ctrl Pts',(-0.0108895732038333,-0.0365275899143818,
-0.0115770497201106));
#29952=CARTESIAN_POINT('Ctrl Pts',(-0.0111272874546357,-0.036448013182065,
-0.0132064615227055));
#29953=CARTESIAN_POINT('Ctrl Pts',(-0.0126248635043253,-0.0363684364497484,
-0.0138882893794445));
#29954=CARTESIAN_POINT('Ctrl Pts',(-0.0140087691380537,-0.0362888597174317,
-0.012995773416449));
#29955=CARTESIAN_POINT('Ctrl Pts',(-0.0140049571578653,-0.036209282985115,
-0.0113494208859793));
#29956=CARTESIAN_POINT('Ctrl Pts',(-0.0126178231273385,-0.0361297062527983,
-0.0104628832890415));
#29957=CARTESIAN_POINT('Ctrl Pts',(-0.011122205955397,-0.0360501295204815,
-0.0111512105635114));
#29958=CARTESIAN_POINT('Ctrl Pts',(-0.0108933875443916,-0.0359705527881648,
-0.0127815762525112));
#29959=CARTESIAN_POINT('Ctrl Pts',(-0.0121416129538115,-0.0358909760558482,
-0.0138550511345852));
#29960=CARTESIAN_POINT('Ctrl Pts',(-0.0137193546369261,-0.0358113993235314,
-0.0133847062273992));
#29961=CARTESIAN_POINT('Ctrl Pts',(-0.014176034641121,-0.0357318225912147,
-0.0118029660266803));
#29962=CARTESIAN_POINT('Ctrl Pts',(-0.0130918084300643,-0.035652245858898,
-0.0105640510179696));
#29963=CARTESIAN_POINT('Ctrl Pts',(-0.0114634823504808,-0.0355726691265813,
-0.0108069942823203));
#29964=CARTESIAN_POINT('Ctrl Pts',(-0.010788111269722,-0.0354930923942647,
-0.0123084388550532));
#29965=CARTESIAN_POINT('Ctrl Pts',(-0.011686615166931,-0.035413515661948,
-0.0136879869128362));
#29966=CARTESIAN_POINT('Ctrl Pts',(-0.0133329290621209,-0.0353339389296312,
-0.0136773099424865));
#29967=CARTESIAN_POINT('Ctrl Pts',(-0.0142134646061913,-0.0352543621973146,
-0.0122862241125889));
#29968=CARTESIAN_POINT('Ctrl Pts',(-0.013518675602922,-0.0351747854649978,
-0.0107936655836147));
#29969=CARTESIAN_POINT('Ctrl Pts',(-0.0118873368100842,-0.0350952087326811,
-0.0105718624439518));
#29970=CARTESIAN_POINT('Ctrl Pts',(-0.0108192681836631,-0.0350156320003644,
-0.0118247360128269));
#29971=CARTESIAN_POINT('Ctrl Pts',(-0.0112964303450682,-0.0349360552680477,
-0.0134004196941601));
#29972=CARTESIAN_POINT('Ctrl Pts',(-0.0128801300896323,-0.034856478535731,
-0.013850261812295));
#29973=CARTESIAN_POINT('Ctrl Pts',(-0.0141143459209346,-0.0347769018034143,
-0.0127606866305524));
#29974=CARTESIAN_POINT('Ctrl Pts',(-0.0138643647978225,-0.0346973250710977,
-0.011133427512522));
#29975=CARTESIAN_POINT('Ctrl Pts',(-0.0123600143002392,-0.034617748338781,
-0.0104645535469199));
#29976=CARTESIAN_POINT('Ctrl Pts',(-0.010984363821632,-0.0345381716064643,
-0.0113690139162556));
#29977=CARTESIAN_POINT('Ctrl Pts',(-0.0110021585606239,-0.0344585948741475,
-0.0130152660679645));
#29978=CARTESIAN_POINT('Ctrl Pts',(-0.01239703839497,-0.0343790181418309,
-0.0138897791025832));
#29979=CARTESIAN_POINT('Ctrl Pts',(-0.0138865790444026,-0.0342994414095142,
-0.0131885434408178));
#29980=CARTESIAN_POINT('Ctrl Pts',(-0.0141013269921123,-0.0342198646771974,
-0.0115562609534022));
#29981=CARTESIAN_POINT('Ctrl Pts',(-0.0128438473225283,-0.0341402879448807,
-0.010493619113282));
#29982=CARTESIAN_POINT('Ctrl Pts',(-0.0112702413859032,-0.034060711212564,
-0.0109775893148056));
#29983=CARTESIAN_POINT('Ctrl Pts',(-0.0108272506222901,-0.0339811344802474,
-0.0125632191527937));
#29984=CARTESIAN_POINT('Ctrl Pts',(-0.0119221517713024,-0.0339015577479307,
-0.0137927126556872));
#29985=CARTESIAN_POINT('Ctrl Pts',(-0.0135483148830904,-0.0338219810156139,
-0.0135356983883403));
#29986=CARTESIAN_POINT('Ctrl Pts',(-0.0142106785147725,-0.0337424042832973,
-0.0120284700648312));
#29987=CARTESIAN_POINT('Ctrl Pts',(-0.0133002789531021,-0.0336628275509806,
-0.0106567428915664));
#29988=CARTESIAN_POINT('Ctrl Pts',(-0.0116541191238046,-0.0335832508186639,
-0.0106816550606734));
#29989=CARTESIAN_POINT('Ctrl Pts',(-0.0107856450470035,-0.0335036740863471,
-0.0120803028282286));
#29990=CARTESIAN_POINT('Ctrl Pts',(-0.0114933142064273,-0.0334240973540305,
-0.0135667977527282));
#29991=CARTESIAN_POINT('Ctrl Pts',(-0.0131265099038471,-0.0333445206217137,
-0.0137744864950621));
#29992=CARTESIAN_POINT('Ctrl Pts',(-0.0141837050795251,-0.0332649438893971,
-0.012512424230241));
#29993=CARTESIAN_POINT('Ctrl Pts',(-0.0136929358921335,-0.0331853671570804,
-0.0109409254537638));
#29994=CARTESIAN_POINT('Ctrl Pts',(-0.0121054055968104,-0.0331057904247637,
-0.0105047943253235));
#29995=CARTESIAN_POINT('Ctrl Pts',(-0.0108806574071141,-0.033026213692447,
-0.0116050009748212));
#29996=CARTESIAN_POINT('Ctrl Pts',(-0.0111447000133064,-0.0329466369601303,
-0.0132300376826758));
#29997=CARTESIAN_POINT('Ctrl Pts',(-0.012654777988866,-0.0328670602278136,
-0.013885878598978));
#29998=CARTESIAN_POINT('Ctrl Pts',(-0.0140225562149815,-0.0327874834954969,
-0.0129695568629433));
#29999=CARTESIAN_POINT('Ctrl Pts',(-0.0139905270815905,-0.0327079067631802,
-0.0113235201275212));
#30000=CARTESIAN_POINT('Ctrl Pts',(-0.0125881375254875,-0.0326283300308635,
-0.0104611012427995));
#30001=CARTESIAN_POINT('Ctrl Pts',(-0.0111047161128272,-0.0325487532985468,
-0.011175190671534));
#30002=CARTESIAN_POINT('Ctrl Pts',(-0.010904090458133,-0.0324691765662301,
-0.0128092690498018));
#30003=CARTESIAN_POINT('Ctrl Pts',(-0.0121707117266613,-0.0323895998339134,
-0.0138609977990977));
#30004=CARTESIAN_POINT('Ctrl Pts',(-0.013740073967109,-0.0323100231015967,
-0.0133634387995829));
#30005=CARTESIAN_POINT('Ctrl Pts',(-0.0141693373079339,-0.03223044636928,
-0.0117740377226941));
#30006=CARTESIAN_POINT('Ctrl Pts',(-0.0130638457237835,-0.0321508696369633,
-0.0105540577397387));
#30007=CARTESIAN_POINT('Ctrl Pts',(-0.0114399657968253,-0.0320712929046466,
-0.0108251237500537));
#30008=CARTESIAN_POINT('Ctrl Pts',(-0.0107906598547619,-0.0319917161723299,
-0.0123380231480665));
#30009=CARTESIAN_POINT('Ctrl Pts',(-0.0117128866378026,-0.0319121394400132,
-0.0137018268629841));
#30010=CARTESIAN_POINT('Ctrl Pts',(-0.0133587695076506,-0.0318325627076965,
-0.0136626813570119));
#30011=CARTESIAN_POINT('Ctrl Pts',(-0.0142151170840931,-0.0317529859753798,
-0.0122565762405104));
#30012=CARTESIAN_POINT('Ctrl Pts',(-0.0134946207250529,-0.0316734092430631,
-0.0107762560432585));
#30013=CARTESIAN_POINT('Ctrl Pts',(-0.0118596902295519,-0.0315938325107464,
-0.0105826972760627));
#30014=CARTESIAN_POINT('Ctrl Pts',(-0.0108134475319248,-0.0315142557784297,
-0.0118538537763313));
#30015=CARTESIAN_POINT('Ctrl Pts',(-0.0113177871090574,-0.031434679046113,
-0.0134210503275425));
#30016=CARTESIAN_POINT('Ctrl Pts',(-0.0129090291297876,-0.0313551023137963,
-0.013843437505964));
#30017=CARTESIAN_POINT('Ctrl Pts',(-0.0141242183453171,-0.0312755255814796,
-0.0127326823249381));
#30018=CARTESIAN_POINT('Ctrl Pts',(-0.0138461335290945,-0.0311959488491629,
-0.0111099882422067));
#30019=CARTESIAN_POINT('Ctrl Pts',(-0.0123304418888237,-0.0311163721168462,
-0.0104672318908852));
#30020=CARTESIAN_POINT('Ctrl Pts',(-0.0109706364515652,-0.0310367953845295,
-0.0113953417236122));
#30021=CARTESIAN_POINT('Ctrl Pts',(-0.0110169009129712,-0.0309572186522128,
-0.0130410490943084));
#30022=CARTESIAN_POINT('Ctrl Pts',(-0.0124266889438992,-0.0308776419198961,
-0.0138912918261311));
#30023=CARTESIAN_POINT('Ctrl Pts',(-0.0139038924648172,-0.0307980651875794,
-0.0131644356485622));
#30024=CARTESIAN_POINT('Ctrl Pts',(-0.0140903572902061,-0.0307184884552627,
-0.0115286190235464));
#30025=CARTESIAN_POINT('Ctrl Pts',(-0.0128147343019823,-0.030638911722946,
-0.0104880058767215));
#30026=CARTESIAN_POINT('Ctrl Pts',(-0.0112496463962452,-0.0305593349906293,
-0.0109988786917086));
#30027=CARTESIAN_POINT('Ctrl Pts',(-0.0108343090179921,-0.0304797582583126,
-0.0125923887825122));
#30028=CARTESIAN_POINT('Ctrl Pts',(-0.0119499886600349,-0.0304001815259959,
-0.0138018854493781));
#30029=CARTESIAN_POINT('Ctrl Pts',(-0.0135720799940484,-0.0303206047936792,
-0.0135184942152367));
#30030=CARTESIAN_POINT('Ctrl Pts',(-0.0142070920787441,-0.0302410259785769,
-0.0119965393797492));
#30031=CARTESIAN_POINT('Ctrl Pts',(-0.0135860713130062,-0.0301879727409135,
-0.0110981414046974));
#30032=CARTESIAN_POINT('Ctrl Pts',(-0.0131541181402127,-0.0301614450806891,
-0.0108800893118964));
#30033=CARTESIAN_POINT('Ctrl Pts',(-0.0135933120633907,-0.0367413093788616,
-0.01108278638379));
#30034=CARTESIAN_POINT('Ctrl Pts',(-0.0132289214753065,-0.0367147808270613,
-0.0107183076053843));
#30035=CARTESIAN_POINT('Ctrl Pts',(-0.0121132315573896,-0.0366617266978222,
-0.0103889931429711));
#30036=CARTESIAN_POINT('Ctrl Pts',(-0.0107847316759526,-0.0365821469911441,
-0.0115380665878402));
#30037=CARTESIAN_POINT('Ctrl Pts',(-0.0110379215294415,-0.0365025702588274,
-0.0132735558745762));
#30038=CARTESIAN_POINT('Ctrl Pts',(-0.0126329923311686,-0.0364229935265107,
-0.0139997718863199));
#30039=CARTESIAN_POINT('Ctrl Pts',(-0.0141069925792118,-0.036343416794194,
-0.0130491516136838));
#30040=CARTESIAN_POINT('Ctrl Pts',(-0.0141029324326193,-0.0362638400618773,
-0.0112956187288288));
#30041=CARTESIAN_POINT('Ctrl Pts',(-0.0126254936136463,-0.0361842633295606,
-0.010351366024065));
#30042=CARTESIAN_POINT('Ctrl Pts',(-0.0110325092159457,-0.0361046865972439,
-0.0110845045767061));
#30043=CARTESIAN_POINT('Ctrl Pts',(-0.0107887943365794,-0.0360251098649272,
-0.0128210098494769));
#30044=CARTESIAN_POINT('Ctrl Pts',(-0.0121182813465727,-0.0359455331326105,
-0.0139643697750972));
#30045=CARTESIAN_POINT('Ctrl Pts',(-0.0137987367010273,-0.0358659564002938,
-0.0134634046131951));
#30046=CARTESIAN_POINT('Ctrl Pts',(-0.0142851473514748,-0.0357863796679771,
-0.0117786904308283));
#30047=CARTESIAN_POINT('Ctrl Pts',(-0.0131303361670396,-0.0357068029356604,
-0.010459119944491));
#30048=CARTESIAN_POINT('Ctrl Pts',(-0.0113960032857326,-0.0356272262033437,
-0.0107178792292181));
#30049=CARTESIAN_POINT('Ctrl Pts',(-0.0106766643970847,-0.035547649471027,
-0.0123170704014292));
#30050=CARTESIAN_POINT('Ctrl Pts',(-0.0116336624286527,-0.0354680727387103,
-0.0137864293879092));
#30051=CARTESIAN_POINT('Ctrl Pts',(-0.0133871541630052,-0.0353884960063937,
-0.013775057328601));
#30052=CARTESIAN_POINT('Ctrl Pts',(-0.0143250140710351,-0.0353089192740769,
-0.0122934094413862));
#30053=CARTESIAN_POINT('Ctrl Pts',(-0.0135849931200419,-0.0352293425417602,
-0.0107036828095206));
#30054=CARTESIAN_POINT('Ctrl Pts',(-0.0118474513927153,-0.0351497658094436,
-0.0104674399076118));
#30055=CARTESIAN_POINT('Ctrl Pts',(-0.0107098496792009,-0.0350701890771268,
-0.0118018776801594));
#30056=CARTESIAN_POINT('Ctrl Pts',(-0.0112180759101854,-0.0349906123448101,
-0.0134801410534109));
#30057=CARTESIAN_POINT('Ctrl Pts',(-0.0129048772060397,-0.0349110356124935,
-0.0139592686597671));
#30058=CARTESIAN_POINT('Ctrl Pts',(-0.014219442590514,-0.0348314588801767,
-0.0127987602775421));
#30059=CARTESIAN_POINT('Ctrl Pts',(-0.0139531872704309,-0.0347518821478601,
-0.0110655638188028));
#30060=CARTESIAN_POINT('Ctrl Pts',(-0.0123509009927115,-0.0346723054155433,
-0.0103531450185766));
#30061=CARTESIAN_POINT('Ctrl Pts',(-0.0108856933244511,-0.0345927286832267,
-0.0113164872987539));
#30062=CARTESIAN_POINT('Ctrl Pts',(-0.0109046465312656,-0.03451315195091,
-0.0130699132700196));
#30063=CARTESIAN_POINT('Ctrl Pts',(-0.0123903354190819,-0.0344335752185932,
-0.014001358592973));
#30064=CARTESIAN_POINT('Ctrl Pts',(-0.0139768477023065,-0.0343539984862765,
-0.0132544712950332));
#30065=CARTESIAN_POINT('Ctrl Pts',(-0.014205576107247,-0.0342744217539599,
-0.0115159244370042));
#30066=CARTESIAN_POINT('Ctrl Pts',(-0.0128662323689877,-0.0341948450216431,
-0.0103841028028237));
#30067=CARTESIAN_POINT('Ctrl Pts',(-0.0111901820051644,-0.0341152682893264,
-0.0108995802889362));
#30068=CARTESIAN_POINT('Ctrl Pts',(-0.0107183517881809,-0.0340356915570098,
-0.0125884373305846));
#30069=CARTESIAN_POINT('Ctrl Pts',(-0.0118845328672181,-0.0339561148246931,
-0.0138979729550261));
#30070=CARTESIAN_POINT('Ctrl Pts',(-0.0136165619678413,-0.0338765380923764,
-0.0136242266210369));
#30071=CARTESIAN_POINT('Ctrl Pts',(-0.0143220466003186,-0.0337969613600597,
-0.0120188751660214));
#30072=CARTESIAN_POINT('Ctrl Pts',(-0.013352378476268,-0.0337173846277429,
-0.0105578462169646));
#30073=CARTESIAN_POINT('Ctrl Pts',(-0.0115990508377599,-0.0336378078954263,
-0.0105843802107197));
#30074=CARTESIAN_POINT('Ctrl Pts',(-0.010674037619066,-0.0335582311631095,
-0.0120740823306159));
#30075=CARTESIAN_POINT('Ctrl Pts',(-0.0114277772463213,-0.0334786544307928,
-0.0136573506070259));
#30076=CARTESIAN_POINT('Ctrl Pts',(-0.0131672967658813,-0.0333990776984761,
-0.013878560240295));
#30077=CARTESIAN_POINT('Ctrl Pts',(-0.014293317148486,-0.0333195009661594,
-0.0125343355720417));
#30078=CARTESIAN_POINT('Ctrl Pts',(-0.013770598050943,-0.0332399242338428,
-0.0108605295480818));
#30079=CARTESIAN_POINT('Ctrl Pts',(-0.0120797168289496,-0.0331603475015261,
-0.0103960055402067));
#30080=CARTESIAN_POINT('Ctrl Pts',(-0.0107752354456785,-0.0330807707692093,
-0.0115678375168489));
#30081=CARTESIAN_POINT('Ctrl Pts',(-0.0110564676753449,-0.0330011940368927,
-0.013298666882724));
#30082=CARTESIAN_POINT('Ctrl Pts',(-0.012664854299614,-0.0329216173045759,
-0.0139972041599381));
#30083=CARTESIAN_POINT('Ctrl Pts',(-0.0141216772183346,-0.0328420405722592,
-0.0130212283178836));
#30084=CARTESIAN_POINT('Ctrl Pts',(-0.0140875629337964,-0.0327624638399425,
-0.0112680317868718));
#30085=CARTESIAN_POINT('Ctrl Pts',(-0.0125938754285439,-0.0326828871076258,
-0.0103494679635769));
#30086=CARTESIAN_POINT('Ctrl Pts',(-0.0110138807548298,-0.0326033103753091,
-0.0111100458306123));
#30087=CARTESIAN_POINT('Ctrl Pts',(-0.0108001940282382,-0.0325237336429924,
-0.0128505054950474));
#30088=CARTESIAN_POINT('Ctrl Pts',(-0.0121492744991063,-0.0324441569106758,
-0.0139707035775999));
#30089=CARTESIAN_POINT('Ctrl Pts',(-0.0138208048949018,-0.0323645801783591,
-0.0134407526395977));
#30090=CARTESIAN_POINT('Ctrl Pts',(-0.014278014010488,-0.0322850034460424,
-0.0117478788449718));
#30091=CARTESIAN_POINT('Ctrl Pts',(-0.0131005530409439,-0.0322054267137256,
-0.0104484760868233));
#30092=CARTESIAN_POINT('Ctrl Pts',(-0.0113709557643723,-0.032125849981409,
-0.0107371889561855));
#30093=CARTESIAN_POINT('Ctrl Pts',(-0.0106793788993524,-0.0320462732490923,
-0.0123485806823159));
#30094=CARTESIAN_POINT('Ctrl Pts',(-0.0116616442170328,-0.0319666965167755,
-0.0138011703423888));
#30095=CARTESIAN_POINT('Ctrl Pts',(-0.0134146768655595,-0.0318871197844589,
-0.0137594763972914));
#30096=CARTESIAN_POINT('Ctrl Pts',(-0.0143267741280635,-0.0318075430521422,
-0.0122618314423287));
#30097=CARTESIAN_POINT('Ctrl Pts',(-0.0135593722286447,-0.0317279663198255,
-0.0106851398784292));
#30098=CARTESIAN_POINT('Ctrl Pts',(-0.011818004972693,-0.0316483895875088,
-0.010478980105751));
#30099=CARTESIAN_POINT('Ctrl Pts',(-0.0107036500931186,-0.031568812855192,
-0.0118328910596716));
#30100=CARTESIAN_POINT('Ctrl Pts',(-0.0112408230358926,-0.0314892361228754,
-0.0135021147761719));
#30101=CARTESIAN_POINT('Ctrl Pts',(-0.0129356576229402,-0.0314096593905587,
-0.0139520000794683));
#30102=CARTESIAN_POINT('Ctrl Pts',(-0.0142299577265421,-0.031330082658242,
-0.0127689328439255));
#30103=CARTESIAN_POINT('Ctrl Pts',(-0.0139337691150506,-0.0312505059259253,
-0.01104059861206));
#30104=CARTESIAN_POINT('Ctrl Pts',(-0.0123194033669345,-0.0311709291936086,
-0.0103559977272969));
#30105=CARTESIAN_POINT('Ctrl Pts',(-0.0108710722792076,-0.0310913524612919,
-0.0113445290912203));
#30106=CARTESIAN_POINT('Ctrl Pts',(-0.0109203486358651,-0.0310117757289752,
-0.0130973748153013));
#30107=CARTESIAN_POINT('Ctrl Pts',(-0.0124219162692576,-0.0309321989966585,
-0.0140029697974007));
#30108=CARTESIAN_POINT('Ctrl Pts',(-0.0139952882558845,-0.0308526222643418,
-0.0132287940444329));
#30109=CARTESIAN_POINT('Ctrl Pts',(-0.0141938922590592,-0.0307730455320251,
-0.0114864829704253));
#30110=CARTESIAN_POINT('Ctrl Pts',(-0.0128352240412084,-0.0306934687997084,
-0.0103781241350006));
#30111=CARTESIAN_POINT('Ctrl Pts',(-0.011168246246595,-0.0306138920673917,
-0.0109222556405432));
#30112=CARTESIAN_POINT('Ctrl Pts',(-0.0107258696974676,-0.030534315335075,
-0.0126195059528898));
#30113=CARTESIAN_POINT('Ctrl Pts',(-0.0119141819848288,-0.0304547386027583,
-0.0139077429132125));
#30114=CARTESIAN_POINT('Ctrl Pts',(-0.013641874228008,-0.0303751618704416,
-0.013605902426956));
#30115=CARTESIAN_POINT('Ctrl Pts',(-0.0143182266811951,-0.0302955830553393,
-0.0119848657389449));
#30116=CARTESIAN_POINT('Ctrl Pts',(-0.0136567764056649,-0.030242529817676,
-0.011027980525247));
#30117=CARTESIAN_POINT('Ctrl Pts',(-0.0131967023454666,-0.0302160021574515,
-0.0107957328697411));
#30118=CARTESIAN_POINT('Ctrl Pts',(-0.0131954570230152,-0.0302142743898723,
-0.0107984686165627));
#30119=CARTESIAN_POINT('Ctrl Pts',(-0.0133260842763136,-0.0302142743898723,
-0.0108797587666653));
#30120=CARTESIAN_POINT('Ctrl Pts',(-0.0134431964764062,-0.0302142743898653,
-0.0109820158739861));
#30121=CARTESIAN_POINT('Ctrl Pts',(-0.0135427737583255,-0.0302142743898653,
-0.0110992550752643));
#30122=CARTESIAN_POINT('Ctrl Pts',(-0.0136693246268282,-0.0302142743898653,
-0.0112482521402409));
#30123=CARTESIAN_POINT('Ctrl Pts',(-0.0137677960716114,-0.0302142743898653,
-0.0114216612142502));
#30124=CARTESIAN_POINT('Ctrl Pts',(-0.0138291125118522,-0.0302142743898653,
-0.0116070749220759));
#30125=CARTESIAN_POINT('Ctrl Pts',(-0.0138679675928177,-0.0302142743898653,
-0.0117245681196817));
#30126=CARTESIAN_POINT('Ctrl Pts',(-0.0138918683604881,-0.0302142743898653,
-0.0118468920339111));
#30127=CARTESIAN_POINT('Ctrl Pts',(-0.0138981744272313,-0.0302142743898653,
-0.0119704513331141));
#30128=CARTESIAN_POINT('Ctrl Pts',(-0.0138992054768938,-0.0302142743898653,
-0.0119906534303858));
#30129=CARTESIAN_POINT('Ctrl Pts',(-0.0138997541990176,-0.0302142743898653,
-0.012010717926216));
#30130=CARTESIAN_POINT('Ctrl Pts',(-0.0138998410206969,-0.0302142743898653,
-0.0120304353897606));
#30131=CARTESIAN_POINT('Ctrl Pts',(-0.0139004085534207,-0.0302142743898653,
-0.0121593237721184));
#30132=CARTESIAN_POINT('Ctrl Pts',(-0.0138816703521106,-0.0302142743898653,
-0.0122755108733013));
#30133=CARTESIAN_POINT('Ctrl Pts',(-0.0138553750738999,-0.0302142743898653,
-0.0123756473142824));
#30134=CARTESIAN_POINT('Ctrl Pts',(-0.0138312935973491,-0.0302142743898653,
-0.0124673532599672));
#30135=CARTESIAN_POINT('Ctrl Pts',(-0.0138018158230822,-0.0302142743898653,
-0.0125455369110881));
#30136=CARTESIAN_POINT('Ctrl Pts',(-0.0137643803753388,-0.0302142743898653,
-0.0126240412720506));
#30137=CARTESIAN_POINT('Ctrl Pts',(-0.0137113315160428,-0.0302142743898653,
-0.0127352878858845));
#30138=CARTESIAN_POINT('Ctrl Pts',(-0.0136436767058198,-0.0302142743898653,
-0.0128397240745112));
#30139=CARTESIAN_POINT('Ctrl Pts',(-0.0135632704999152,-0.0302142743898653,
-0.0129326775871141));
#30140=CARTESIAN_POINT('Ctrl Pts',(-0.013482385375445,-0.0302142743898653,
-0.0130261847530378));
#30141=CARTESIAN_POINT('Ctrl Pts',(-0.0133921506665608,-0.0302142743898714,
-0.0131045911547339));
#30142=CARTESIAN_POINT('Ctrl Pts',(-0.0132924108208383,-0.0302142743898722,
-0.0131679081118086));
#30143=CARTESIAN_POINT('Ctrl Pts',(-0.0132850639690017,-0.0302142743898722,
-0.0131725720482625));
#30144=CARTESIAN_POINT('Ctrl Pts',(-0.0132776640935926,-0.0302142743898723,
-0.0131771523321702));
#30145=CARTESIAN_POINT('Ctrl Pts',(-0.0132702116598217,-0.0302142743898723,
-0.0131816495199757));
#30146=CARTESIAN_POINT('Ctrl Pts',(-0.0118276163558221,-0.0365771045634534,
-0.0135678901963669));
#30147=CARTESIAN_POINT('Ctrl Pts',(-0.0122917136632024,-0.0365505737722603,
-0.0137920680337233));
#30148=CARTESIAN_POINT('Ctrl Pts',(-0.0134536276171895,-0.0364975174036282,
-0.0137355881186744));
#30149=CARTESIAN_POINT('Ctrl Pts',(-0.0143295251580393,-0.0364179354575572,
-0.0122131193629488));
#30150=CARTESIAN_POINT('Ctrl Pts',(-0.0135189123462146,-0.0363383587252405,
-0.0106579330577131));
#30151=CARTESIAN_POINT('Ctrl Pts',(-0.0117737475226801,-0.0362587819929238,
-0.0104975924690421));
#30152=CARTESIAN_POINT('Ctrl Pts',(-0.0106951402918064,-0.0361792052606071,
-0.0118805694294325));
#30153=CARTESIAN_POINT('Ctrl Pts',(-0.0112764794961299,-0.0360996285282904,
-0.0135348382648464));
#30154=CARTESIAN_POINT('Ctrl Pts',(-0.0129823888886079,-0.0360200517959737,
-0.0139397807062913));
#30155=CARTESIAN_POINT('Ctrl Pts',(-0.0142449610580027,-0.035940475063657,
-0.0127229535318522));
#30156=CARTESIAN_POINT('Ctrl Pts',(-0.0139031673111846,-0.0358608983313403,
-0.0110031597499392));
#30157=CARTESIAN_POINT('Ctrl Pts',(-0.0122713737247802,-0.0357813215990236,
-0.0103615029742666));
#30158=CARTESIAN_POINT('Ctrl Pts',(-0.0108497517033239,-0.0357017448667069,
-0.0113879302746));
#30159=CARTESIAN_POINT('Ctrl Pts',(-0.010945346434419,-0.0356221681343902,
-0.0131387543260284));
#30160=CARTESIAN_POINT('Ctrl Pts',(-0.012470251992075,-0.0355425914020735,
-0.0140043085907352));
#30161=CARTESIAN_POINT('Ctrl Pts',(-0.0140225104888412,-0.0354630146697568,
-0.0131888170585244));
#30162=CARTESIAN_POINT('Ctrl Pts',(-0.0141750019870238,-0.0353834379374401,
-0.0114420276670381));
#30163=CARTESIAN_POINT('Ctrl Pts',(-0.0127875314436345,-0.0353038612051234,
-0.0103699024202048));
#30164=CARTESIAN_POINT('Ctrl Pts',(-0.0111357098566257,-0.0352242844728067,
-0.0109581319803875));
#30165=CARTESIAN_POINT('Ctrl Pts',(-0.0107381892442877,-0.03514470774049,
-0.0126659097821878));
#30166=CARTESIAN_POINT('Ctrl Pts',(-0.0119604416488503,-0.0350651310081733,
-0.0139231396018729));
#30167=CARTESIAN_POINT('Ctrl Pts',(-0.0136787531423359,-0.0349855542758566,
-0.0135739497373915));
#30168=CARTESIAN_POINT('Ctrl Pts',(-0.0143133428273887,-0.0349059775435399,
-0.0119393783113244));
#30169=CARTESIAN_POINT('Ctrl Pts',(-0.0132807818460022,-0.0348264008112232,
-0.0105222171845282));
#30170=CARTESIAN_POINT('Ctrl Pts',(-0.0115303858334339,-0.0347468240789065,
-0.010625375614492));
#30171=CARTESIAN_POINT('Ctrl Pts',(-0.0106714334602556,-0.0346672473465898,
-0.0121540118248493));
#30172=CARTESIAN_POINT('Ctrl Pts',(-0.0114936281414464,-0.0345876706142731,
-0.0137027286336875));
#30173=CARTESIAN_POINT('Ctrl Pts',(-0.0132410607364181,-0.0345080938819564,
-0.0138476671599599));
#30174=CARTESIAN_POINT('Ctrl Pts',(-0.0143071770926239,-0.0344285171496397,
-0.0124555738575412));
#30175=CARTESIAN_POINT('Ctrl Pts',(-0.0137118114169886,-0.0343489404173231,
-0.010806311125067));
#30176=CARTESIAN_POINT('Ctrl Pts',(-0.0120023308578284,-0.0342693636850063,
-0.0104161777291886));
#30177=CARTESIAN_POINT('Ctrl Pts',(-0.0107503972326347,-0.0341897869526896,
-0.0116438544156386));
#30178=CARTESIAN_POINT('Ctrl Pts',(-0.011107012970546,-0.0341102102203729,
-0.0133606400935724));
#30179=CARTESIAN_POINT('Ctrl Pts',(-0.0127443127819797,-0.0340306334880562,
-0.0139881567674452));
#30180=CARTESIAN_POINT('Ctrl Pts',(-0.0141569963678234,-0.0339510567557395,
-0.0129494783115481));
#30181=CARTESIAN_POINT('Ctrl Pts',(-0.0140462710394181,-0.0338714800234228,
-0.0111995446699121));
#30182=CARTESIAN_POINT('Ctrl Pts',(-0.012513935422026,-0.0337919032911062,
-0.0103472094048007));
#30183=CARTESIAN_POINT('Ctrl Pts',(-0.0109687878597513,-0.0337123265587894,
-0.0111760923032072));
#30184=CARTESIAN_POINT('Ctrl Pts',(-0.0108314057394338,-0.0336327498264727,
-0.0129241352092867));
#30185=CARTESIAN_POINT('Ctrl Pts',(-0.0122280954011582,-0.033553173094156,
-0.0139842228647708));
#30186=CARTESIAN_POINT('Ctrl Pts',(-0.0138747686462785,-0.0334735963618394,
-0.0133817321409568));
#30187=CARTESIAN_POINT('Ctrl Pts',(-0.0142575074305579,-0.0333940196295226,
-0.0116705808117385));
#30188=CARTESIAN_POINT('Ctrl Pts',(-0.0130244294643756,-0.0333144428972059,
-0.0104239667664972));
#30189=CARTESIAN_POINT('Ctrl Pts',(-0.0113092016658568,-0.0332348661648893,
-0.0107880017204034));
#30190=CARTESIAN_POINT('Ctrl Pts',(-0.0106887697477285,-0.0331552894325725,
-0.0124279993068177));
#30191=CARTESIAN_POINT('Ctrl Pts',(-0.0117335462547127,-0.0330757127002559,
-0.0138361789469668));
#30192=CARTESIAN_POINT('Ctrl Pts',(-0.0134829848180596,-0.0329961359679391,
-0.0137178887886596));
#30193=CARTESIAN_POINT('Ctrl Pts',(-0.0143286870404645,-0.0329165592356225,
-0.0121818824086282));
#30194=CARTESIAN_POINT('Ctrl Pts',(-0.0134931314201099,-0.0328369825033058,
-0.0106403329758275));
#30195=CARTESIAN_POINT('Ctrl Pts',(-0.0117445108783079,-0.032757405770989,
-0.0105105098297045));
#30196=CARTESIAN_POINT('Ctrl Pts',(-0.010690471739919,-0.0326778290386723,
-0.0119117697425059));
#30197=CARTESIAN_POINT('Ctrl Pts',(-0.0113000762494755,-0.0325982523063557,
-0.0135558227192634));
#30198=CARTESIAN_POINT('Ctrl Pts',(-0.0130128663625058,-0.0325186755740389,
-0.0139311597374413));
#30199=CARTESIAN_POINT('Ctrl Pts',(-0.0142541375249437,-0.0324390988417222,
-0.0126927035412902));
#30200=CARTESIAN_POINT('Ctrl Pts',(-0.0138826901599497,-0.0323595221094056,
-0.0109790656847457));
#30201=CARTESIAN_POINT('Ctrl Pts',(-0.0122400254547557,-0.0322799453770889,
-0.0103657301199557));
#30202=CARTESIAN_POINT('Ctrl Pts',(-0.010836376083328,-0.0322003686447722,
-0.0114165851482747));
#30203=CARTESIAN_POINT('Ctrl Pts',(-0.0109622288601596,-0.0321207919124554,
-0.0131654959310685));
#30204=CARTESIAN_POINT('Ctrl Pts',(-0.01250187729083,-0.0320412151801387,
-0.0140045493026142));
#30205=CARTESIAN_POINT('Ctrl Pts',(-0.014039799777464,-0.0319616384478221,
-0.0131623365783801));
#30206=CARTESIAN_POINT('Ctrl Pts',(-0.0141620615239816,-0.0318820617155053,
-0.0114131710892561));
#30207=CARTESIAN_POINT('Ctrl Pts',(-0.0127562575510713,-0.0318024849831886,
-0.0103652001677907));
#30208=CARTESIAN_POINT('Ctrl Pts',(-0.0111148555797449,-0.0317229082508719,
-0.0109819070739547));
#30209=CARTESIAN_POINT('Ctrl Pts',(-0.010746927334201,-0.0316433315185553,
-0.0126963039420751));
#30210=CARTESIAN_POINT('Ctrl Pts',(-0.0119907386284374,-0.0315637547862386,
-0.0139322090413572));
#30211=CARTESIAN_POINT('Ctrl Pts',(-0.0137027544748348,-0.0314841780539219,
-0.0135533561653636));
#30212=CARTESIAN_POINT('Ctrl Pts',(-0.0143089822891687,-0.0314046013216051,
-0.0119080551306944));
#30213=CARTESIAN_POINT('Ctrl Pts',(-0.0132520682526874,-0.0313250245892885,
-0.0105089621065284));
#30214=CARTESIAN_POINT('Ctrl Pts',(-0.0115037181928097,-0.0312454478569718,
-0.0106423754559198));
#30215=CARTESIAN_POINT('Ctrl Pts',(-0.0106713288761103,-0.0311658711246551,
-0.0121856365681985));
#30216=CARTESIAN_POINT('Ctrl Pts',(-0.0115201838829843,-0.0310862943923384,
-0.0137199044904323));
#30217=CARTESIAN_POINT('Ctrl Pts',(-0.0132698598521949,-0.0310067176600217,
-0.0138346003826415));
#30218=CARTESIAN_POINT('Ctrl Pts',(-0.0143117463657834,-0.030927140927705,
-0.0124242827927081));
#30219=CARTESIAN_POINT('Ctrl Pts',(-0.0136879420663563,-0.0308475641953883,
-0.0107855545142021));
#30220=CARTESIAN_POINT('Ctrl Pts',(-0.0119719830161943,-0.0307679874630716,
-0.0104250572679376));
#30221=CARTESIAN_POINT('Ctrl Pts',(-0.0107414430352204,-0.0306884107307549,
-0.0116741709428668));
#30222=CARTESIAN_POINT('Ctrl Pts',(-0.0111277405067114,-0.0306088339984382,
-0.0133845893474986));
#30223=CARTESIAN_POINT('Ctrl Pts',(-0.0127755584842204,-0.0305292572661215,
-0.0139835894720614));
#30224=CARTESIAN_POINT('Ctrl Pts',(-0.0141702391738808,-0.0304496805338048,
-0.0129208447123972));
#30225=CARTESIAN_POINT('Ctrl Pts',(-0.0140289409519074,-0.0303701038014881,
-0.011172687498663));
#30226=CARTESIAN_POINT('Ctrl Pts',(-0.0124827243982298,-0.0302905270691714,
-0.0103477488737881));
#30227=CARTESIAN_POINT('Ctrl Pts',(-0.0109509240039545,-0.0302109503368547,
-0.011201730797944));
#30228=CARTESIAN_POINT('Ctrl Pts',(-0.0108462080022495,-0.0301313676081364,
-0.0129550712823894));
#30229=CARTESIAN_POINT('Ctrl Pts',(-0.0117860020704321,-0.030078310456857,
-0.0136406945510677));
#30230=CARTESIAN_POINT('Ctrl Pts',(-0.0122969585536011,-0.0300517788830164,
-0.0137083808366907));
#30231=CARTESIAN_POINT('Ctrl Pts',(-0.0118688946792067,-0.0366318983236434,
-0.0134824316189254));
#30232=CARTESIAN_POINT('Ctrl Pts',(-0.0123045005756168,-0.0366053675324501,
-0.0136928469483057));
#30233=CARTESIAN_POINT('Ctrl Pts',(-0.0133950834370751,-0.0365523111638182,
-0.0136398343933247));
#30234=CARTESIAN_POINT('Ctrl Pts',(-0.0142172087271331,-0.0364727292177471,
-0.0122108315601954));
#30235=CARTESIAN_POINT('Ctrl Pts',(-0.0134563602694476,-0.0363931524854304,
-0.0107511197415665));
#30236=CARTESIAN_POINT('Ctrl Pts',(-0.0118183329091291,-0.0363135757531137,
-0.0106006226265257));
#30237=CARTESIAN_POINT('Ctrl Pts',(-0.0108059424853809,-0.0362339990207971,
-0.0118986972090865));
#30238=CARTESIAN_POINT('Ctrl Pts',(-0.0113515926781112,-0.0361544222884804,
-0.013451408779471));
#30239=CARTESIAN_POINT('Ctrl Pts',(-0.0129527745386553,-0.0360748455561636,
-0.0138314913879993));
#30240=CARTESIAN_POINT('Ctrl Pts',(-0.0141378361041622,-0.035995268823847,
-0.0126893664851646));
#30241=CARTESIAN_POINT('Ctrl Pts',(-0.0138170254269563,-0.0359156920915303,
-0.0110751526121313));
#30242=CARTESIAN_POINT('Ctrl Pts',(-0.0122854093269314,-0.0358361153592136,
-0.0104728878057866));
#30243=CARTESIAN_POINT('Ctrl Pts',(-0.0109510621433456,-0.0357565386268968,
-0.0114363016785914));
#30244=CARTESIAN_POINT('Ctrl Pts',(-0.0110407882155906,-0.0356769618945802,
-0.0130796408409835));
#30245=CARTESIAN_POINT('Ctrl Pts',(-0.0124720782528739,-0.0355973851622634,
-0.0138920578392579));
#30246=CARTESIAN_POINT('Ctrl Pts',(-0.0139290420042062,-0.0355178084299468,
-0.0131266301708478));
#30247=CARTESIAN_POINT('Ctrl Pts',(-0.0140721718924953,-0.0354382316976301,
-0.0114870779764748));
#30248=CARTESIAN_POINT('Ctrl Pts',(-0.0127698795926172,-0.0353586549653134,
-0.0104807716011009));
#30249=CARTESIAN_POINT('Ctrl Pts',(-0.0112194650315414,-0.0352790782329967,
-0.0110328891436582));
#30250=CARTESIAN_POINT('Ctrl Pts',(-0.0108463486183986,-0.0351995015006799,
-0.012635824709955));
#30251=CARTESIAN_POINT('Ctrl Pts',(-0.0119935656909004,-0.0351199247683633,
-0.0138158718980947));
#30252=CARTESIAN_POINT('Ctrl Pts',(-0.0136063882747172,-0.0350403480360466,
-0.0134881191584951));
#30253=CARTESIAN_POINT('Ctrl Pts',(-0.0142020198464027,-0.0349607713037299,
-0.011953895753241));
#30254=CARTESIAN_POINT('Ctrl Pts',(-0.0132328488455326,-0.0348811945714132,
-0.0106237356054045));
#30255=CARTESIAN_POINT('Ctrl Pts',(-0.011589911444255,-0.0348016178390965,
-0.0107205610332662));
#30256=CARTESIAN_POINT('Ctrl Pts',(-0.0107836910405988,-0.0347220411067798,
-0.0121553526946449));
#30257=CARTESIAN_POINT('Ctrl Pts',(-0.0115554103447796,-0.0346424643744631,
-0.0136089921859133));
#30258=CARTESIAN_POINT('Ctrl Pts',(-0.0131955662557146,-0.0345628876421464,
-0.0137450327870055));
#30259=CARTESIAN_POINT('Ctrl Pts',(-0.014196232632436,-0.0344833109098297,
-0.0124384015240285));
#30260=CARTESIAN_POINT('Ctrl Pts',(-0.0136374170678924,-0.034403734177513,
-0.010890388726776));
#30261=CARTESIAN_POINT('Ctrl Pts',(-0.0120328832782612,-0.0343241574451963,
-0.0105242060212774));
#30262=CARTESIAN_POINT('Ctrl Pts',(-0.0108578071457864,-0.0342445807128796,
-0.0116765143734234));
#30263=CARTESIAN_POINT('Ctrl Pts',(-0.0111925298768096,-0.0341650039805629,
-0.0132879048130742));
#30264=CARTESIAN_POINT('Ctrl Pts',(-0.0127293141690466,-0.0340854272482462,
-0.01387689759301));
#30265=CARTESIAN_POINT('Ctrl Pts',(-0.0140552716567745,-0.0340058505159295,
-0.0129019846756805));
#30266=CARTESIAN_POINT('Ctrl Pts',(-0.0139513438701481,-0.0339262737836128,
-0.0112594812599081));
#30267=CARTESIAN_POINT('Ctrl Pts',(-0.0125130799121368,-0.0338466970512961,
-0.0104594717332497));
#30268=CARTESIAN_POINT('Ctrl Pts',(-0.0110627905477149,-0.0337671203189794,
-0.0112374686581132));
#30269=CARTESIAN_POINT('Ctrl Pts',(-0.0109338424570453,-0.0336875435866627,
-0.0128781974125294));
#30270=CARTESIAN_POINT('Ctrl Pts',(-0.0122447879041034,-0.033607966854346,
-0.0138732051966662));
#30271=CARTESIAN_POINT('Ctrl Pts',(-0.0137903701852936,-0.0335283901220293,
-0.013307701997979));
#30272=CARTESIAN_POINT('Ctrl Pts',(-0.0141496122420036,-0.0334488133897126,
-0.0117016000085817));
#30273=CARTESIAN_POINT('Ctrl Pts',(-0.0129922342002428,-0.0333692366573959,
-0.0105315168815755));
#30274=CARTESIAN_POINT('Ctrl Pts',(-0.0113823060001877,-0.0332896599250792,
-0.0108732033552937));
#30275=CARTESIAN_POINT('Ctrl Pts',(-0.0107999630355553,-0.0332100831927625,
-0.0124125198033311));
#30276=CARTESIAN_POINT('Ctrl Pts',(-0.0117805996383446,-0.0331305064604458,
-0.0137342498472222));
#30277=CARTESIAN_POINT('Ctrl Pts',(-0.0134226383691933,-0.0330509297281291,
-0.0136232216433812));
#30278=CARTESIAN_POINT('Ctrl Pts',(-0.0142164220624582,-0.0329713529958124,
-0.012181512274624));
#30279=CARTESIAN_POINT('Ctrl Pts',(-0.0134321620609091,-0.0328917762634957,
-0.0107346001468076));
#30280=CARTESIAN_POINT('Ctrl Pts',(-0.0117908911324214,-0.0328121995311791,
-0.010612746977133));
#30281=CARTESIAN_POINT('Ctrl Pts',(-0.010801560540695,-0.0327326227988623,
-0.0119279821028546));
#30282=CARTESIAN_POINT('Ctrl Pts',(-0.0113737408025024,-0.0326530460665456,
-0.0134711049766514));
#30283=CARTESIAN_POINT('Ctrl Pts',(-0.012981380969088,-0.0325734693342289,
-0.0138233996692927));
#30284=CARTESIAN_POINT('Ctrl Pts',(-0.0141464492183606,-0.0324938926019122,
-0.0126609735726318));
#30285=CARTESIAN_POINT('Ctrl Pts',(-0.0137978053890942,-0.0324143158695955,
-0.0110525377063779));
#30286=CARTESIAN_POINT('Ctrl Pts',(-0.0122559855594419,-0.0323347391372789,
-0.0104768554426548));
#30287=CARTESIAN_POINT('Ctrl Pts',(-0.0109385076664164,-0.0322551624049621,
-0.011463197400103));
#30288=CARTESIAN_POINT('Ctrl Pts',(-0.0110566342118533,-0.0321755856726455,
-0.0131047407513895));
#30289=CARTESIAN_POINT('Ctrl Pts',(-0.0125017620420153,-0.0320960089403287,
-0.013892283773587));
#30290=CARTESIAN_POINT('Ctrl Pts',(-0.0139452698856203,-0.032016432208012,
-0.0131017753546116));
#30291=CARTESIAN_POINT('Ctrl Pts',(-0.0140600258577871,-0.0319368554756953,
-0.0114599929336785));
#30292=CARTESIAN_POINT('Ctrl Pts',(-0.0127405256364799,-0.0318572787433787,
-0.0104763580247982));
#30293=CARTESIAN_POINT('Ctrl Pts',(-0.0111998910201647,-0.0317777020110619,
-0.0110552046597814));
#30294=CARTESIAN_POINT('Ctrl Pts',(-0.010854550267986,-0.0316981252787452,
-0.0126643529411099));
#30295=CARTESIAN_POINT('Ctrl Pts',(-0.0120220027077538,-0.0316185485464285,
-0.0138243845553623));
#30296=CARTESIAN_POINT('Ctrl Pts',(-0.0136289161407313,-0.0315389718141119,
-0.013468789847032));
#30297=CARTESIAN_POINT('Ctrl Pts',(-0.0141979270061085,-0.0314593950817952,
-0.0119244955348821));
#30298=CARTESIAN_POINT('Ctrl Pts',(-0.01320589800924,-0.0313798183494785,
-0.0106112942702744));
#30299=CARTESIAN_POINT('Ctrl Pts',(-0.0115648809575133,-0.0313002416171617,
-0.0107365172369465));
#30300=CARTESIAN_POINT('Ctrl Pts',(-0.0107835928769817,-0.031220664884845,
-0.0121850359624776));
#30301=CARTESIAN_POINT('Ctrl Pts',(-0.011580335802035,-0.0311410881525283,
-0.0136251135991492));
#30302=CARTESIAN_POINT('Ctrl Pts',(-0.0132225973641571,-0.0310615114202117,
-0.0137327681925843));
#30303=CARTESIAN_POINT('Ctrl Pts',(-0.0142005213932173,-0.0309819346878949,
-0.0124090314498447));
#30304=CARTESIAN_POINT('Ctrl Pts',(-0.0136150130812423,-0.0309023579555782,
-0.0108709063855978));
#30305=CARTESIAN_POINT('Ctrl Pts',(-0.0120043985218343,-0.0308227812232616,
-0.0105325404360109));
#30306=CARTESIAN_POINT('Ctrl Pts',(-0.0108494026557598,-0.0307432044909448,
-0.0117049697378681));
#30307=CARTESIAN_POINT('Ctrl Pts',(-0.0112119849282138,-0.0306636277586282,
-0.0133103837976729));
#30308=CARTESIAN_POINT('Ctrl Pts',(-0.0127586416654942,-0.0305840510263114,
-0.0138726106885867));
#30309=CARTESIAN_POINT('Ctrl Pts',(-0.0140677014733492,-0.0305044742939948,
-0.0128751089226279));
#30310=CARTESIAN_POINT('Ctrl Pts',(-0.0139350776945317,-0.030424897561678,
-0.0112342728780215));
#30311=CARTESIAN_POINT('Ctrl Pts',(-0.0124837849651884,-0.0303453208293614,
-0.0104599780836811));
#30312=CARTESIAN_POINT('Ctrl Pts',(-0.0110460233723964,-0.0302657440970446,
-0.0112615331792919));
#30313=CARTESIAN_POINT('Ctrl Pts',(-0.0109477359937244,-0.0301861613683264,
-0.01290723428829));
#30314=CARTESIAN_POINT('Ctrl Pts',(-0.0118298351375922,-0.0301331042170469,
-0.0135507664394204));
#30315=CARTESIAN_POINT('Ctrl Pts',(-0.0123094234768001,-0.0301065726432064,
-0.0136142973943615));
#30316=CARTESIAN_POINT('Ctrl Pts',(-0.0119101730025912,-0.0366866920838333,
-0.013396973041484));
#30317=CARTESIAN_POINT('Ctrl Pts',(-0.012317287488031,-0.0366601612926402,
-0.0135936258628881));
#30318=CARTESIAN_POINT('Ctrl Pts',(-0.0133365392569605,-0.036607104924008,
-0.013544080667975));
#30319=CARTESIAN_POINT('Ctrl Pts',(-0.0141048922962269,-0.0365275229779372,
-0.0122085437574418));
#30320=CARTESIAN_POINT('Ctrl Pts',(-0.0133938081926804,-0.0364479462456204,
-0.0108443064254199));
#30321=CARTESIAN_POINT('Ctrl Pts',(-0.011862918295578,-0.0363683695133038,
-0.0107036527840094));
#30322=CARTESIAN_POINT('Ctrl Pts',(-0.0109167446789555,-0.0362887927809871,
-0.0119168249887406));
#30323=CARTESIAN_POINT('Ctrl Pts',(-0.0114267058600925,-0.0362092160486704,
-0.0133679792940958));
#30324=CARTESIAN_POINT('Ctrl Pts',(-0.0129231601887028,-0.0361296393163537,
-0.0137232020697075));
#30325=CARTESIAN_POINT('Ctrl Pts',(-0.0140307111503216,-0.0360500625840369,
-0.0126557794384769));
#30326=CARTESIAN_POINT('Ctrl Pts',(-0.0137308835427282,-0.0359704858517202,
-0.0111471454743235));
#30327=CARTESIAN_POINT('Ctrl Pts',(-0.0122994449290827,-0.0358909091194036,
-0.0105842726373068));
#30328=CARTESIAN_POINT('Ctrl Pts',(-0.0110523725833671,-0.0358113323870868,
-0.0114846730825829));
#30329=CARTESIAN_POINT('Ctrl Pts',(-0.0111362299967622,-0.0357317556547701,
-0.0130205273559385));
#30330=CARTESIAN_POINT('Ctrl Pts',(-0.0124739045136727,-0.0356521789224534,
-0.0137798070877806));
#30331=CARTESIAN_POINT('Ctrl Pts',(-0.013835573519571,-0.0355726021901367,
-0.0130644432831712));
#30332=CARTESIAN_POINT('Ctrl Pts',(-0.013969341797967,-0.0354930254578201,
-0.0115321282859115));
#30333=CARTESIAN_POINT('Ctrl Pts',(-0.0127522277415997,-0.0354134487255034,
-0.0105916407819971));
#30334=CARTESIAN_POINT('Ctrl Pts',(-0.011303220206457,-0.0353338719931866,
-0.0111076463069289));
#30335=CARTESIAN_POINT('Ctrl Pts',(-0.0109545079925095,-0.03525429526087,
-0.0126057396377221));
#30336=CARTESIAN_POINT('Ctrl Pts',(-0.0120266897329506,-0.0351747185285532,
-0.0137086041943165));
#30337=CARTESIAN_POINT('Ctrl Pts',(-0.0135340234070985,-0.0350951417962365,
-0.0134022885795985));
#30338=CARTESIAN_POINT('Ctrl Pts',(-0.0140906968654169,-0.0350155650639198,
-0.0119684131951576));
#30339=CARTESIAN_POINT('Ctrl Pts',(-0.0131849158450631,-0.0349359883316031,
-0.0107252540262807));
#30340=CARTESIAN_POINT('Ctrl Pts',(-0.0116494370550759,-0.0348564115992864,
-0.0108157464520407));
#30341=CARTESIAN_POINT('Ctrl Pts',(-0.010895948620942,-0.0347768348669697,
-0.0121566935644407));
#30342=CARTESIAN_POINT('Ctrl Pts',(-0.0116171925481127,-0.0346972581346531,
-0.0135152557381391));
#30343=CARTESIAN_POINT('Ctrl Pts',(-0.013150071775011,-0.0346176814023364,
-0.0136423984140509));
#30344=CARTESIAN_POINT('Ctrl Pts',(-0.0140852881722481,-0.0345381046700197,
-0.0124212291905156));
#30345=CARTESIAN_POINT('Ctrl Pts',(-0.0135630227187962,-0.0344585279377029,
-0.0109744663284849));
#30346=CARTESIAN_POINT('Ctrl Pts',(-0.012063435698694,-0.0343789512053863,
-0.0106322343133662));
#30347=CARTESIAN_POINT('Ctrl Pts',(-0.0109652170589382,-0.0342993744730696,
-0.0117091743312082));
#30348=CARTESIAN_POINT('Ctrl Pts',(-0.0112780467830731,-0.0342197977407528,
-0.013215169532576));
#30349=CARTESIAN_POINT('Ctrl Pts',(-0.0127143155561136,-0.0341402210084361,
-0.0137656384185746));
#30350=CARTESIAN_POINT('Ctrl Pts',(-0.0139535469457255,-0.0340606442761194,
-0.0128544910398128));
#30351=CARTESIAN_POINT('Ctrl Pts',(-0.0138564167008781,-0.0339810675438028,
-0.011319417849904));
#30352=CARTESIAN_POINT('Ctrl Pts',(-0.0125122244022477,-0.0339014908114861,
-0.0105717340616986));
#30353=CARTESIAN_POINT('Ctrl Pts',(-0.0111567932356787,-0.0338219140791693,
-0.0112988450130191));
#30354=CARTESIAN_POINT('Ctrl Pts',(-0.0110362791746569,-0.0337423373468527,
-0.0128322596157721));
#30355=CARTESIAN_POINT('Ctrl Pts',(-0.0122614804070487,-0.033662760614536,
-0.0137621875285618));
#30356=CARTESIAN_POINT('Ctrl Pts',(-0.0137059717243087,-0.0335831838822193,
-0.013233671855001));
#30357=CARTESIAN_POINT('Ctrl Pts',(-0.0140417170534496,-0.0335036071499025,
-0.011732619205425));
#30358=CARTESIAN_POINT('Ctrl Pts',(-0.01296003893611,-0.0334240304175859,
-0.0106390669966539));
#30359=CARTESIAN_POINT('Ctrl Pts',(-0.0114554103345184,-0.0333444536852691,
-0.0109584049901842));
#30360=CARTESIAN_POINT('Ctrl Pts',(-0.0109111563233822,-0.0332648769529525,
-0.0123970402998445));
#30361=CARTESIAN_POINT('Ctrl Pts',(-0.0118276530219764,-0.0331853002206357,
-0.0136323207474776));
#30362=CARTESIAN_POINT('Ctrl Pts',(-0.0133622919203268,-0.0331057234883191,
-0.0135285544981027));
#30363=CARTESIAN_POINT('Ctrl Pts',(-0.0141041570844519,-0.0330261467560024,
-0.0121811421406199));
#30364=CARTESIAN_POINT('Ctrl Pts',(-0.0133711927017082,-0.0329465700236857,
-0.0108288673177876));
#30365=CARTESIAN_POINT('Ctrl Pts',(-0.0118372713865348,-0.032866993291369,
-0.0107149841245616));
#30366=CARTESIAN_POINT('Ctrl Pts',(-0.010912649341471,-0.0327874165590523,
-0.011944194463203));
#30367=CARTESIAN_POINT('Ctrl Pts',(-0.0114474053555292,-0.0327078398267356,
-0.0133863872340393));
#30368=CARTESIAN_POINT('Ctrl Pts',(-0.0129498955756703,-0.0326282630944189,
-0.0137156396011444));
#30369=CARTESIAN_POINT('Ctrl Pts',(-0.0140387609117777,-0.0325486863621022,
-0.0126292436039734));
#30370=CARTESIAN_POINT('Ctrl Pts',(-0.0137129206182386,-0.0324691096297855,
-0.0111260097280104));
#30371=CARTESIAN_POINT('Ctrl Pts',(-0.0122719456641281,-0.0323895328974688,
-0.010587980765354));
#30372=CARTESIAN_POINT('Ctrl Pts',(-0.0110406392495048,-0.0323099561651521,
-0.0115098096519313));
#30373=CARTESIAN_POINT('Ctrl Pts',(-0.0111510395635473,-0.0322303794328354,
-0.0130439855717105));
#30374=CARTESIAN_POINT('Ctrl Pts',(-0.0125016467932006,-0.0321508027005187,
-0.0137800182445599));
#30375=CARTESIAN_POINT('Ctrl Pts',(-0.0138507399937766,-0.032071225968202,
-0.0130412141308432));
#30376=CARTESIAN_POINT('Ctrl Pts',(-0.0139579901915926,-0.0319916492358853,
-0.011506814778101));
#30377=CARTESIAN_POINT('Ctrl Pts',(-0.0127247937218885,-0.0319120725035686,
-0.0105875158818058));
#30378=CARTESIAN_POINT('Ctrl Pts',(-0.0112849264605842,-0.0318324957712519,
-0.0111285022456082));
#30379=CARTESIAN_POINT('Ctrl Pts',(-0.0109621732017711,-0.0317529190389352,
-0.0126324019401447));
#30380=CARTESIAN_POINT('Ctrl Pts',(-0.0120532667870702,-0.0316733423066185,
-0.0137165600693672));
#30381=CARTESIAN_POINT('Ctrl Pts',(-0.013555077806628,-0.0315937655743018,
-0.0133842235287005));
#30382=CARTESIAN_POINT('Ctrl Pts',(-0.0140868717230483,-0.0315141888419851,
-0.0119409359390699));
#30383=CARTESIAN_POINT('Ctrl Pts',(-0.0131597277657927,-0.0314346121096684,
-0.0107136264340204));
#30384=CARTESIAN_POINT('Ctrl Pts',(-0.0116260437222168,-0.0313550353773517,
-0.0108306590179733));
#30385=CARTESIAN_POINT('Ctrl Pts',(-0.0108958568778532,-0.031275458645035,
-0.0121844353567568));
#30386=CARTESIAN_POINT('Ctrl Pts',(-0.0116404877210857,-0.0311958819127183,
-0.0135303227078661));
#30387=CARTESIAN_POINT('Ctrl Pts',(-0.0131753348761194,-0.0311163051804016,
-0.0136309360025271));
#30388=CARTESIAN_POINT('Ctrl Pts',(-0.0140892964206512,-0.0310367284480849,
-0.0123937801069812));
#30389=CARTESIAN_POINT('Ctrl Pts',(-0.0135420840961283,-0.0309571517157682,
-0.0109562582569936));
#30390=CARTESIAN_POINT('Ctrl Pts',(-0.0120368140274742,-0.0308775749834515,
-0.0106400236040845));
#30391=CARTESIAN_POINT('Ctrl Pts',(-0.0109573622762991,-0.0307979982511348,
-0.0117357685328693));
#30392=CARTESIAN_POINT('Ctrl Pts',(-0.0112962293497164,-0.0307184215188181,
-0.013236178247847));
#30393=CARTESIAN_POINT('Ctrl Pts',(-0.012741724846768,-0.0306388447865014,
-0.0137616319051119));
#30394=CARTESIAN_POINT('Ctrl Pts',(-0.0139651637728177,-0.0305592680541847,
-0.0128293731328584));
#30395=CARTESIAN_POINT('Ctrl Pts',(-0.013841214437156,-0.030479691321868,
-0.0112958582573798));
#30396=CARTESIAN_POINT('Ctrl Pts',(-0.012484845532147,-0.0304001145895513,
-0.0105722072935741));
#30397=CARTESIAN_POINT('Ctrl Pts',(-0.0111411227408385,-0.0303205378572346,
-0.0113213355606397));
#30398=CARTESIAN_POINT('Ctrl Pts',(-0.0110492639851992,-0.0302409551285162,
-0.0128593972941908));
#30399=CARTESIAN_POINT('Ctrl Pts',(-0.0118736682047523,-0.0301878979772368,
-0.0134608383277731));
#30400=CARTESIAN_POINT('Ctrl Pts',(-0.012321888399999,-0.0301613664033963,
-0.0135202139520323));
#30401=CARTESIAN_POINT('Ctrl Pts',(-0.0119514513259758,-0.0367414858440234,
-0.0133115144640425));
#30402=CARTESIAN_POINT('Ctrl Pts',(-0.0123300744004454,-0.0367149550528302,
-0.0134944047774705));
#30403=CARTESIAN_POINT('Ctrl Pts',(-0.013277995076846,-0.0366618986841981,
-0.0134483269426253));
#30404=CARTESIAN_POINT('Ctrl Pts',(-0.0139925758653207,-0.0365823167381272,
-0.0122062559546884));
#30405=CARTESIAN_POINT('Ctrl Pts',(-0.0133312561159133,-0.0365027400058105,
-0.0109374931092734));
#30406=CARTESIAN_POINT('Ctrl Pts',(-0.011907503682027,-0.0364231632734937,
-0.0108066829414929));
#30407=CARTESIAN_POINT('Ctrl Pts',(-0.01102754687253,-0.036343586541177,
-0.0119349527683947));
#30408=CARTESIAN_POINT('Ctrl Pts',(-0.0115018190420739,-0.0362640098088604,
-0.0132845498087204));
#30409=CARTESIAN_POINT('Ctrl Pts',(-0.0128935458387502,-0.0361844330765436,
-0.0136149127514156));
#30410=CARTESIAN_POINT('Ctrl Pts',(-0.013923586196481,-0.0361048563442269,
-0.0126221923917892));
#30411=CARTESIAN_POINT('Ctrl Pts',(-0.0136447416585,-0.0360252796119103,
-0.0112191383365156));
#30412=CARTESIAN_POINT('Ctrl Pts',(-0.0123134805312341,-0.0359457028795936,
-0.0106956574688269));
#30413=CARTESIAN_POINT('Ctrl Pts',(-0.0111536830233888,-0.0358661261472768,
-0.0115330444865743));
#30414=CARTESIAN_POINT('Ctrl Pts',(-0.0112316717779339,-0.0357865494149602,
-0.0129614138708936));
#30415=CARTESIAN_POINT('Ctrl Pts',(-0.0124757307744716,-0.0357069726826434,
-0.0136675563363033));
#30416=CARTESIAN_POINT('Ctrl Pts',(-0.0137421050349358,-0.0356273959503267,
-0.0130022563954946));
#30417=CARTESIAN_POINT('Ctrl Pts',(-0.0138665117034386,-0.03554781921801,
-0.0115771785953483));
#30418=CARTESIAN_POINT('Ctrl Pts',(-0.0127345758905823,-0.0354682424856935,
-0.0107025099628932));
#30419=CARTESIAN_POINT('Ctrl Pts',(-0.0113869753813728,-0.0353886657533766,
-0.0111824034701997));
#30420=CARTESIAN_POINT('Ctrl Pts',(-0.0110626673666204,-0.0353090890210599,
-0.0125756545654891));
#30421=CARTESIAN_POINT('Ctrl Pts',(-0.0120598137750008,-0.0352295122887433,
-0.0136013364905383));
#30422=CARTESIAN_POINT('Ctrl Pts',(-0.0134616585394798,-0.0351499355564267,
-0.0133164580007021));
#30423=CARTESIAN_POINT('Ctrl Pts',(-0.0139793738844311,-0.0350703588241098,
-0.0119829306370743));
#30424=CARTESIAN_POINT('Ctrl Pts',(-0.0131369828445936,-0.0349907820917932,
-0.010826772447157));
#30425=CARTESIAN_POINT('Ctrl Pts',(-0.011708962665897,-0.0349112053594765,
-0.0109109318708149));
#30426=CARTESIAN_POINT('Ctrl Pts',(-0.0110082062012852,-0.0348316286271599,
-0.0121580344342364));
#30427=CARTESIAN_POINT('Ctrl Pts',(-0.0116789747514459,-0.034752051894843,
-0.0134215192903648));
#30428=CARTESIAN_POINT('Ctrl Pts',(-0.0131045772943074,-0.0346724751625264,
-0.0135397640410964));
#30429=CARTESIAN_POINT('Ctrl Pts',(-0.0139743437120601,-0.0345928984302097,
-0.0124040568570029));
#30430=CARTESIAN_POINT('Ctrl Pts',(-0.0134886283696999,-0.034513321697893,
-0.0110585439301939));
#30431=CARTESIAN_POINT('Ctrl Pts',(-0.0120939881191268,-0.0344337449655762,
-0.0107402626054551));
#30432=CARTESIAN_POINT('Ctrl Pts',(-0.01107262697209,-0.0343541682332596,
-0.0117418342889929));
#30433=CARTESIAN_POINT('Ctrl Pts',(-0.0113635636893366,-0.0342745915009429,
-0.0131424342520777));
#30434=CARTESIAN_POINT('Ctrl Pts',(-0.0126993169431805,-0.0341950147686261,
-0.0136543792441393));
#30435=CARTESIAN_POINT('Ctrl Pts',(-0.0138518222346766,-0.0341154380363095,
-0.0128069974039453));
#30436=CARTESIAN_POINT('Ctrl Pts',(-0.013761489531608,-0.0340358613039928,
-0.0113793544398999));
#30437=CARTESIAN_POINT('Ctrl Pts',(-0.0125113688923585,-0.0339562845716761,
-0.0106839963901475));
#30438=CARTESIAN_POINT('Ctrl Pts',(-0.0112507959236424,-0.0338767078393595,
-0.0113602213679251));
#30439=CARTESIAN_POINT('Ctrl Pts',(-0.0111387158922684,-0.0337971311070428,
-0.0127863218190147));
#30440=CARTESIAN_POINT('Ctrl Pts',(-0.0122781729099938,-0.0337175543747259,
-0.0136511698604572));
#30441=CARTESIAN_POINT('Ctrl Pts',(-0.0136215732633237,-0.0336379776424093,
-0.0131596417120232));
#30442=CARTESIAN_POINT('Ctrl Pts',(-0.0139338218648953,-0.0335584009100925,
-0.0117636384022682));
#30443=CARTESIAN_POINT('Ctrl Pts',(-0.0129278436719772,-0.0334788241777758,
-0.0107466171117322));
#30444=CARTESIAN_POINT('Ctrl Pts',(-0.0115285146688493,-0.0333992474454591,
-0.0110436066250744));
#30445=CARTESIAN_POINT('Ctrl Pts',(-0.0110223496112091,-0.0333196707131425,
-0.0123815607963578));
#30446=CARTESIAN_POINT('Ctrl Pts',(-0.0118747064056083,-0.0332400939808259,
-0.013530391647733));
#30447=CARTESIAN_POINT('Ctrl Pts',(-0.0133019454714604,-0.0331605172485091,
-0.0134338873528243));
#30448=CARTESIAN_POINT('Ctrl Pts',(-0.0139918921064455,-0.0330809405161923,
-0.0121807720066158));
#30449=CARTESIAN_POINT('Ctrl Pts',(-0.0133102233425074,-0.0330013637838758,
-0.0109231344887676));
#30450=CARTESIAN_POINT('Ctrl Pts',(-0.0118836516406484,-0.0329217870515589,
-0.0108172212719902));
#30451=CARTESIAN_POINT('Ctrl Pts',(-0.011023738142247,-0.0328422103192422,
-0.0119604068235517));
#30452=CARTESIAN_POINT('Ctrl Pts',(-0.0115210699085561,-0.0327626335869256,
-0.0133016694914273));
#30453=CARTESIAN_POINT('Ctrl Pts',(-0.0129184101822527,-0.0326830568546089,
-0.0136078795329958));
#30454=CARTESIAN_POINT('Ctrl Pts',(-0.0139310726051947,-0.0326034801222921,
-0.0125975136353148));
#30455=CARTESIAN_POINT('Ctrl Pts',(-0.0136280358473832,-0.0325239033899755,
-0.0111994817496426));
#30456=CARTESIAN_POINT('Ctrl Pts',(-0.0122879057688142,-0.0324443266576589,
-0.0106991060880532));
#30457=CARTESIAN_POINT('Ctrl Pts',(-0.0111427708325933,-0.0323647499253422,
-0.0115564219037597));
#30458=CARTESIAN_POINT('Ctrl Pts',(-0.011245444915241,-0.0322851731930254,
-0.0129832303920315));
#30459=CARTESIAN_POINT('Ctrl Pts',(-0.0125015315443861,-0.0322055964607087,
-0.0136677527155328));
#30460=CARTESIAN_POINT('Ctrl Pts',(-0.0137562101019329,-0.0321260197283921,
-0.0129806529070748));
#30461=CARTESIAN_POINT('Ctrl Pts',(-0.0138559545253982,-0.0320464429960753,
-0.0115536366225233));
#30462=CARTESIAN_POINT('Ctrl Pts',(-0.0127090618072971,-0.0319668662637586,
-0.0106986737388134));
#30463=CARTESIAN_POINT('Ctrl Pts',(-0.0113699619010038,-0.0318872895314419,
-0.0112017998314348));
#30464=CARTESIAN_POINT('Ctrl Pts',(-0.0110697961355561,-0.0318077127991252,
-0.0126004509391794));
#30465=CARTESIAN_POINT('Ctrl Pts',(-0.0120845308663866,-0.0317281360668085,
-0.0136087355833722));
#30466=CARTESIAN_POINT('Ctrl Pts',(-0.0134812394725246,-0.0316485593344919,
-0.0132996572103688));
#30467=CARTESIAN_POINT('Ctrl Pts',(-0.0139758164399881,-0.0315689826021751,
-0.0119573763432578));
#30468=CARTESIAN_POINT('Ctrl Pts',(-0.0131135575223454,-0.0314894058698584,
-0.0108159585977663));
#30469=CARTESIAN_POINT('Ctrl Pts',(-0.0116872064869202,-0.0314098291375418,
-0.010924800799));
#30470=CARTESIAN_POINT('Ctrl Pts',(-0.0110081208787246,-0.031330252405225,
-0.0121838347510359));
#30471=CARTESIAN_POINT('Ctrl Pts',(-0.0117006396401363,-0.0312506756729083,
-0.0134355318165829));
#30472=CARTESIAN_POINT('Ctrl Pts',(-0.0131280723880818,-0.0311710989405916,
-0.0135291038124697));
#30473=CARTESIAN_POINT('Ctrl Pts',(-0.013978071448085,-0.031091522208275,
-0.0123785287641178));
#30474=CARTESIAN_POINT('Ctrl Pts',(-0.0134691551110141,-0.0310119454759582,
-0.0110416101283893));
#30475=CARTESIAN_POINT('Ctrl Pts',(-0.0120692295331141,-0.0309323687436415,
-0.0107475067721579));
#30476=CARTESIAN_POINT('Ctrl Pts',(-0.0110653218968386,-0.0308527920113249,
-0.0117665673278705));
#30477=CARTESIAN_POINT('Ctrl Pts',(-0.0113804737712188,-0.0307732152790082,
-0.0131619726980214));
#30478=CARTESIAN_POINT('Ctrl Pts',(-0.0127248080280418,-0.0306936385466914,
-0.0136506531216372));
#30479=CARTESIAN_POINT('Ctrl Pts',(-0.0138626260722862,-0.0306140618143747,
-0.012783637343089));
#30480=CARTESIAN_POINT('Ctrl Pts',(-0.0137473511797801,-0.0305344850820581,
-0.0113574436367382));
#30481=CARTESIAN_POINT('Ctrl Pts',(-0.0124859060991057,-0.0304549083497413,
-0.0106844365034671));
#30482=CARTESIAN_POINT('Ctrl Pts',(-0.0112362221092804,-0.0303753316174246,
-0.0113811379419875));
#30483=CARTESIAN_POINT('Ctrl Pts',(-0.0111507919766741,-0.0302957488887063,
-0.0128115603000916));
#30484=CARTESIAN_POINT('Ctrl Pts',(-0.0119175012719124,-0.0302426917374269,
-0.0133709102161257));
#30485=CARTESIAN_POINT('Ctrl Pts',(-0.012334353323198,-0.0302161601635864,
-0.0134261305097031));
#30486=CARTESIAN_POINT('Ctrl Pts',(-0.012333636867918,-0.0302142743898723,
-0.0134293617860453));
#30487=CARTESIAN_POINT('Ctrl Pts',(-0.0121831476494517,-0.0302142743898723,
-0.013425843584848));
#30488=CARTESIAN_POINT('Ctrl Pts',(-0.0120341035714372,-0.030214274389864,
-0.0133932994687964));
#30489=CARTESIAN_POINT('Ctrl Pts',(-0.0118942833424323,-0.030214274389864,
-0.0133373140318196));
#30490=CARTESIAN_POINT('Ctrl Pts',(-0.0117668876252743,-0.030214274389864,
-0.013286303495327));
#30491=CARTESIAN_POINT('Ctrl Pts',(-0.0116469983405503,-0.030214274389864,
-0.0132157825727993));
#30492=CARTESIAN_POINT('Ctrl Pts',(-0.0115400467092915,-0.030214274389864,
-0.0131295918764286));
#30493=CARTESIAN_POINT('Ctrl Pts',(-0.011467013779984,-0.030214274389864,
-0.0130707357471586));
#30494=CARTESIAN_POINT('Ctrl Pts',(-0.0113969920402463,-0.030214274389864,
-0.0130030912482422));
#30495=CARTESIAN_POINT('Ctrl Pts',(-0.0113289969754534,-0.030214274389864,
-0.0129177922909469));
#30496=CARTESIAN_POINT('Ctrl Pts',(-0.011293993783658,-0.0302142743898639,
-0.012873881225177));
#30497=CARTESIAN_POINT('Ctrl Pts',(-0.0112601502658924,-0.0302142743898639,
-0.0128257337008467));
#30498=CARTESIAN_POINT('Ctrl Pts',(-0.0112287294385481,-0.0302142743898639,
-0.0127729949610184));
#30499=CARTESIAN_POINT('Ctrl Pts',(-0.0111686663713541,-0.0302142743898639,
-0.0126721812415285));
#30500=CARTESIAN_POINT('Ctrl Pts',(-0.0111196338579071,-0.030214274389864,
-0.0125561133975683));
#30501=CARTESIAN_POINT('Ctrl Pts',(-0.0110871847907948,-0.030214274389864,
-0.0124384291957896));
#30502=CARTESIAN_POINT('Ctrl Pts',(-0.011026262475289,-0.030214274389864,
-0.0122174800373441));
#30503=CARTESIAN_POINT('Ctrl Pts',(-0.0110174454473768,-0.0302142743898639,
-0.0119820737242676));
#30504=CARTESIAN_POINT('Ctrl Pts',(-0.0110588114931852,-0.030214274389864,
-0.0117565343966462));
#30505=CARTESIAN_POINT('Ctrl Pts',(-0.0110777497677168,-0.030214274389864,
-0.0116532775921661));
#30506=CARTESIAN_POINT('Ctrl Pts',(-0.0111143381091383,-0.0302142743898714,
-0.0115105391820177));
#30507=CARTESIAN_POINT('Ctrl Pts',(-0.0111936560887727,-0.0302142743898722,
-0.0113546716118303));
#30508=CARTESIAN_POINT('Ctrl Pts',(-0.0111983292156988,-0.0302142743898722,
-0.0113454884613957));
#30509=CARTESIAN_POINT('Ctrl Pts',(-0.0112031507400948,-0.0302142743898723,
-0.0113362652498508));
#30510=CARTESIAN_POINT('Ctrl Pts',(-0.0112081237276435,-0.0302142743898723,
-0.0113270082871182));
#30511=CARTESIAN_POINT('Origin',(0.006,-0.0355287743898723,-0.00417585328655812));
#30512=CARTESIAN_POINT('',(0.00445,-0.0355287743898723,-0.00417585328655812));
#30513=CARTESIAN_POINT('',(0.00721995334505415,-0.0364849196904892,-0.0112310978494783));
#30514=CARTESIAN_POINT('',(0.00708453011998519,-0.0366362514743427,-0.0115256574169581));
#30515=CARTESIAN_POINT('Ctrl Pts',(0.00721995334504645,-0.0364849196904987,
-0.0112310978494762));
#30516=CARTESIAN_POINT('Ctrl Pts',(0.00719897063095221,-0.0365116917012283,
-0.011283959762924));
#30517=CARTESIAN_POINT('Ctrl Pts',(0.00717654508557251,-0.0365384837930159,
-0.0113366586152459));
#30518=CARTESIAN_POINT('Ctrl Pts',(0.00715270723066132,-0.0365650012185064,
-0.0113883725609347));
#30519=CARTESIAN_POINT('Ctrl Pts',(0.00713138418908878,-0.0365887211449947,
-0.0114346308596746));
#30520=CARTESIAN_POINT('Ctrl Pts',(0.00710860625998018,-0.0366125765485143,
-0.0114808035328048));
#30521=CARTESIAN_POINT('Ctrl Pts',(0.00708453754730291,-0.0366361489012686,
-0.0115256728563643));
#30522=CARTESIAN_POINT('',(0.00700668322306563,-0.0367087073891193,-0.0114115336377739));
#30523=CARTESIAN_POINT('Ctrl Pts',(0.00708451613677846,-0.0366361698698464,
-0.0115256340934646));
#30524=CARTESIAN_POINT('Ctrl Pts',(0.00706046816155679,-0.0366597210019003,
-0.0114855239006838));
#30525=CARTESIAN_POINT('Ctrl Pts',(0.00703434025913843,-0.0366837566058097,
-0.0114470041691646));
#30526=CARTESIAN_POINT('Ctrl Pts',(0.00700646285490531,-0.0367075587304944,
-0.0114103516394692));
#30527=CARTESIAN_POINT('',(0.00671669833332503,-0.0369031264201922,-0.0108094007648104));
#30528=CARTESIAN_POINT('Ctrl Pts',(0.00700524248433158,-0.0367085996090022,
-0.0114112785004056));
#30529=CARTESIAN_POINT('Ctrl Pts',(0.00697164972371802,-0.036737221535019,
-0.0113040197252933));
#30530=CARTESIAN_POINT('Ctrl Pts',(0.00693135743213202,-0.0367690921506772,
-0.0111983546505858));
#30531=CARTESIAN_POINT('Ctrl Pts',(0.0068368208233598,-0.0368347373794732,
-0.0109973266739168));
#30532=CARTESIAN_POINT('Ctrl Pts',(0.00678126879680362,-0.0368694541553801,
-0.0108991521238439));
#30533=CARTESIAN_POINT('Ctrl Pts',(0.00671669833068704,-0.036903126420027,
-0.0108094007666463));
#30534=CARTESIAN_POINT('',(0.00634923972919489,-0.0370392946212466,-0.010672896044278));
#30535=CARTESIAN_POINT('Ctrl Pts',(0.00671669833340338,-0.0369031264186105,
-0.0108094007630884));
#30536=CARTESIAN_POINT('Ctrl Pts',(0.00668434001035949,-0.0369200006660466,
-0.0107924289650939));
#30537=CARTESIAN_POINT('Ctrl Pts',(0.00665104602607226,-0.0369359068209843,
-0.0107764344608264));
#30538=CARTESIAN_POINT('Ctrl Pts',(0.00653214916248705,-0.0369874926958288,
-0.0107245701498326));
#30539=CARTESIAN_POINT('Ctrl Pts',(0.00644209798508761,-0.0370174454481331,
-0.010694470505926));
#30540=CARTESIAN_POINT('Ctrl Pts',(0.00634919653914119,-0.0370389272884398,
-0.0106728859625448));
#30541=CARTESIAN_POINT('Ctrl Pts',(0.00634889289767975,-0.0370389974680792,
-0.010674460128291));
#30542=CARTESIAN_POINT('Ctrl Pts',(0.00628453094295314,-0.0370538664163882,
-0.0106801749938966));
#30543=CARTESIAN_POINT('Ctrl Pts',(0.00621892219545928,-0.0370646669836523,
-0.0106815858596051));
#30544=CARTESIAN_POINT('Ctrl Pts',(0.00613401119738346,-0.0370730877719417,
-0.010679137413212));
#30545=CARTESIAN_POINT('Ctrl Pts',(0.00611502706975014,-0.0370746174397915,
-0.0106783151674329));
#30546=CARTESIAN_POINT('Ctrl Pts',(0.00609289604103467,-0.0370759913228217,
-0.0106770563132658));
#30547=CARTESIAN_POINT('Ctrl Pts',(0.00608975354297057,-0.0370761767965982,
-0.0106768705011461));
#30548=CARTESIAN_POINT('Ctrl Pts',(0.00608576149263246,-0.0370764002135845,
-0.0106766255696088));
#30549=CARTESIAN_POINT('Ctrl Pts',(0.00608491202614355,-0.0370764470527918,
-0.0106765729396212));
#30550=CARTESIAN_POINT('Ctrl Pts',(0.00608355432315204,-0.037076520794857,
-0.0106764880061428));
#30551=CARTESIAN_POINT('Ctrl Pts',(0.00608304609026255,-0.0370765481478644,
-0.0106764560302396));
#30552=CARTESIAN_POINT('Ctrl Pts',(0.00608208535556954,-0.0370765993798952,
-0.0106763952402986));
#30553=CARTESIAN_POINT('Ctrl Pts',(0.00608163285407564,-0.0370766233109422,
-0.0106763664640596));
#30554=CARTESIAN_POINT('Ctrl Pts',(0.00608061127185519,-0.037076676889254,
-0.010676301172149));
#30555=CARTESIAN_POINT('Ctrl Pts',(0.00608004219029104,-0.0370767064208356,
-0.0106762645725075));
#30556=CARTESIAN_POINT('Ctrl Pts',(0.00607834196728137,-0.0370767937111384,
-0.0106761545444927));
#30557=CARTESIAN_POINT('Ctrl Pts',(0.00607721082082661,-0.0370768505416594,
-0.0106760804435228));
#30558=CARTESIAN_POINT('Ctrl Pts',(0.00606775814820463,-0.0370773150733444,
-0.01067545370425));
#30559=CARTESIAN_POINT('Ctrl Pts',(0.00605943626584679,-0.0370776567709202,
-0.0106748533872717));
#30560=CARTESIAN_POINT('Ctrl Pts',(0.00603153518532823,-0.0370785773976582,
-0.0106726813288391));
#30561=CARTESIAN_POINT('Ctrl Pts',(0.00601195864463628,-0.0370788514854428,
-0.0106708943268714));
#30562=CARTESIAN_POINT('Ctrl Pts',(0.00593170148651683,-0.0370784586746065,
-0.0106625286154495));
#30563=CARTESIAN_POINT('Ctrl Pts',(0.00587115571686308,-0.0370745767210469,
-0.0106537962981553));
#30564=CARTESIAN_POINT('Ctrl Pts',(0.00581155370696253,-0.0370672762568326,
-0.010642763081521));
#30565=CARTESIAN_POINT('',(0.0051699690934982,-0.0368386696897961,-0.0112224559460341));
#30566=CARTESIAN_POINT('Ctrl Pts',(0.00543336738962369,-0.036971489706509,
-0.0107406611507994));
#30567=CARTESIAN_POINT('Ctrl Pts',(0.00537662766820104,-0.036949204938273,
-0.0108121501534098));
#30568=CARTESIAN_POINT('Ctrl Pts',(0.00532685230785057,-0.0369258210465427,
-0.0108903032522527));
#30569=CARTESIAN_POINT('Ctrl Pts',(0.00524052614104284,-0.0368808358599697,
-0.0110513873789148));
#30570=CARTESIAN_POINT('Ctrl Pts',(0.00520302724223552,-0.0368587245012713,
-0.0111360978982334));
#30571=CARTESIAN_POINT('Ctrl Pts',(0.00517104225064472,-0.0368384801010089,
-0.0112223933179672));
#30572=CARTESIAN_POINT('',(0.00508837275154337,-0.0367823435977278,-0.0112995565278748));
#30573=CARTESIAN_POINT('Ctrl Pts',(0.00517029079620948,-0.0368380041776274,
-0.0112216295773864));
#30574=CARTESIAN_POINT('Ctrl Pts',(0.00514776779428583,-0.0368237304862038,
-0.0112412136034523));
#30575=CARTESIAN_POINT('Ctrl Pts',(0.00512627760027647,-0.0368092952781386,
-0.0112613026366608));
#30576=CARTESIAN_POINT('Ctrl Pts',(0.00509999117843507,-0.0367907315219668,
-0.0112875890585023));
#30577=CARTESIAN_POINT('Ctrl Pts',(0.00509415983457079,-0.036786552111337,
-0.0112935361211783));
#30578=CARTESIAN_POINT('Ctrl Pts',(0.00508837275129895,-0.0367823435979441,
-0.011299556527791));
#30579=CARTESIAN_POINT('',(0.00489985734136505,-0.0366206471529012,-0.0110939405679692));
#30580=CARTESIAN_POINT('Ctrl Pts',(0.00508837275077811,-0.0367823435975653,
-0.0112995565289848));
#30581=CARTESIAN_POINT('Ctrl Pts',(0.00505343997080538,-0.0367569395961701,
-0.0112717537544348));
#30582=CARTESIAN_POINT('Ctrl Pts',(0.00502114020158271,-0.0367312295393717,
-0.0112411171694515));
#30583=CARTESIAN_POINT('Ctrl Pts',(0.00499110859515615,-0.0367054808669651,
-0.0112083991960897));
#30584=CARTESIAN_POINT('Ctrl Pts',(0.00495813976451085,-0.0366772138602703,
-0.011172481259916));
#30585=CARTESIAN_POINT('Ctrl Pts',(0.00492779975572552,-0.0366488012044239,
-0.0111339368794957));
#30586=CARTESIAN_POINT('Ctrl Pts',(0.00489985734136859,-0.0366206471529081,
-0.0110939405679709));
#30587=CARTESIAN_POINT('',(0.0048020155877565,-0.0365123054509049,-0.0112033912831791));
#30588=CARTESIAN_POINT('Origin',(0.00584908854435658,-0.0356866920263109,
-0.0120603327566456));
#30589=CARTESIAN_POINT('',(0.00473550000001,-0.036425178177226,-0.0117172854002574));
#30590=CARTESIAN_POINT('Ctrl Pts',(0.00480201558775629,-0.0365123054509075,
-0.0112033912831797));
#30591=CARTESIAN_POINT('Ctrl Pts',(0.00478601756319877,-0.0364928191481298,
-0.0112873168359884));
#30592=CARTESIAN_POINT('Ctrl Pts',(0.00477251148750761,-0.0364754056904488,
-0.0113723549961358));
#30593=CARTESIAN_POINT('Ctrl Pts',(0.00475037618306168,-0.0364459871029898,
-0.0115437515601713));
#30594=CARTESIAN_POINT('Ctrl Pts',(0.00474172253563746,-0.0364339559138146,
-0.0116302694145159));
#30595=CARTESIAN_POINT('Ctrl Pts',(0.00473550000000279,-0.0364251781772399,
-0.0117172854002583));
#30596=CARTESIAN_POINT('',(0.00473549206322617,-0.0364251864739627,-0.012361204277891));
#30597=CARTESIAN_POINT('',(0.00473550000001,-0.036425178177226,-0.00417585328655812));
#30598=CARTESIAN_POINT('',(0.0049082256814125,-0.036629014744185,-0.0132662100342696));
#30599=CARTESIAN_POINT('Ctrl Pts',(0.00473551176325926,-0.0364251947706894,
-0.0123613358119503));
#30600=CARTESIAN_POINT('Ctrl Pts',(0.00473977927981908,-0.0364312145183496,
-0.0124184833562194));
#30601=CARTESIAN_POINT('Ctrl Pts',(0.0047451967074644,-0.0364387690287892,
-0.012475379285434));
#30602=CARTESIAN_POINT('Ctrl Pts',(0.00476256626397218,-0.0364623651597535,
-0.0126256583208612));
#30603=CARTESIAN_POINT('Ctrl Pts',(0.00477650468131714,-0.0364807673113787,
-0.0127187012120098));
#30604=CARTESIAN_POINT('Ctrl Pts',(0.00482227803519832,-0.0365375236924042,
-0.0129655152140196));
#30605=CARTESIAN_POINT('Ctrl Pts',(0.00486032803510807,-0.0365814856566146,
-0.0131191817101595));
#30606=CARTESIAN_POINT('Ctrl Pts',(0.00490822568140912,-0.0366290147441883,
-0.013266210034263));
#30607=CARTESIAN_POINT('',(0.00505141064578676,-0.0367547927210949,-0.013392827911221));
#30608=CARTESIAN_POINT('Origin',(0.00581953823041687,-0.0357498950543636,
-0.0123679117387863));
#30609=CARTESIAN_POINT('',(0.00532350116102365,-0.0369233529358313,-0.013244174198489));
#30610=CARTESIAN_POINT('Ctrl Pts',(0.00505164266800161,-0.0367547916698667,
-0.0133924971879909));
#30611=CARTESIAN_POINT('Ctrl Pts',(0.00509087188926385,-0.036785136527333,
-0.0133575836405446));
#30612=CARTESIAN_POINT('Ctrl Pts',(0.00513346141989738,-0.0368151056157171,
-0.0133268047857448));
#30613=CARTESIAN_POINT('Ctrl Pts',(0.00518023319210897,-0.0368442523945079,
-0.0133013178572232));
#30614=CARTESIAN_POINT('Ctrl Pts',(0.00522512071345914,-0.0368722249641455,
-0.0132768576968728));
#30615=CARTESIAN_POINT('Ctrl Pts',(0.00527254249817658,-0.0368986332982427,
-0.0132579818935523));
#30616=CARTESIAN_POINT('Ctrl Pts',(0.00532350116101516,-0.0369233529358324,
-0.013244174198484));
#30617=CARTESIAN_POINT('',(0.00550885620308809,-0.0369996744090014,-0.0133404525414052));
#30618=CARTESIAN_POINT('Ctrl Pts',(0.0053235011610258,-0.0369233529358359,
-0.0132441741984879));
#30619=CARTESIAN_POINT('Ctrl Pts',(0.0053828710383028,-0.0369521527859156,
-0.0132817693186428));
#30620=CARTESIAN_POINT('Ctrl Pts',(0.00544487207496328,-0.0369775422367839,
-0.0133141218395921));
#30621=CARTESIAN_POINT('Ctrl Pts',(0.00550913196779272,-0.036998994987575,
-0.0133411896435628));
#30622=CARTESIAN_POINT('Ctrl Pts',(0.00550973902764092,-0.0369991975191047,
-0.0133401758005509));
#30623=CARTESIAN_POINT('Ctrl Pts',(0.00557239949470718,-0.0370200894521147,
-0.0133958926875114));
#30624=CARTESIAN_POINT('Ctrl Pts',(0.0056432881507905,-0.0370392637429235,
-0.0134441367408925));
#30625=CARTESIAN_POINT('Ctrl Pts',(0.00575851694623828,-0.0370603101471249,
-0.013493473393482));
#30626=CARTESIAN_POINT('Ctrl Pts',(0.00579699572419665,-0.0370659426799965,
-0.0135059326595814));
#30627=CARTESIAN_POINT('Ctrl Pts',(0.00585469055904418,-0.0370720537271489,
-0.0135180201626379));
#30628=CARTESIAN_POINT('Ctrl Pts',(0.00587282257791823,-0.037073656915028,
-0.0135209210756684));
#30629=CARTESIAN_POINT('Ctrl Pts',(0.00589513658530892,-0.0370752283829208,
-0.0135233528248468));
#30630=CARTESIAN_POINT('Ctrl Pts',(0.00589916799537088,-0.0370754964933055,
-0.0135237473367194));
#30631=CARTESIAN_POINT('Ctrl Pts',(0.00590423872634902,-0.037075813772681,
-0.0135241868836967));
#30632=CARTESIAN_POINT('Ctrl Pts',(0.00590527310976059,-0.0370758774539166,
-0.0135242735905519));
#30633=CARTESIAN_POINT('Ctrl Pts',(0.00590690057550275,-0.0370759760088702,
-0.0135244053545441));
#30634=CARTESIAN_POINT('Ctrl Pts',(0.00590749344823749,-0.03707601156973,
-0.0135244523834596));
#30635=CARTESIAN_POINT('Ctrl Pts',(0.00590853919498026,-0.0370760736908727,
-0.0135245336210213));
#30636=CARTESIAN_POINT('Ctrl Pts',(0.00590899202748707,-0.0370761003913174,
-0.0135245682318516));
#30637=CARTESIAN_POINT('Ctrl Pts',(0.00591002705405027,-0.0370761609637588,
-0.0135246460444136));
#30638=CARTESIAN_POINT('Ctrl Pts',(0.0059106092813878,-0.0370761947075729,
-0.0135246888786905));
#30639=CARTESIAN_POINT('Ctrl Pts',(0.00591220602721993,-0.0370762863448517,
-0.013524803778942));
#30640=CARTESIAN_POINT('Ctrl Pts',(0.00591322071215222,-0.0370763435768412,
-0.0135248739487088));
#30641=CARTESIAN_POINT('Ctrl Pts',(0.00591851083039439,-0.0370766367379395,
-0.0135252249287804));
#30642=CARTESIAN_POINT('Ctrl Pts',(0.00592278981535103,-0.0370768560956537,
-0.0135254582713297));
#30643=CARTESIAN_POINT('Ctrl Pts',(0.00594514557399332,-0.0370779091031153,
-0.0135264121346295));
#30644=CARTESIAN_POINT('Ctrl Pts',(0.00596323246802831,-0.0370784437138682,
-0.0135262796754723));
#30645=CARTESIAN_POINT('Ctrl Pts',(0.00601731944718832,-0.0370790959258226,
-0.0135231506769677));
#30646=CARTESIAN_POINT('Ctrl Pts',(0.00605283405859192,-0.037078266965631,
-0.0135174708951169));
#30647=CARTESIAN_POINT('Ctrl Pts',(0.00614970529758117,-0.0370727779032569,
-0.0134922183002785));
#30648=CARTESIAN_POINT('Ctrl Pts',(0.00622246849129482,-0.0370647759109164,
-0.0134620967630096));
#30649=CARTESIAN_POINT('Ctrl Pts',(0.00630029331254413,-0.0370494071287153,
-0.0134053749986389));
#30650=CARTESIAN_POINT('',(0.00680869722628235,-0.0368513852118003,-0.0134899528977776));
#30651=CARTESIAN_POINT('Ctrl Pts',(0.00648836437726054,-0.0369998285136294,
-0.0133422410801523));
#30652=CARTESIAN_POINT('Ctrl Pts',(0.00654817215037741,-0.0369799733734263,
-0.013360182848383));
#30653=CARTESIAN_POINT('Ctrl Pts',(0.0066053348750835,-0.036956968639739,
-0.013381036200993));
#30654=CARTESIAN_POINT('Ctrl Pts',(0.00666013990064864,-0.0369311706646718,
-0.0134061770452628));
#30655=CARTESIAN_POINT('Ctrl Pts',(0.00671261604440717,-0.0369064689473686,
-0.0134302495558493));
#30656=CARTESIAN_POINT('Ctrl Pts',(0.00676176143889012,-0.0368797672711963,
-0.0134577138102791));
#30657=CARTESIAN_POINT('Ctrl Pts',(0.00680820361295115,-0.0368513880598503,
-0.0134890451831761));
#30658=CARTESIAN_POINT('',(0.0069608110048393,-0.036745056517083,-0.0133832021230568));
#30659=CARTESIAN_POINT('Origin',(0.00617971096306188,-0.0357989913886571,
-0.0124240807529343));
#30660=CARTESIAN_POINT('',(0.00710501796773384,-0.03661664768168,-0.0127892153648441));
#30661=CARTESIAN_POINT('Ctrl Pts',(0.00696081100483564,-0.036745056517089,
-0.0133832021230525));
#30662=CARTESIAN_POINT('Ctrl Pts',(0.00699435314294245,-0.0367185596585908,
-0.013288099714129));
#30663=CARTESIAN_POINT('Ctrl Pts',(0.00702288481908988,-0.0366937839905792,
-0.0131901514676876));
#30664=CARTESIAN_POINT('Ctrl Pts',(0.00704667882519898,-0.0366719994057288,
-0.013090924388801));
#30665=CARTESIAN_POINT('Ctrl Pts',(0.00707034230680265,-0.0366503343224936,
-0.0129922416304184));
#30666=CARTESIAN_POINT('Ctrl Pts',(0.00708952955233279,-0.0366314365546728,
-0.0128914214092024));
#30667=CARTESIAN_POINT('Ctrl Pts',(0.0071042246890736,-0.036616518769789,
-0.0127897291648212));
#30668=CARTESIAN_POINT('',(0.00715706304473573,-0.036560233653124,-0.0126859173614613));
#30669=CARTESIAN_POINT('Ctrl Pts',(0.00710521494511478,-0.0366155125943608,
-0.0127902311630274));
#30670=CARTESIAN_POINT('Ctrl Pts',(0.00712399117977778,-0.0365964171258507,
-0.012756454271057));
#30671=CARTESIAN_POINT('Ctrl Pts',(0.00714131329460908,-0.0365778042956974,
-0.0127216438762269));
#30672=CARTESIAN_POINT('Ctrl Pts',(0.00715705640924412,-0.0365601426392513,
-0.0126859324135836));
#30673=CARTESIAN_POINT('',(0.0072645000000106,-0.0364251781772283,-0.012945467333915));
#30674=CARTESIAN_POINT('Ctrl Pts',(0.0071570835597271,-0.0365601121792552,
-0.0126858905925983));
#30675=CARTESIAN_POINT('Ctrl Pts',(0.00717621068139738,-0.0365386529849375,
-0.0127267486831773));
#30676=CARTESIAN_POINT('Ctrl Pts',(0.00719440998528269,-0.036517030430569,
-0.0127682118485989));
#30677=CARTESIAN_POINT('Ctrl Pts',(0.00721166125580552,-0.0364954061714623,
-0.0128098344234972));
#30678=CARTESIAN_POINT('Ctrl Pts',(0.00723023900793353,-0.0364721191836949,
-0.0128546574339745));
#30679=CARTESIAN_POINT('Ctrl Pts',(0.007247849025769,-0.0364486666510824,
-0.0128999824936057));
#30680=CARTESIAN_POINT('Ctrl Pts',(0.00726450000000412,-0.0364251781772302,
-0.0129454673339182));
#30681=CARTESIAN_POINT('',(0.007264500000004,-0.0364251781772306,-0.0112916085523411));
#30682=CARTESIAN_POINT('',(0.00726450000001,-0.036425178177226,-0.00417585328655812));
#30683=CARTESIAN_POINT('Origin',(0.00607243076165687,-0.0356158716997798,
-0.0121519018301174));
#30684=CARTESIAN_POINT('Origin',(0.008,-0.0301787743898723,-0.00457585328655812));
#30685=CARTESIAN_POINT('',(0.00760000000001,-0.0297787743898623,-0.00457585328656812));
#30686=CARTESIAN_POINT('Origin',(-0.0146,-0.0301787743898723,-0.00417585328655812));
#30687=CARTESIAN_POINT('',(-0.015,-0.0301787743898623,-0.00457585328656812));
#30688=CARTESIAN_POINT('Ctrl Pts',(0.0007247979407562,-0.0405744211147313,
-0.0150948585672975));
#30689=CARTESIAN_POINT('Ctrl Pts',(-0.000237867174816089,-0.0405219330120263,
-0.015333921225633));
#30690=CARTESIAN_POINT('Ctrl Pts',(-0.00240155359114006,-0.0404169768530862,
-0.0147817233443831));
#30691=CARTESIAN_POINT('Ctrl Pts',(-0.00349898809073308,-0.0402595526379108,
-0.0115953997864184));
#30692=CARTESIAN_POINT('Ctrl Pts',(-0.00143658133088921,-0.0401021484692049,
-0.00893630820182674));
#30693=CARTESIAN_POINT('Ctrl Pts',(0.0019164823364414,-0.0399447443004989,
-0.0091940107250774));
#30694=CARTESIAN_POINT('Ctrl Pts',(0.00354474713388061,-0.0397873401317929,
-0.0121391462709199));
#30695=CARTESIAN_POINT('Ctrl Pts',(0.00197842869696902,-0.0396299359630869,
-0.0151168671994064));
#30696=CARTESIAN_POINT('Ctrl Pts',(-0.00136986320203818,-0.0394725317943809,
-0.0154451367971516));
#30697=CARTESIAN_POINT('Ctrl Pts',(-0.00348423018666191,-0.0393151276256749,
-0.0128278237290509));
#30698=CARTESIAN_POINT('Ctrl Pts',(-0.00245935806117728,-0.0391577234569689,
-0.00962318496292607));
#30699=CARTESIAN_POINT('Ctrl Pts',(0.00078120175765321,-0.0390003192882629,
-0.00871833392572952));
#30700=CARTESIAN_POINT('Ctrl Pts',(0.00331797335358058,-0.038842915119557,
-0.0109285455423723));
#30701=CARTESIAN_POINT('Ctrl Pts',(0.00286540590808132,-0.038685510950851,
-0.0142625077104432));
#30702=CARTESIAN_POINT('Ctrl Pts',(-0.000168734413497188,-0.038528106782145,
-0.0157165072437804));
#30703=CARTESIAN_POINT('Ctrl Pts',(-0.00305085839970424,-0.038370702613439,
-0.0139805591784971));
#30704=CARTESIAN_POINT('Ctrl Pts',(-0.00318431512310994,-0.038213298444733,
-0.0106186660841466));
#30705=CARTESIAN_POINT('Ctrl Pts',(-0.000448870589781203,-0.0380558942760271,
-0.0086597171282114));
#30706=CARTESIAN_POINT('Ctrl Pts',(0.00269098364593626,-0.037898490107321,
-0.00986862447417986));
#30707=CARTESIAN_POINT('Ctrl Pts',(0.00340640111752454,-0.037741085938615,
-0.0131562249345524));
#30708=CARTESIAN_POINT('Ctrl Pts',(0.00105282834073001,-0.0375836817699092,
-0.0155605615635386));
#30709=CARTESIAN_POINT('Ctrl Pts',(-0.00224928815150608,-0.0374262776012032,
-0.0149154518584878));
#30710=CARTESIAN_POINT('Ctrl Pts',(-0.00352491284701288,-0.0372688734324972,
-0.0118021062096773));
#30711=CARTESIAN_POINT('Ctrl Pts',(-0.00162477424132635,-0.0371114692637911,
-0.00902548724613536));
#30712=CARTESIAN_POINT('Ctrl Pts',(0.00173920154528507,-0.0369540650950852,
-0.00908718440036995));
#30713=CARTESIAN_POINT('Ctrl Pts',(0.0035362471012298,-0.0367966609263792,
-0.0119316117332855));
#30714=CARTESIAN_POINT('Ctrl Pts',(0.0021473177625627,-0.0366392567576732,
-0.0149960880166491));
#30715=CARTESIAN_POINT('Ctrl Pts',(-0.00117623330881229,-0.0364818525889673,
-0.0155196793445491));
#30716=CARTESIAN_POINT('Ctrl Pts',(-0.00344005928429201,-0.0363244484202613,
-0.0130306571371357));
#30717=CARTESIAN_POINT('Ctrl Pts',(-0.00260457058776481,-0.0361670442515553,
-0.00977150107506731));
#30718=CARTESIAN_POINT('Ctrl Pts',(0.000577500877143375,-0.0360096400828493,
-0.0086785414274407));
#30719=CARTESIAN_POINT('Ctrl Pts',(0.00323927405812123,-0.0358522359141433,
-0.0107364780472958));
#30720=CARTESIAN_POINT('Ctrl Pts',(0.00298262962287774,-0.0356948317454372,
-0.0140912169689667));
#30721=CARTESIAN_POINT('Ctrl Pts',(3.8790872444014E-5,-0.0355374275767314,
-0.0157203127335408));
#30722=CARTESIAN_POINT('Ctrl Pts',(-0.00293999643850483,-0.0353800234080254,
-0.014156034703666));
#30723=CARTESIAN_POINT('Ctrl Pts',(-0.00326999971823222,-0.0352226192393194,
-0.0108077161056251));
#30724=CARTESIAN_POINT('Ctrl Pts',(-0.000653903158401233,-0.0350652150706134,
-0.00869201802027602));
#30725=CARTESIAN_POINT('Ctrl Pts',(0.00255132617086471,-0.0349078109019074,
-0.00971507449258273));
#30726=CARTESIAN_POINT('Ctrl Pts',(0.0034579431850454,-0.0347504067332014,
-0.0129551647981007));
#30727=CARTESIAN_POINT('Ctrl Pts',(0.00124913306147382,-0.0345930025644954,
-0.0154931359242426));
#30728=CARTESIAN_POINT('Ctrl Pts',(-0.00208508104655071,-0.0344355983957894,
-0.0150424077569494));
#30729=CARTESIAN_POINT('Ctrl Pts',(-0.00354074547073748,-0.0342781942270835,
-0.0120090629561708));
#30730=CARTESIAN_POINT('Ctrl Pts',(-0.00180638220017174,-0.0341207900583776,
-0.00912598757588634));
#30731=CARTESIAN_POINT('Ctrl Pts',(0.0015554375747254,-0.0339633858896715,
-0.00899068273407062));
#30732=CARTESIAN_POINT('Ctrl Pts',(0.00351588891379242,-0.0338059817209656,
-0.0117250510577476));
#30733=CARTESIAN_POINT('Ctrl Pts',(0.002308707024885,-0.0336485775522596,
-0.0148655687728454));
#30734=CARTESIAN_POINT('Ctrl Pts',(-0.000978499935992214,-0.0334911733835535,
-0.0155827925774432));
#30735=CARTESIAN_POINT('Ctrl Pts',(-0.00338412929443487,-0.0333337692148475,
-0.0132305411277567));
#30736=CARTESIAN_POINT('Ctrl Pts',(-0.00274083399948854,-0.0331763650461416,
-0.00992807068529279));
#30737=CARTESIAN_POINT('Ctrl Pts',(0.000371810325715763,-0.0330189608774355,
-0.00865073566818646));
#30738=CARTESIAN_POINT('Ctrl Pts',(0.00314947285033218,-0.0328615567087297,
-0.0105493482787621));
#30739=CARTESIAN_POINT('Ctrl Pts',(0.00308962401220603,-0.0327041525400237,
-0.013913357748021));
#30740=CARTESIAN_POINT('Ctrl Pts',(0.000246184412511208,-0.0325467483713177,
-0.0157119652787973));
#30741=CARTESIAN_POINT('Ctrl Pts',(-0.0028190544326237,-0.0323893442026117,
-0.0143247209970861));
#30742=CARTESIAN_POINT('Ctrl Pts',(-0.00334447194084124,-0.0322319400339057,
-0.0110014559159814));
#30743=CARTESIAN_POINT('Ctrl Pts',(-0.000856693556614904,-0.0320745358651996,
-0.00873626699561545));
#30744=CARTESIAN_POINT('Ctrl Pts',(0.00240292033326581,-0.0319171316964937,
-0.00956995657798453));
#30745=CARTESIAN_POINT('Ctrl Pts',(0.00349762956160217,-0.0317597275277878,
-0.0127514432156497));
#30746=CARTESIAN_POINT('Ctrl Pts',(0.00144115296983182,-0.0316023233590818,
-0.015414315230305));
#30747=CARTESIAN_POINT('Ctrl Pts',(-0.00191372110484731,-0.0314449191903758,
-0.0151595752884196));
#30748=CARTESIAN_POINT('Ctrl Pts',(-0.00354444447940972,-0.0312875150216698,
-0.0122165128157948));
#30749=CARTESIAN_POINT('Ctrl Pts',(-0.00198178305265353,-0.0311301108529639,
-0.00923709863930153));
#30750=CARTESIAN_POINT('Ctrl Pts',(0.00136631424027315,-0.0309727066842579,
-0.00890480375391904));
#30751=CARTESIAN_POINT('Ctrl Pts',(0.00348352636012016,-0.0308153025155519,
-0.0115206176757296));
#30752=CARTESIAN_POINT('Ctrl Pts',(0.00246208004358717,-0.0306578983468459,
-0.014724692264453));
#30753=CARTESIAN_POINT('Ctrl Pts',(-0.000777205389354121,-0.0305004941781399,
-0.0156364595495813));
#30754=CARTESIAN_POINT('Ctrl Pts',(-0.00331711149080357,-0.030343090009434,
-0.0134221865174339));
#30755=CARTESIAN_POINT('Ctrl Pts',(-0.00301603592565593,-0.0302381538969633,
-0.0112101605671168));
#30756=CARTESIAN_POINT('Ctrl Pts',(-0.0024332353179461,-0.030185685840728,
-0.0104080043474256));
#30757=CARTESIAN_POINT('Ctrl Pts',(0.000683754430426,-0.0406727527782625,
-0.0149295625355936));
#30758=CARTESIAN_POINT('Ctrl Pts',(-0.00022439734647116,-0.0406202646755577,
-0.0151550876683166));
#30759=CARTESIAN_POINT('Ctrl Pts',(-0.00226555956565516,-0.0405153085166175,
-0.0146341593839695));
#30760=CARTESIAN_POINT('Ctrl Pts',(-0.00330084907050131,-0.040357884301442,
-0.0116282694289622));
#30761=CARTESIAN_POINT('Ctrl Pts',(-0.00135523129196235,-0.0402004801327361,
-0.00911975560788823));
#30762=CARTESIAN_POINT('Ctrl Pts',(0.00180795669343061,-0.0400430759640301,
-0.00936286507619158));
#30763=CARTESIAN_POINT('Ctrl Pts',(0.00334401689248984,-0.039885671795324,
-0.0121412248982046));
#30764=CARTESIAN_POINT('Ctrl Pts',(0.00186639518515057,-0.0397282676266182,
-0.0149503248734341));
#30765=CARTESIAN_POINT('Ctrl Pts',(-0.00129229124532808,-0.0395708634579122,
-0.0152600053777664));
#30766=CARTESIAN_POINT('Ctrl Pts',(-0.00328692686994726,-0.0394134592892061,
-0.0127909042593799));
#30767=CARTESIAN_POINT('Ctrl Pts',(-0.00232009071187387,-0.0392560551205001,
-0.00976773624103997));
#30768=CARTESIAN_POINT('Ctrl Pts',(0.000736964239018967,-0.0390986509517941,
-0.00891412467460375));
#30769=CARTESIAN_POINT('Ctrl Pts',(0.0031300847491082,-0.0389412467830881,
-0.0109991774873666));
#30770=CARTESIAN_POINT('Ctrl Pts',(0.00270314507595757,-0.0387838426143821,
-0.0141443456440431));
#30771=CARTESIAN_POINT('Ctrl Pts',(-0.000159179402018772,-0.0386264384456762,
-0.0155160087888353));
#30772=CARTESIAN_POINT('Ctrl Pts',(-0.00287809585278843,-0.0384690342769703,
-0.0138783631584014));
#30773=CARTESIAN_POINT('Ctrl Pts',(-0.00300399525283862,-0.0383116301082643,
-0.010706845734549));
#30774=CARTESIAN_POINT('Ctrl Pts',(-0.000423452161205861,-0.0381542259395583,
-0.00885882720099533));
#30775=CARTESIAN_POINT('Ctrl Pts',(0.00253859991405746,-0.0379968217708523,
-0.00999927712131107));
#30776=CARTESIAN_POINT('Ctrl Pts',(0.00321350506802662,-0.0378394176021462,
-0.0131007089188475));
#30777=CARTESIAN_POINT('Ctrl Pts',(0.000993209282163632,-0.0376820134334403,
-0.0153688939258157));
#30778=CARTESIAN_POINT('Ctrl Pts',(-0.00212191654034275,-0.0375246092647344,
-0.0147603151838852));
#30779=CARTESIAN_POINT('Ctrl Pts',(-0.00332530577211061,-0.0373672050960284,
-0.0118232705799774));
#30780=CARTESIAN_POINT('Ctrl Pts',(-0.00153276730448458,-0.0372098009273224,
-0.00920388466402705));
#30781=CARTESIAN_POINT('Ctrl Pts',(0.00164071487392983,-0.0370523967586164,
-0.00926208806138846));
#30782=CARTESIAN_POINT('Ctrl Pts',(0.00333599819561317,-0.0368949925899104,
-0.0119454425268779));
#30783=CARTESIAN_POINT('Ctrl Pts',(0.00202572048170102,-0.0367375884212043,
-0.0148363851163382));
#30784=CARTESIAN_POINT('Ctrl Pts',(-0.00110962613287212,-0.0365801842524984,
-0.0153303267655248));
#30785=CARTESIAN_POINT('Ctrl Pts',(-0.00324525725626169,-0.0364227800837924,
-0.0129822517144672));
#30786=CARTESIAN_POINT('Ctrl Pts',(-0.00245708021311881,-0.0362653759150866,
-0.00990765357948378));
#30787=CARTESIAN_POINT('Ctrl Pts',(0.000544798434319117,-0.0361079717463805,
-0.008876585526832));
#30788=CARTESIAN_POINT('Ctrl Pts',(0.00305584199962463,-0.0359505675776744,
-0.0108179862983266));
#30789=CARTESIAN_POINT('Ctrl Pts',(0.00281373070242807,-0.0357931634089685,
-0.0139827546725603));
#30790=CARTESIAN_POINT('Ctrl Pts',(3.65942415151312E-5,-0.0356357592402625,
-0.0155195987831459));
#30791=CARTESIAN_POINT('Ctrl Pts',(-0.00277351172958201,-0.0354783550715565,
-0.0140439019396519));
#30792=CARTESIAN_POINT('Ctrl Pts',(-0.00308482774178444,-0.0353209509028505,
-0.0108851903220393));
#30793=CARTESIAN_POINT('Ctrl Pts',(-0.000616874243820103,-0.0351635467341445,
-0.00888929897362878));
#30794=CARTESIAN_POINT('Ctrl Pts',(0.00240685089553428,-0.0350061425654386,
-0.00985442229446193));
#30795=CARTESIAN_POINT('Ctrl Pts',(0.00326212843605663,-0.0348487383967326,
-0.012911034319417));
#30796=CARTESIAN_POINT('Ctrl Pts',(0.00117839775328719,-0.0346913342280267,
-0.0153052864332988));
#30797=CARTESIAN_POINT('Ctrl Pts',(-0.00196700807660791,-0.0345339300593206,
-0.0148800818845899));
#30798=CARTESIAN_POINT('Ctrl Pts',(-0.00334024183360881,-0.0343765258906146,
-0.0120185078790428));
#30799=CARTESIAN_POINT('Ctrl Pts',(-0.00170409125489704,-0.0342191217219087,
-0.00929869390928347));
#30800=CARTESIAN_POINT('Ctrl Pts',(0.00146735700140084,-0.0340617175532028,
-0.00917105104518666));
#30801=CARTESIAN_POINT('Ctrl Pts',(0.00331679284185456,-0.0339043133844968,
-0.0117505788702519));
#30802=CARTESIAN_POINT('Ctrl Pts',(0.00217797067024458,-0.0337469092157907,
-0.0147132568537032));
#30803=CARTESIAN_POINT('Ctrl Pts',(-0.000923089910697239,-0.0335895050470848,
-0.0153898660525223));
#30804=CARTESIAN_POINT('Ctrl Pts',(-0.00319249444305807,-0.0334321008783788,
-0.0131708167702892));
#30805=CARTESIAN_POINT('Ctrl Pts',(-0.0025856273656865,-0.0332746967096728,
-0.0100553570408789));
#30806=CARTESIAN_POINT('Ctrl Pts',(0.000350755628832307,-0.0331172925409668,
-0.00885035433878307));
#30807=CARTESIAN_POINT('Ctrl Pts',(0.00297112601158075,-0.032959888372261,
-0.0106414532246178));
#30808=CARTESIAN_POINT('Ctrl Pts',(0.00291466626476923,-0.0328024842035548,
-0.0138149671783149));
#30809=CARTESIAN_POINT('Ctrl Pts',(0.00023224359961718,-0.032645080034849,
-0.015511724024068));
#30810=CARTESIAN_POINT('Ctrl Pts',(-0.00265941836963197,-0.0324876758661428,
-0.0142030359465141));
#30811=CARTESIAN_POINT('Ctrl Pts',(-0.00315508278707255,-0.0323302716974368,
-0.0110679591272914));
#30812=CARTESIAN_POINT('Ctrl Pts',(-0.000808181124578904,-0.0321728675287309,
-0.00893104223920506));
#30813=CARTESIAN_POINT('Ctrl Pts',(0.00226684891256305,-0.0320154633600249,
-0.00971752204756393));
#30814=CARTESIAN_POINT('Ctrl Pts',(0.00329956747150683,-0.0318580591913191,
-0.0127188489850756));
#30815=CARTESIAN_POINT('Ctrl Pts',(0.00135954405032654,-0.0317006550226131,
-0.015230929159832));
#30816=CARTESIAN_POINT('Ctrl Pts',(-0.00180535182353563,-0.0315432508539071,
-0.0149906145092565));
#30817=CARTESIAN_POINT('Ctrl Pts',(-0.00334373137659125,-0.0313858466852011,
-0.0122142103674649));
#30818=CARTESIAN_POINT('Ctrl Pts',(-0.00186955959198933,-0.031228442516495,
-0.00940351302866479));
#30819=CARTESIAN_POINT('Ctrl Pts',(0.00128894325246858,-0.031071038347789,
-0.00909003517875381));
#30820=CARTESIAN_POINT('Ctrl Pts',(0.00328626289935744,-0.0309136341790831,
-0.0115577220437879));
#30821=CARTESIAN_POINT('Ctrl Pts',(0.0023226585551687,-0.0307562300103771,
-0.0145803578326937));
#30822=CARTESIAN_POINT('Ctrl Pts',(-0.000733194175148143,-0.0305988258416712,
-0.0154404939970894));
#30823=CARTESIAN_POINT('Ctrl Pts',(-0.00312927169148336,-0.0304414216729651,
-0.0133516097567121));
#30824=CARTESIAN_POINT('Ctrl Pts',(-0.00284524528910707,-0.0303364855604945,
-0.0112648453514926));
#30825=CARTESIAN_POINT('Ctrl Pts',(-0.00229544723482355,-0.0302840175042591,
-0.0105081132496665));
#30826=CARTESIAN_POINT('Ctrl Pts',(0.000642710920095802,-0.0407710844417939,
-0.0147642665038899));
#30827=CARTESIAN_POINT('Ctrl Pts',(-0.000210927518126123,-0.040718596339089,
-0.0149762541110002));
#30828=CARTESIAN_POINT('Ctrl Pts',(-0.00212956554017036,-0.0406136401801488,
-0.0144865954235559));
#30829=CARTESIAN_POINT('Ctrl Pts',(-0.00310271005026966,-0.0404562159649733,
-0.0116611390715061));
#30830=CARTESIAN_POINT('Ctrl Pts',(-0.00127388125303559,-0.0402988117962673,
-0.00930320301394971));
#30831=CARTESIAN_POINT('Ctrl Pts',(0.00169943105041994,-0.0401414076275612,
-0.00953171942730572));
#30832=CARTESIAN_POINT('Ctrl Pts',(0.00314328665109908,-0.0399840034588552,
-0.0121433035254893));
#30833=CARTESIAN_POINT('Ctrl Pts',(0.00175436167333222,-0.0398265992901494,
-0.0147837825474619));
#30834=CARTESIAN_POINT('Ctrl Pts',(-0.00121471928861808,-0.0396691951214434,
-0.0150748739583816));
#30835=CARTESIAN_POINT('Ctrl Pts',(-0.0030896235532325,-0.0395117909527374,
-0.0127539847897086));
#30836=CARTESIAN_POINT('Ctrl Pts',(-0.00218082336257045,-0.0393543867840314,
-0.00991228751915392));
#30837=CARTESIAN_POINT('Ctrl Pts',(0.000692726720384725,-0.0391969826153254,
-0.00910991542347796));
#30838=CARTESIAN_POINT('Ctrl Pts',(0.00294219614463583,-0.0390395784466194,
-0.011069809432361));
#30839=CARTESIAN_POINT('Ctrl Pts',(0.00254088424383383,-0.0388821742779135,
-0.0140261835776428));
#30840=CARTESIAN_POINT('Ctrl Pts',(-0.000149624390540353,-0.0387247701092075,
-0.0153155103338901));
#30841=CARTESIAN_POINT('Ctrl Pts',(-0.00270533330587274,-0.0385673659405015,
-0.0137761671383057));
#30842=CARTESIAN_POINT('Ctrl Pts',(-0.0028236753825673,-0.0384099617717955,
-0.0107950253849515));
#30843=CARTESIAN_POINT('Ctrl Pts',(-0.000398033732630625,-0.0382525576030895,
-0.00905793727377927));
#30844=CARTESIAN_POINT('Ctrl Pts',(0.00238621618217868,-0.0380951534343835,
-0.0101299297684424));
#30845=CARTESIAN_POINT('Ctrl Pts',(0.00302060901852883,-0.0379377492656776,
-0.0130451929031425));
#30846=CARTESIAN_POINT('Ctrl Pts',(0.000933590223597251,-0.0377803450969715,
-0.0151772262880931));
#30847=CARTESIAN_POINT('Ctrl Pts',(-0.00199454492917932,-0.0376229409282657,
-0.0146051785092827));
#30848=CARTESIAN_POINT('Ctrl Pts',(-0.00312569869720836,-0.0374655367595595,
-0.0118444349502773));
#30849=CARTESIAN_POINT('Ctrl Pts',(-0.00144076036764282,-0.0373081325908537,
-0.00938228208191872));
#30850=CARTESIAN_POINT('Ctrl Pts',(0.00154222820257447,-0.0371507284221477,
-0.00943699172240697));
#30851=CARTESIAN_POINT('Ctrl Pts',(0.00313574928999666,-0.0369933242534416,
-0.0119592733204704));
#30852=CARTESIAN_POINT('Ctrl Pts',(0.00190412320083946,-0.0368359200847357,
-0.0146766822160272));
#30853=CARTESIAN_POINT('Ctrl Pts',(-0.00104301895693193,-0.0366785159160298,
-0.0151409741865006));
#30854=CARTESIAN_POINT('Ctrl Pts',(-0.00305045522823148,-0.0365211117473236,
-0.0129338462917988));
#30855=CARTESIAN_POINT('Ctrl Pts',(-0.0023095898384728,-0.0363637075786177,
-0.0100438060839003));
#30856=CARTESIAN_POINT('Ctrl Pts',(0.000512095991494752,-0.0362063034099118,
-0.00907462962622331));
#30857=CARTESIAN_POINT('Ctrl Pts',(0.00287240994112814,-0.0360488992412058,
-0.0108994945493574));
#30858=CARTESIAN_POINT('Ctrl Pts',(0.00264483178197851,-0.0358914950724998,
-0.0138742923761538));
#30859=CARTESIAN_POINT('Ctrl Pts',(3.43976105861402E-5,-0.0357340909037938,
-0.0153188848327509));
#30860=CARTESIAN_POINT('Ctrl Pts',(-0.00260702702065921,-0.0355766867350878,
-0.0139317691756377));
#30861=CARTESIAN_POINT('Ctrl Pts',(-0.00289965576533666,-0.0354192825663817,
-0.0109626645384537));
#30862=CARTESIAN_POINT('Ctrl Pts',(-0.00057984532923908,-0.0352618783976759,
-0.00908657992698152));
#30863=CARTESIAN_POINT('Ctrl Pts',(0.00226237562020386,-0.0351044742289698,
-0.00999377009634113));
#30864=CARTESIAN_POINT('Ctrl Pts',(0.00306631368706786,-0.0349470700602639,
-0.0128669038407335));
#30865=CARTESIAN_POINT('Ctrl Pts',(0.00110766244510046,-0.0347896658915579,
-0.0151174369423551));
#30866=CARTESIAN_POINT('Ctrl Pts',(-0.00184893510666519,-0.0346322617228519,
-0.0147177560122302));
#30867=CARTESIAN_POINT('Ctrl Pts',(-0.00313973819648023,-0.0344748575541459,
-0.0120279528019148));
#30868=CARTESIAN_POINT('Ctrl Pts',(-0.00160180030962234,-0.0343174533854399,
-0.00947140024268058));
#30869=CARTESIAN_POINT('Ctrl Pts',(0.00137927642807616,-0.0341600492167341,
-0.00935141935630271));
#30870=CARTESIAN_POINT('Ctrl Pts',(0.0031176967699168,-0.0340026450480281,
-0.0117761066827561));
#30871=CARTESIAN_POINT('Ctrl Pts',(0.00204723431560415,-0.033845240879322,
-0.0145609449345611));
#30872=CARTESIAN_POINT('Ctrl Pts',(-0.000867679885402264,-0.0336878367106161,
-0.0151969395276014));
#30873=CARTESIAN_POINT('Ctrl Pts',(-0.00300085959168136,-0.0335304325419101,
-0.0131110924128218));
#30874=CARTESIAN_POINT('Ctrl Pts',(-0.00243042073188435,-0.033373028373204,
-0.0101826433964649));
#30875=CARTESIAN_POINT('Ctrl Pts',(0.000329700931948742,-0.0332156242044981,
-0.00904997300937973));
#30876=CARTESIAN_POINT('Ctrl Pts',(0.00279277917282932,-0.0330582200357922,
-0.0107335581704735));
#30877=CARTESIAN_POINT('Ctrl Pts',(0.00273970851733244,-0.032900815867086,
-0.0137165766086087));
#30878=CARTESIAN_POINT('Ctrl Pts',(0.000218302786723153,-0.0327434116983802,
-0.0153114827693384));
#30879=CARTESIAN_POINT('Ctrl Pts',(-0.00249978230664013,-0.0325860075296742,
-0.0140813508959422));
#30880=CARTESIAN_POINT('Ctrl Pts',(-0.00296569363330397,-0.0324286033609682,
-0.0111344623386012));
#30881=CARTESIAN_POINT('Ctrl Pts',(-0.000759668692542901,-0.0322711991922623,
-0.00912581748279469));
#30882=CARTESIAN_POINT('Ctrl Pts',(0.00213077749186029,-0.0321137950235563,
-0.00986508751714331));
#30883=CARTESIAN_POINT('Ctrl Pts',(0.00310150538141159,-0.0319563908548502,
-0.0126862547545015));
#30884=CARTESIAN_POINT('Ctrl Pts',(0.00127793513082136,-0.0317989866861443,
-0.0150475430893589));
#30885=CARTESIAN_POINT('Ctrl Pts',(-0.00169698254222384,-0.0316415825174383,
-0.0148216537300935));
#30886=CARTESIAN_POINT('Ctrl Pts',(-0.00314301827377279,-0.0314841783487323,
-0.0122119079191349));
#30887=CARTESIAN_POINT('Ctrl Pts',(-0.00175733613132536,-0.0313267741800263,
-0.00956992741802806));
#30888=CARTESIAN_POINT('Ctrl Pts',(0.00121157226466413,-0.0311693700113203,
-0.00927526660358858));
#30889=CARTESIAN_POINT('Ctrl Pts',(0.00308899943859484,-0.0310119658426143,
-0.0115948264118463));
#30890=CARTESIAN_POINT('Ctrl Pts',(0.00218323706675035,-0.0308545616739084,
-0.0144360234009344));
#30891=CARTESIAN_POINT('Ctrl Pts',(-0.000689182960942163,-0.0306971575052024,
-0.0152445284445975));
#30892=CARTESIAN_POINT('Ctrl Pts',(-0.00294143189216317,-0.0305397533364964,
-0.0132810329959904));
#30893=CARTESIAN_POINT('Ctrl Pts',(-0.00267445465255833,-0.0304348172240258,
-0.0113195301358683));
#30894=CARTESIAN_POINT('Ctrl Pts',(-0.0021576591517009,-0.0303823491677905,
-0.0106082221519074));
#30895=CARTESIAN_POINT('Ctrl Pts',(0.000601667409765497,-0.0408694161053251,
-0.0145989704721862));
#30896=CARTESIAN_POINT('Ctrl Pts',(-0.000197457689781191,-0.0408169280026203,
-0.0147974205536838));
#30897=CARTESIAN_POINT('Ctrl Pts',(-0.00199357151468546,-0.0407119718436801,
-0.0143390314631424));
#30898=CARTESIAN_POINT('Ctrl Pts',(-0.00290457103003801,-0.0405545476285045,
-0.01169400871405));
#30899=CARTESIAN_POINT('Ctrl Pts',(-0.00119253121410882,-0.0403971434597985,
-0.0094866504200112));
#30900=CARTESIAN_POINT('Ctrl Pts',(0.00159090540740915,-0.0402397392910926,
-0.0097005737784199));
#30901=CARTESIAN_POINT('Ctrl Pts',(0.00294255640970842,-0.0400823351223866,
-0.012145382152774));
#30902=CARTESIAN_POINT('Ctrl Pts',(0.00164232816151378,-0.0399249309536806,
-0.0146172402214899));
#30903=CARTESIAN_POINT('Ctrl Pts',(-0.00113714733190809,-0.0397675267849747,
-0.0148897425389965));
#30904=CARTESIAN_POINT('Ctrl Pts',(-0.00289232023651785,-0.0396101226162687,
-0.0127170653200376));
#30905=CARTESIAN_POINT('Ctrl Pts',(-0.00204155601326713,-0.0394527184475627,
-0.0100568387972678));
#30906=CARTESIAN_POINT('Ctrl Pts',(0.00064848920175059,-0.0392953142788567,
-0.00930570617235219));
#30907=CARTESIAN_POINT('Ctrl Pts',(0.00275430754016345,-0.0391379101101507,
-0.0111404413773551));
#30908=CARTESIAN_POINT('Ctrl Pts',(0.0023786234117102,-0.0389805059414447,
-0.0139080215112426));
#30909=CARTESIAN_POINT('Ctrl Pts',(-0.000140069379062041,-0.0388231017727388,
-0.015115011878945));
#30910=CARTESIAN_POINT('Ctrl Pts',(-0.00253257075895693,-0.0386656976040327,
-0.0136739711182101));
#30911=CARTESIAN_POINT('Ctrl Pts',(-0.00264335551229598,-0.0385082934353268,
-0.0108832050353539));
#30912=CARTESIAN_POINT('Ctrl Pts',(-0.000372615304055287,-0.0383508892666208,
-0.00925704734656319));
#30913=CARTESIAN_POINT('Ctrl Pts',(0.00223383245029989,-0.0381934850979148,
-0.0102605824155735));
#30914=CARTESIAN_POINT('Ctrl Pts',(0.00282771296903102,-0.0380360809292088,
-0.0129896768874376));
#30915=CARTESIAN_POINT('Ctrl Pts',(0.000873971165030867,-0.0378786767605029,
-0.0149855586503702));
#30916=CARTESIAN_POINT('Ctrl Pts',(-0.00186717331801599,-0.0377212725917968,
-0.0144500418346802));
#30917=CARTESIAN_POINT('Ctrl Pts',(-0.002926091622306,-0.0375638684230909,
-0.0118655993205774));
#30918=CARTESIAN_POINT('Ctrl Pts',(-0.00134875343080115,-0.0374064642543849,
-0.00956067949981042));
#30919=CARTESIAN_POINT('Ctrl Pts',(0.00144374153121912,-0.0372490600856789,
-0.00961189538342548));
#30920=CARTESIAN_POINT('Ctrl Pts',(0.00293550038438004,-0.0370916559169729,
-0.0119731041140629));
#30921=CARTESIAN_POINT('Ctrl Pts',(0.00178252591997789,-0.036934251748267,
-0.0145169793157163));
#30922=CARTESIAN_POINT('Ctrl Pts',(-0.000976411780991844,-0.0367768475795609,
-0.0149516216074763));
#30923=CARTESIAN_POINT('Ctrl Pts',(-0.00285565320020116,-0.036619443410855,
-0.0128854408691303));
#30924=CARTESIAN_POINT('Ctrl Pts',(-0.0021620994638269,-0.036462039242149,
-0.0101799585883167));
#30925=CARTESIAN_POINT('Ctrl Pts',(0.000479393548670495,-0.0363046350734431,
-0.00927267372561462));
#30926=CARTESIAN_POINT('Ctrl Pts',(0.00268897788263155,-0.0361472309047371,
-0.0109810028003882));
#30927=CARTESIAN_POINT('Ctrl Pts',(0.00247593286152883,-0.0359898267360311,
-0.0137658300797473));
#30928=CARTESIAN_POINT('Ctrl Pts',(3.22009796572556E-5,-0.0358324225673251,
-0.0151181708823559));
#30929=CARTESIAN_POINT('Ctrl Pts',(-0.00244054231173649,-0.0356750183986191,
-0.0138196364116234));
#30930=CARTESIAN_POINT('Ctrl Pts',(-0.00271448378888876,-0.0355176142299131,
-0.0110401387548681));
#30931=CARTESIAN_POINT('Ctrl Pts',(-0.00054281641465795,-0.0353602100612072,
-0.00928386088033424));
#30932=CARTESIAN_POINT('Ctrl Pts',(0.00211790034487343,-0.0352028058925012,
-0.0101331178982203));
#30933=CARTESIAN_POINT('Ctrl Pts',(0.00287049893807899,-0.0350454017237951,
-0.0128227733620499));
#30934=CARTESIAN_POINT('Ctrl Pts',(0.00103692713691383,-0.0348879975550892,
-0.0149295874514114));
#30935=CARTESIAN_POINT('Ctrl Pts',(-0.00173086213672248,-0.0347305933863832,
-0.0145554301398706));
#30936=CARTESIAN_POINT('Ctrl Pts',(-0.00293923455935166,-0.0345731892176772,
-0.0120373977247868));
#30937=CARTESIAN_POINT('Ctrl Pts',(-0.00149950936434765,-0.0344157850489713,
-0.0096441065760777));
#30938=CARTESIAN_POINT('Ctrl Pts',(0.0012911958547517,-0.0342583808802653,
-0.00953178766741874));
#30939=CARTESIAN_POINT('Ctrl Pts',(0.00291860069797893,-0.0341009767115593,
-0.0118016344952603));
#30940=CARTESIAN_POINT('Ctrl Pts',(0.00191649796096373,-0.0339435725428533,
-0.014408633015419));
#30941=CARTESIAN_POINT('Ctrl Pts',(-0.00081226986010739,-0.0337861683741473,
-0.0150040130026805));
#30942=CARTESIAN_POINT('Ctrl Pts',(-0.00280922474030466,-0.0336287642054413,
-0.0130513680553543));
#30943=CARTESIAN_POINT('Ctrl Pts',(-0.00227521409808231,-0.0334713600367354,
-0.010309929752051));
#30944=CARTESIAN_POINT('Ctrl Pts',(0.000308646235065284,-0.0333139558680293,
-0.00924959167997635));
#30945=CARTESIAN_POINT('Ctrl Pts',(0.0026144323340779,-0.0331565516993234,
-0.0108256631163291));
#30946=CARTESIAN_POINT('Ctrl Pts',(0.00256475076989575,-0.0329991475306174,
-0.0136181860389024));
#30947=CARTESIAN_POINT('Ctrl Pts',(0.000204361973829126,-0.0328417433619114,
-0.0151112415146089));
#30948=CARTESIAN_POINT('Ctrl Pts',(-0.0023401462436483,-0.0326843391932055,
-0.0139596658453702));
#30949=CARTESIAN_POINT('Ctrl Pts',(-0.00277630447953526,-0.0325269350244995,
-0.0112009655499111));
#30950=CARTESIAN_POINT('Ctrl Pts',(-0.000711156260506898,-0.0323695308557934,
-0.00932059272638428));
#30951=CARTESIAN_POINT('Ctrl Pts',(0.00199470607115752,-0.0322121266870875,
-0.0100126529867227));
#30952=CARTESIAN_POINT('Ctrl Pts',(0.00290344329131625,-0.0320547225183815,
-0.0126536605239274));
#30953=CARTESIAN_POINT('Ctrl Pts',(0.00119632621131608,-0.0318973183496755,
-0.0148641570188858));
#30954=CARTESIAN_POINT('Ctrl Pts',(-0.00158861326091204,-0.0317399141809696,
-0.0146526929509304));
#30955=CARTESIAN_POINT('Ctrl Pts',(-0.00294230517095442,-0.0315825100122636,
-0.0122096054708049));
#30956=CARTESIAN_POINT('Ctrl Pts',(-0.00164511267066117,-0.0314251058435576,
-0.00973634180739135));
#30957=CARTESIAN_POINT('Ctrl Pts',(0.00113420127685958,-0.0312677016748516,
-0.00946049802842335));
#30958=CARTESIAN_POINT('Ctrl Pts',(0.00289173597783214,-0.0311102975061456,
-0.0116319307799048));
#30959=CARTESIAN_POINT('Ctrl Pts',(0.0020438155783319,-0.0309528933374397,
-0.0142916889691752));
#30960=CARTESIAN_POINT('Ctrl Pts',(-0.000645171746736182,-0.0307954891687337,
-0.0150485628921055));
#30961=CARTESIAN_POINT('Ctrl Pts',(-0.00275359209284296,-0.0306380850000277,
-0.0132104562352686));
#30962=CARTESIAN_POINT('Ctrl Pts',(-0.00250366401600948,-0.030533148887557,
-0.0113742149202441));
#30963=CARTESIAN_POINT('Ctrl Pts',(-0.00201987106857834,-0.0304806808313217,
-0.0107083310541483));
#30964=CARTESIAN_POINT('',(-0.00112535951647366,-0.0304787743898623,-0.0149567822606029));
#30965=CARTESIAN_POINT('Ctrl Pts',(-0.00202254248593818,-0.0304787743898724,
-0.010706390155828));
#30966=CARTESIAN_POINT('Ctrl Pts',(-0.00207933679775776,-0.0304787743898759,
-0.010768823046726));
#30967=CARTESIAN_POINT('Ctrl Pts',(-0.00213253650680991,-0.0304787743898759,
-0.0108341592693267));
#30968=CARTESIAN_POINT('Ctrl Pts',(-0.00218216719076719,-0.0304787743898759,
-0.0109020191122561));
#30969=CARTESIAN_POINT('Ctrl Pts',(-0.00228485960892478,-0.0304787743898758,
-0.0110424300598912));
#30970=CARTESIAN_POINT('Ctrl Pts',(-0.00237230998742211,-0.0304787743898757,
-0.0111936097303547));
#30971=CARTESIAN_POINT('Ctrl Pts',(-0.00244435095552589,-0.0304787743898755,
-0.0113527208897216));
#30972=CARTESIAN_POINT('Ctrl Pts',(-0.00245258921046642,-0.0304787743898755,
-0.0113709160685101));
#30973=CARTESIAN_POINT('Ctrl Pts',(-0.00246062531162263,-0.0304787743898755,
-0.0113892155623281));
#30974=CARTESIAN_POINT('Ctrl Pts',(-0.00246845849194243,-0.0304787743898755,
-0.0114076155457809));
#30975=CARTESIAN_POINT('Ctrl Pts',(-0.00247483468516254,-0.0304787743898755,
-0.0114225930957609));
#30976=CARTESIAN_POINT('Ctrl Pts',(-0.00248107304918276,-0.0304787743898755,
-0.0114376294063823));
#30977=CARTESIAN_POINT('Ctrl Pts',(-0.00248717124270606,-0.0304787743898755,
-0.0114527162532319));
#30978=CARTESIAN_POINT('Ctrl Pts',(-0.00255536474803799,-0.0304787743898753,
-0.0116214260469026));
#30979=CARTESIAN_POINT('Ctrl Pts',(-0.00260618039173054,-0.030478774389875,
-0.0117966365888452));
#30980=CARTESIAN_POINT('Ctrl Pts',(-0.00263944649157874,-0.0304787743898749,
-0.0119752482167937));
#30981=CARTESIAN_POINT('Ctrl Pts',(-0.00264856017282487,-0.0304787743898748,
-0.0120241811981592));
#30982=CARTESIAN_POINT('Ctrl Pts',(-0.00265635281447305,-0.0304787743898747,
-0.0120733723859067));
#30983=CARTESIAN_POINT('Ctrl Pts',(-0.00266281171147326,-0.0304787743898747,
-0.0121227634589119));
#30984=CARTESIAN_POINT('Ctrl Pts',(-0.00266823331331669,-0.0304787743898746,
-0.0121642223538975));
#30985=CARTESIAN_POINT('Ctrl Pts',(-0.00267271510098182,-0.0304787743898745,
-0.0122058221316629));
#30986=CARTESIAN_POINT('Ctrl Pts',(-0.00267624717494561,-0.0304787743898745,
-0.0122475289422248));
#30987=CARTESIAN_POINT('Ctrl Pts',(-0.00267748798737737,-0.0304787743898745,
-0.0122621804839435));
#30988=CARTESIAN_POINT('Ctrl Pts',(-0.00267861105896926,-0.0304787743898745,
-0.0122768396339577));
#30989=CARTESIAN_POINT('Ctrl Pts',(-0.00267961576376998,-0.0304787743898744,
-0.0122914972696341));
#30990=CARTESIAN_POINT('Ctrl Pts',(-0.00269915394615531,-0.030478774389874,
-0.0125765397607023));
#30991=CARTESIAN_POINT('Ctrl Pts',(-0.00267434900802219,-0.0304787743898735,
-0.0128617661037894));
#30992=CARTESIAN_POINT('Ctrl Pts',(-0.00260324668114919,-0.0304787743898729,
-0.0131363711390872));
#30993=CARTESIAN_POINT('Ctrl Pts',(-0.00260161897333744,-0.0304787743898729,
-0.0131426575263372));
#30994=CARTESIAN_POINT('Ctrl Pts',(-0.00259996681043361,-0.0304787743898729,
-0.0131489383768583));
#30995=CARTESIAN_POINT('Ctrl Pts',(-0.00259829014110119,-0.0304787743898729,
-0.0131552135626665));
#30996=CARTESIAN_POINT('Ctrl Pts',(-0.00258319016612878,-0.0304787743898728,
-0.0132117274779743));
#30997=CARTESIAN_POINT('Ctrl Pts',(-0.0025660879293159,-0.0304787743898726,
-0.0132678257833988));
#30998=CARTESIAN_POINT('Ctrl Pts',(-0.00254710084680293,-0.0304787743898725,
-0.0133233047976962));
#30999=CARTESIAN_POINT('Ctrl Pts',(-0.00243724439375196,-0.0304787743898718,
-0.013644298174394));
#31000=CARTESIAN_POINT('Ctrl Pts',(-0.00226595903811895,-0.0304787743898712,
-0.0139422543456244));
#31001=CARTESIAN_POINT('Ctrl Pts',(-0.00204792614583985,-0.0304787743898704,
-0.0142063722525525));
#31002=CARTESIAN_POINT('Ctrl Pts',(-0.00203805779522129,-0.0304787743898703,
-0.0142183264493847));
#31003=CARTESIAN_POINT('Ctrl Pts',(-0.00202809230240618,-0.0304787743898703,
-0.0142302109176497));
#31004=CARTESIAN_POINT('Ctrl Pts',(-0.00201803066157199,-0.0304787743898703,
-0.014242024505078));
#31005=CARTESIAN_POINT('Ctrl Pts',(-0.00200805701449532,-0.0304787743898702,
-0.0142537347771559));
#31006=CARTESIAN_POINT('Ctrl Pts',(-0.00199799386009692,-0.0304787743898703,
-0.0142653695213677));
#31007=CARTESIAN_POINT('Ctrl Pts',(-0.00198784674813982,-0.0304787743898702,
-0.0142769230298409));
#31008=CARTESIAN_POINT('Ctrl Pts',(-0.00179041923550486,-0.0304787743898696,
-0.0145017141280078));
#31009=CARTESIAN_POINT('Ctrl Pts',(-0.00156103476696635,-0.030478774389869,
-0.0146964800346998));
#31010=CARTESIAN_POINT('Ctrl Pts',(-0.0013081573752397,-0.0304787743898684,
-0.0148540088522852));
#31011=CARTESIAN_POINT('Ctrl Pts',(-0.00124886968763201,-0.0304787743898683,
-0.0148909418468184));
#31012=CARTESIAN_POINT('Ctrl Pts',(-0.00118827577426145,-0.0304787743881383,
-0.0149258181448674));
#31013=CARTESIAN_POINT('Ctrl Pts',(-0.00112646089251171,-0.030478774389873,
-0.0149585221565764));
#31014=CARTESIAN_POINT('',(-0.00299999968372376,-0.0402901830710539,-0.012175061470323));
#31015=CARTESIAN_POINT('Ctrl Pts',(-0.00299999999996642,-0.0402902259228274,
-0.0121758674800884));
#31016=CARTESIAN_POINT('Ctrl Pts',(-0.0029999973909628,-0.0403194684506487,
-0.0127273166757509));
#31017=CARTESIAN_POINT('Ctrl Pts',(-0.00284359154959909,-0.0403487109784699,
-0.0132796810926993));
#31018=CARTESIAN_POINT('Ctrl Pts',(-0.00255417076918103,-0.0403779535062912,
-0.0137494516094668));
#31019=CARTESIAN_POINT('Ctrl Pts',(-0.00236761854760589,-0.0403968023896424,
-0.0140522520283134));
#31020=CARTESIAN_POINT('Ctrl Pts',(-0.00212699904315092,-0.0404156512729936,
-0.0143208130958077));
#31021=CARTESIAN_POINT('Ctrl Pts',(-0.00184856593603868,-0.0404345001563449,
-0.0145386490839383));
#31022=CARTESIAN_POINT('Ctrl Pts',(-0.00141659934526726,-0.0404637426841661,
-0.0148766041142004));
#31023=CARTESIAN_POINT('Ctrl Pts',(-0.000886891013127971,-0.0404929852119873,
-0.015094515020395));
#31024=CARTESIAN_POINT('Ctrl Pts',(-0.000337993503381779,-0.0405222277398086,
-0.0151567525454516));
#31025=CARTESIAN_POINT('Ctrl Pts',(1.58098749104893E-5,-0.0405410766231597,
-0.0151968690448537));
#31026=CARTESIAN_POINT('Ctrl Pts',(0.000376850571609003,-0.0405599255065109,
-0.0151732399838831));
#31027=CARTESIAN_POINT('Ctrl Pts',(0.000721855543562045,-0.0405787743898621,
-0.0150877125850526));
#31028=CARTESIAN_POINT('',(-0.00299999946992021,-0.0392900367108314,-0.0121771409863751));
#31029=CARTESIAN_POINT('Ctrl Pts',(-0.00299999898776283,-0.0392900992552675,
-0.012178317717926));
#31030=CARTESIAN_POINT('Ctrl Pts',(-0.00299954158667841,-0.0393196461574803,
-0.0127351207225248));
#31031=CARTESIAN_POINT('Ctrl Pts',(-0.00283976987755387,-0.039349193059693,
-0.0132919112893292));
#31032=CARTESIAN_POINT('Ctrl Pts',(-0.00254505043098655,-0.0393787399619057,
-0.0137641600276302));
#31033=CARTESIAN_POINT('Ctrl Pts',(-0.00242416025283272,-0.0393908597263596,
-0.0139578704691063));
#31034=CARTESIAN_POINT('Ctrl Pts',(-0.002281166455956,-0.0394029794908136,
-0.0141375264551638));
#31035=CARTESIAN_POINT('Ctrl Pts',(-0.00212000447914795,-0.0394150992552675,
-0.0142984886787988));
#31036=CARTESIAN_POINT('Ctrl Pts',(-0.00173434249492379,-0.039444101954913,
-0.0146836726519771));
#31037=CARTESIAN_POINT('Ctrl Pts',(-0.00123911027380901,-0.0394731046545585,
-0.0149622077535727));
#31038=CARTESIAN_POINT('Ctrl Pts',(-0.000707581479706982,-0.0395021073542039,
-0.0150912140617583));
#31039=CARTESIAN_POINT('Ctrl Pts',(-0.000475490563978323,-0.0395147713212251,
-0.0151475443914296));
#31040=CARTESIAN_POINT('Ctrl Pts',(-0.000236850429755516,-0.0395274352882463,
-0.0151759527300397));
#31041=CARTESIAN_POINT('Ctrl Pts',(1.25624153382951E-6,-0.0395400992552675,
-0.0151758530235343));
#31042=CARTESIAN_POINT('Ctrl Pts',(0.000548578657520092,-0.039569209204134,
-0.0151756238337971));
#31043=CARTESIAN_POINT('Ctrl Pts',(0.0010976461232431,-0.0395983191530005,
-0.0150212816042846));
#31044=CARTESIAN_POINT('Ctrl Pts',(0.00156584391071221,-0.039627429101867,
-0.0147347852605045));
#31045=CARTESIAN_POINT('Ctrl Pts',(0.00176780329988407,-0.0396399858196672,
-0.0146112036714019));
#31046=CARTESIAN_POINT('Ctrl Pts',(0.00195487121302341,-0.0396525425374674,
-0.0144636952428034));
#31047=CARTESIAN_POINT('Ctrl Pts',(0.00212178143067051,-0.0396650992552675,
-0.0142967124427639));
#31048=CARTESIAN_POINT('Ctrl Pts',(0.00250865271321648,-0.0396942037258529,
-0.0139096729258002));
#31049=CARTESIAN_POINT('Ctrl Pts',(0.00278783414274103,-0.0397233081964383,
-0.0134124406496366));
#31050=CARTESIAN_POINT('Ctrl Pts',(0.00291644867266022,-0.0397524126670237,
-0.0128789373069557));
#31051=CARTESIAN_POINT('Ctrl Pts',(0.00297196182618088,-0.039764974863105,
-0.0126486643122587));
#31052=CARTESIAN_POINT('Ctrl Pts',(0.00300000378267172,-0.0397775370591862,
-0.0124119928788954));
#31053=CARTESIAN_POINT('Ctrl Pts',(0.00299999999961518,-0.0397900992552675,
-0.0121758052350621));
#31054=CARTESIAN_POINT('Ctrl Pts',(0.00299999123491694,-0.0398192037258529,
-0.0116285986568405));
#31055=CARTESIAN_POINT('Ctrl Pts',(0.00284593322591044,-0.0398483081964383,
-0.0110795663259316));
#31056=CARTESIAN_POINT('Ctrl Pts',(0.00255972584052127,-0.0398774126670237,
-0.0106113074670412));
#31057=CARTESIAN_POINT('Ctrl Pts',(0.00243619178465802,-0.039889974863105,
-0.0104091955755051));
#31058=CARTESIAN_POINT('Ctrl Pts',(0.00228870187842766,-0.0399025370591862,
-0.010221976464095));
#31059=CARTESIAN_POINT('Ctrl Pts',(0.00212171348927827,-0.0399150992552675,
-0.0100549261615926));
#31060=CARTESIAN_POINT('Ctrl Pts',(0.00173475698597329,-0.039944209204134,
-0.00966782618858453));
#31061=CARTESIAN_POINT('Ctrl Pts',(0.00123753050888079,-0.0399733191530005,
-0.00938841725028805));
#31062=CARTESIAN_POINT('Ctrl Pts',(0.000703965181250702,-0.040002429101867,
-0.00925961718096125));
#31063=CARTESIAN_POINT('Ctrl Pts',(0.000473809186208603,-0.0400149858196672,
-0.00920405864560988));
#31064=CARTESIAN_POINT('Ctrl Pts',(0.00023725032350367,-0.0400275425374673,
-0.00917594480999342));
#31065=CARTESIAN_POINT('Ctrl Pts',(1.16013854950112E-6,-0.0400400992552675,
-0.00917585351087835));
#31066=CARTESIAN_POINT('Ctrl Pts',(-0.000544145795090869,-0.040069101954913,
-0.00917564263405095));
#31067=CARTESIAN_POINT('Ctrl Pts',(-0.00109148312293973,-0.0400981046545585,
-0.00932844585482911));
#31068=CARTESIAN_POINT('Ctrl Pts',(-0.00155873907649531,-0.0401271073542039,
-0.00961258730515731));
#31069=CARTESIAN_POINT('Ctrl Pts',(-0.00176276539330768,-0.0401397713212251,
-0.00973665706418991));
#31070=CARTESIAN_POINT('Ctrl Pts',(-0.00195167937928901,-0.0401524352882463,
-0.00988509065248151));
#31071=CARTESIAN_POINT('Ctrl Pts',(-0.00212007247526431,-0.0401650992552675,
-0.0100532858083312));
#31072=CARTESIAN_POINT('Ctrl Pts',(-0.00251295839574671,-0.0401946461574802,
-0.0104457099053165));
#31073=CARTESIAN_POINT('Ctrl Pts',(-0.00279479323571491,-0.0402241930596929,
-0.0109512266395961));
#31074=CARTESIAN_POINT('Ctrl Pts',(-0.00292147013814697,-0.0402537399619056,
-0.0114939352328922));
#31075=CARTESIAN_POINT('Ctrl Pts',(-0.00297343139649411,-0.0402658597263596,
-0.0117165474130297));
#31076=CARTESIAN_POINT('Ctrl Pts',(-0.00299981876148167,-0.0402779794908135,
-0.0119450914234068));
#31077=CARTESIAN_POINT('Ctrl Pts',(-0.00299999906516995,-0.0402900992552675,
-0.0121734849581512));
#31078=CARTESIAN_POINT('',(-0.00299999999997869,-0.0382901316627664,-0.0121758419798184));
#31079=CARTESIAN_POINT('Ctrl Pts',(-0.00299999999997869,-0.0382901316627664,
-0.0121758419798184));
#31080=CARTESIAN_POINT('Ctrl Pts',(-0.00300000209850155,-0.0383196658629544,
-0.0127326398498295));
#31081=CARTESIAN_POINT('Ctrl Pts',(-0.0028406928257506,-0.0383492000631425,
-0.0132895576126836));
#31082=CARTESIAN_POINT('Ctrl Pts',(-0.00254636805818545,-0.0383787342633305,
-0.0137620467527698));
#31083=CARTESIAN_POINT('Ctrl Pts',(-0.00242552924534037,-0.0383908599084761,
-0.0139560332366208));
#31084=CARTESIAN_POINT('Ctrl Pts',(-0.0022825348872017,-0.0384029855536217,
-0.0141359579429274));
#31085=CARTESIAN_POINT('Ctrl Pts',(-0.00212132786731001,-0.0384151111987673,
-0.0142971661063407));
#31086=CARTESIAN_POINT('Ctrl Pts',(-0.00173591447646292,-0.0384441011646814,
-0.0146825822311167));
#31087=CARTESIAN_POINT('Ctrl Pts',(-0.00124086710218791,-0.0384730911305954,
-0.014961424000368));
#31088=CARTESIAN_POINT('Ctrl Pts',(-0.000709429170937981,-0.0385020810965095,
-0.0150907649921544));
#31089=CARTESIAN_POINT('Ctrl Pts',(-0.000477167617824278,-0.038514750975929,
-0.0151472926464054));
#31090=CARTESIAN_POINT('Ctrl Pts',(-0.000238327411029265,-0.0385274208553486,
-0.0151758524942411));
#31091=CARTESIAN_POINT('Ctrl Pts',(-9.97367769725772E-9,-0.0385400907347681,
-0.0151758532865415));
#31092=CARTESIAN_POINT('Ctrl Pts',(0.000547301483854578,-0.0385691879349098,
-0.0151758551061109));
#31093=CARTESIAN_POINT('Ctrl Pts',(0.0010964252806087,-0.0385982851350515,
-0.0150217505661102));
#31094=CARTESIAN_POINT('Ctrl Pts',(0.0015647392256642,-0.0386273823351932,
-0.0147354609040784));
#31095=CARTESIAN_POINT('Ctrl Pts',(0.00176693262920518,-0.0386399449803851,
-0.0146118560407683));
#31096=CARTESIAN_POINT('Ctrl Pts',(0.00195421808405336,-0.038652507625577,
-0.0144642748528175));
#31097=CARTESIAN_POINT('Ctrl Pts',(0.00212131376240286,-0.0386650702707689,
-0.0142971802112541));
#31098=CARTESIAN_POINT('Ctrl Pts',(0.00250826280330305,-0.038694162007648,
-0.0139102335712741));
#31099=CARTESIAN_POINT('Ctrl Pts',(0.00278755190614221,-0.0387232537445272,
-0.0134130729657069));
#31100=CARTESIAN_POINT('Ctrl Pts',(0.00291628703057831,-0.0387523454814063,
-0.012879607473246));
#31101=CARTESIAN_POINT('Ctrl Pts',(0.00297190272009648,-0.0387649135898608,
-0.0126491416129975));
#31102=CARTESIAN_POINT('Ctrl Pts',(0.00299999931911397,-0.0387774816983152,
-0.0124122595203428));
#31103=CARTESIAN_POINT('Ctrl Pts',(0.00299999999998756,-0.0387900498067697,
-0.0121758619271738));
#31104=CARTESIAN_POINT('Ctrl Pts',(0.00300000157602387,-0.0388191415436489,
-0.0116286660938282));
#31105=CARTESIAN_POINT('Ctrl Pts',(0.00284595972857232,-0.038848233280528,
-0.0110796393911313));
#31106=CARTESIAN_POINT('Ctrl Pts',(0.00255977000054816,-0.0388773250174071,
-0.0106113797187745));
#31107=CARTESIAN_POINT('Ctrl Pts',(0.00243613133451351,-0.0388898931258616,
-0.0104090838444685));
#31108=CARTESIAN_POINT('Ctrl Pts',(0.00228849336430286,-0.0389024612343161,
-0.0102217068524303));
#31109=CARTESIAN_POINT('Ctrl Pts',(0.00212132598208153,-0.0389150293427706,
-0.0100545385815353));
#31110=CARTESIAN_POINT('Ctrl Pts',(0.00173430650375096,-0.0389441265429123,
-0.00966751704578188));
#31111=CARTESIAN_POINT('Ctrl Pts',(0.00123703934374884,-0.038973223743054,
-0.00938820096654016));
#31112=CARTESIAN_POINT('Ctrl Pts',(0.000703460243350564,-0.0390023209431956,
-0.00925949533767302));
#31113=CARTESIAN_POINT('Ctrl Pts',(0.000473088768174648,-0.0390148835883876,
-0.00920392699632787));
#31114=CARTESIAN_POINT('Ctrl Pts',(0.000236307694429044,-0.0390274462335795,
-0.00917585386215959));
#31115=CARTESIAN_POINT('Ctrl Pts',(7.30755370494918E-9,-0.0390400088787714,
-0.009175853286567));
#31116=CARTESIAN_POINT('Ctrl Pts',(-0.000545287099503098,-0.0390689988446854,
-0.00917585195831094));
#31117=CARTESIAN_POINT('Ctrl Pts',(-0.00109255643801982,-0.0390979888105995,
-0.00932885928753787));
#31118=CARTESIAN_POINT('Ctrl Pts',(-0.00155969815203688,-0.0391269787765136,
-0.00961317077119793));
#31119=CARTESIAN_POINT('Ctrl Pts',(-0.00176385945412274,-0.0391396486559331,
-0.00973742728899603));
#31120=CARTESIAN_POINT('Ctrl Pts',(-0.00195287221682881,-0.0391523185353526,
-0.00988608556203413));
#31121=CARTESIAN_POINT('Ctrl Pts',(-0.00212131564764227,-0.0391649884147722,
-0.0100545282470915));
#31122=CARTESIAN_POINT('Ctrl Pts',(-0.0025139667409373,-0.0391945226149602,
-0.0104471776019871));
#31123=CARTESIAN_POINT('Ctrl Pts',(-0.00279550442572559,-0.0392240568151483,
-0.0109528531345857));
#31124=CARTESIAN_POINT('Ctrl Pts',(-0.00292186532648642,-0.0392535910153363,
-0.0114956305187266));
#31125=CARTESIAN_POINT('Ctrl Pts',(-0.0029737444169357,-0.0392657166604818,
-0.0117184747437687));
#31126=CARTESIAN_POINT('Ctrl Pts',(-0.00299999954473676,-0.0392778423056274,
-0.0119472467965074));
#31127=CARTESIAN_POINT('Ctrl Pts',(-0.00299999999999405,-0.039289967950773,
-0.0121758473120664));
#31128=CARTESIAN_POINT('',(-0.00299999975524206,-0.0372901454620687,-0.012175006789073));
#31129=CARTESIAN_POINT('Ctrl Pts',(-0.00299999999992875,-0.0372901916688699,
-0.0121758739623732));
#31130=CARTESIAN_POINT('Ctrl Pts',(-0.00299999616250721,-0.037319729033795,
-0.0127326725489632));
#31131=CARTESIAN_POINT('Ctrl Pts',(-0.00284068056307778,-0.0373492663987202,
-0.0132895892145799));
#31132=CARTESIAN_POINT('Ctrl Pts',(-0.00254635010445755,-0.0373788037636454,
-0.0137620755741108));
#31133=CARTESIAN_POINT('Ctrl Pts',(-0.00242552383528,-0.0373909292148201,
-0.0139560370292964));
#31134=CARTESIAN_POINT('Ctrl Pts',(-0.00228254760308849,-0.0374030546659948,
-0.0141359399142671));
#31135=CARTESIAN_POINT('Ctrl Pts',(-0.00212136282185931,-0.0374151801171696,
-0.0142971311509674));
#31136=CARTESIAN_POINT('Ctrl Pts',(-0.00173595466511071,-0.0374441732252743,
-0.0146825547433621));
#31137=CARTESIAN_POINT('Ctrl Pts',(-0.00124091039930104,-0.037473166333379,
-0.0149614049572775));
#31138=CARTESIAN_POINT('Ctrl Pts',(-0.000709473212190282,-0.0375021594414836,
-0.0150907542730728));
#31139=CARTESIAN_POINT('Ctrl Pts',(-0.000477240298278814,-0.0375148291494789,
-0.0151472786737888));
#31140=CARTESIAN_POINT('Ctrl Pts',(-0.000238429889195819,-0.0375274988574741,
-0.0151758420976629));
#31141=CARTESIAN_POINT('Ctrl Pts',(-1.40823792993672E-7,-0.0375401685654693,
-0.0151758532832529));
#31142=CARTESIAN_POINT('Ctrl Pts',(0.000547172115070815,-0.0375692689151043,
-0.0151758789748142));
#31143=CARTESIAN_POINT('Ctrl Pts',(0.00109630381278015,-0.0375983692647393,
-0.0150217975875743));
#31144=CARTESIAN_POINT('Ctrl Pts',(0.00156463088029391,-0.0376274696143742,
-0.0147355271346158));
#31145=CARTESIAN_POINT('Ctrl Pts',(0.00176680518933334,-0.0376400320808392,
-0.0146119456996743));
#31146=CARTESIAN_POINT('Ctrl Pts',(0.00195407617399039,-0.0376525945473041,
-0.0144643931084875));
#31147=CARTESIAN_POINT('Ctrl Pts',(0.00212116366158087,-0.037665157013769,
-0.0142973303005247));
#31148=CARTESIAN_POINT('Ctrl Pts',(0.00250814109920495,-0.03769425189785,
-0.0139104100213344));
#31149=CARTESIAN_POINT('Ctrl Pts',(0.00278746564107153,-0.037723346781931,
-0.0134132678179795));
#31150=CARTESIAN_POINT('Ctrl Pts',(0.00291623811122977,-0.0377524416660121,
-0.0128798101592506));
#31151=CARTESIAN_POINT('Ctrl Pts',(0.00297186313610854,-0.0377650095980309,
-0.0126493758474594));
#31152=CARTESIAN_POINT('Ctrl Pts',(0.00299997616477368,-0.0377775775300498,
-0.0124125249373827));
#31153=CARTESIAN_POINT('Ctrl Pts',(0.00299999998476676,-0.0377901454620687,
-0.0121761556099587));
#31154=CARTESIAN_POINT('Ctrl Pts',(0.00300005512828093,-0.0378192403461497,
-0.0116289583326836));
#31155=CARTESIAN_POINT('Ctrl Pts',(0.00284606624918581,-0.0378483352302307,
-0.0110799154030114));
#31156=CARTESIAN_POINT('Ctrl Pts',(0.00255992117660712,-0.0378774301143118,
-0.0106116270978122));
#31157=CARTESIAN_POINT('Ctrl Pts',(0.00243631690962701,-0.0378899980463306,
-0.0104093435771565));
#31158=CARTESIAN_POINT('Ctrl Pts',(0.00228871769291662,-0.0379025659783495,
-0.0102219730135154));
#31159=CARTESIAN_POINT('Ctrl Pts',(0.00212159119992591,-0.0379151339103684,
-0.0100548038339529));
#31160=CARTESIAN_POINT('Ctrl Pts',(0.00173461907340646,-0.0379442342600034,
-0.00966773286904355));
#31161=CARTESIAN_POINT('Ctrl Pts',(0.00123738544701644,-0.0379733346096384,
-0.00938835434554213));
#31162=CARTESIAN_POINT('Ctrl Pts',(0.000703821130662529,-0.0380024349592733,
-0.00925958241161645));
#31163=CARTESIAN_POINT('Ctrl Pts',(0.000473484247595724,-0.0380149974257383,
-0.00920399225129686));
#31164=CARTESIAN_POINT('Ctrl Pts',(0.000236735910866754,-0.0380275598922032,
-0.00917588985189061));
#31165=CARTESIAN_POINT('Ctrl Pts',(4.63823007370569E-7,-0.0380401223586681,
-0.00917585332241339));
#31166=CARTESIAN_POINT('Ctrl Pts',(-0.000544832134960051,-0.0380691154667728,
-0.00917576901547534));
#31167=CARTESIAN_POINT('Ctrl Pts',(-0.00109212599337851,-0.0380981085748774,
-0.00932869389979686));
#31168=CARTESIAN_POINT('Ctrl Pts',(-0.00155931164168855,-0.0381271016829821,
-0.0096129355734634));
#31169=CARTESIAN_POINT('Ctrl Pts',(-0.00176346725419761,-0.0381397713909773,
-0.00973714643738421));
#31170=CARTESIAN_POINT('Ctrl Pts',(-0.00195248165559007,-0.0381524410989726,
-0.0098857554706572));
#31171=CARTESIAN_POINT('Ctrl Pts',(-0.00212093523748278,-0.0381651108069678,
-0.0100541479068213));
#31172=CARTESIAN_POINT('Ctrl Pts',(-0.00251365738413268,-0.038194648171893,
-0.0104467275021434));
#31173=CARTESIAN_POINT('Ctrl Pts',(-0.00279528586443748,-0.0382241855368181,
-0.0109523533829576));
#31174=CARTESIAN_POINT('Ctrl Pts',(-0.00292174382330747,-0.0382537229017433,
-0.011495108818373));
#31175=CARTESIAN_POINT('Ctrl Pts',(-0.00297365636898722,-0.038265848352918,
-0.01171791659248));
#31176=CARTESIAN_POINT('Ctrl Pts',(-0.00299995229094424,-0.0382779738040928,
-0.011946655308718));
#31177=CARTESIAN_POINT('Ctrl Pts',(-0.0029999999348286,-0.0382900992552675,
-0.0121752279639453));
#31178=CARTESIAN_POINT('',(-0.00299999945826961,-0.0362900263245557,-0.0121770992877974));
#31179=CARTESIAN_POINT('Ctrl Pts',(-0.00299999885509523,-0.0362900992552675,
-0.0121784742457941));
#31180=CARTESIAN_POINT('Ctrl Pts',(-0.00299951240275064,-0.0363196453473993,
-0.0127352766778096));
#31181=CARTESIAN_POINT('Ctrl Pts',(-0.00283971194097578,-0.0363491914395311,
-0.0132920584481428));
#31182=CARTESIAN_POINT('Ctrl Pts',(-0.00254496835509526,-0.0363787375316629,
-0.0137642915357714));
#31183=CARTESIAN_POINT('Ctrl Pts',(-0.00242405687937795,-0.0363908581061978,
-0.013958013815892));
#31184=CARTESIAN_POINT('Ctrl Pts',(-0.00228103836935438,-0.0364029786807326,
-0.0141376778523285));
#31185=CARTESIAN_POINT('Ctrl Pts',(-0.00211984966677049,-0.0364150992552675,
-0.0142986432880168));
#31186=CARTESIAN_POINT('Ctrl Pts',(-0.00173416044612212,-0.0364441011323918,
-0.0146837982799409));
#31187=CARTESIAN_POINT('Ctrl Pts',(-0.00123890904906828,-0.0364731030095161,
-0.0149622970438916));
#31188=CARTESIAN_POINT('Ctrl Pts',(-0.000707371908332917,-0.0365021048866404,
-0.0150912649184381));
#31189=CARTESIAN_POINT('Ctrl Pts',(-0.000475255690733393,-0.0365147696761827,
-0.0151475837209026));
#31190=CARTESIAN_POINT('Ctrl Pts',(-0.000236591057320712,-0.0365274344657251,
-0.0151759749177501));
#31191=CARTESIAN_POINT('Ctrl Pts',(1.53730189014851E-6,-0.0365400992552675,
-0.0151758528926752));
#31192=CARTESIAN_POINT('Ctrl Pts',(0.000548858560926287,-0.0365692083818778,
-0.0151755724266364));
#31193=CARTESIAN_POINT('Ctrl Pts',(0.00109791066251957,-0.0365983175084881,
-0.0150211793683654));
#31194=CARTESIAN_POINT('Ctrl Pts',(0.00156608112127079,-0.0366274266350983,
-0.014734640093152));
#31195=CARTESIAN_POINT('Ctrl Pts',(0.00176804765113956,-0.0366399841751547,
-0.0146110284000086));
#31196=CARTESIAN_POINT('Ctrl Pts',(0.00195511772629248,-0.0366525417152111,
-0.0144634868178142));
#31197=CARTESIAN_POINT('Ctrl Pts',(0.00212202413257601,-0.0366650992552675,
-0.0142964696075283));
#31198=CARTESIAN_POINT('Ctrl Pts',(0.00250885034003301,-0.0366942029050504,
-0.0139093865981128));
#31199=CARTESIAN_POINT('Ctrl Pts',(0.00278797466275618,-0.0367233065548334,
-0.0134121234152743));
#31200=CARTESIAN_POINT('Ctrl Pts',(0.00291652844246022,-0.0367524102046163,
-0.0128786063330264));
#31201=CARTESIAN_POINT('Ctrl Pts',(0.00297202056516426,-0.0367649732215,
-0.0126483058668639));
#31202=CARTESIAN_POINT('Ctrl Pts',(0.00300003568403275,-0.0367775362383838,
-0.0124116088997408));
#31203=CARTESIAN_POINT('Ctrl Pts',(0.00299999996570114,-0.0367900992552675,
-0.0121753996422144));
#31204=CARTESIAN_POINT('Ctrl Pts',(0.00299991722014538,-0.0368192029050504,
-0.0116281941763492));
#31205=CARTESIAN_POINT('Ctrl Pts',(0.00284578558050993,-0.0368483065548334,
-0.0110791835577832));
#31206=CARTESIAN_POINT('Ctrl Pts',(0.00255951579718336,-0.0368774102046163,
-0.0106109638706667));
#31207=CARTESIAN_POINT('Ctrl Pts',(0.00243594325050775,-0.0368899732215001,
-0.0104088499819136));
#31208=CARTESIAN_POINT('Ctrl Pts',(0.00228841242440986,-0.0369025362383838,
-0.0102216348455878));
#31209=CARTESIAN_POINT('Ctrl Pts',(0.00212138269847324,-0.0369150992552675,
-0.010054595299745));
#31210=CARTESIAN_POINT('Ctrl Pts',(0.00173436662701786,-0.0369442083818778,
-0.0096675564750851));
#31211=CARTESIAN_POINT('Ctrl Pts',(0.00123709764722942,-0.036973317508488,
-0.00938822529176232));
#31212=CARTESIAN_POINT('Ctrl Pts',(0.000703513242994816,-0.0370024266350983,
-0.00925950812232754));
#31213=CARTESIAN_POINT('Ctrl Pts',(0.000473327445277312,-0.0370149841751547,
-0.00920398014195341));
#31214=CARTESIAN_POINT('Ctrl Pts',(0.000236741851205871,-0.0370275417152111,
-0.00917590293724171));
#31215=CARTESIAN_POINT('Ctrl Pts',(6.30013261930167E-7,-0.0370400992552675,
-0.00917585335271088));
#31216=CARTESIAN_POINT('Ctrl Pts',(-0.000544674758284476,-0.0370691011323918,
-0.00917573883629573));
#31217=CARTESIAN_POINT('Ctrl Pts',(-0.00109198412557387,-0.0370981030095161,
-0.00932863813475086));
#31218=CARTESIAN_POINT('Ctrl Pts',(-0.00155918934501321,-0.0371271048866403,
-0.00961286117061289));
#31219=CARTESIAN_POINT('Ctrl Pts',(-0.00176321254502702,-0.0371397696761827,
-0.00973697813438268));
#31220=CARTESIAN_POINT('Ctrl Pts',(-0.00195211634701312,-0.0371524344657251,
-0.0098854607582095));
#31221=CARTESIAN_POINT('Ctrl Pts',(-0.00212049156426993,-0.0371650992552675,
-0.0100537044873783));
#31222=CARTESIAN_POINT('Ctrl Pts',(-0.00251329948777596,-0.0371946453473993,
-0.0104462056581232));
#31223=CARTESIAN_POINT('Ctrl Pts',(-0.00279503440366669,-0.0372241914395311,
-0.0109517773932172));
#31224=CARTESIAN_POINT('Ctrl Pts',(-0.00292160434126632,-0.037253737531663,
-0.011494510441073));
#31225=CARTESIAN_POINT('Ctrl Pts',(-0.00297352661767779,-0.0372658581061978,
-0.0117171536363121));
#31226=CARTESIAN_POINT('Ctrl Pts',(-0.00299986903456971,-0.0372779786807327,
-0.0119457247437539));
#31227=CARTESIAN_POINT('Ctrl Pts',(-0.00299999951055537,-0.0372900992552675,
-0.0121741396157728));
#31228=CARTESIAN_POINT('',(-0.00299999981883512,-0.0352901375595625,-0.0121751042430183));
#31229=CARTESIAN_POINT('Ctrl Pts',(-0.00299999999990529,-0.0352901758638575,
-0.0121758294485129));
#31230=CARTESIAN_POINT('Ctrl Pts',(-0.00300000442417536,-0.03531962354091,
-0.0127326204983985));
#31231=CARTESIAN_POINT('Ctrl Pts',(-0.00284070124558744,-0.0353490857174387,
-0.0132895327727721));
#31232=CARTESIAN_POINT('Ctrl Pts',(-0.00254638511743984,-0.0353785627573661,
-0.0137620193666647));
#31233=CARTESIAN_POINT('Ctrl Pts',(-0.00242551849306003,-0.0353906680753287,
-0.0139560551472655));
#31234=CARTESIAN_POINT('Ctrl Pts',(-0.00228248521019157,-0.0354027758999937,
-0.0141360222982122));
#31235=CARTESIAN_POINT('Ctrl Pts',(-0.00212123128764963,-0.0354148862565662,
-0.0142972626822892));
#31236=CARTESIAN_POINT('Ctrl Pts',(-0.00173579965280455,-0.0354438326192885,
-0.0146826619572847));
#31237=CARTESIAN_POINT('Ctrl Pts',(-0.00124073796889185,-0.0354727934471282,
-0.0149614820143835));
#31238=CARTESIAN_POINT('Ctrl Pts',(-0.0007092914864209,-0.0355017677075181,
-0.0150907984982715));
#31239=CARTESIAN_POINT('Ctrl Pts',(-0.000476980661877979,-0.0355144332054444,
-0.015147326521299));
#31240=CARTESIAN_POINT('Ctrl Pts',(-0.000238089691008945,-0.0355271012700895,
-0.0151758751813239));
#31241=CARTESIAN_POINT('Ctrl Pts',(2.75720825596021E-7,-0.0355397718152056,
-0.0151758532738878));
#31242=CARTESIAN_POINT('Ctrl Pts',(0.000547620237042205,-0.0355688664448895,
-0.0151758029691269));
#31243=CARTESIAN_POINT('Ctrl Pts',(0.00109675921247324,-0.0355979741534132,
-0.0150216280988535));
#31244=CARTESIAN_POINT('Ctrl Pts',(0.00156506425454912,-0.0356270987696597,
-0.0147352621790824));
#31245=CARTESIAN_POINT('Ctrl Pts',(0.00176725681833465,-0.0356396734385167,
-0.0146116225546986));
#31246=CARTESIAN_POINT('Ctrl Pts',(0.00195453657837562,-0.0356522512591675,
-0.0144640047557032));
#31247=CARTESIAN_POINT('Ctrl Pts',(0.00212162119625327,-0.0356648325397757,
-0.0142968727347501));
#31248=CARTESIAN_POINT('Ctrl Pts',(0.00250834357656535,-0.0356939522926649,
-0.0139100406385923));
#31249=CARTESIAN_POINT('Ctrl Pts',(0.00278749542059164,-0.0357230905807174,
-0.0134130907688648));
#31250=CARTESIAN_POINT('Ctrl Pts',(0.00291622194525164,-0.0357522331609794,
-0.0128798771256664));
#31251=CARTESIAN_POINT('Ctrl Pts',(0.00297192783867808,-0.035764844497101,
-0.0126491310346025));
#31252=CARTESIAN_POINT('Ctrl Pts',(0.00300004532431104,-0.0357774566370209,
-0.012411954683267));
#31253=CARTESIAN_POINT('Ctrl Pts',(0.00299999994485589,-0.0357900684264905,
-0.0121752780781935));
#31254=CARTESIAN_POINT('Ctrl Pts',(0.00299989497427525,-0.0358192416913352,
-0.0116278038835947));
#31255=CARTESIAN_POINT('Ctrl Pts',(0.00284559472580302,-0.0358484130809994,
-0.0110785757190366));
#31256=CARTESIAN_POINT('Ctrl Pts',(0.002559075740545,-0.0358775721901715,
-0.0106102443461921));
#31257=CARTESIAN_POINT('Ctrl Pts',(0.00243550281909295,-0.0358901482374588,
-0.010408257465993));
#31258=CARTESIAN_POINT('Ctrl Pts',(0.00228799813798229,-0.0359027220004333,
-0.0102211624528925));
#31259=CARTESIAN_POINT('Ctrl Pts',(0.00212101329930002,-0.0359152926443287,
-0.0100542259431746));
#31260=CARTESIAN_POINT('Ctrl Pts',(0.00173396166844446,-0.0359444299496015,
-0.00966728633329421));
#31261=CARTESIAN_POINT('Ctrl Pts',(0.00123668840944808,-0.0359735504973407,
-0.00938805148393656));
#31262=CARTESIAN_POINT('Ctrl Pts',(0.000703125243084155,-0.0360026570765507,
-0.00925941455198165));
#31263=CARTESIAN_POINT('Ctrl Pts',(0.000472761400329676,-0.0360152237300586,
-0.00920387605188761));
#31264=CARTESIAN_POINT('Ctrl Pts',(0.000235992071111057,-0.0360277877797665,
-0.00917583020942042));
#31265=CARTESIAN_POINT('Ctrl Pts',(-2.93181185161645E-7,-0.0360403494501322,
-0.00917585330088396));
#31266=CARTESIAN_POINT('Ctrl Pts',(-0.000545584584361914,-0.0360693388635356,
-0.00917590659061083));
#31267=CARTESIAN_POINT('Ctrl Pts',(-0.00109283637569486,-0.036098315605061,
-0.00932896709632053));
#31268=CARTESIAN_POINT('Ctrl Pts',(-0.00155994867156055,-0.0361272789223249,
-0.00961332325900789));
#31269=CARTESIAN_POINT('Ctrl Pts',(-0.00176405935357533,-0.0361399348136222,
-0.00973757631510365));
#31270=CARTESIAN_POINT('Ctrl Pts',(-0.00195302492857976,-0.0361525881417386,
-0.00988622044894215));
#31271=CARTESIAN_POINT('Ctrl Pts',(-0.00212142793965345,-0.036165238843901,
-0.01005464054455));
#31272=CARTESIAN_POINT('Ctrl Pts',(-0.00251406372729111,-0.0361947342690484,
-0.0104473161652017));
#31273=CARTESIAN_POINT('Ctrl Pts',(-0.00279557613143336,-0.0362242154194899,
-0.0109530141278591));
#31274=CARTESIAN_POINT('Ctrl Pts',(-0.00292190601481382,-0.0362536825604244,
-0.0114958053172245));
#31275=CARTESIAN_POINT('Ctrl Pts',(-0.00297375949271995,-0.0362657776696774,
-0.0117185998785131));
#31276=CARTESIAN_POINT('Ctrl Pts',(-0.00300000084973987,-0.0362778704186345,
-0.0119473179106401));
#31277=CARTESIAN_POINT('Ctrl Pts',(-0.00299999999997926,-0.0362899608256352,
-0.0121758644408811));
#31278=CARTESIAN_POINT('',(-0.00299999994316498,-0.0342901216939704,-0.0121754481730699));
#31279=CARTESIAN_POINT('Ctrl Pts',(-0.0029999999999601,-0.0342901441326733,
-0.0121758687597579));
#31280=CARTESIAN_POINT('Ctrl Pts',(-0.00299999712813671,-0.0343196842733559,
-0.0127326682745884));
#31281=CARTESIAN_POINT('Ctrl Pts',(-0.00284068199001415,-0.0343492244140385,
-0.0132895859952222));
#31282=CARTESIAN_POINT('Ctrl Pts',(-0.00254635150369563,-0.0343787645547211,
-0.0137620733279228));
#31283=CARTESIAN_POINT('Ctrl Pts',(-0.00242554449866458,-0.0343908892108132,
-0.0139560042397105));
#31284=CARTESIAN_POINT('Ctrl Pts',(-0.00228259454224132,-0.0344030138669054,
-0.0141358810797341));
#31285=CARTESIAN_POINT('Ctrl Pts',(-0.0021214410730114,-0.0344151385229976,
-0.0142970528937946));
#31286=CARTESIAN_POINT('Ctrl Pts',(-0.00173604568796275,-0.0344441344020535,
-0.0146824921501484));
#31287=CARTESIAN_POINT('Ctrl Pts',(-0.00124100978379169,-0.0344731302811094,
-0.0149613609980348));
#31288=CARTESIAN_POINT('Ctrl Pts',(-0.000709575571708124,-0.0345021261601653,
-0.0150907293573431));
#31289=CARTESIAN_POINT('Ctrl Pts',(-0.000477380634872773,-0.0345147950778842,
-0.0151472531515119));
#31290=CARTESIAN_POINT('Ctrl Pts',(-0.000238609269103201,-0.034527463995603,
-0.0151758249166817));
#31291=CARTESIAN_POINT('Ctrl Pts',(-3.56957372812207E-7,-0.0345401329133219,
-0.0151758532653217));
#31292=CARTESIAN_POINT('Ctrl Pts',(0.000546957897806089,-0.03456923603856,
-0.0151759183880131));
#31293=CARTESIAN_POINT('Ctrl Pts',(0.00109610222331674,-0.0345983391637982,
-0.0150218755290798));
#31294=CARTESIAN_POINT('Ctrl Pts',(0.00156445073765424,-0.0346274422890363,
-0.0147356372402255));
#31295=CARTESIAN_POINT('Ctrl Pts',(0.00176660223010131,-0.0346400039605729,
-0.0146120892935233));
#31296=CARTESIAN_POINT('Ctrl Pts',(0.00195385675957504,-0.0346525656321095,
-0.0144645766535138));
#31297=CARTESIAN_POINT('Ctrl Pts',(0.00212093622771983,-0.0346651273036461,
-0.0142975576764168));
#31298=CARTESIAN_POINT('Ctrl Pts',(0.00250795646106377,-0.034694224960607,
-0.0139106775635777));
#31299=CARTESIAN_POINT('Ctrl Pts',(0.00278733463553876,-0.0347233226175679,
-0.013413563544606));
#31300=CARTESIAN_POINT('Ctrl Pts',(0.00291616377405434,-0.0347524202745288,
-0.0128801180399663));
#31301=CARTESIAN_POINT('Ctrl Pts',(0.00297180446698019,-0.0347649874143427,
-0.0126497254606296));
#31302=CARTESIAN_POINT('Ctrl Pts',(0.00299994245192145,-0.0347775545541565,
-0.0124129153826804));
#31303=CARTESIAN_POINT('Ctrl Pts',(0.00299999991133221,-0.0347901216939704,
-0.012176582674498));
#31304=CARTESIAN_POINT('Ctrl Pts',(0.00300013295148676,-0.0348192193509313,
-0.0116293835366518));
#31305=CARTESIAN_POINT('Ctrl Pts',(0.00284622122408974,-0.0348483170078922,
-0.0110803172019551));
#31306=CARTESIAN_POINT('Ctrl Pts',(0.00256014128152566,-0.0348774146648531,
-0.0106119873656339));
#31307=CARTESIAN_POINT('Ctrl Pts',(0.00243658471334654,-0.034889981804667,
-0.0104097179341138));
#31308=CARTESIAN_POINT('Ctrl Pts',(0.0022890386047289,-0.0349025489444808,
-0.0102223534133573));
#31309=CARTESIAN_POINT('Ctrl Pts',(0.00212196767400703,-0.0349151160842947,
-0.0100551804710419));
#31310=CARTESIAN_POINT('Ctrl Pts',(0.00173506291345904,-0.0349442192095328,
-0.00966803947088609));
#31311=CARTESIAN_POINT('Ctrl Pts',(0.00123787708173055,-0.034973322334771,
-0.0093885723356771));
#31312=CARTESIAN_POINT('Ctrl Pts',(0.000704333931740814,-0.0350024254600091,
-0.00925970622020521));
#31313=CARTESIAN_POINT('Ctrl Pts',(0.00047404272603916,-0.0350149871315457,
-0.00920408422766968));
#31314=CARTESIAN_POINT('Ctrl Pts',(0.000237337238801211,-0.0350275488030823,
-0.00917594025174976));
#31315=CARTESIAN_POINT('Ctrl Pts',(1.10181849570871E-6,-0.0350401104746189,
-0.0091758534888921));
#31316=CARTESIAN_POINT('Ctrl Pts',(-0.000544196126601482,-0.0350691063536748,
-0.00917565321575806));
#31317=CARTESIAN_POINT('Ctrl Pts',(-0.00109152410457655,-0.0350981022327307,
-0.00932846278863097));
#31318=CARTESIAN_POINT('Ctrl Pts',(-0.00155877106600548,-0.0351270981117866,
-0.00961260675846444));
#31319=CARTESIAN_POINT('Ctrl Pts',(-0.00176292122463022,-0.0351397670295055,
-0.00973675531651256));
#31320=CARTESIAN_POINT('Ctrl Pts',(-0.00195194004144232,-0.0351524359472243,
-0.00988529763263816));
#31321=CARTESIAN_POINT('Ctrl Pts',(-0.00212040937062949,-0.0351651048649432,
-0.0100536223611057));
#31322=CARTESIAN_POINT('Ctrl Pts',(-0.0025132296411,-0.0351946450056258,
-0.0104461054657901));
#31323=CARTESIAN_POINT('Ctrl Pts',(-0.00279498358199015,-0.0352241851463083,
-0.0109516626246059));
#31324=CARTESIAN_POINT('Ctrl Pts',(-0.0029215756990028,-0.0352537252869909,
-0.011494387634455));
#31325=CARTESIAN_POINT('Ctrl Pts',(-0.00297353502781077,-0.0352658499430831,
-0.0117171473757763));
#31326=CARTESIAN_POINT('Ctrl Pts',(-0.00299988733115571,-0.0352779745991753,
-0.011945842488321));
#31327=CARTESIAN_POINT('Ctrl Pts',(-0.00299999963776494,-0.0352900992552675,
-0.0121743790375236));
#31328=CARTESIAN_POINT('',(-0.00299998807114563,-0.0332900774868462,-0.0121782217945205));
#31329=CARTESIAN_POINT('Ctrl Pts',(-0.0029999990241015,-0.0332900992552675,
-0.012178273077878));
#31330=CARTESIAN_POINT('Ctrl Pts',(-0.00299954990966587,-0.033319643576341,
-0.0127350743431392));
#31331=CARTESIAN_POINT('Ctrl Pts',(-0.00283978743580498,-0.0333491878974145,
-0.0132918658231327));
#31332=CARTESIAN_POINT('Ctrl Pts',(-0.00254507661055699,-0.033378732218488,
-0.0137641180775787));
#31333=CARTESIAN_POINT('Ctrl Pts',(-0.00242415366009201,-0.0333908545640812,
-0.0139578881432805));
#31334=CARTESIAN_POINT('Ctrl Pts',(-0.00228111365948316,-0.0334029769096743,
-0.0141375956861433));
#31335=CARTESIAN_POINT('Ctrl Pts',(-0.0021198956782073,-0.0334150992552675,
-0.0142985973393157));
#31336=CARTESIAN_POINT('Ctrl Pts',(-0.00173421667443884,-0.033444099334134,
-0.0146837588250832));
#31337=CARTESIAN_POINT('Ctrl Pts',(-0.0012389737994231,-0.0334730994130005,
-0.0149622678449037));
#31338=CARTESIAN_POINT('Ctrl Pts',(-0.000707441773154454,-0.033502099491867,
-0.0150912479661163));
#31339=CARTESIAN_POINT('Ctrl Pts',(-0.000475280436272606,-0.0335147660796672,
-0.015147583607041));
#31340=CARTESIAN_POINT('Ctrl Pts',(-0.000236567380074324,-0.0335274326674673,
-0.0151759805508666));
#31341=CARTESIAN_POINT('Ctrl Pts',(1.60841856303651E-6,-0.0335400992552675,
-0.0151758528553897));
#31342=CARTESIAN_POINT('Ctrl Pts',(0.000548927193259567,-0.0335692065841986,
-0.0151755594161218));
#31343=CARTESIAN_POINT('Ctrl Pts',(0.00109797366274001,-0.0335983139131297,
-0.0150211546781943));
#31344=CARTESIAN_POINT('Ctrl Pts',(0.00156613626676192,-0.0336274212420608,
-0.014734606341062));
#31345=CARTESIAN_POINT('Ctrl Pts',(0.00176814079534584,-0.0336399805797964,
-0.0146109654067762));
#31346=CARTESIAN_POINT('Ctrl Pts',(0.00195524231623712,-0.033652539917532,
-0.0144633852168754));
#31347=CARTESIAN_POINT('Ctrl Pts',(0.0021221706331302,-0.0336650992552675,
-0.0142963229995886));
#31348=CARTESIAN_POINT('Ctrl Pts',(0.00250896839453303,-0.0336942011105502,
-0.0139092149710394));
#31349=CARTESIAN_POINT('Ctrl Pts',(0.00278805792401258,-0.033723302965833,
-0.0134119347801851));
#31350=CARTESIAN_POINT('Ctrl Pts',(0.00291657551373059,-0.0337524048211157,
-0.0128784109515986));
#31351=CARTESIAN_POINT('Ctrl Pts',(0.00297206336007698,-0.0337649696324996,
-0.0126480604736002));
#31352=CARTESIAN_POINT('Ctrl Pts',(0.00300006266320082,-0.0337775344438836,
-0.01241131275598));
#31353=CARTESIAN_POINT('Ctrl Pts',(0.00299999989411969,-0.0337900992552675,
-0.0121750562408696));
#31354=CARTESIAN_POINT('Ctrl Pts',(0.00299985451217487,-0.0338192011105503,
-0.0116278532067562));
#31355=CARTESIAN_POINT('Ctrl Pts',(0.00284566133290258,-0.033848302965833,
-0.0110788621567055));
#31356=CARTESIAN_POINT('Ctrl Pts',(0.00255933993882043,-0.0338774048211158,
-0.0106106762749844));
#31357=CARTESIAN_POINT('Ctrl Pts',(0.0024357198370479,-0.0338899696324997,
-0.0104085356472037));
#31358=CARTESIAN_POINT('Ctrl Pts',(0.00228813344676387,-0.0339025344438836,
-0.0102213024932187));
#31359=CARTESIAN_POINT('Ctrl Pts',(0.002121043592747,-0.0339150992552675,
-0.0100542562282864));
#31360=CARTESIAN_POINT('Ctrl Pts',(0.00173396740088748,-0.0339442065841986,
-0.00966728101381411));
#31361=CARTESIAN_POINT('Ctrl Pts',(0.00123665610771317,-0.0339733139131297,
-0.00938802977500934));
#31362=CARTESIAN_POINT('Ctrl Pts',(0.000703053329552393,-0.0340024212420608,
-0.00925939721526106));
#31363=CARTESIAN_POINT('Ctrl Pts',(0.00047281243306158,-0.0340149805797964,
-0.00920389436353972));
#31364=CARTESIAN_POINT('Ctrl Pts',(0.00023617348649114,-0.0340275399175319,
-0.00917585441442896));
#31365=CARTESIAN_POINT('Ctrl Pts',(1.43272443721777E-8,-0.0340400992552675,
-0.0091758532865923));
#31366=CARTESIAN_POINT('Ctrl Pts',(-0.000545287852488846,-0.034069099334134,
-0.00917585068236644));
#31367=CARTESIAN_POINT('Ctrl Pts',(-0.0010925637511624,-0.0340980994130005,
-0.00932886090342198));
#31368=CARTESIAN_POINT('Ctrl Pts',(-0.00155970950087997,-0.034127099491867,
-0.0096131776783578));
#31369=CARTESIAN_POINT('Ctrl Pts',(-0.0017637483478606,-0.0341397660796672,
-0.00973736090590557));
#31370=CARTESIAN_POINT('Ctrl Pts',(-0.00195265675439628,-0.0341524326674673,
-0.00988591653299666));
#31371=CARTESIAN_POINT('Ctrl Pts',(-0.00212102332822392,-0.0341650992552675,
-0.0100542359692433));
#31372=CARTESIAN_POINT('Ctrl Pts',(-0.00251373178244158,-0.034194643576341,
-0.0104468344768953));
#31373=CARTESIAN_POINT('Ctrl Pts',(-0.00279533977602888,-0.0342241878974145,
-0.0109524753987744));
#31374=CARTESIAN_POINT('Ctrl Pts',(-0.00292177413971409,-0.0342537322184881,
-0.0114952389489939));
#31375=CARTESIAN_POINT('Ctrl Pts',(-0.0029736514885835,-0.0342658545640812,
-0.0117179405407735));
#31376=CARTESIAN_POINT('Ctrl Pts',(-0.00299993700613952,-0.0342779769096744,
-0.01194656610685));
#31377=CARTESIAN_POINT('Ctrl Pts',(-0.00299999988636987,-0.0342900992552675,
-0.0121750275863819));
#31378=CARTESIAN_POINT('',(-0.00299999923530355,-0.0322900992552675,-0.0121737112832657));
#31379=CARTESIAN_POINT('Ctrl Pts',(-0.00299928376163152,-0.0322889717262675,
-0.0121758863199214));
#31380=CARTESIAN_POINT('Ctrl Pts',(-0.00299707236492287,-0.0323173669008297,
-0.012733832497412));
#31381=CARTESIAN_POINT('Ctrl Pts',(-0.00284002430592934,-0.0323491139306059,
-0.0132916136153277));
#31382=CARTESIAN_POINT('Ctrl Pts',(-0.00254536692236663,-0.0323804597583334,
-0.0137653979546681));
#31383=CARTESIAN_POINT('Ctrl Pts',(-0.00249618206423861,-0.0323856920727965,
-0.0138444830779797));
#31384=CARTESIAN_POINT('Ctrl Pts',(-0.0024433588192564,-0.0323907730793508,
-0.0139212959050287));
#31385=CARTESIAN_POINT('Ctrl Pts',(-0.00238695367579395,-0.032395720501742,
-0.0139953450637139));
#31386=CARTESIAN_POINT('Ctrl Pts',(-0.00230563882969713,-0.032402852810351,
-0.0141020958947989));
#31387=CARTESIAN_POINT('Ctrl Pts',(-0.00221687403707554,-0.0324097074948069,
-0.0142030993270911));
#31388=CARTESIAN_POINT('Ctrl Pts',(-0.00212192556767052,-0.0324163376568695,
-0.014297658716942));
#31389=CARTESIAN_POINT('Ctrl Pts',(-0.00173712109141055,-0.0324432081904971,
-0.0146808863425696));
#31390=CARTESIAN_POINT('Ctrl Pts',(-0.00124386889560183,-0.0324704443965446,
-0.0149566887355417));
#31391=CARTESIAN_POINT('Ctrl Pts',(-0.000715762144362272,-0.0325008177702179,
-0.0150883592010786));
#31392=CARTESIAN_POINT('Ctrl Pts',(-0.000481664421721094,-0.0325142815965923,
-0.0151467257264998));
#31393=CARTESIAN_POINT('Ctrl Pts',(-0.000240658071332929,-0.0325283955544535,
-0.0151765843830709));
#31394=CARTESIAN_POINT('Ctrl Pts',(-1.19791577169947E-7,-0.032541788645564,
-0.0151769364537194));
#31395=CARTESIAN_POINT('Ctrl Pts',(6.94614908600466E-5,-0.0325456629081396,
-0.0151770382983292));
#31396=CARTESIAN_POINT('Ctrl Pts',(0.000139033018747938,-0.0325494372625684,
-0.0151747452494295));
#31397=CARTESIAN_POINT('Ctrl Pts',(0.000208448528243256,-0.0325531337590053,
-0.0151699393817332));
#31398=CARTESIAN_POINT('Ctrl Pts',(0.000683492535792095,-0.0325784306774321,
-0.0151370504975804));
#31399=CARTESIAN_POINT('Ctrl Pts',(0.00115287566896183,-0.0326000812500363,
-0.0149853965230064));
#31400=CARTESIAN_POINT('Ctrl Pts',(0.00156079505898092,-0.0326251526157813,
-0.0147365832276358));
#31401=CARTESIAN_POINT('Ctrl Pts',(0.00176417689901714,-0.0326376527827804,
-0.0146125290466478));
#31402=CARTESIAN_POINT('Ctrl Pts',(0.00195273924601373,-0.0326508722292597,
-0.0144645794174125));
#31403=CARTESIAN_POINT('Ctrl Pts',(0.00212112665312921,-0.0326644232833442,
-0.0142969471212208));
#31404=CARTESIAN_POINT('Ctrl Pts',(0.00231445119514261,-0.0326799811648364,
-0.0141044895173947));
#31405=CARTESIAN_POINT('Ctrl Pts',(0.00248237593275498,-0.0326956646976751,
-0.0138857000773177));
#31406=CARTESIAN_POINT('Ctrl Pts',(0.00261628761582927,-0.0327103721403783,
-0.0136471685813781));
#31407=CARTESIAN_POINT('Ctrl Pts',(0.00267475686196265,-0.032716793783865,
-0.0135430196645213));
#31408=CARTESIAN_POINT('Ctrl Pts',(0.00272676038214198,-0.0327230293438048,
-0.0134350970847119));
#31409=CARTESIAN_POINT('Ctrl Pts',(0.00277240400992479,-0.0327289871122913,
-0.0133243027587875));
#31410=CARTESIAN_POINT('Ctrl Pts',(0.00284749445580838,-0.0327387885131408,
-0.0131420298821745));
#31411=CARTESIAN_POINT('Ctrl Pts',(0.00290434841955195,-0.0327482951808992,
-0.0129517210769552));
#31412=CARTESIAN_POINT('Ctrl Pts',(0.00294186480225773,-0.0327579060333934,
-0.0127609850341249));
#31413=CARTESIAN_POINT('Ctrl Pts',(0.00296062299361062,-0.0327627114596405,
-0.0126656170127098));
#31414=CARTESIAN_POINT('Ctrl Pts',(0.00297478607666181,-0.0327675320197591,
-0.0125702102217573));
#31415=CARTESIAN_POINT('Ctrl Pts',(0.0029845603754328,-0.0327726924870258,
-0.0124697194406367));
#31416=CARTESIAN_POINT('Ctrl Pts',(0.00299433467420379,-0.0327778529542926,
-0.0123692286595161));
#31417=CARTESIAN_POINT('Ctrl Pts',(0.00299882345649107,-0.0327833774686131,
-0.0122635383972968));
#31418=CARTESIAN_POINT('Ctrl Pts',(0.00299882727697248,-0.0327880563174707,
-0.0121757451535895));
#31419=CARTESIAN_POINT('Ctrl Pts',(0.00299883109745389,-0.0327927351663284,
-0.0120879519098822));
#31420=CARTESIAN_POINT('Ctrl Pts',(0.00299567769338781,-0.0327965359930861,
-0.012018041578474));
#31421=CARTESIAN_POINT('Ctrl Pts',(0.00298989568302409,-0.0328006876304326,
-0.0119428049059826));
#31422=CARTESIAN_POINT('Ctrl Pts',(0.00298411367266037,-0.0328048392677792,
-0.0118675682334912));
#31423=CARTESIAN_POINT('Ctrl Pts',(0.00297496288616724,-0.032809356386336,
-0.0117870879822373));
#31424=CARTESIAN_POINT('Ctrl Pts',(0.00296250651140142,-0.03281391386738,
-0.0117073372799718));
#31425=CARTESIAN_POINT('Ctrl Pts',(0.00293759376186978,-0.032823028829468,
-0.0115478358754407));
#31426=CARTESIAN_POINT('Ctrl Pts',(0.00290023790677386,-0.0328323084983074,
-0.0113910507489261));
#31427=CARTESIAN_POINT('Ctrl Pts',(0.00284915939399223,-0.0328416873337566,
-0.0112351214523587));
#31428=CARTESIAN_POINT('Ctrl Pts',(0.00280089480223856,-0.0328505494881035,
-0.0110877823183193));
#31429=CARTESIAN_POINT('Ctrl Pts',(0.00274055321868181,-0.0328592599446676,
-0.0109411939081582));
#31430=CARTESIAN_POINT('Ctrl Pts',(0.00266693795030175,-0.0328677954873264,
-0.0107985473240077));
#31431=CARTESIAN_POINT('Ctrl Pts',(0.00258473885082951,-0.0328773263079768,
-0.010639267584655));
#31432=CARTESIAN_POINT('Ctrl Pts',(0.00248593869287483,-0.0328866390452035,
-0.0104849338592383));
#31433=CARTESIAN_POINT('Ctrl Pts',(0.00237225614196163,-0.0328957013778296,
-0.0103388482527745));
#31434=CARTESIAN_POINT('Ctrl Pts',(0.00215676260346663,-0.0329128796880359,
-0.0100619323672036));
#31435=CARTESIAN_POINT('Ctrl Pts',(0.00188566631662303,-0.0329304353752007,
-0.0098149684751571));
#31436=CARTESIAN_POINT('Ctrl Pts',(0.00156935168882271,-0.0329504815267945,
-0.00962048083750371));
#31437=CARTESIAN_POINT('Ctrl Pts',(0.00125303706102239,-0.0329705276783882,
-0.00942599319985031));
#31438=CARTESIAN_POINT('Ctrl Pts',(0.000891738231477182,-0.0329932455839496,
-0.00928410707949561));
#31439=CARTESIAN_POINT('Ctrl Pts',(0.00050374597097403,-0.0330150737761611,
-0.00921745827629187));
#31440=CARTESIAN_POINT('Ctrl Pts',(0.000441300376803264,-0.0330185869246723,
-0.00920673145377373));
#31441=CARTESIAN_POINT('Ctrl Pts',(0.000378291871362253,-0.0330220258529512,
-0.00919792040728071));
#31442=CARTESIAN_POINT('Ctrl Pts',(0.000314806651507004,-0.0330254091399757,
-0.00919118498220827));
#31443=CARTESIAN_POINT('Ctrl Pts',(-0.000134903341485572,-0.0330493753164735,
-0.0091434732790901));
#31444=CARTESIAN_POINT('Ctrl Pts',(-0.000611424908498898,-0.0330705494844869,
-0.00920099273624149));
#31445=CARTESIAN_POINT('Ctrl Pts',(-0.00105907198302849,-0.0330955355600564,
-0.00937022262920045));
#31446=CARTESIAN_POINT('Ctrl Pts',(-0.00133351553764533,-0.0331108540280759,
-0.00947397412454952));
#31447=CARTESIAN_POINT('Ctrl Pts',(-0.00159729233888611,-0.033127593814194,
-0.00961938212286541));
#31448=CARTESIAN_POINT('Ctrl Pts',(-0.00183679345966173,-0.0331449433303733,
-0.00980394576024457));
#31449=CARTESIAN_POINT('Ctrl Pts',(-0.00201242281432988,-0.0331576659611506,
-0.00993928872825712));
#31450=CARTESIAN_POINT('Ctrl Pts',(-0.00217675104965253,-0.0331699846688671,
-0.0100954580292239));
#31451=CARTESIAN_POINT('Ctrl Pts',(-0.00232166018894287,-0.0331820424692315,
-0.0102718389100069));
#31452=CARTESIAN_POINT('Ctrl Pts',(-0.00251064840497445,-0.0331977680624638,
-0.0105018720753718));
#31453=CARTESIAN_POINT('Ctrl Pts',(-0.00266639130070364,-0.0332130498792843,
-0.0107665103491488));
#31454=CARTESIAN_POINT('Ctrl Pts',(-0.00278109594182748,-0.0332282051689312,
-0.0110521365491834));
#31455=CARTESIAN_POINT('Ctrl Pts',(-0.00292162366242661,-0.0332467723192073,
-0.0114020648384051));
#31456=CARTESIAN_POINT('Ctrl Pts',(-0.00299867836658016,-0.0332669737194449,
-0.0117854146205141));
#31457=CARTESIAN_POINT('Ctrl Pts',(-0.00299949806419125,-0.0332891036239059,
-0.0121759275095697));
#31458=CARTESIAN_POINT('',(-0.00299999999422887,-0.0312900992552675,-0.012176039369213));
#31459=CARTESIAN_POINT('Ctrl Pts',(-0.00299999999422887,-0.0312900992552675,
-0.012176039369213));
#31460=CARTESIAN_POINT('Ctrl Pts',(-0.00299996545726101,-0.0313196420846964,
-0.012732839805292));
#31461=CARTESIAN_POINT('Ctrl Pts',(-0.0028406181462586,-0.0313491849141254,
-0.0132897492385463));
#31462=CARTESIAN_POINT('Ctrl Pts',(-0.0025462599484267,-0.0313787277435543,
-0.0137622202917111));
#31463=CARTESIAN_POINT('Ctrl Pts',(-0.00242546072407741,-0.031390851580792,
-0.0139561137764863));
#31464=CARTESIAN_POINT('Ctrl Pts',(-0.00228252633754426,-0.0314029754180298,
-0.0141359563616402));
#31465=CARTESIAN_POINT('Ctrl Pts',(-0.002121394537641,-0.0314150992552675,
-0.0142970994334413));
#31466=CARTESIAN_POINT('Ctrl Pts',(-0.00173598925954655,-0.0314440978195793,
-0.0146825316723773));
#31467=CARTESIAN_POINT('Ctrl Pts',(-0.00124094532465347,-0.0314730963838911,
-0.0149613900299818));
#31468=CARTESIAN_POINT('Ctrl Pts',(-0.000709506489134427,-0.0315020949482029,
-0.0150907461734197));
#31469=CARTESIAN_POINT('Ctrl Pts',(-0.000477345976244627,-0.0315147630505578,
-0.0151472557594695));
#31470=CARTESIAN_POINT('Ctrl Pts',(-0.000238611731454913,-0.0315274311529127,
-0.0151758218207988));
#31471=CARTESIAN_POINT('Ctrl Pts',(-3.95938876176992E-7,-0.0315400992552675,
-0.0151758532604302));
#31472=CARTESIAN_POINT('Ctrl Pts',(0.000546920822706506,-0.0315692050701306,
-0.0151759254950919));
#31473=CARTESIAN_POINT('Ctrl Pts',(0.0010960686685288,-0.0315983108849936,
-0.0150218887442718));
#31474=CARTESIAN_POINT('Ctrl Pts',(0.0015644217207454,-0.0316274166998567,
-0.014735654974123));
#31475=CARTESIAN_POINT('Ctrl Pts',(0.00176654330051676,-0.0316399775516603,
-0.0146121284559705));
#31476=CARTESIAN_POINT('Ctrl Pts',(0.00195377283282597,-0.0316525384034639,
-0.0144646445384834));
#31477=CARTESIAN_POINT('Ctrl Pts',(0.0021208345411987,-0.0316650992552675,
-0.0142976593212508));
#31478=CARTESIAN_POINT('Ctrl Pts',(0.00250787462741079,-0.0316941995991603,
-0.0139107964458297));
#31479=CARTESIAN_POINT('Ctrl Pts',(0.00278727696472124,-0.0317232999430531,
-0.0134136940661085));
#31480=CARTESIAN_POINT('Ctrl Pts',(0.00291613115480297,-0.0317524002869459,
-0.0128802530934771));
#31481=CARTESIAN_POINT('Ctrl Pts',(0.00297177391109823,-0.0317649666097197,
-0.0126498987214601));
#31482=CARTESIAN_POINT('Ctrl Pts',(0.00299992281111363,-0.0317775329324936,
-0.0124131275687113));
#31483=CARTESIAN_POINT('Ctrl Pts',(0.00299999984059891,-0.0317900992552675,
-0.0121768312469505));
#31484=CARTESIAN_POINT('Ctrl Pts',(0.00300017822090568,-0.0318191995991603,
-0.0116296302600293));
#31485=CARTESIAN_POINT('Ctrl Pts',(0.00284631098608129,-0.0318482999430531,
-0.011080549694383));
#31486=CARTESIAN_POINT('Ctrl Pts',(0.00256026832300205,-0.0318774002869458,
-0.0106121953590585));
#31487=CARTESIAN_POINT('Ctrl Pts',(0.00243674729367678,-0.0318899666097197,
-0.0104099471735415));
#31488=CARTESIAN_POINT('Ctrl Pts',(0.00228924297230858,-0.0319025329324936,
-0.010222597311479));
#31489=CARTESIAN_POINT('Ctrl Pts',(0.00212221745188226,-0.0319150992552675,
-0.0100554304308695));
#31490=CARTESIAN_POINT('Ctrl Pts',(0.00173535695478928,-0.0319442050701306,
-0.00966824251871701));
#31491=CARTESIAN_POINT('Ctrl Pts',(0.00123820225068015,-0.0319733108849936,
-0.00938871647213873));
#31492=CARTESIAN_POINT('Ctrl Pts',(0.000704672593883375,-0.0320024166998567,
-0.00925978803772882));
#31493=CARTESIAN_POINT('Ctrl Pts',(0.000474423518797268,-0.0320149775516603,
-0.00920414792026393));
#31494=CARTESIAN_POINT('Ctrl Pts',(0.00023775896460552,-0.0320275384034639,
-0.00917597651420902));
#31495=CARTESIAN_POINT('Ctrl Pts',(1.55998187177509E-6,-0.0320400992552675,
-0.00917585369214869));
#31496=CARTESIAN_POINT('Ctrl Pts',(-0.000543739930768506,-0.0320690978195793,
-0.00917557013945089));
#31497=CARTESIAN_POINT('Ctrl Pts',(-0.00109109283963647,-0.0320980963838911,
-0.00932829719717779));
#31498=CARTESIAN_POINT('Ctrl Pts',(-0.00155838406046309,-0.0321270949482029,
-0.00961237145122268));
#31499=CARTESIAN_POINT('Ctrl Pts',(-0.0017625215119349,-0.0321397630505578,
-0.00973647006824121));
#31500=CARTESIAN_POINT('Ctrl Pts',(-0.00195153599591617,-0.0321524311529126,
-0.0098849571721927));
#31501=CARTESIAN_POINT('Ctrl Pts',(-0.0021200110903683,-0.0321650992552675,
-0.010053224497364));
#31502=CARTESIAN_POINT('Ctrl Pts',(-0.00251290584595237,-0.0321946420846964,
-0.0104456347216228));
#31503=CARTESIAN_POINT('Ctrl Pts',(-0.00279475481519703,-0.0322241849141254,
-0.0109511400793834));
#31504=CARTESIAN_POINT('Ctrl Pts',(-0.00292144843250678,-0.0322537277435543,
-0.0114938422483749));
#31505=CARTESIAN_POINT('Ctrl Pts',(-0.00297344117744736,-0.032265851580792,
-0.0117165572994583));
#31506=CARTESIAN_POINT('Ctrl Pts',(-0.0029998360855368,-0.0322779754180298,
-0.0119452106188514));
#31507=CARTESIAN_POINT('Ctrl Pts',(-0.00299999923530355,-0.0322900992552675,
-0.0121737112832657));
#31508=CARTESIAN_POINT('Ctrl Pts',(-0.00112535951647366,-0.0304787743898623,
-0.0149567822606029));
#31509=CARTESIAN_POINT('Ctrl Pts',(-0.000605826549099741,-0.0305085119470451,
-0.0151670218511904));
#31510=CARTESIAN_POINT('Ctrl Pts',(-2.6152100817094E-5,-0.0305382495042279,
-0.0152275772346542));
#31511=CARTESIAN_POINT('Ctrl Pts',(0.000525287215145681,-0.0305679870614107,
-0.015129507521841));
#31512=CARTESIAN_POINT('Ctrl Pts',(0.000600707865615942,-0.0305720542830272,
-0.0151160944747156));
#31513=CARTESIAN_POINT('Ctrl Pts',(0.000675597023227879,-0.0305761215046438,
-0.0150997942648813));
#31514=CARTESIAN_POINT('Ctrl Pts',(0.000749732422933762,-0.0305801887262604,
-0.0150806598711695));
#31515=CARTESIAN_POINT('Ctrl Pts',(0.00128509963884293,-0.0306095600808629,
-0.0149424812529891));
#31516=CARTESIAN_POINT('Ctrl Pts',(0.00178186922311124,-0.0306389314354654,
-0.0146519824220399));
#31517=CARTESIAN_POINT('Ctrl Pts',(0.00216497392884224,-0.0306683027900679,
-0.0142526026425068));
#31518=CARTESIAN_POINT('Ctrl Pts',(0.00222280121312341,-0.0306727362142648,
-0.0141923187365622));
#31519=CARTESIAN_POINT('Ctrl Pts',(0.00227809198190826,-0.0306771696384616,
-0.0141296356243967));
#31520=CARTESIAN_POINT('Ctrl Pts',(0.00233065306415271,-0.0306816030626585,
-0.0140647832202919));
#31521=CARTESIAN_POINT('Ctrl Pts',(0.00267983604782405,-0.0307110559624626,
-0.0136339443753407));
#31522=CARTESIAN_POINT('Ctrl Pts',(0.00290653022343286,-0.0307405088622667,
-0.0131032252539013));
#31523=CARTESIAN_POINT('Ctrl Pts',(0.00297623693573143,-0.0307699617620708,
-0.0125527003409289));
#31524=CARTESIAN_POINT('Ctrl Pts',(0.00298653660670087,-0.0307743136410661,
-0.0124713563027851));
#31525=CARTESIAN_POINT('Ctrl Pts',(0.00299349653931312,-0.0307786655200613,
-0.0123896120634787));
#31526=CARTESIAN_POINT('Ctrl Pts',(0.00299709913212865,-0.0307830173990565,
-0.012307750186422));
#31527=CARTESIAN_POINT('Ctrl Pts',(0.00302147207072706,-0.0308124595494659,
-0.0117539228167411));
#31528=CARTESIAN_POINT('Ctrl Pts',(0.00288808641085541,-0.0308419016998753,
-0.0111926614903797));
#31529=CARTESIAN_POINT('Ctrl Pts',(0.0026168203245709,-0.0308713438502847,
-0.0107087979403245));
#31530=CARTESIAN_POINT('Ctrl Pts',(0.00257662512439674,-0.0308757064786746,
-0.0106371008383467));
#31531=CARTESIAN_POINT('Ctrl Pts',(0.00253349270277464,-0.0308800691070646,
-0.0105670767113343));
#31532=CARTESIAN_POINT('Ctrl Pts',(0.00248757826106265,-0.0308844317354546,
-0.0104989649792792));
#31533=CARTESIAN_POINT('Ctrl Pts',(0.00217771462428059,-0.030913873885864,
-0.0100392980811281));
#31534=CARTESIAN_POINT('Ctrl Pts',(0.00173661880752667,-0.0309433160362734,
-0.00966749296217343));
#31535=CARTESIAN_POINT('Ctrl Pts',(0.00123072528973799,-0.0309727581866828,
-0.00943992286690203));
#31536=CARTESIAN_POINT('Ctrl Pts',(0.00115576386904273,-0.0309771208150727,
-0.00940620237622671));
#31537=CARTESIAN_POINT('Ctrl Pts',(0.00107943649137909,-0.0309814834434627,
-0.00937557394026337));
#31538=CARTESIAN_POINT('Ctrl Pts',(0.00100201033104887,-0.0309858460718527,
-0.00934813772510723));
#31539=CARTESIAN_POINT('Ctrl Pts',(0.000479292203677936,-0.0310152989716568,
-0.00916291083348046));
#31540=CARTESIAN_POINT('Ctrl Pts',(-9.66640762191366E-5,-0.031044751871461,
-0.00912649295579771));
#31541=CARTESIAN_POINT('Ctrl Pts',(-0.000638860917020236,-0.0310742047712651,
-0.00924466637189296));
#31542=CARTESIAN_POINT('Ctrl Pts',(-0.000718974422259154,-0.0310785566502604,
-0.00926212734893491));
#31543=CARTESIAN_POINT('Ctrl Pts',(-0.000798349784612914,-0.0310829085292556,
-0.00928287002814561));
#31544=CARTESIAN_POINT('Ctrl Pts',(-0.000876714771932716,-0.0310872604082508,
-0.00930681665230697));
#31545=CARTESIAN_POINT('Ctrl Pts',(-0.00140560949384823,-0.0311166317628533,
-0.0094684352980799));
#31546=CARTESIAN_POINT('Ctrl Pts',(-0.00188910772167505,-0.0311460031174558,
-0.00978055728136447));
#31547=CARTESIAN_POINT('Ctrl Pts',(-0.00225421567954084,-0.0311753744720583,
-0.0101963301949746));
#31548=CARTESIAN_POINT('Ctrl Pts',(-0.00230932646611429,-0.0311798078962552,
-0.0102590885430504));
#31549=CARTESIAN_POINT('Ctrl Pts',(-0.00236179690657229,-0.031184241320452,
-0.0103241295731634));
#31550=CARTESIAN_POINT('Ctrl Pts',(-0.00241144471782708,-0.0311886747446489,
-0.0103912148433815));
#31551=CARTESIAN_POINT('Ctrl Pts',(-0.00274446149236254,-0.0312184123018317,
-0.0108411948070944));
#31552=CARTESIAN_POINT('Ctrl Pts',(-0.00294825228095729,-0.0312481498590144,
-0.011387140196714));
#31553=CARTESIAN_POINT('Ctrl Pts',(-0.0029911879473685,-0.0312778874161972,
-0.0119460823930198));
#31554=CARTESIAN_POINT('Ctrl Pts',(-0.0029970602814502,-0.0312819546378138,
-0.0120225292164516));
#31555=CARTESIAN_POINT('Ctrl Pts',(-0.00299999988367143,-0.0312860218594304,
-0.0120991943468039));
#31556=CARTESIAN_POINT('Ctrl Pts',(-0.00299999999999654,-0.031290089081047,
-0.0121758487339766));
#31557=CARTESIAN_POINT('Ctrl Pts',(-0.00176573724564316,-0.0405768567115634,
-0.0104108332259136));
#31558=CARTESIAN_POINT('Ctrl Pts',(-0.00118375689512938,-0.0405243778792318,
-0.00982859805607285));
#31559=CARTESIAN_POINT('Ctrl Pts',(0.000590938148187802,-0.0404194309906651,
-0.00929427447494101));
#31560=CARTESIAN_POINT('Ctrl Pts',(0.002736334709133,-0.0402620160458629,
-0.0110892695029399));
#31561=CARTESIAN_POINT('Ctrl Pts',(0.00240943420965453,-0.040104611877157,
-0.0138634638989389));
#31562=CARTESIAN_POINT('Ctrl Pts',(-8.4854924110494E-5,-0.039947207708451,
-0.0151169866770628));
#31563=CARTESIAN_POINT('Ctrl Pts',(-0.00250442120103688,-0.039789803539745,
-0.013720818532592));
#31564=CARTESIAN_POINT('Ctrl Pts',(-0.00266674786335135,-0.039632399371039,
-0.0109326563015306));
#31565=CARTESIAN_POINT('Ctrl Pts',(-0.000426928585076152,-0.039474995202333,
-0.00926458117117055));
#31566=CARTESIAN_POINT('Ctrl Pts',(0.00219776514813444,-0.039317591033627,
-0.0102193949058226));
#31567=CARTESIAN_POINT('Ctrl Pts',(0.00284226643201514,-0.039160186864921,
-0.0129368842307664));
#31568=CARTESIAN_POINT('Ctrl Pts',(0.000926095137602526,-0.0390027826962151,
-0.014968719980181));
#31569=CARTESIAN_POINT('Ctrl Pts',(-0.00182447151375588,-0.0388453785275091,
-0.0144843301313878));
#31570=CARTESIAN_POINT('Ctrl Pts',(-0.00293126780897562,-0.0386879743588031,
-0.0119201214729091));
#31571=CARTESIAN_POINT('Ctrl Pts',(-0.00139715250182972,-0.0385305701900971,
-0.00958631446602781));
#31572=CARTESIAN_POINT('Ctrl Pts',(0.00139572892480361,-0.0383731660213911,
-0.00958554709051689));
#31573=CARTESIAN_POINT('Ctrl Pts',(0.00293112889605655,-0.0382157618526851,
-0.0119185111592916));
#31574=CARTESIAN_POINT('Ctrl Pts',(0.00182573516943588,-0.0380583576839792,
-0.0144833270353835));
#31575=CARTESIAN_POINT('Ctrl Pts',(-0.000924551666121453,-0.0379009535152732,
-0.0149692289983903));
#31576=CARTESIAN_POINT('Ctrl Pts',(-0.00284186518882352,-0.0377435493465672,
-0.0129384445659896));
#31577=CARTESIAN_POINT('Ctrl Pts',(-0.00219880599194375,-0.0375861451778613,
-0.010220605025049));
#31578=CARTESIAN_POINT('Ctrl Pts',(0.000425263234877395,-0.0374287410091553,
-0.00926434256914682));
#31579=CARTESIAN_POINT('Ctrl Pts',(0.00266619234260643,-0.0372713368404493,
-0.010931199992661));
#31580=CARTESIAN_POINT('Ctrl Pts',(0.00250502070384008,-0.0371139326717433,
-0.0137194253613483));
#31581=CARTESIAN_POINT('Ctrl Pts',(8.69555590101293E-5,-0.0369565285030373,
-0.0151169724941598));
#31582=CARTESIAN_POINT('Ctrl Pts',(-0.00240945202080823,-0.0367991243343313,
-0.0138647240387452));
#31583=CARTESIAN_POINT('Ctrl Pts',(-0.00273506852592541,-0.0366417201656253,
-0.0110908907881794));
#31584=CARTESIAN_POINT('Ctrl Pts',(-0.000596530399695241,-0.0364843159969194,
-0.0092945523747685));
#31585=CARTESIAN_POINT('Ctrl Pts',(0.00207945062066594,-0.0363269118282134,
-0.0100941163728396));
#31586=CARTESIAN_POINT('Ctrl Pts',(0.00288195467878527,-0.0361695076595074,
-0.0127692171647587));
#31587=CARTESIAN_POINT('Ctrl Pts',(0.00108796731518194,-0.0360121034908014,
-0.0149097279331455));
#31588=CARTESIAN_POINT('Ctrl Pts',(-0.00168622206938664,-0.0358546993220954,
-0.014587159694891));
#31589=CARTESIAN_POINT('Ctrl Pts',(-0.00294121298424043,-0.0356972951533894,
-0.0120921296722862));
#31590=CARTESIAN_POINT('Ctrl Pts',(-0.00154632382334315,-0.0355398909846835,
-0.00967253027592494));
#31591=CARTESIAN_POINT('Ctrl Pts',(0.00124172275662489,-0.0353824868159775,
-0.00950829484148566));
#31592=CARTESIAN_POINT('Ctrl Pts',(0.00291104165179871,-0.0352250826472715,
-0.0117473909618462));
#31593=CARTESIAN_POINT('Ctrl Pts',(0.00195766327410342,-0.0350676784785655,
-0.0143725093742236));
#31594=CARTESIAN_POINT('Ctrl Pts',(-0.000759467994954353,-0.0349102743098595,
-0.0150185547880869));
#31595=CARTESIAN_POINT('Ctrl Pts',(-0.00279235806187805,-0.0347528701411535,
-0.0131034738536127));
#31596=CARTESIAN_POINT('Ctrl Pts',(-0.00230947860380213,-0.0345954659724475,
-0.0103526549865628));
#31597=CARTESIAN_POINT('Ctrl Pts',(0.000254121077754658,-0.0344380618037416,
-0.00924444305604325));
#31598=CARTESIAN_POINT('Ctrl Pts',(0.0025887708719542,-0.0342806576350356,
-0.0107772794291727));
#31599=CARTESIAN_POINT('Ctrl Pts',(0.00259107262143253,-0.0341232534663297,
-0.0135701581796352));
#31600=CARTESIAN_POINT('Ctrl Pts',(0.000258952568197248,-0.0339658492976236,
-0.0151068406672191));
#31601=CARTESIAN_POINT('Ctrl Pts',(-0.00230647029233221,-0.0338084451289177,
-0.0140028558188922));
#31602=CARTESIAN_POINT('Ctrl Pts',(-0.00279388326509801,-0.0336510409602117,
-0.011252836614041));
#31603=CARTESIAN_POINT('Ctrl Pts',(-0.000764152577578523,-0.0334936367915057,
-0.00933440748064133));
#31604=CARTESIAN_POINT('Ctrl Pts',(0.00195403986518134,-0.0333362326227997,
-0.00997597336214831));
#31605=CARTESIAN_POINT('Ctrl Pts',(0.00291174394389237,-0.0331788284540937,
-0.0125995167845713));
#31606=CARTESIAN_POINT('Ctrl Pts',(0.00124611797408996,-0.0330214242853877,
-0.014841361344239));
#31607=CARTESIAN_POINT('Ctrl Pts',(-0.00154219545170772,-0.0328640201166818,
-0.0146817217666492));
#31608=CARTESIAN_POINT('Ctrl Pts',(-0.00294107108454518,-0.0327066159479758,
-0.0122644246480997));
#31609=CARTESIAN_POINT('Ctrl Pts',(-0.00169019413996331,-0.0325492117792698,
-0.00976732980836716));
#31610=CARTESIAN_POINT('Ctrl Pts',(0.00108345923042443,-0.0323918076105638,
-0.00944018855622451));
#31611=CARTESIAN_POINT('Ctrl Pts',(0.00288097343976189,-0.0322344034418578,
-0.011577740875895));
#31612=CARTESIAN_POINT('Ctrl Pts',(0.00208287772409016,-0.0320769992731518,
-0.0142541579117125));
#31613=CARTESIAN_POINT('Ctrl Pts',(-0.000591777636590497,-0.0319195951044459,
-0.0150581372552976));
#31614=CARTESIAN_POINT('Ctrl Pts',(-0.0027332817459633,-0.0317621909357399,
-0.013265315295727));
#31615=CARTESIAN_POINT('Ctrl Pts',(-0.00241222224189072,-0.0316047867670339,
-0.0104909703753948));
#31616=CARTESIAN_POINT('Ctrl Pts',(8.20876226880905E-5,-0.0314473825983279,
-0.00923456740040116));
#31617=CARTESIAN_POINT('Ctrl Pts',(0.00250251191094569,-0.0312899784296219,
-0.0106282074995115));
#31618=CARTESIAN_POINT('Ctrl Pts',(0.00266816463044997,-0.031132574260916,
-0.0134160066702516));
#31619=CARTESIAN_POINT('Ctrl Pts',(0.000430208913922906,-0.03097517009221,
-0.0150868605785511));
#31620=CARTESIAN_POINT('Ctrl Pts',(-0.00219586682886496,-0.030817765923504,
-0.0141343309731242));
#31621=CARTESIAN_POINT('Ctrl Pts',(-0.00284255863625992,-0.030660361754798,
-0.011418711827452));
#31622=CARTESIAN_POINT('Ctrl Pts',(-0.000930263045673305,-0.0305029575860921,
-0.00938250357249028));
#31623=CARTESIAN_POINT('Ctrl Pts',(0.00182468775185338,-0.0303455303363401,
-0.00986851078086045));
#31624=CARTESIAN_POINT('Ctrl Pts',(0.00255836733623353,-0.0302405711428233,
-0.0115708398779804));
#31625=CARTESIAN_POINT('Ctrl Pts',(0.00248731861744851,-0.0301880800055419,
-0.0123911899040882));
#31626=CARTESIAN_POINT('Ctrl Pts',(-0.00188644671560341,-0.0406753955675595,
-0.0102901727842112));
#31627=CARTESIAN_POINT('Ctrl Pts',(-0.00126468097810125,-0.0406229167352281,
-0.00966813480740289));
#31628=CARTESIAN_POINT('Ctrl Pts',(0.000631335908853008,-0.0405179698466612,
-0.00909728375513973));
#31629=CARTESIAN_POINT('Ctrl Pts',(0.0029233962400536,-0.0403605549018591,
-0.0110149883759423));
#31630=CARTESIAN_POINT('Ctrl Pts',(0.00257414814264154,-0.0402031507331532,
-0.0139788324697851));
#31631=CARTESIAN_POINT('Ctrl Pts',(-9.0655783178371E-5,-0.0400457465644472,
-0.0153180486717205));
#31632=CARTESIAN_POINT('Ctrl Pts',(-0.00267562864228014,-0.0398883423957412,
-0.0138264355695641));
#31633=CARTESIAN_POINT('Ctrl Pts',(-0.00284905229278846,-0.0397309382270353,
-0.0108476687704077));
#31634=CARTESIAN_POINT('Ctrl Pts',(-0.000456114310949391,-0.0395735340583293,
-0.00906556055537634));
#31635=CARTESIAN_POINT('Ctrl Pts',(0.00234800894391053,-0.0394161298896233,
-0.0100856473424632));
#31636=CARTESIAN_POINT('Ctrl Pts',(0.00303656967579679,-0.0392587257209173,
-0.0129889098886754));
#31637=CARTESIAN_POINT('Ctrl Pts',(0.00098940492702264,-0.0391013215522113,
-0.0151596461551195));
#31638=CARTESIAN_POINT('Ctrl Pts',(-0.00194919618042227,-0.0389439173835053,
-0.0146421424089747));
#31639=CARTESIAN_POINT('Ctrl Pts',(-0.00313165537196454,-0.0387865132147993,
-0.0119026391143341));
#31640=CARTESIAN_POINT('Ctrl Pts',(-0.0014926647522315,-0.0386291090460934,
-0.00940928820731397));
#31641=CARTESIAN_POINT('Ctrl Pts',(0.00149114385651963,-0.0384717048773874,
-0.00940846837241741));
#31642=CARTESIAN_POINT('Ctrl Pts',(0.00313150696266941,-0.0383143007086814,
-0.0119009187163291));
#31643=CARTESIAN_POINT('Ctrl Pts',(0.00195054622223225,-0.0381568965399754,
-0.0146410707392416));
#31644=CARTESIAN_POINT('Ctrl Pts',(-0.000987755940621543,-0.0379994923712694,
-0.0151601899708721));
#31645=CARTESIAN_POINT('Ctrl Pts',(-0.00303614100278615,-0.0378420882025634,
-0.012990576891659));
#31646=CARTESIAN_POINT('Ctrl Pts',(-0.00234912094196705,-0.0376846840338575,
-0.0100869401879562));
#31647=CARTESIAN_POINT('Ctrl Pts',(0.00045433511394796,-0.0375272798651515,
-0.00906530564202212));
#31648=CARTESIAN_POINT('Ctrl Pts',(0.00284845879549029,-0.0373698756964455,
-0.0108461129052353));
#31649=CARTESIAN_POINT('Ctrl Pts',(0.00267626912834154,-0.0372124715277395,
-0.0138249471582369));
#31650=CARTESIAN_POINT('Ctrl Pts',(9.29000218480465E-5,-0.0370550673590335,
-0.0153180335192447));
#31651=CARTESIAN_POINT('Ctrl Pts',(-0.00257416717140274,-0.0368976631903275,
-0.0139801787553691));
#31652=CARTESIAN_POINT('Ctrl Pts',(-0.00292204349792889,-0.0367402590216216,
-0.0110167204956124));
#31653=CARTESIAN_POINT('Ctrl Pts',(-0.000637310458302599,-0.0365828548529156,
-0.00909758065277731));
#31654=CARTESIAN_POINT('Ctrl Pts',(0.00222160618930928,-0.0364254506842097,
-0.00995180450844874));
#31655=CARTESIAN_POINT('Ctrl Pts',(0.00307897109364783,-0.0362680465155037,
-0.0128097807533718));
#31656=CARTESIAN_POINT('Ctrl Pts',(0.00116234302327428,-0.0361106423467977,
-0.0150966212890749));
#31657=CARTESIAN_POINT('Ctrl Pts',(-0.00180149571654633,-0.0359532381780916,
-0.0147520016152729));
#31658=CARTESIAN_POINT('Ctrl Pts',(-0.00314228042009149,-0.0357958340093857,
-0.0120864061519114));
#31659=CARTESIAN_POINT('Ctrl Pts',(-0.00165203373548518,-0.0356384298406797,
-0.00950139790926134));
#31660=CARTESIAN_POINT('Ctrl Pts',(0.00132660950642858,-0.0354810256719738,
-0.00932593499899645));
#31661=CARTESIAN_POINT('Ctrl Pts',(0.0031100465126227,-0.0353236215032677,
-0.0117181003863419));
#31662=CARTESIAN_POINT('Ctrl Pts',(0.00209149320647923,-0.0351662173345617,
-0.0145226773523198));
#31663=CARTESIAN_POINT('Ctrl Pts',(-0.000811386806402,-0.0350088131658558,
-0.0152128877741252));
#31664=CARTESIAN_POINT('Ctrl Pts',(-0.00298324946569276,-0.0348514089971498,
-0.0131668879245621));
#31665=CARTESIAN_POINT('Ctrl Pts',(-0.00246735936371563,-0.0346940048284438,
-0.0102280173594368));
#31666=CARTESIAN_POINT('Ctrl Pts',(0.000271493323074386,-0.0345366006597379,
-0.00904404575682176));
#31667=CARTESIAN_POINT('Ctrl Pts',(0.00276574463210646,-0.0343791964910318,
-0.0106816700119495));
#31668=CARTESIAN_POINT('Ctrl Pts',(0.00276820373396548,-0.0342217923223258,
-0.0136654757615811));
#31669=CARTESIAN_POINT('Ctrl Pts',(0.00027665510425068,-0.0340643881536199,
-0.0153072090595452));
#31670=CARTESIAN_POINT('Ctrl Pts',(-0.00246414539781781,-0.0339069839849139,
-0.0141277535112517));
#31671=CARTESIAN_POINT('Ctrl Pts',(-0.00298487893497639,-0.0337495798162079,
-0.0111897372748958));
#31672=CARTESIAN_POINT('Ctrl Pts',(-0.000816391636836017,-0.033592175647502,
-0.00914016033656626));
#31673=CARTESIAN_POINT('Ctrl Pts',(0.00208762209378833,-0.0334347714787959,
-0.00982558499586843));
#31674=CARTESIAN_POINT('Ctrl Pts',(0.00311079681486421,-0.0332773673100899,
-0.012628479302303));
#31675=CARTESIAN_POINT('Ctrl Pts',(0.00133130519009939,-0.033119963141384,
-0.0150235810179823));
#31676=CARTESIAN_POINT('Ctrl Pts',(-0.00164762313977976,-0.032962558972678,
-0.0148530281468983));
#31677=CARTESIAN_POINT('Ctrl Pts',(-0.00314212881983791,-0.0328051548039721,
-0.0122704795705587));
#31678=CARTESIAN_POINT('Ctrl Pts',(-0.00180573932612758,-0.0326477506352661,
-0.0096026781348768));
#31679=CARTESIAN_POINT('Ctrl Pts',(0.00115752675646824,-0.03249034646656,
-0.00925317282644791));
#31680=CARTESIAN_POINT('Ctrl Pts',(0.00307792277508429,-0.032332942297854,
-0.0115368526677282));
#31681=CARTESIAN_POINT('Ctrl Pts',(0.00222526757665021,-0.0321755381291481,
-0.0143962351377196));
#31682=CARTESIAN_POINT('Ctrl Pts',(-0.000632232786428663,-0.0320181339604421,
-0.0152551761811062));
#31683=CARTESIAN_POINT('Ctrl Pts',(-0.00292013456997303,-0.0318607297917362,
-0.0133397931842086));
#31684=CARTESIAN_POINT('Ctrl Pts',(-0.00257712677055912,-0.0317033256230302,
-0.0103757882758759));
#31685=CARTESIAN_POINT('Ctrl Pts',(8.76993032760954E-5,-0.0315459214543242,
-0.00903349498082356));
#31686=CARTESIAN_POINT('Ctrl Pts',(0.00267358882914799,-0.0313885172856182,
-0.0105224072151816));
#31687=CARTESIAN_POINT('Ctrl Pts',(0.00285056591303206,-0.0312311131169122,
-0.0135007861344581));
#31688=CARTESIAN_POINT('Ctrl Pts',(0.000459618889897568,-0.0310737089482062,
-0.0152858630904674));
#31689=CARTESIAN_POINT('Ctrl Pts',(-0.00234598085158822,-0.0309163047795002,
-0.0142682165804294));
#31690=CARTESIAN_POINT('Ctrl Pts',(-0.00303688185573135,-0.0307589006107943,
-0.0113669520628329));
#31691=CARTESIAN_POINT('Ctrl Pts',(-0.000993857761956247,-0.0306014964420883,
-0.00919154437726977));
#31692=CARTESIAN_POINT('Ctrl Pts',(0.00194942720100573,-0.0304440691923362,
-0.00971077604905543));
#31693=CARTESIAN_POINT('Ctrl Pts',(0.00273326264745976,-0.0303391099988195,
-0.0115294799032454));
#31694=CARTESIAN_POINT('Ctrl Pts',(0.00265735689051292,-0.0302866188615381,
-0.0124059107630547));
#31695=CARTESIAN_POINT('Ctrl Pts',(-0.00200715618556375,-0.0407739344235557,
-0.0101695123425088));
#31696=CARTESIAN_POINT('Ctrl Pts',(-0.00134560506107313,-0.0407214555912242,
-0.00950767155873293));
#31697=CARTESIAN_POINT('Ctrl Pts',(0.000671733669518215,-0.0406165087026574,
-0.00890029303533848));
#31698=CARTESIAN_POINT('Ctrl Pts',(0.0031104577709741,-0.0404590937578553,
-0.0109407072489448));
#31699=CARTESIAN_POINT('Ctrl Pts',(0.00273886207562857,-0.0403016895891492,
-0.0140942010406314));
#31700=CARTESIAN_POINT('Ctrl Pts',(-9.64566422462461E-5,-0.0401442854204432,
-0.0155191106663781));
#31701=CARTESIAN_POINT('Ctrl Pts',(-0.00284683608352339,-0.0399868812517372,
-0.013932052606536));
#31702=CARTESIAN_POINT('Ctrl Pts',(-0.00303135672222567,-0.0398294770830313,
-0.0107626812392848));
#31703=CARTESIAN_POINT('Ctrl Pts',(-0.000485300036822523,-0.0396720729143253,
-0.00886653993958215));
#31704=CARTESIAN_POINT('Ctrl Pts',(0.00249825273968653,-0.0395146687456193,
-0.00995189977910353));
#31705=CARTESIAN_POINT('Ctrl Pts',(0.00323087291957833,-0.0393572645769133,
-0.0130409355465842));
#31706=CARTESIAN_POINT('Ctrl Pts',(0.00105271471644265,-0.0391998604082073,
-0.0153505723300579));
#31707=CARTESIAN_POINT('Ctrl Pts',(-0.00207392084708856,-0.0390424562395013,
-0.0147999546865617));
#31708=CARTESIAN_POINT('Ctrl Pts',(-0.00333204293495346,-0.0388850520707954,
-0.0118851567557591));
#31709=CARTESIAN_POINT('Ctrl Pts',(-0.00158817700263329,-0.0387276479020894,
-0.00923226194860017));
#31710=CARTESIAN_POINT('Ctrl Pts',(0.00158655878823555,-0.0385702437333834,
-0.00923138965431788));
#31711=CARTESIAN_POINT('Ctrl Pts',(0.00333188502928228,-0.0384128395646775,
-0.0118833262733665));
#31712=CARTESIAN_POINT('Ctrl Pts',(0.00207535727502861,-0.0382554353959714,
-0.0147988144430997));
#31713=CARTESIAN_POINT('Ctrl Pts',(-0.00105096021512142,-0.0380980312272654,
-0.0153511509433537));
#31714=CARTESIAN_POINT('Ctrl Pts',(-0.00323041681674889,-0.0379406270585595,
-0.0130427092173285));
#31715=CARTESIAN_POINT('Ctrl Pts',(-0.00249943589199024,-0.0377832228898535,
-0.00995327535086339));
#31716=CARTESIAN_POINT('Ctrl Pts',(0.000483406993018524,-0.0376258187211476,
-0.0088662687148974));
#31717=CARTESIAN_POINT('Ctrl Pts',(0.00303072524837413,-0.0374684145524415,
-0.0107610258178098));
#31718=CARTESIAN_POINT('Ctrl Pts',(0.00284751755284311,-0.0373110103837356,
-0.0139304689551257));
#31719=CARTESIAN_POINT('Ctrl Pts',(9.88444846859617E-5,-0.0371536062150296,
-0.0155190945443297));
#31720=CARTESIAN_POINT('Ctrl Pts',(-0.00273888232199736,-0.0369962020463236,
-0.014095633471993));
#31721=CARTESIAN_POINT('Ctrl Pts',(-0.00310901846993227,-0.0368387978776176,
-0.0109425502030451));
#31722=CARTESIAN_POINT('Ctrl Pts',(-0.000678090516909955,-0.0366813937089118,
-0.00890060893078614));
#31723=CARTESIAN_POINT('Ctrl Pts',(0.00236376175795272,-0.0365239895402056,
-0.00980949264405794));
#31724=CARTESIAN_POINT('Ctrl Pts',(0.00327598750851028,-0.0363665853714997,
-0.0128503443419849));
#31725=CARTESIAN_POINT('Ctrl Pts',(0.00123671873136661,-0.0362091812027937,
-0.0152835146450041));
#31726=CARTESIAN_POINT('Ctrl Pts',(-0.00191676936370603,-0.0360517770340877,
-0.0149168435356549));
#31727=CARTESIAN_POINT('Ctrl Pts',(-0.00334334785594242,-0.0358943728653817,
-0.0120806826315366));
#31728=CARTESIAN_POINT('Ctrl Pts',(-0.0017577436476271,-0.0357369686966757,
-0.00933026554259774));
#31729=CARTESIAN_POINT('Ctrl Pts',(0.00141149625623215,-0.0355795645279697,
-0.00914357515650723));
#31730=CARTESIAN_POINT('Ctrl Pts',(0.00330905137344668,-0.0354221603592638,
-0.0116888098108379));
#31731=CARTESIAN_POINT('Ctrl Pts',(0.00222532313885494,-0.0352647561905578,
-0.0146728453304159));
#31732=CARTESIAN_POINT('Ctrl Pts',(-0.000863305617849753,-0.0351073520218518,
-0.0154072207601635));
#31733=CARTESIAN_POINT('Ctrl Pts',(-0.00317414086950739,-0.0349499478531458,
-0.0132303019955118));
#31734=CARTESIAN_POINT('Ctrl Pts',(-0.00262524012362902,-0.0347925436844399,
-0.0101033797323109));
#31735=CARTESIAN_POINT('Ctrl Pts',(0.000288865568394113,-0.0346351395157338,
-0.00884364845760027));
#31736=CARTESIAN_POINT('Ctrl Pts',(0.00294271839225862,-0.0344777353470279,
-0.0105860605947262));
#31737=CARTESIAN_POINT('Ctrl Pts',(0.00294533484649854,-0.0343203311783219,
-0.013760793343527));
#31738=CARTESIAN_POINT('Ctrl Pts',(0.00029435764030422,-0.0341629270096159,
-0.0155075774518714));
#31739=CARTESIAN_POINT('Ctrl Pts',(-0.00262182050330342,-0.03400552284091,
-0.0142526512036113));
#31740=CARTESIAN_POINT('Ctrl Pts',(-0.0031758746048549,-0.0338481186722039,
-0.0111266379357506));
#31741=CARTESIAN_POINT('Ctrl Pts',(-0.000868630696093512,-0.033690714503498,
-0.00894591319249119));
#31742=CARTESIAN_POINT('Ctrl Pts',(0.00222120432239532,-0.033533310334792,
-0.00967519662958854));
#31743=CARTESIAN_POINT('Ctrl Pts',(0.00330984968583626,-0.033375906166086,
-0.0126574418200349));
#31744=CARTESIAN_POINT('Ctrl Pts',(0.00141649240610871,-0.0332185019973801,
-0.0152058006917256));
#31745=CARTESIAN_POINT('Ctrl Pts',(-0.00175305082785179,-0.0330610978286742,
-0.0150243345271474));
#31746=CARTESIAN_POINT('Ctrl Pts',(-0.00334318655513065,-0.032903693659968,
-0.0122765344930177));
#31747=CARTESIAN_POINT('Ctrl Pts',(-0.00192128451229188,-0.0327462894912621,
-0.00943802646138645));
#31748=CARTESIAN_POINT('Ctrl Pts',(0.00123159428251195,-0.0325888853225561,
-0.00906615709667131));
#31749=CARTESIAN_POINT('Ctrl Pts',(0.00327487211040667,-0.0324314811538501,
-0.0114959644595614));
#31750=CARTESIAN_POINT('Ctrl Pts',(0.00236765742921036,-0.0322740769851443,
-0.0145383123637269));
#31751=CARTESIAN_POINT('Ctrl Pts',(-0.000672687936266725,-0.0321166728164382,
-0.0154522151069147));
#31752=CARTESIAN_POINT('Ctrl Pts',(-0.00310698739398267,-0.0319592686477321,
-0.0134142710726901));
#31753=CARTESIAN_POINT('Ctrl Pts',(-0.00274203129922751,-0.0318018644790262,
-0.010260606176357));
#31754=CARTESIAN_POINT('Ctrl Pts',(9.33109838642071E-5,-0.0316444603103202,
-0.00883242256124597));
#31755=CARTESIAN_POINT('Ctrl Pts',(0.00284466574735029,-0.0314870561416142,
-0.0104166069308519));
#31756=CARTESIAN_POINT('Ctrl Pts',(0.00303296719561427,-0.0313296519729082,
-0.0135855655986646));
#31757=CARTESIAN_POINT('Ctrl Pts',(0.000489028865872123,-0.0311722478042024,
-0.0154848656023836));
#31758=CARTESIAN_POINT('Ctrl Pts',(-0.0024960948743115,-0.0310148436354963,
-0.0144021021877348));
#31759=CARTESIAN_POINT('Ctrl Pts',(-0.00323120507520287,-0.0308574394667903,
-0.0113151922982138));
#31760=CARTESIAN_POINT('Ctrl Pts',(-0.00105745247823908,-0.0307000352980843,
-0.00900058518204926));
#31761=CARTESIAN_POINT('Ctrl Pts',(0.00207416665015809,-0.0305426080483322,
-0.00955304131725042));
#31762=CARTESIAN_POINT('Ctrl Pts',(0.00290815795868601,-0.0304376488548157,
-0.0114881199285106));
#31763=CARTESIAN_POINT('Ctrl Pts',(0.0028273951635772,-0.0303851577175343,
-0.0124206316220213));
#31764=CARTESIAN_POINT('Ctrl Pts',(-0.00212786565552399,-0.0408724732795518,
-0.0100488519008064));
#31765=CARTESIAN_POINT('Ctrl Pts',(-0.00142652914404491,-0.0408199944472204,
-0.00934720831006298));
#31766=CARTESIAN_POINT('Ctrl Pts',(0.000712131430183422,-0.0407150475586535,
-0.00870330231553719));
#31767=CARTESIAN_POINT('Ctrl Pts',(0.00329751930189471,-0.0405576326138514,
-0.0108664261219471));
#31768=CARTESIAN_POINT('Ctrl Pts',(0.0029035760086157,-0.0404002284451454,
-0.0142095696114775));
#31769=CARTESIAN_POINT('Ctrl Pts',(-0.000102257501314122,-0.0402428242764393,
-0.0157201726610358));
#31770=CARTESIAN_POINT('Ctrl Pts',(-0.00301804352476665,-0.0400854201077334,
-0.0140376696435079));
#31771=CARTESIAN_POINT('Ctrl Pts',(-0.00321366115166276,-0.0399280159390274,
-0.010677693708162));
#31772=CARTESIAN_POINT('Ctrl Pts',(-0.000514485762695765,-0.0397706117703215,
-0.00866751932378795));
#31773=CARTESIAN_POINT('Ctrl Pts',(0.00264849653546252,-0.0396132076016156,
-0.00981815221574397));
#31774=CARTESIAN_POINT('Ctrl Pts',(0.00342517616335999,-0.0394558034329095,
-0.0130929612044931));
#31775=CARTESIAN_POINT('Ctrl Pts',(0.00111602450586276,-0.0392983992642035,
-0.0155414985049964));
#31776=CARTESIAN_POINT('Ctrl Pts',(-0.00219864551375484,-0.0391409950954976,
-0.0149577669641485));
#31777=CARTESIAN_POINT('Ctrl Pts',(-0.00353243049794239,-0.0389835909267915,
-0.0118676743971841));
#31778=CARTESIAN_POINT('Ctrl Pts',(-0.00168368925303498,-0.0388261867580856,
-0.00905523568988633));
#31779=CARTESIAN_POINT('Ctrl Pts',(0.00168197371995147,-0.0386687825893795,
-0.00905431093621841));
#31780=CARTESIAN_POINT('Ctrl Pts',(0.00353226309589514,-0.0385113784206737,
-0.011865733830404));
#31781=CARTESIAN_POINT('Ctrl Pts',(0.00220016832782498,-0.0383539742519676,
-0.0149565581469579));
#31782=CARTESIAN_POINT('Ctrl Pts',(-0.00111416448962141,-0.0381965700832616,
-0.0155421119158356));
#31783=CARTESIAN_POINT('Ctrl Pts',(-0.00342469263071152,-0.0380391659145558,
-0.013094841542998));
#31784=CARTESIAN_POINT('Ctrl Pts',(-0.00264975084201354,-0.0378817617458498,
-0.00981961051377058));
#31785=CARTESIAN_POINT('Ctrl Pts',(0.000512478872088983,-0.0377243575771436,
-0.00866723178777268));
#31786=CARTESIAN_POINT('Ctrl Pts',(0.00321299170125789,-0.0375669534084378,
-0.0106759387303842));
#31787=CARTESIAN_POINT('Ctrl Pts',(0.0030187659773448,-0.0374095492397318,
-0.0140359907520142));
#31788=CARTESIAN_POINT('Ctrl Pts',(0.000104788947523881,-0.0372521450710258,
-0.0157201555694146));
#31789=CARTESIAN_POINT('Ctrl Pts',(-0.00290359747259187,-0.0370947409023197,
-0.0142110881886168));
#31790=CARTESIAN_POINT('Ctrl Pts',(-0.00329599344193575,-0.0369373367336139,
-0.0108683799104779));
#31791=CARTESIAN_POINT('Ctrl Pts',(-0.000718870575517203,-0.0367799325649078,
-0.00870363720879496));
#31792=CARTESIAN_POINT('Ctrl Pts',(0.00250591732659617,-0.0366225283962018,
-0.00966718077966711));
#31793=CARTESIAN_POINT('Ctrl Pts',(0.00347300392337274,-0.0364651242274959,
-0.012890907930598));
#31794=CARTESIAN_POINT('Ctrl Pts',(0.00131109443945905,-0.0363077200587899,
-0.0154704080009334));
#31795=CARTESIAN_POINT('Ctrl Pts',(-0.00203204301086584,-0.0361503158900839,
-0.0150816854560369));
#31796=CARTESIAN_POINT('Ctrl Pts',(-0.00354441529179335,-0.0359929117213779,
-0.0120749591111619));
#31797=CARTESIAN_POINT('Ctrl Pts',(-0.00186345355976913,-0.035835507552672,
-0.00915913317593414));
#31798=CARTESIAN_POINT('Ctrl Pts',(0.00149638300603574,-0.0356781033839659,
-0.00896121531401801));
#31799=CARTESIAN_POINT('Ctrl Pts',(0.00350805623427067,-0.0355206992152599,
-0.0116595192353337));
#31800=CARTESIAN_POINT('Ctrl Pts',(0.00235915307123073,-0.0353632950465541,
-0.0148230133085119));
#31801=CARTESIAN_POINT('Ctrl Pts',(-0.000915224429297398,-0.0352058908778481,
-0.0156015537462018));
#31802=CARTESIAN_POINT('Ctrl Pts',(-0.00336503227332211,-0.035048486709142,
-0.0132937160664613));
#31803=CARTESIAN_POINT('Ctrl Pts',(-0.00278312088354253,-0.0348910825404361,
-0.00997874210518484));
#31804=CARTESIAN_POINT('Ctrl Pts',(0.000306237813713841,-0.0347336783717301,
-0.00864325115837878));
#31805=CARTESIAN_POINT('Ctrl Pts',(0.0031196921524109,-0.034576274203024,
-0.0104904511775031));
#31806=CARTESIAN_POINT('Ctrl Pts',(0.0031224659590316,-0.0344188700343182,
-0.0138561109254727));
#31807=CARTESIAN_POINT('Ctrl Pts',(0.000312060176357651,-0.0342614658656122,
-0.0157079458441975));
#31808=CARTESIAN_POINT('Ctrl Pts',(-0.00277949560878902,-0.0341040616969062,
-0.0143775488959709));
#31809=CARTESIAN_POINT('Ctrl Pts',(-0.00336687027473339,-0.0339466575282002,
-0.0110635385966054));
#31810=CARTESIAN_POINT('Ctrl Pts',(-0.000920869755351007,-0.0337892533594942,
-0.00875166604841612));
#31811=CARTESIAN_POINT('Ctrl Pts',(0.00235478655100232,-0.0336318491907882,
-0.00952480826330864));
#31812=CARTESIAN_POINT('Ctrl Pts',(0.0035089025568082,-0.0334744450220822,
-0.0126864043377667));
#31813=CARTESIAN_POINT('Ctrl Pts',(0.00150167962211813,-0.0333170408533761,
-0.015388020365469));
#31814=CARTESIAN_POINT('Ctrl Pts',(-0.00185847851592382,-0.0331596366846703,
-0.0151956409073963));
#31815=CARTESIAN_POINT('Ctrl Pts',(-0.00354424429042339,-0.0330022325159643,
-0.0122825894154766));
#31816=CARTESIAN_POINT('Ctrl Pts',(-0.00203682969845604,-0.0328448283472583,
-0.00927337478789609));
#31817=CARTESIAN_POINT('Ctrl Pts',(0.00130566180855576,-0.0326874241785523,
-0.00887914136689471));
#31818=CARTESIAN_POINT('Ctrl Pts',(0.00347182144572907,-0.0325300200098464,
-0.0114550762513946));
#31819=CARTESIAN_POINT('Ctrl Pts',(0.0025100472817705,-0.0323726158411403,
-0.0146803895897339));
#31820=CARTESIAN_POINT('Ctrl Pts',(-0.000713143086104787,-0.0322152116724343,
-0.0156492540327232));
#31821=CARTESIAN_POINT('Ctrl Pts',(-0.00329384021799231,-0.0320578075037284,
-0.0134887489611716));
#31822=CARTESIAN_POINT('Ctrl Pts',(-0.00290693582789601,-0.0319004033350224,
-0.0101454240768384));
#31823=CARTESIAN_POINT('Ctrl Pts',(9.89226644522099E-5,-0.0317429991663165,
-0.0086313501416684));
#31824=CARTESIAN_POINT('Ctrl Pts',(0.00301574266555261,-0.0315855949976104,
-0.0103108066465221));
#31825=CARTESIAN_POINT('Ctrl Pts',(0.00321536847819648,-0.0314281908289045,
-0.0136703450628712));
#31826=CARTESIAN_POINT('Ctrl Pts',(0.000518438841846787,-0.0312707866601984,
-0.0156838681142999));
#31827=CARTESIAN_POINT('Ctrl Pts',(-0.00264620889703467,-0.0311133824914924,
-0.0145359877950401));
#31828=CARTESIAN_POINT('Ctrl Pts',(-0.0034255282946743,-0.0309559783227865,
-0.0112634325335946));
#31829=CARTESIAN_POINT('Ctrl Pts',(-0.00112104719452203,-0.0307985741540806,
-0.00880962598682875));
#31830=CARTESIAN_POINT('Ctrl Pts',(0.00219890609931043,-0.0306411469043285,
-0.00939530658544539));
#31831=CARTESIAN_POINT('Ctrl Pts',(0.00308305326991214,-0.0305361877108118,
-0.0114467599537756));
#31832=CARTESIAN_POINT('Ctrl Pts',(0.00299743343664159,-0.0304836965735304,
-0.0124353524809878));
#31833=CARTESIAN_POINT('',(0.00298893256437761,-0.0304787743898623,-0.0124333064388995));
#31834=CARTESIAN_POINT('Ctrl Pts',(0.00298893256437029,-0.0304787743898723,
-0.012433306438892));
#31835=CARTESIAN_POINT('Ctrl Pts',(0.00298837300754948,-0.030478774389874,
-0.0123352674302941));
#31836=CARTESIAN_POINT('Ctrl Pts',(0.00298261840524365,-0.0304787743898738,
-0.0122375191512274));
#31837=CARTESIAN_POINT('Ctrl Pts',(0.00297189591856322,-0.0304787743898736,
-0.0121403782556776));
#31838=CARTESIAN_POINT('Ctrl Pts',(0.0029506659422511,-0.0304787743898733,
-0.0119480442409175));
#31839=CARTESIAN_POINT('Ctrl Pts',(0.0029099981664046,-0.0304787743898729,
-0.0117580651785402));
#31840=CARTESIAN_POINT('Ctrl Pts',(0.00285112369699802,-0.0304787743898726,
-0.0115730963590973));
#31841=CARTESIAN_POINT('Ctrl Pts',(0.00284398971481766,-0.0304787743898726,
-0.0115506831760126));
#31842=CARTESIAN_POINT('Ctrl Pts',(0.00283658767728467,-0.0304787743898725,
-0.0115283440580714));
#31843=CARTESIAN_POINT('Ctrl Pts',(0.00282891920321681,-0.0304787743898725,
-0.0115060841919811));
#31844=CARTESIAN_POINT('Ctrl Pts',(0.00282186171808973,-0.0304787743898724,
-0.011485597890212));
#31845=CARTESIAN_POINT('Ctrl Pts',(0.00281457673346536,-0.0304787743898724,
-0.011465174083367));
#31846=CARTESIAN_POINT('Ctrl Pts',(0.00280707621326217,-0.0304787743898724,
-0.0114448451703835));
#31847=CARTESIAN_POINT('Ctrl Pts',(0.00270641710168845,-0.0304787743898717,
-0.0111720253839232));
#31848=CARTESIAN_POINT('Ctrl Pts',(0.00256690712160261,-0.0304787743898713,
-0.0109151889309775));
#31849=CARTESIAN_POINT('Ctrl Pts',(0.0023924314614952,-0.0304787743898706,
-0.0106839334442482));
#31850=CARTESIAN_POINT('Ctrl Pts',(0.00238354432219219,-0.0304787743898706,
-0.0106721541523751));
#31851=CARTESIAN_POINT('Ctrl Pts',(0.00237456589083953,-0.0304787743898706,
-0.0106604419288824));
#31852=CARTESIAN_POINT('Ctrl Pts',(0.00236549651133127,-0.0304787743898705,
-0.0106487982886585));
#31853=CARTESIAN_POINT('Ctrl Pts',(0.00235654131236866,-0.0304787743898705,
-0.0106373012380874));
#31854=CARTESIAN_POINT('Ctrl Pts',(0.00234750304637241,-0.0304787743898705,
-0.0106258782674));
#31855=CARTESIAN_POINT('Ctrl Pts',(0.00233838354414271,-0.0304787743898705,
-0.0106145320289449));
#31856=CARTESIAN_POINT('Ctrl Pts',(0.0021652597390184,-0.0304787743898699,
-0.0103991360648103));
#31857=CARTESIAN_POINT('Ctrl Pts',(0.00196289502114972,-0.0304787743898692,
-0.0102109270530416));
#31858=CARTESIAN_POINT('Ctrl Pts',(0.00173430499794,-0.0304787743898686,
-0.0100590786561608));
#31859=CARTESIAN_POINT('Ctrl Pts',(0.00172022400467282,-0.0304787743898685,
-0.0100497248959919));
#31860=CARTESIAN_POINT('Ctrl Pts',(0.00170604292827687,-0.0304787743898685,
-0.0100405103160519));
#31861=CARTESIAN_POINT('Ctrl Pts',(0.00169176227320023,-0.0304787743898685,
-0.0100314375701239));
#31862=CARTESIAN_POINT('Ctrl Pts',(0.00166701763122726,-0.0304787743898684,
-0.0100157168732445));
#31863=CARTESIAN_POINT('Ctrl Pts',(0.00164197401157139,-0.0304787743898683,
-0.0100004219931363));
#31864=CARTESIAN_POINT('Ctrl Pts',(0.00161664364654793,-0.0304787743898682,
-0.00998555579774938));
#31865=CARTESIAN_POINT('Ctrl Pts',(0.00160269290467747,-0.0304787743898682,
-0.00997736821520777));
#31866=CARTESIAN_POINT('Ctrl Pts',(0.00158865518509774,-0.0304787743898682,
-0.00996931067307717));
#31867=CARTESIAN_POINT('Ctrl Pts',(0.00157453253482917,-0.0304787743898681,
-0.00996138371355764));
#31868=CARTESIAN_POINT('Ctrl Pts',(0.0015624910192888,-0.0304787743898681,
-0.00995462488257144));
#31869=CARTESIAN_POINT('Ctrl Pts',(0.00155038831353741,-0.0304787743898681,
-0.00994796137764227));
#31870=CARTESIAN_POINT('Ctrl Pts',(0.00153823739716388,-0.030478774389868,
-0.00994139960184977));
#31871=CARTESIAN_POINT('Ctrl Pts',(0.00125129790158513,-0.0304787743898672,
-0.00978644563968585));
#31872=CARTESIAN_POINT('Ctrl Pts',(0.000935868208510309,-0.0304787743898666,
-0.00968658593292551));
#31873=CARTESIAN_POINT('Ctrl Pts',(0.000609871031302533,-0.030478774389866,
-0.00964440028463229));
#31874=CARTESIAN_POINT('Ctrl Pts',(0.000593206497894966,-0.030478774389866,
-0.00964224381152622));
#31875=CARTESIAN_POINT('Ctrl Pts',(0.000576512109012424,-0.030478774389866,
-0.00964023965127942));
#31876=CARTESIAN_POINT('Ctrl Pts',(0.000559813525617774,-0.030478774389866,
-0.0096383909861675));
#31877=CARTESIAN_POINT('Ctrl Pts',(0.000296852526983212,-0.0304787743898655,
-0.00960927912604843));
#31878=CARTESIAN_POINT('Ctrl Pts',(3.15475597085231E-5,-0.0304787743898651,
-0.00961823760304827));
#31879=CARTESIAN_POINT('Ctrl Pts',(-0.000226290956562403,-0.0304787743898647,
-0.00966738870262534));
#31880=CARTESIAN_POINT('Ctrl Pts',(-0.000282359974600194,-0.0304787743898646,
-0.00967807699671196));
#31881=CARTESIAN_POINT('Ctrl Pts',(-0.00033806990970888,-0.0304787743898646,
-0.00969068022176533));
#31882=CARTESIAN_POINT('Ctrl Pts',(-0.000393306057963943,-0.0304787743898718,
-0.00970524382248907));
#31883=CARTESIAN_POINT('',(-0.00299999910843776,-0.0309924495244571,-0.0121735404154808));
#31884=CARTESIAN_POINT('Ctrl Pts',(-0.00299999910843776,-0.0309924495244571,
-0.0121735404154808));
#31885=CARTESIAN_POINT('Ctrl Pts',(-0.00299957015955796,-0.0309629253341015,
-0.0116171556391684));
#31886=CARTESIAN_POINT('Ctrl Pts',(-0.00284005225347564,-0.0309334011437459,
-0.0110606943513532));
#31887=CARTESIAN_POINT('Ctrl Pts',(-0.00254572450208166,-0.0309038769533902,
-0.0105886271654584));
#31888=CARTESIAN_POINT('Ctrl Pts',(-0.00241331504383175,-0.0308905948825296,
-0.0103762579272678));
#31889=CARTESIAN_POINT('Ctrl Pts',(-0.002254325614464,-0.030877312811669,
-0.0101807858430437));
#31890=CARTESIAN_POINT('Ctrl Pts',(-0.00207401368765223,-0.0308640307408084,
-0.0100082584850716));
#31891=CARTESIAN_POINT('Ctrl Pts',(-0.00168100707884367,-0.0308350812324804,
-0.00963221906781163));
#31892=CARTESIAN_POINT('Ctrl Pts',(-0.00118098993580744,-0.0308061317241523,
-0.00936454502561941));
#31893=CARTESIAN_POINT('Ctrl Pts',(-0.000647803879971564,-0.0307771822158243,
-0.00924662981725879));
#31894=CARTESIAN_POINT('Ctrl Pts',(-0.000392593071710581,-0.0307633254629361,
-0.00919018941469651));
#31895=CARTESIAN_POINT('Ctrl Pts',(-0.000130218005705817,-0.0307494687100479,
-0.00916738448966662));
#31896=CARTESIAN_POINT('Ctrl Pts',(0.000130000822421629,-0.0307356119571597,
-0.00917867131240808));
#31897=CARTESIAN_POINT('Ctrl Pts',(0.000673649626204348,-0.0307066624488317,
-0.00920225172634686));
#31898=CARTESIAN_POINT('Ctrl Pts',(0.00121291501584666,-0.0306777129405036,
-0.00937818640396837));
#31899=CARTESIAN_POINT('Ctrl Pts',(0.00166686823158946,-0.0306487634321756,
-0.00968154971671783));
#31900=CARTESIAN_POINT('Ctrl Pts',(0.00188415404736492,-0.0306349066792874,
-0.00982675530751699));
#31901=CARTESIAN_POINT('Ctrl Pts',(0.002082085130544,-0.0306210499263992,
-0.0100003750833504));
#31902=CARTESIAN_POINT('Ctrl Pts',(0.00225390745583324,-0.030607193173511,
-0.0101959792550754));
#31903=CARTESIAN_POINT('Ctrl Pts',(0.00262000441087861,-0.0305776689831554,
-0.0106127475157898));
#31904=CARTESIAN_POINT('Ctrl Pts',(0.00286825892999133,-0.0305481447927997,
-0.0111350521502138));
#31905=CARTESIAN_POINT('Ctrl Pts',(0.00295948265647319,-0.0305186206024441,
-0.0116844650428705));
#31906=CARTESIAN_POINT('Ctrl Pts',(0.00300052154643768,-0.0305053385315835,
-0.0119316298553198));
#31907=CARTESIAN_POINT('Ctrl Pts',(0.00301041285349739,-0.030492056460723,
-0.0121839285032162));
#31908=CARTESIAN_POINT('Ctrl Pts',(0.00298893256436973,-0.0304787743898624,
-0.0124333064388988));
#31909=CARTESIAN_POINT('',(-0.00299999981352153,-0.0319945472736604,-0.0121769110534293));
#31910=CARTESIAN_POINT('Ctrl Pts',(-0.00299999981352153,-0.0319945472736604,
-0.0121769110534293));
#31911=CARTESIAN_POINT('Ctrl Pts',(-0.00300001642542353,-0.0319922152497922,
-0.0121297969829771));
#31912=CARTESIAN_POINT('Ctrl Pts',(-0.00299892317095584,-0.0319898566084726,
-0.0120826905849812));
#31913=CARTESIAN_POINT('Ctrl Pts',(-0.00299515512313883,-0.0319857664535245,
-0.0120021629381566));
#31914=CARTESIAN_POINT('Ctrl Pts',(-0.00299302858819974,-0.031984050903241,
-0.0119687245641428));
#31915=CARTESIAN_POINT('Ctrl Pts',(-0.00298877904546892,-0.0319813101095438,
-0.0119158915587133));
#31916=CARTESIAN_POINT('Ctrl Pts',(-0.00298702610746423,-0.0319802960930753,
-0.011896469513365));
#31917=CARTESIAN_POINT('Ctrl Pts',(-0.00298320600118927,-0.0319782901614954,
-0.0118583040786077));
#31918=CARTESIAN_POINT('Ctrl Pts',(-0.00298115121742591,-0.0319772986694851,
-0.0118395603452952));
#31919=CARTESIAN_POINT('Ctrl Pts',(-0.0029764027823879,-0.0319751770471325,
-0.0117997164611982));
#31920=CARTESIAN_POINT('Ctrl Pts',(-0.00297366114976589,-0.0319740454863181,
-0.0117786231650717));
#31921=CARTESIAN_POINT('Ctrl Pts',(-0.00296601432529667,-0.0319711098676958,
-0.0117243156949625));
#31922=CARTESIAN_POINT('Ctrl Pts',(-0.00296077554499708,-0.0319692956207431,
-0.0116911521179402));
#31923=CARTESIAN_POINT('Ctrl Pts',(-0.00293534004140591,-0.0319612568581492,
-0.0115459880653948));
#31924=CARTESIAN_POINT('Ctrl Pts',(-0.00290933809512656,-0.0319548560777858,
-0.0114351112327025));
#31925=CARTESIAN_POINT('Ctrl Pts',(-0.00283030627595261,-0.0319388149721708,
-0.0111675597328889));
#31926=CARTESIAN_POINT('Ctrl Pts',(-0.00277050385213032,-0.0319290335683348,
-0.0110132731158511));
#31927=CARTESIAN_POINT('Ctrl Pts',(-0.00266259098944409,-0.0319145847252816,
-0.0107911910668462));
#31928=CARTESIAN_POINT('Ctrl Pts',(-0.00262387856782943,-0.0319098400276056,
-0.0107191642974873));
#31929=CARTESIAN_POINT('Ctrl Pts',(-0.00256546348083541,-0.0319033297703317,
-0.0106203831154059));
#31930=CARTESIAN_POINT('Ctrl Pts',(-0.00254818702925803,-0.0319014746892419,
-0.0105922392738789));
#31931=CARTESIAN_POINT('Ctrl Pts',(-0.00251689521595761,-0.0318982430011514,
-0.0105431024978857));
#31932=CARTESIAN_POINT('Ctrl Pts',(-0.00250307315484794,-0.0318968568820697,
-0.0105219906775617));
#31933=CARTESIAN_POINT('Ctrl Pts',(-0.00248160693976785,-0.031894769038704,
-0.0104900888591791));
#31934=CARTESIAN_POINT('Ctrl Pts',(-0.00247415540277629,-0.0318940557475992,
-0.0104791712998327));
#31935=CARTESIAN_POINT('Ctrl Pts',(-0.00246030964179461,-0.0318927517986779,
-0.0104591704848017));
#31936=CARTESIAN_POINT('Ctrl Pts',(-0.0024539369867617,-0.0318921598417614,
-0.0104500732760709));
#31937=CARTESIAN_POINT('Ctrl Pts',(-0.00243920990448888,-0.0318908102733566,
-0.0104292963211079));
#31938=CARTESIAN_POINT('Ctrl Pts',(-0.00243082198851743,-0.0318900548883533,
-0.0104176409364644));
#31939=CARTESIAN_POINT('Ctrl Pts',(-0.00240349380418427,-0.0318876346538313,
-0.0103802366141087));
#31940=CARTESIAN_POINT('Ctrl Pts',(-0.00238422506486495,-0.0318859902850841,
-0.0103547292669735));
#31941=CARTESIAN_POINT('Ctrl Pts',(-0.00224440813997212,-0.031874453183327,
-0.0101756679812831));
#31942=CARTESIAN_POINT('Ctrl Pts',(-0.00210952066103542,-0.0318653282790874,
-0.0100338805378428));
#31943=CARTESIAN_POINT('Ctrl Pts',(-0.00182762110192053,-0.0318476390290283,
-0.00979021793073736));
#31944=CARTESIAN_POINT('Ctrl Pts',(-0.00168343109687408,-0.0318391306117249,
-0.00968637407129882));
#31945=CARTESIAN_POINT('Ctrl Pts',(-0.00149723877718005,-0.0318281472838993,
-0.00957588973391417));
#31946=CARTESIAN_POINT('Ctrl Pts',(-0.00146316413035672,-0.0318261387297483,
-0.009556562355812));
#31947=CARTESIAN_POINT('Ctrl Pts',(-0.00140897504517393,-0.031822942057075,
-0.00952721332681065));
#31948=CARTESIAN_POINT('Ctrl Pts',(-0.00138910921764175,-0.0318217696587595,
-0.00951674067893614));
#31949=CARTESIAN_POINT('Ctrl Pts',(-0.00135157780893566,-0.0318195529749003,
-0.00949749064022305));
#31950=CARTESIAN_POINT('Ctrl Pts',(-0.00133393953136627,-0.0318185105134473,
-0.00948866249676546));
#31951=CARTESIAN_POINT('Ctrl Pts',(-0.00129394467084666,-0.031816144615133,
-0.00946913545393362));
#31952=CARTESIAN_POINT('Ctrl Pts',(-0.00127154016664873,-0.0318148177994003,
-0.00945853847382943));
#31953=CARTESIAN_POINT('Ctrl Pts',(-0.00121314042737946,-0.0318113546597345,
-0.00943179671227953));
#31954=CARTESIAN_POINT('Ctrl Pts',(-0.00117695424730294,-0.0318092042269369,
-0.00941608252075385));
#31955=CARTESIAN_POINT('Ctrl Pts',(-0.0009009913001464,-0.0317927662081466,
-0.00930265768544881));
#31956=CARTESIAN_POINT('Ctrl Pts',(-0.000649805607183565,-0.0317774500921903,
-0.00923565791379496));
#31957=CARTESIAN_POINT('Ctrl Pts',(-0.000310970476071452,-0.0317574426099795,
-0.00919086122100353));
#31958=CARTESIAN_POINT('Ctrl Pts',(-0.000228318885291927,-0.0317526247646428,
-0.00918340410543012));
#31959=CARTESIAN_POINT('Ctrl Pts',(-9.66138540080629E-5,-0.0317451418381697,
-0.00917701060556102));
#31960=CARTESIAN_POINT('Ctrl Pts',(-4.77133307582583E-5,-0.031742406153735,
-0.00917583401678422));
#31961=CARTESIAN_POINT('Ctrl Pts',(1.8263743597101E-5,-0.031738791577688,
-0.009175860332671));
#31962=CARTESIAN_POINT('Ctrl Pts',(3.53309251822941E-5,-0.0317378634542682,
-0.00917601278406565));
#31963=CARTESIAN_POINT('Ctrl Pts',(6.38725522234893E-5,-0.0317363239422441,
-0.00917651135165962));
#31964=CARTESIAN_POINT('Ctrl Pts',(7.53478726622746E-5,-0.0317357083833803,
-0.00917677768611424));
#31965=CARTESIAN_POINT('Ctrl Pts',(9.88576639912124E-5,-0.0317344546351368,
-0.00917745835791557));
#31966=CARTESIAN_POINT('Ctrl Pts',(0.00011089162661713,-0.0317338167977515,
-0.00917787929685429));
#31967=CARTESIAN_POINT('Ctrl Pts',(0.000142654880958706,-0.0317321428488871,
-0.00917918186822764));
#31968=CARTESIAN_POINT('Ctrl Pts',(0.000162378861661807,-0.0317311131642323,
-0.00918018589020346));
#31969=CARTESIAN_POINT('Ctrl Pts',(0.000250653753600739,-0.0317265430617562,
-0.00918555383768674));
#31970=CARTESIAN_POINT('Ctrl Pts',(0.000319056744679814,-0.0317231049958787,
-0.00919207679906972));
#31971=CARTESIAN_POINT('Ctrl Pts',(0.000550364637773504,-0.0317116562800663,
-0.00922218113501574));
#31972=CARTESIAN_POINT('Ctrl Pts',(0.000711533127640449,-0.0317039669075692,
-0.00925681122974356));
#31973=CARTESIAN_POINT('Ctrl Pts',(0.000975195187799041,-0.0316908606773177,
-0.0093366117995718));
#31974=CARTESIAN_POINT('Ctrl Pts',(0.00107946837399842,-0.0316855340704567,
-0.00937459572977345));
#31975=CARTESIAN_POINT('Ctrl Pts',(0.00122609970636494,-0.0316776467731615,
-0.0094374148967181));
#31976=CARTESIAN_POINT('Ctrl Pts',(0.00127033040785503,-0.0316752139754418,
-0.00945765063389414));
#31977=CARTESIAN_POINT('Ctrl Pts',(0.00134939760217658,-0.0316707531341619,
-0.00949617563153442));
#31978=CARTESIAN_POINT('Ctrl Pts',(0.00138440366752245,-0.0316687372427017,
-0.00951409211620556));
#31979=CARTESIAN_POINT('Ctrl Pts',(0.00143884485791577,-0.031665532423469,
-0.0095433202040005));
#31980=CARTESIAN_POINT('Ctrl Pts',(0.00145852280510933,-0.0316643594058127,
-0.0095541713556147));
#31981=CARTESIAN_POINT('Ctrl Pts',(0.00149521458475665,-0.0316621437523772,
-0.00957494552087175));
#31982=CARTESIAN_POINT('Ctrl Pts',(0.00151225627130588,-0.0316611029706844,
-0.00958481704496393));
#31983=CARTESIAN_POINT('Ctrl Pts',(0.00155043989818843,-0.031658743935678,
-0.00960744022355745));
#31984=CARTESIAN_POINT('Ctrl Pts',(0.00157152392498763,-0.0316574223525361,
-0.00962028641323898));
#31985=CARTESIAN_POINT('Ctrl Pts',(0.00162564777565868,-0.031653979468501,
-0.00965418636345596));
#31986=CARTESIAN_POINT('Ctrl Pts',(0.00165843731727481,-0.0316518442906599,
-0.00967562925045361));
#31987=CARTESIAN_POINT('Ctrl Pts',(0.00190574893413454,-0.03163535362645,
-0.00984436573858123));
#31988=CARTESIAN_POINT('Ctrl Pts',(0.00210068014239803,-0.031619955545076,
-0.0100183516693828));
#31989=CARTESIAN_POINT('Ctrl Pts',(0.00234356759871333,-0.0315982011335395,
-0.0102996531862232));
#31990=CARTESIAN_POINT('Ctrl Pts',(0.00241169036278049,-0.0315917429710965,
-0.010388064348014));
#31991=CARTESIAN_POINT('Ctrl Pts',(0.00249048120709294,-0.0315839850065132,
-0.0105030474825988));
#31992=CARTESIAN_POINT('Ctrl Pts',(0.00250590632681066,-0.0315824508338868,
-0.0105262443964411));
#31993=CARTESIAN_POINT('Ctrl Pts',(0.00252845151920646,-0.0315801890589914,
-0.010561194949764));
#31994=CARTESIAN_POINT('Ctrl Pts',(0.00253581719650946,-0.031579446888502,
-0.0105727875393121));
#31995=CARTESIAN_POINT('Ctrl Pts',(0.00254897232253479,-0.0315781160616994,
-0.0105938095097945));
#31996=CARTESIAN_POINT('Ctrl Pts',(0.00255478946401977,-0.0315775256986796,
-0.0106032207120483));
#31997=CARTESIAN_POINT('Ctrl Pts',(0.00256782252689628,-0.0315761986505758,
-0.0106245692958359));
#31998=CARTESIAN_POINT('Ctrl Pts',(0.00257500739135149,-0.0315754639056578,
-0.0106365250243147));
#31999=CARTESIAN_POINT('Ctrl Pts',(0.00259684262389686,-0.0315732197606075,
-0.0106734399130476));
#32000=CARTESIAN_POINT('Ctrl Pts',(0.00261121580047175,-0.0315717266550666,
-0.0106985619415731));
#32001=CARTESIAN_POINT('Ctrl Pts',(0.00270767657634611,-0.0315615671502975,
-0.0108729678100802));
#32002=CARTESIAN_POINT('Ctrl Pts',(0.0027772896014038,-0.0315535054335339,
-0.0110288148879857));
#32003=CARTESIAN_POINT('Ctrl Pts',(0.00285808667288348,-0.0315418533076306,
-0.0112609613874801));
#32004=CARTESIAN_POINT('Ctrl Pts',(0.00288017974912521,-0.0315382818902255,
-0.0113330893767142));
#32005=CARTESIAN_POINT('Ctrl Pts',(0.0029235356635223,-0.0315301929040391,
-0.0114963767211787));
#32006=CARTESIAN_POINT('Ctrl Pts',(0.00294329748342001,-0.0315256579285381,
-0.01158785019842));
#32007=CARTESIAN_POINT('Ctrl Pts',(0.00296928999080422,-0.031517839414608,
-0.01174297656792));
#32008=CARTESIAN_POINT('Ctrl Pts',(0.0029778186060514,-0.0315146195824636,
-0.0118061764811226));
#32009=CARTESIAN_POINT('Ctrl Pts',(0.00298708176151363,-0.0315099498587432,
-0.0118964418428674));
#32010=CARTESIAN_POINT('Ctrl Pts',(0.00298947417383292,-0.0315085504569989,
-0.0119233214907006));
#32011=CARTESIAN_POINT('Ctrl Pts',(0.00299300791378566,-0.0315060943842574,
-0.0119701746278096));
#32012=CARTESIAN_POINT('Ctrl Pts',(0.00299431269243673,-0.0315050427904204,
-0.0119901342597551));
#32013=CARTESIAN_POINT('Ctrl Pts',(0.00299659741348077,-0.0315028558999542,
-0.0120314239748961));
#32014=CARTESIAN_POINT('Ctrl Pts',(0.00299754941927381,-0.0315017198077756,
-0.0120527544163292));
#32015=CARTESIAN_POINT('Ctrl Pts',(0.00299942465819,-0.031498759956318,
-0.0121080065268212));
#32016=CARTESIAN_POINT('Ctrl Pts',(0.00300000016225006,-0.0314969256987105,
-0.0121419363032316));
#32017=CARTESIAN_POINT('Ctrl Pts',(0.00299999937983027,-0.0314879988457174,
-0.0123055290472804));
#32018=CARTESIAN_POINT('Ctrl Pts',(0.00299159289392699,-0.0314806719372835,
-0.0124350397607784));
#32019=CARTESIAN_POINT('Ctrl Pts',(0.00295954566551207,-0.0314663367216377,
-0.0126809167156226));
#32020=CARTESIAN_POINT('Ctrl Pts',(0.00293732611516207,-0.0314593704234008,
-0.0127972332192756));
#32021=CARTESIAN_POINT('Ctrl Pts',(0.0028744531151376,-0.0314443185765894,
-0.0130456498495619));
#32022=CARTESIAN_POINT('Ctrl Pts',(0.00283142401875427,-0.0314362555019756,
-0.0131768879571909));
#32023=CARTESIAN_POINT('Ctrl Pts',(0.00276838468732164,-0.0314269139106782,
-0.0133321061977503));
#32024=CARTESIAN_POINT('Ctrl Pts',(0.0027568518141252,-0.031425282738302,
-0.0133593408339047));
#32025=CARTESIAN_POINT('Ctrl Pts',(0.00273923638612753,-0.0314229068615499,
-0.0133992838132518));
#32026=CARTESIAN_POINT('Ctrl Pts',(0.00273346434505124,-0.0314221455117122,
-0.0134121262833714));
#32027=CARTESIAN_POINT('Ctrl Pts',(0.00272297990476607,-0.0314207934097788,
-0.0134350211369915));
#32028=CARTESIAN_POINT('Ctrl Pts',(0.00271830189775692,-0.0314202007195567,
-0.0134450885044606));
#32029=CARTESIAN_POINT('Ctrl Pts',(0.00270772252782384,-0.0314188837085149,
-0.0134675291809873));
#32030=CARTESIAN_POINT('Ctrl Pts',(0.00270179214476104,-0.0314181611189366,
-0.0134798882265156));
#32031=CARTESIAN_POINT('Ctrl Pts',(0.00268369992440968,-0.0314160018911859,
-0.0135169395259518));
#32032=CARTESIAN_POINT('Ctrl Pts',(0.00267128248936854,-0.03141457968553,
-0.0135415060786094));
#32033=CARTESIAN_POINT('Ctrl Pts',(0.00260836656966896,-0.0314076439463513,
-0.0136618357521572));
#32034=CARTESIAN_POINT('Ctrl Pts',(0.00255304433699022,-0.0314023686725732,
-0.0137549949500218));
#32035=CARTESIAN_POINT('Ctrl Pts',(0.00234555301063521,-0.0313844856593905,
-0.0140648811823205));
#32036=CARTESIAN_POINT('Ctrl Pts',(0.00216986257507423,-0.031372258725037,
-0.0142643313843433));
#32037=CARTESIAN_POINT('Ctrl Pts',(0.00194162326719827,-0.0313569468116363,
-0.0144631100612533));
#32038=CARTESIAN_POINT('Ctrl Pts',(0.00191249201525883,-0.0313550042851653,
-0.0144875233746481));
#32039=CARTESIAN_POINT('Ctrl Pts',(0.00186391953869556,-0.0313517796866947,
-0.0145266826544384));
#32040=CARTESIAN_POINT('Ctrl Pts',(0.00184474790698277,-0.0313505104817068,
-0.0145417568936433));
#32041=CARTESIAN_POINT('Ctrl Pts',(0.0018097362839726,-0.0313481979203354,
-0.0145686014810363));
#32042=CARTESIAN_POINT('Ctrl Pts',(0.00179395978156127,-0.0313471577603407,
-0.0145804525498803));
#32043=CARTESIAN_POINT('Ctrl Pts',(0.0017596852443438,-0.0313449015345491,
-0.0146056740082139));
#32044=CARTESIAN_POINT('Ctrl Pts',(0.00174114931429377,-0.0313436835206924,
-0.0146189905985285));
#32045=CARTESIAN_POINT('Ctrl Pts',(0.00168906324631621,-0.0313402661006848,
-0.0146555164768901));
#32046=CARTESIAN_POINT('Ctrl Pts',(0.00165518982470938,-0.0313380494875459,
-0.0146782542558063));
#32047=CARTESIAN_POINT('Ctrl Pts',(0.00150954489042835,-0.031328539967362,
-0.0147717683267744));
#32048=CARTESIAN_POINT('Ctrl Pts',(0.0013936315773998,-0.0313210145901129,
-0.0148357941041013));
#32049=CARTESIAN_POINT('Ctrl Pts',(0.00110419203668995,-0.0313024486817675,
-0.0149715444243269));
#32050=CARTESIAN_POINT('Ctrl Pts',(0.000927422306658285,-0.0312912761316168,
-0.0150350515790807));
#32051=CARTESIAN_POINT('Ctrl Pts',(0.000677576093376061,-0.0312764320854631,
-0.0150991843095618));
#32052=CARTESIAN_POINT('Ctrl Pts',(0.000608664657924585,-0.0312724369399736,
-0.0151143056568378));
#32053=CARTESIAN_POINT('Ctrl Pts',(0.000519680685953666,-0.0312674566004465,
-0.0151305662917295));
#32054=CARTESIAN_POINT('Ctrl Pts',(0.00050004570725103,-0.0312663687127424,
-0.0151339525564994));
#32055=CARTESIAN_POINT('Ctrl Pts',(0.000468444621791647,-0.0312646371653898,
-0.0151390788581003));
#32056=CARTESIAN_POINT('Ctrl Pts',(0.000456499499758228,-0.0312639870672388,
-0.0151409425547589));
#32057=CARTESIAN_POINT('Ctrl Pts',(0.000433288890776407,-0.0312627328709774,
-0.0151444203215003));
#32058=CARTESIAN_POINT('Ctrl Pts',(0.000422025082156765,-0.0312621283866448,
-0.0151460425626311));
#32059=CARTESIAN_POINT('Ctrl Pts',(0.000394099656790599,-0.0312606395336177,
-0.0151499023892932));
#32060=CARTESIAN_POINT('Ctrl Pts',(0.000377427687005065,-0.03125975925898,
-0.0151520641277922));
#32061=CARTESIAN_POINT('Ctrl Pts',(0.000313582607630233,-0.0312564181606006,
-0.0151597973557237));
#32062=CARTESIAN_POINT('Ctrl Pts',(0.000266295691851007,-0.0312540058774051,
-0.0151643886013324));
#32063=CARTESIAN_POINT('Ctrl Pts',(0.000139661459569341,-0.0312476659085832,
-0.0151736541142784));
#32064=CARTESIAN_POINT('Ctrl Pts',(6.02021837856961E-5,-0.0312438128450981,
-0.0151763019387494));
#32065=CARTESIAN_POINT('Ctrl Pts',(-0.000288572217971681,-0.0312271127560565,
-0.0151740613578506));
#32066=CARTESIAN_POINT('Ctrl Pts',(-0.000556394659976168,-0.0312147155435352,
-0.0151360813573633));
#32067=CARTESIAN_POINT('Ctrl Pts',(-0.000851726205064238,-0.0311991931166643,
-0.0150526527310513));
#32068=CARTESIAN_POINT('Ctrl Pts',(-0.000887698667210124,-0.0311972724847522,
-0.0150417568947233));
#32069=CARTESIAN_POINT('Ctrl Pts',(-0.000946434687803124,-0.0311940824632114,
-0.0150227541753678));
#32070=CARTESIAN_POINT('Ctrl Pts',(-0.000969322326243007,-0.0311928257654935,
-0.0150150428667718));
#32071=CARTESIAN_POINT('Ctrl Pts',(-0.00101056608453178,-0.0311905353697205,
-0.015000590173402));
#32072=CARTESIAN_POINT('Ctrl Pts',(-0.00102895427187244,-0.0311895048288794,
-0.0149939440184654));
#32073=CARTESIAN_POINT('Ctrl Pts',(-0.00106847473170203,-0.031187269128904,
-0.0149792215291683));
#32074=CARTESIAN_POINT('Ctrl Pts',(-0.00108958315579977,-0.0311860620337089,
-0.0149710849879555));
#32075=CARTESIAN_POINT('Ctrl Pts',(-0.00114815581022576,-0.031182675446898,
-0.014947743060055));
#32076=CARTESIAN_POINT('Ctrl Pts',(-0.0011854067107046,-0.0311804789028494,
-0.0149320182660841));
#32077=CARTESIAN_POINT('Ctrl Pts',(-0.00134182742489207,-0.031171069675751,
-0.0148622304006374));
#32078=CARTESIAN_POINT('Ctrl Pts',(-0.00145769855270647,-0.0311636277363491,
-0.0148011592425416));
#32079=CARTESIAN_POINT('Ctrl Pts',(-0.00171305811342673,-0.0311462287398832,
-0.0146444400279809));
#32080=CARTESIAN_POINT('Ctrl Pts',(-0.00184920007179521,-0.0311361912019695,
-0.0145441745032702));
#32081=CARTESIAN_POINT('Ctrl Pts',(-0.00204258170369307,-0.0311212761457188,
-0.0143748638842227));
#32082=CARTESIAN_POINT('Ctrl Pts',(-0.00210638558295247,-0.0311162334913952,
-0.0143138265843286));
#32083=CARTESIAN_POINT('Ctrl Pts',(-0.00218204905555556,-0.0311101946113171,
-0.0142347632501576));
#32084=CARTESIAN_POINT('Ctrl Pts',(-0.0021965265517318,-0.0311090363285574,
-0.0142193110122424));
#32085=CARTESIAN_POINT('Ctrl Pts',(-0.00221916517892087,-0.0311072225151594,
-0.0141946295525209));
#32086=CARTESIAN_POINT('Ctrl Pts',(-0.00222743489747744,-0.0311065593823568,
-0.0141855013879904));
#32087=CARTESIAN_POINT('Ctrl Pts',(-0.00224318690042803,-0.0311052956349731,
-0.0141678975476417));
#32088=CARTESIAN_POINT('Ctrl Pts',(-0.00225067781662052,-0.0311046944215979,
-0.0141594301508696));
#32089=CARTESIAN_POINT('Ctrl Pts',(-0.00226874273178424,-0.0311032434619999,
-0.0141387762921927));
#32090=CARTESIAN_POINT('Ctrl Pts',(-0.00227926679560667,-0.0311023972457476,
-0.0141265462931545));
#32091=CARTESIAN_POINT('Ctrl Pts',(-0.00231679023185935,-0.0310993742522334,
-0.0140822220752352));
#32092=CARTESIAN_POINT('Ctrl Pts',(-0.00234321561369952,-0.0310972343076884,
-0.0140496461915277));
#32093=CARTESIAN_POINT('Ctrl Pts',(-0.00248316577396171,-0.031085775467706,
-0.0138695299299743));
#32094=CARTESIAN_POINT('Ctrl Pts',(-0.00258346125922145,-0.0310770765415037,
-0.0137122102260625));
#32095=CARTESIAN_POINT('Ctrl Pts',(-0.00273862325436582,-0.0310609522218785,
-0.0134101444924896));
#32096=CARTESIAN_POINT('Ctrl Pts',(-0.00279814150714647,-0.0310535972509047,
-0.0132685248418041));
#32097=CARTESIAN_POINT('Ctrl Pts',(-0.0028630507036099,-0.0310432847386282,
-0.0130734427079798));
#32098=CARTESIAN_POINT('Ctrl Pts',(-0.00287823778146051,-0.0310406300511755,
-0.0130234811346886));
#32099=CARTESIAN_POINT('Ctrl Pts',(-0.00289878162064657,-0.031036638817784,
-0.0129489604864606));
#32100=CARTESIAN_POINT('Ctrl Pts',(-0.00290514642074537,-0.0310353339747879,
-0.0129246882828097));
#32101=CARTESIAN_POINT('Ctrl Pts',(-0.0029159950978677,-0.0310329806480193,
-0.0128810950030002));
#32102=CARTESIAN_POINT('Ctrl Pts',(-0.00292059329966039,-0.0310319358267159,
-0.0128618037529944));
#32103=CARTESIAN_POINT('Ctrl Pts',(-0.00292998490398528,-0.0310296961654827,
-0.0128205949190631));
#32104=CARTESIAN_POINT('Ctrl Pts',(-0.00293472436702019,-0.0310284997103785,
-0.012798666391128));
#32105=CARTESIAN_POINT('Ctrl Pts',(-0.0029439065293226,-0.0310260388579148,
-0.0127537481998373));
#32106=CARTESIAN_POINT('Ctrl Pts',(-0.00294832691177362,-0.0310247738605681,
-0.01273075558765));
#32107=CARTESIAN_POINT('Ctrl Pts',(-0.00296272745672576,-0.0310203565785813,
-0.0126508149482916));
#32108=CARTESIAN_POINT('Ctrl Pts',(-0.00297132983262019,-0.0310171630659669,
-0.0125936343075038));
#32109=CARTESIAN_POINT('Ctrl Pts',(-0.00299283479013691,-0.0310071339804914,
-0.0124159166586095));
#32110=CARTESIAN_POINT('Ctrl Pts',(-0.00300008853944841,-0.031000148781098,
-0.0122948279177128));
#32111=CARTESIAN_POINT('Ctrl Pts',(-0.00299999918450973,-0.0309930707801491,
-0.0121736412872464));
#32112=CARTESIAN_POINT('',(-0.00299999972093215,-0.0369945846061161,-0.0121745592977555));
#32113=CARTESIAN_POINT('Ctrl Pts',(-0.00299999981352154,-0.0319945472736604,
-0.0121769110534288));
#32114=CARTESIAN_POINT('Ctrl Pts',(-0.00299992166945358,-0.0320055173499198,
-0.0123985404084296));
#32115=CARTESIAN_POINT('Ctrl Pts',(-0.00297528701221253,-0.0320157939746235,
-0.0126194602075733));
#32116=CARTESIAN_POINT('Ctrl Pts',(-0.00290221263423182,-0.0320317016547023,
-0.0129435765333841));
#32117=CARTESIAN_POINT('Ctrl Pts',(-0.00287193455456266,-0.0320370815248905,
-0.0130500529918593));
#32118=CARTESIAN_POINT('Ctrl Pts',(-0.00282675542114908,-0.0320441503505141,
-0.0131809557000143));
#32119=CARTESIAN_POINT('Ctrl Pts',(-0.00281729432308356,-0.0320455899518007,
-0.0132071775153452));
#32120=CARTESIAN_POINT('Ctrl Pts',(-0.00280259606184744,-0.0320477731400695,
-0.0132462020566344));
#32121=CARTESIAN_POINT('Ctrl Pts',(-0.00279763329257718,-0.0320485018376998,
-0.0132591072369983));
#32122=CARTESIAN_POINT('Ctrl Pts',(-0.0027884946320194,-0.0320498294736284,
-0.0132823896872612));
#32123=CARTESIAN_POINT('Ctrl Pts',(-0.00278434967702218,-0.0320504266391192,
-0.0132927785238499));
#32124=CARTESIAN_POINT('Ctrl Pts',(-0.00277481854911974,-0.0320517886265605,
-0.0133162843788565));
#32125=CARTESIAN_POINT('Ctrl Pts',(-0.00276939743826002,-0.0320525554163635,
-0.0133293864979761));
#32126=CARTESIAN_POINT('Ctrl Pts',(-0.00275232871801576,-0.0320549446140336,
-0.0133698254784093));
#32127=CARTESIAN_POINT('Ctrl Pts',(-0.00274036799482192,-0.0320565838122045,
-0.0133970273486267));
#32128=CARTESIAN_POINT('Ctrl Pts',(-0.00266562925274479,-0.0320666026904978,
-0.0135603736836576));
#32129=CARTESIAN_POINT('Ctrl Pts',(-0.00259312580604794,-0.0320753989577528,
-0.0136918243278081));
#32130=CARTESIAN_POINT('Ctrl Pts',(-0.00246031502295989,-0.0320896669141343,
-0.0138950008108519));
#32131=CARTESIAN_POINT('Ctrl Pts',(-0.00240594014769667,-0.0320951245132674,
-0.0139703089356163));
#32132=CARTESIAN_POINT('Ctrl Pts',(-0.00226686810629769,-0.0321080957540019,
-0.0141452108714532));
#32133=CARTESIAN_POINT('Ctrl Pts',(-0.00217898026176169,-0.0321155239350369,
-0.0142420361567347));
#32134=CARTESIAN_POINT('Ctrl Pts',(-0.00205580627442135,-0.0321249357397831,
-0.0143611027083987));
#32135=CARTESIAN_POINT('Ctrl Pts',(-0.00202598825148812,-0.0321271458988904,
-0.0143887758558819));
#32136=CARTESIAN_POINT('Ctrl Pts',(-0.00197851292600666,-0.0321305613644986,
-0.0144310719609503));
#32137=CARTESIAN_POINT('Ctrl Pts',(-0.00196123594672582,-0.0321317837147886,
-0.0144461128021712));
#32138=CARTESIAN_POINT('Ctrl Pts',(-0.00192863706421125,-0.0321340525430364,
-0.0144738425658064));
#32139=CARTESIAN_POINT('Ctrl Pts',(-0.00191335802319091,-0.032135100934317,
-0.0144865797423342));
#32140=CARTESIAN_POINT('Ctrl Pts',(-0.00187882236376268,-0.0321374378502508,
-0.0145147925241981));
#32141=CARTESIAN_POINT('Ctrl Pts',(-0.0018594988906304,-0.0321387230276193,
-0.0145301842222729));
#32142=CARTESIAN_POINT('Ctrl Pts',(-0.00180938542209416,-0.0321420006718816,
-0.0145690991062663));
#32143=CARTESIAN_POINT('Ctrl Pts',(-0.00177832543406964,-0.0321439796091278,
-0.0145922679819327));
#32144=CARTESIAN_POINT('Ctrl Pts',(-0.00153333466509974,-0.0321592102277868,
-0.0147677333599231));
#32145=CARTESIAN_POINT('Ctrl Pts',(-0.00130070754058425,-0.0321713400748168,
-0.0148919384817944));
#32146=CARTESIAN_POINT('Ctrl Pts',(-0.000978870743146697,-0.0321878039105082,
-0.0150128242086367));
#32147=CARTESIAN_POINT('Ctrl Pts',(-0.000901740788853144,-0.0321917386608914,
-0.0150382743173766));
#32148=CARTESIAN_POINT('Ctrl Pts',(-0.000777222210865428,-0.032198202836921,
-0.0150738283954862));
#32149=CARTESIAN_POINT('Ctrl Pts',(-0.000730455062710333,-0.0322006553988329,
-0.0150859682357734));
#32150=CARTESIAN_POINT('Ctrl Pts',(-0.000666774969706172,-0.0322040525418524,
-0.0151008666680006));
#32151=CARTESIAN_POINT('Ctrl Pts',(-0.000650099628271567,-0.0322049474242707,
-0.0151046179730234));
#32152=CARTESIAN_POINT('Ctrl Pts',(-0.000622088780710364,-0.0322064608534237,
-0.0151106683247944));
#32153=CARTESIAN_POINT('Ctrl Pts',(-0.000610770112324474,-0.032207075195398,
-0.0151130447387011));
#32154=CARTESIAN_POINT('Ctrl Pts',(-0.000587450282326003,-0.0322083471450999,
-0.0151178002350297));
#32155=CARTESIAN_POINT('Ctrl Pts',(-0.000575447915660388,-0.032209005132621,
-0.0151201714364311));
#32156=CARTESIAN_POINT('Ctrl Pts',(-0.000543547495604881,-0.0322107621833263,
-0.015126271215151));
#32157=CARTESIAN_POINT('Ctrl Pts',(-0.000523625946324464,-0.0322118679167358,
-0.0151298718474032));
#32158=CARTESIAN_POINT('Ctrl Pts',(-0.000432001044636205,-0.0322169875534955,
-0.015145476245953));
#32159=CARTESIAN_POINT('Ctrl Pts',(-0.000359916816942563,-0.032221110388206,
-0.0151550719481401));
#32160=CARTESIAN_POINT('Ctrl Pts',(-6.04147719155483E-5,-0.032238446194825,
-0.0151839130931893));
#32161=CARTESIAN_POINT('Ctrl Pts',(0.00016849004050524,-0.0322521145788547,
-0.0151798002863055));
#32162=CARTESIAN_POINT('Ctrl Pts',(0.000498703642215855,-0.0322711847942824,
-0.0151359707762295));
#32163=CARTESIAN_POINT('Ctrl Pts',(0.000601888687158601,-0.0322770618066293,
-0.0151167263528632));
#32164=CARTESIAN_POINT('Ctrl Pts',(0.000735151277624789,-0.0322845272222606,
-0.0150845623862352));
#32165=CARTESIAN_POINT('Ctrl Pts',(0.000766317425899855,-0.0322862644083889,
-0.0150765073058159));
#32166=CARTESIAN_POINT('Ctrl Pts',(0.000817715459811999,-0.0322891156359211,
-0.0150623369186903));
#32167=CARTESIAN_POINT('Ctrl Pts',(0.000838022619209465,-0.0322902385815438,
-0.0150565067631455));
#32168=CARTESIAN_POINT('Ctrl Pts',(0.000877620389305425,-0.0322924217567312,
-0.0150446841287081));
#32169=CARTESIAN_POINT('Ctrl Pts',(0.000896915375805811,-0.032293482515093,
-0.0150387103880561));
#32170=CARTESIAN_POINT('Ctrl Pts',(0.000943240260131015,-0.032296022587275,
-0.0150238538555277));
#32171=CARTESIAN_POINT('Ctrl Pts',(0.000970207238362803,-0.0322974957037417,
-0.0150147804456876));
#32172=CARTESIAN_POINT('Ctrl Pts',(0.0010609398053361,-0.0323024367613863,
-0.0149828083417565));
#32173=CARTESIAN_POINT('Ctrl Pts',(0.00112405938926173,-0.0323058476588138,
-0.014958133157303));
#32174=CARTESIAN_POINT('Ctrl Pts',(0.00140089283297222,-0.03232077438795,
-0.0148389508221372));
#32175=CARTESIAN_POINT('Ctrl Pts',(0.00160395511914783,-0.0323315630356229,
-0.0147218138867613));
#32176=CARTESIAN_POINT('Ctrl Pts',(0.00185109379034802,-0.0323463686431329,
-0.0145378430138683));
#32177=CARTESIAN_POINT('Ctrl Pts',(0.00190913996170871,-0.0323499928684846,
-0.0144911777132555));
#32178=CARTESIAN_POINT('Ctrl Pts',(0.0019998457344721,-0.0323560011650617,
-0.0144125243050791));
#32179=CARTESIAN_POINT('Ctrl Pts',(0.00203361676734141,-0.0323583210968015,
-0.0143818638576635));
#32180=CARTESIAN_POINT('Ctrl Pts',(0.00207880516695753,-0.0323615617791868,
-0.0143389180477261));
#32181=CARTESIAN_POINT('Ctrl Pts',(0.00209083931783159,-0.0323624385407105,
-0.0143272879254064));
#32182=CARTESIAN_POINT('Ctrl Pts',(0.00211097734140315,-0.0323639303524099,
-0.0143074974665686));
#32183=CARTESIAN_POINT('Ctrl Pts',(0.00211913293054328,-0.0323645414725223,
-0.0142993899277437));
#32184=CARTESIAN_POINT('Ctrl Pts',(0.00213595447204794,-0.0323658169319017,
-0.0142824740809798));
#32185=CARTESIAN_POINT('Ctrl Pts',(0.00214461287168771,-0.0323664817657812,
-0.0142736588776297));
#32186=CARTESIAN_POINT('Ctrl Pts',(0.00216770254568187,-0.0323682765492183,
-0.0142498587067067));
#32187=CARTESIAN_POINT('Ctrl Pts',(0.00218203257340995,-0.0323694136597469,
-0.0142347769399615));
#32188=CARTESIAN_POINT('Ctrl Pts',(0.00225038940708793,-0.0323749456846762,
-0.014161319011261));
#32189=CARTESIAN_POINT('Ctrl Pts',(0.00230223365563165,-0.0323794710952268,
-0.0141009623659906));
#32190=CARTESIAN_POINT('Ctrl Pts',(0.00244882559842434,-0.0323931170667211,
-0.0139159003603096));
#32191=CARTESIAN_POINT('Ctrl Pts',(0.00253627997155106,-0.0324024102409782,
-0.0137857584550647));
#32192=CARTESIAN_POINT('Ctrl Pts',(0.0026659965369315,-0.0324178222284253,
-0.0135557177743364));
#32193=CARTESIAN_POINT('Ctrl Pts',(0.00271374348830112,-0.0324240166117465,
-0.0134592717120003));
#32194=CARTESIAN_POINT('Ctrl Pts',(0.00278391722210011,-0.0324340017272394,
-0.0132959997482678));
#32195=CARTESIAN_POINT('Ctrl Pts',(0.00280935476756636,-0.0324378775121089,
-0.0132305807779069));
#32196=CARTESIAN_POINT('Ctrl Pts',(0.00284173914581808,-0.0324432025059446,
-0.0131377830954056));
#32197=CARTESIAN_POINT('Ctrl Pts',(0.00285062870797352,-0.0324447135945916,
-0.0131111106693456));
#32198=CARTESIAN_POINT('Ctrl Pts',(0.00286530169601771,-0.0324472971696995,
-0.0130649314129799));
#32199=CARTESIAN_POINT('Ctrl Pts',(0.00287126392981967,-0.0324483753352332,
-0.0130454837809158));
#32200=CARTESIAN_POINT('Ctrl Pts',(0.00288233821074679,-0.0324504346642358,
-0.0130080056730721));
#32201=CARTESIAN_POINT('Ctrl Pts',(0.00288747998499075,-0.0324514167348727,
-0.0129899850404862));
#32202=CARTESIAN_POINT('Ctrl Pts',(0.0029005917386521,-0.032453992290725,
-0.01294234423061));
#32203=CARTESIAN_POINT('Ctrl Pts',(0.0029082769902684,-0.0324555767292192,
-0.0129126475847428));
#32204=CARTESIAN_POINT('Ctrl Pts',(0.00293497830326661,-0.0324613792018762,
-0.0128025350550199));
#32205=CARTESIAN_POINT('Ctrl Pts',(0.00295112583945495,-0.0324655084800149,
-0.0127214588180163));
#32206=CARTESIAN_POINT('Ctrl Pts',(0.00300123153964023,-0.0324814029094778,
-0.0124013705008864));
#32207=CARTESIAN_POINT('Ctrl Pts',(0.00300964554019078,-0.0324924682081842,
-0.0121593119664037));
#32208=CARTESIAN_POINT('Ctrl Pts',(0.00298408003833383,-0.0325069813386115,
-0.0118619600557041));
#32209=CARTESIAN_POINT('Ctrl Pts',(0.0029775629986748,-0.0325097976698275,
-0.0118052043441688));
#32210=CARTESIAN_POINT('Ctrl Pts',(0.00296402610454635,-0.0325145922894124,
-0.0117111064459493));
#32211=CARTESIAN_POINT('Ctrl Pts',(0.00295790980565575,-0.032516534315531,
-0.0116736484394402));
#32212=CARTESIAN_POINT('Ctrl Pts',(0.00294827786134798,-0.0325193253770335,
-0.011620964776072));
#32213=CARTESIAN_POINT('Ctrl Pts',(0.00294535114104303,-0.0325201447529038,
-0.0116056338180784));
#32214=CARTESIAN_POINT('Ctrl Pts',(0.00294009660696255,-0.0325215694117716,
-0.0115792294792531));
#32215=CARTESIAN_POINT('Ctrl Pts',(0.00293782550315667,-0.0325221716079568,
-0.0115681450205364));
#32216=CARTESIAN_POINT('Ctrl Pts',(0.0029328430745997,-0.0325234649045223,
-0.0115445083735146));
#32217=CARTESIAN_POINT('Ctrl Pts',(0.00293011382399383,-0.0325241569266596,
-0.0115319605424998));
#32218=CARTESIAN_POINT('Ctrl Pts',(0.00292239195393721,-0.032526070355148,
-0.0114975250005768));
#32219=CARTESIAN_POINT('Ctrl Pts',(0.00291723416172802,-0.0325273003337825,
-0.0114756756069955));
#32220=CARTESIAN_POINT('Ctrl Pts',(0.00288134451692469,-0.0325355453891919,
-0.0113309256608267));
#32221=CARTESIAN_POINT('Ctrl Pts',(0.00284310164768706,-0.0325428910871948,
-0.011210029056896));
#32222=CARTESIAN_POINT('Ctrl Pts',(0.00273179299120794,-0.032560942920508,
-0.0109227708690137));
#32223=CARTESIAN_POINT('Ctrl Pts',(0.00265103524736783,-0.0325716738933144,
-0.0107598978359552));
#32224=CARTESIAN_POINT('Ctrl Pts',(0.00250625269746859,-0.0325874331740844,
-0.010524264173937));
#32225=CARTESIAN_POINT('Ctrl Pts',(0.00245262243289094,-0.0325927436274197,
-0.0104456235235701));
#32226=CARTESIAN_POINT('Ctrl Pts',(0.00237654438931704,-0.0325996170188491,
-0.0103447302704393));
#32227=CARTESIAN_POINT('Ctrl Pts',(0.00235735903153334,-0.032601300519603,
-0.0103200965054498));
#32228=CARTESIAN_POINT('Ctrl Pts',(0.00232467622422405,-0.0326040876941123,
-0.010279457109224));
#32229=CARTESIAN_POINT('Ctrl Pts',(0.00231138980330054,-0.0326051994718929,
-0.0102632855842512));
#32230=CARTESIAN_POINT('Ctrl Pts',(0.00228486449201811,-0.0326073781131245,
-0.0102316805503514));
#32231=CARTESIAN_POINT('Ctrl Pts',(0.00227163578727992,-0.032608445294884,
-0.0102162399951401));
#32232=CARTESIAN_POINT('Ctrl Pts',(0.00223902535675638,-0.0326110301620434,
-0.0101789510957121));
#32233=CARTESIAN_POINT('Ctrl Pts',(0.00221947940071062,-0.0326125410703105,
-0.010157248774908));
#32234=CARTESIAN_POINT('Ctrl Pts',(0.00215033974763172,-0.0326177579253327,
-0.0100826999844979));
#32235=CARTESIAN_POINT('Ctrl Pts',(0.00209914915478378,-0.0326213975309861,
-0.0100313660262812));
#32236=CARTESIAN_POINT('Ctrl Pts',(0.00189354722922503,-0.0326352770896497,
-0.00983961252477843));
#32237=CARTESIAN_POINT('Ctrl Pts',(0.00172652019459439,-0.0326449848259004,
-0.00971360406131355));
#32238=CARTESIAN_POINT('Ctrl Pts',(0.00144757581956135,-0.0326605420522651,
-0.00954560551421155));
#32239=CARTESIAN_POINT('Ctrl Pts',(0.00134395058867059,-0.032666210434021,
-0.00949117986156228));
#32240=CARTESIAN_POINT('Ctrl Pts',(0.0012113819371863,-0.0326736318921978,
-0.00943115458018942));
#32241=CARTESIAN_POINT('Ctrl Pts',(0.00118517422587893,-0.0326751071197383,
-0.00941973661116304));
#32242=CARTESIAN_POINT('Ctrl Pts',(0.00114592700423578,-0.0326773338713265,
-0.00940330097383683));
#32243=CARTESIAN_POINT('Ctrl Pts',(0.00113300847073552,-0.032678069619199,
-0.00939799677189846));
#32244=CARTESIAN_POINT('Ctrl Pts',(0.00110967773246729,-0.0326794041848032,
-0.00938860725748957));
#32245=CARTESIAN_POINT('Ctrl Pts',(0.00109927907879504,-0.032680001124699,
-0.00938448971386351));
#32246=CARTESIAN_POINT('Ctrl Pts',(0.0010757778988961,-0.0326813550277411,
-0.00937533566589626));
#32247=CARTESIAN_POINT('Ctrl Pts',(0.00106266297292496,-0.0326821138494114,
-0.0093703329387648));
#32248=CARTESIAN_POINT('Ctrl Pts',(0.00102238496414359,-0.0326844532311081,
-0.00935529171375322));
#32249=CARTESIAN_POINT('Ctrl Pts',(0.000995111938646888,-0.0326860496282743,
-0.00934555459038613));
#32250=CARTESIAN_POINT('Ctrl Pts',(0.000805473912642518,-0.0326972141969443,
-0.0092809290075445));
#32251=CARTESIAN_POINT('Ctrl Pts',(0.000638816061479365,-0.0327073312237352,
-0.00923965144348039));
#32252=CARTESIAN_POINT('Ctrl Pts',(0.000268469143708647,-0.0327293653127623,
-0.00918096143610414));
#32253=CARTESIAN_POINT('Ctrl Pts',(6.46302958511912E-5,-0.0327411840007304,
-0.00916964339219376));
#32254=CARTESIAN_POINT('Ctrl Pts',(-0.000179255189209165,-0.0327545947917013,
-0.00918093972414194));
#32255=CARTESIAN_POINT('Ctrl Pts',(-0.00021966381359147,-0.0327567947543597,
-0.0091836320890782));
#32256=CARTESIAN_POINT('Ctrl Pts',(-0.000282790289156459,-0.0327601982062204,
-0.00918912386090277));
#32257=CARTESIAN_POINT('Ctrl Pts',(-0.000305550639576867,-0.0327614185395813,
-0.00919136642020448));
#32258=CARTESIAN_POINT('Ctrl Pts',(-0.000348061143262737,-0.0327636856364911,
-0.0091960463575681));
#32259=CARTESIAN_POINT('Ctrl Pts',(-0.000367816883783583,-0.0327647342841296,
-0.00919842038909919));
#32260=CARTESIAN_POINT('Ctrl Pts',(-0.000412099716339356,-0.0327670743331952,
-0.00920418930028557));
#32261=CARTESIAN_POINT('Ctrl Pts',(-0.000436611481917395,-0.032768362348695,
-0.00920769165267517));
#32262=CARTESIAN_POINT('Ctrl Pts',(-0.000499547970773524,-0.0327716523320715,
-0.00921748082835111));
#32263=CARTESIAN_POINT('Ctrl Pts',(-0.000537899259255123,-0.0327736405948655,
-0.00922421300765051));
#32264=CARTESIAN_POINT('Ctrl Pts',(-0.000832889335224644,-0.0327888299829616,
-0.00928193625555256));
#32265=CARTESIAN_POINT('Ctrl Pts',(-0.0010819778461849,-0.032800919810724,
-0.00936555331976436));
#32266=CARTESIAN_POINT('Ctrl Pts',(-0.00141634338670296,-0.0328187387356199,
-0.00952893421971835));
#32267=CARTESIAN_POINT('Ctrl Pts',(-0.00151285702359624,-0.0328241128642027,
-0.00958288802923117));
#32268=CARTESIAN_POINT('Ctrl Pts',(-0.00162969908636198,-0.0328311746570709,
-0.00965695329224874));
#32269=CARTESIAN_POINT('Ctrl Pts',(-0.00165302178684557,-0.0328326135581808,
-0.00967219692814457));
#32270=CARTESIAN_POINT('Ctrl Pts',(-0.00168759364462411,-0.0328347959268218,
-0.00969548661783823));
#32271=CARTESIAN_POINT('Ctrl Pts',(-0.00169900555087693,-0.0328355245242688,
-0.00970328958785137));
#32272=CARTESIAN_POINT('Ctrl Pts',(-0.0017195536696144,-0.0328368521303197,
-0.00971754892674381));
#32273=CARTESIAN_POINT('Ctrl Pts',(-0.00172870824484938,-0.0328374493685929,
-0.00972397789350106));
#32274=CARTESIAN_POINT('Ctrl Pts',(-0.00174938946421828,-0.0328388117345902,
-0.00973867505776245));
#32275=CARTESIAN_POINT('Ctrl Pts',(-0.00176089351910897,-0.0328395788335015,
-0.00974697387109865));
#32276=CARTESIAN_POINT('Ctrl Pts',(-0.00179633299833518,-0.032841969710869,
-0.00977292336533869));
#32277=CARTESIAN_POINT('Ctrl Pts',(-0.0018200644900702,-0.0328436103089866,
-0.00979084813585035));
#32278=CARTESIAN_POINT('Ctrl Pts',(-0.00195506528379238,-0.0328531547718727,
-0.00989600468785276));
#32279=CARTESIAN_POINT('Ctrl Pts',(-0.00206031650086878,-0.0328614287151167,
-0.0099906576487612));
#32280=CARTESIAN_POINT('Ctrl Pts',(-0.00224502743731311,-0.0328770569085845,
-0.0101820185758428));
#32281=CARTESIAN_POINT('Ctrl Pts',(-0.00232589572411779,-0.0328843895324159,
-0.0102769755549302));
#32282=CARTESIAN_POINT('Ctrl Pts',(-0.0024489312183982,-0.0328962135913298,
-0.0104411419692128));
#32283=CARTESIAN_POINT('Ctrl Pts',(-0.00249462283158707,-0.0329007898126726,
-0.0105075170366111));
#32284=CARTESIAN_POINT('Ctrl Pts',(-0.00256824451806549,-0.032908478129321,
-0.0106242660786101));
#32285=CARTESIAN_POINT('Ctrl Pts',(-0.00259749695443269,-0.0329116327346472,
-0.0106737504437575));
#32286=CARTESIAN_POINT('Ctrl Pts',(-0.00263794261370985,-0.0329161475994535,
-0.010746888606416));
#32287=CARTESIAN_POINT('Ctrl Pts',(-0.00265027569224967,-0.0329175472222114,
-0.0107698945020977));
#32288=CARTESIAN_POINT('Ctrl Pts',(-0.00267154137063943,-0.0329200026785584,
-0.0108108375164946));
#32289=CARTESIAN_POINT('Ctrl Pts',(-0.00268059734261315,-0.0329210627237353,
-0.0108287084315491));
#32290=CARTESIAN_POINT('Ctrl Pts',(-0.00269924922945755,-0.0329232773528835,
-0.0108664486919383));
#32291=CARTESIAN_POINT('Ctrl Pts',(-0.00270880634880097,-0.0329244305671278,
-0.0108863359373756));
#32292=CARTESIAN_POINT('Ctrl Pts',(-0.00273365435223098,-0.0329274801698911,
-0.0109395372340126));
#32293=CARTESIAN_POINT('Ctrl Pts',(-0.0027485557856385,-0.0329293634497668,
-0.0109730296335553));
#32294=CARTESIAN_POINT('Ctrl Pts',(-0.00282912690062542,-0.0329398794232708,
-0.0111634424770784));
#32295=CARTESIAN_POINT('Ctrl Pts',(-0.00288197279446224,-0.0329480801035526,
-0.0113254561754642));
#32296=CARTESIAN_POINT('Ctrl Pts',(-0.00294890414246313,-0.0329620206730747,
-0.011610946592213));
#32297=CARTESIAN_POINT('Ctrl Pts',(-0.0029695988553946,-0.0329678079904462,
-0.0117324161747555));
#32298=CARTESIAN_POINT('Ctrl Pts',(-0.00299010405574497,-0.0329770485944898,
-0.0119229274919511));
#32299=CARTESIAN_POINT('Ctrl Pts',(-0.00299509980891963,-0.0329803971854066,
-0.0119912728145086));
#32300=CARTESIAN_POINT('Ctrl Pts',(-0.00299941996449915,-0.0329859960547779,
-0.012102794483972));
#32301=CARTESIAN_POINT('Ctrl Pts',(-0.00300015994582249,-0.0329881925506409,
-0.0121458923110202));
#32302=CARTESIAN_POINT('Ctrl Pts',(-0.00299989950004612,-0.0329912869608121,
-0.0122053736321074));
#32303=CARTESIAN_POINT('Ctrl Pts',(-0.00299969353153812,-0.0329921458709777,
-0.0122217570393376));
#32304=CARTESIAN_POINT('Ctrl Pts',(-0.00299911592893773,-0.0329936164888288,
-0.01224957198816));
#32305=CARTESIAN_POINT('Ctrl Pts',(-0.0029988131011394,-0.0329942245314662,
-0.0122610048264721));
#32306=CARTESIAN_POINT('Ctrl Pts',(-0.00299804286267508,-0.032995504184675,
-0.0122849172308662));
#32307=CARTESIAN_POINT('Ctrl Pts',(-0.00299756289825817,-0.0329961764108415,
-0.0122973959137909));
#32308=CARTESIAN_POINT('Ctrl Pts',(-0.00299604856014054,-0.0329980120866952,
-0.0123312606805601));
#32309=CARTESIAN_POINT('Ctrl Pts',(-0.00299486313982953,-0.0329991832445347,
-0.0123526389055684));
#32310=CARTESIAN_POINT('Ctrl Pts',(-0.00298757625331354,-0.0330052711742289,
-0.0124627225053163));
#32311=CARTESIAN_POINT('Ctrl Pts',(-0.00297776251179711,-0.0330103511285655,
-0.0125511315738183));
#32312=CARTESIAN_POINT('Ctrl Pts',(-0.00293115631127013,-0.0330278680810998,
-0.0128494225515542));
#32313=CARTESIAN_POINT('Ctrl Pts',(-0.00287594820590763,-0.0330405784405571,
-0.0130558001791282));
#32314=CARTESIAN_POINT('Ctrl Pts',(-0.00276260918550312,-0.0330586007414142,
-0.013349917944923));
#32315=CARTESIAN_POINT('Ctrl Pts',(-0.0027210254768088,-0.033064319410711,
-0.01344331568927));
#32316=CARTESIAN_POINT('Ctrl Pts',(-0.0026602938011974,-0.0330716203207372,
-0.0135628847842095));
#32317=CARTESIAN_POINT('Ctrl Pts',(-0.00264538053097433,-0.0330733431747509,
-0.0135911205535627));
#32318=CARTESIAN_POINT('Ctrl Pts',(-0.00261988110033155,-0.0330761772561545,
-0.0136375875585848));
#32319=CARTESIAN_POINT('Ctrl Pts',(-0.00260954873224065,-0.0330772971725537,
-0.0136559544676992));
#32320=CARTESIAN_POINT('Ctrl Pts',(-0.00258891961630967,-0.0330794789079732,
-0.0136917373424804));
#32321=CARTESIAN_POINT('Ctrl Pts',(-0.00257863854166791,-0.0330805412011469,
-0.0137091610014726));
#32322=CARTESIAN_POINT('Ctrl Pts',(-0.00255337899631024,-0.0330830924035305,
-0.0137509964225757));
#32323=CARTESIAN_POINT('Ctrl Pts',(-0.00253822553245452,-0.0330845749708349,
-0.0137753005087406));
#32324=CARTESIAN_POINT('Ctrl Pts',(-0.00248535592403487,-0.0330895913838888,
-0.0138574520198853));
#32325=CARTESIAN_POINT('Ctrl Pts',(-0.00244599060993135,-0.0330930656584217,
-0.0139142143502755));
#32326=CARTESIAN_POINT('Ctrl Pts',(-0.00227790742465114,-0.0331069760118501,
-0.0141395506315653));
#32327=CARTESIAN_POINT('Ctrl Pts',(-0.00213345448280931,-0.033116842293934,
-0.014295603992161));
#32328=CARTESIAN_POINT('Ctrl Pts',(-0.00188478915500416,-0.0331326118771023,
-0.014512843740485));
#32329=CARTESIAN_POINT('Ctrl Pts',(-0.00179132123783731,-0.0331383334318685,
-0.0145852345641472));
#32330=CARTESIAN_POINT('Ctrl Pts',(-0.00167013892449132,-0.0331458199071841,
-0.0146681334670934));
#32331=CARTESIAN_POINT('Ctrl Pts',(-0.00164620846690638,-0.0331473015546009,
-0.0146840044173829));
#32332=CARTESIAN_POINT('Ctrl Pts',(-0.00161028606276926,-0.0331495361484292,
-0.0147070930053033));
#32333=CARTESIAN_POINT('Ctrl Pts',(-0.00159846485418756,-0.0331502731562743,
-0.0147145745813318));
#32334=CARTESIAN_POINT('Ctrl Pts',(-0.00157709953040147,-0.0331516089681638,
-0.0147278881935737));
#32335=CARTESIAN_POINT('Ctrl Pts',(-0.00156757454384238,-0.0331522058755729,
-0.0147337499100779));
#32336=CARTESIAN_POINT('Ctrl Pts',(-0.00154604276038328,-0.0331535583738044,
-0.0147468352225556));
#32337=CARTESIAN_POINT('Ctrl Pts',(-0.00153401806878773,-0.0331543158040819,
-0.0147540280054991));
#32338=CARTESIAN_POINT('Ctrl Pts',(-0.00149710022190958,-0.0331566466073993,
-0.0147757613656154));
#32339=CARTESIAN_POINT('Ctrl Pts',(-0.00147204812588664,-0.0331582356568215,
-0.0147900272076437));
#32340=CARTESIAN_POINT('Ctrl Pts',(-0.00129101856542265,-0.0331697496668045,
-0.0148896866967588));
#32341=CARTESIAN_POINT('Ctrl Pts',(-0.00112793567096009,-0.0331802654276589,
-0.0149614185908662));
#32342=CARTESIAN_POINT('Ctrl Pts',(-0.00077233170150796,-0.0332023115359165,
-0.0150814541759144));
#32343=CARTESIAN_POINT('Ctrl Pts',(-0.000579384430463109,-0.033213755814049,
-0.015125996809585));
#32344=CARTESIAN_POINT('Ctrl Pts',(-0.000343359078784814,-0.0332268266714737,
-0.0151564132071683));
#32345=CARTESIAN_POINT('Ctrl Pts',(-0.000303179887337522,-0.0332290219563693,
-0.0151607678696518));
#32346=CARTESIAN_POINT('Ctrl Pts',(-0.000240159612160641,-0.0332324198479801,
-0.0151663123768961));
#32347=CARTESIAN_POINT('Ctrl Pts',(-0.000217373075255318,-0.033233639209211,
-0.0151680550169615));
#32348=CARTESIAN_POINT('Ctrl Pts',(-0.000174711645488774,-0.0332359054017205,
-0.0151708277101129));
#32349=CARTESIAN_POINT('Ctrl Pts',(-0.000154842220985072,-0.0332369541039347,
-0.0151719206871323));
#32350=CARTESIAN_POINT('Ctrl Pts',(-0.000110204933870383,-0.033239295422961,
-0.0151739308507323));
#32351=CARTESIAN_POINT('Ctrl Pts',(-8.54334777083388E-5,-0.0332405846366736,
-0.0151747389757358));
#32352=CARTESIAN_POINT('Ctrl Pts',(-2.16470892373925E-5,-0.0332438799663497,
-0.0151760288802137));
#32353=CARTESIAN_POINT('Ctrl Pts',(1.73728845334115E-5,-0.0332458722988661,
-0.0151760567039553));
#32354=CARTESIAN_POINT('Ctrl Pts',(0.000317576084153704,-0.0332610438022461,
-0.0151704135419899));
#32355=CARTESIAN_POINT('Ctrl Pts',(0.000576993607931816,-0.0332731161602666,
-0.0151314117228422));
#32356=CARTESIAN_POINT('Ctrl Pts',(0.000934497588884458,-0.0332909244266531,
-0.0150287415744288));
#32357=CARTESIAN_POINT('Ctrl Pts',(0.00103912771924805,-0.0332963084976614,
-0.0149923168412694));
#32358=CARTESIAN_POINT('Ctrl Pts',(0.00116728565105564,-0.0333033824397116,
-0.0149395866110209));
#32359=CARTESIAN_POINT('Ctrl Pts',(0.00119292487951236,-0.0333048225880542,
-0.0149286169536524));
#32360=CARTESIAN_POINT('Ctrl Pts',(0.00123104408750131,-0.0333070064780859,
-0.0149116752302599));
#32361=CARTESIAN_POINT('Ctrl Pts',(0.0012436423648252,-0.033307735318794,
-0.0149059713988036));
#32362=CARTESIAN_POINT('Ctrl Pts',(0.00126635932555961,-0.0333090631555048,
-0.01489549649891));
#32363=CARTESIAN_POINT('Ctrl Pts',(0.00127649136085391,-0.0333096603774527,
-0.0148907556679226));
#32364=CARTESIAN_POINT('Ctrl Pts',(0.00129940624072964,-0.0333110224300769,
-0.0148798770447648));
#32365=CARTESIAN_POINT('Ctrl Pts',(0.00131217218915115,-0.033311789227905,
-0.014873705245706));
#32366=CARTESIAN_POINT('Ctrl Pts',(0.00135155033166291,-0.0333141782228819,
-0.0148543219627419));
#32367=CARTESIAN_POINT('Ctrl Pts',(0.00137800965682989,-0.0333158172033075,
-0.014840805819731));
#32368=CARTESIAN_POINT('Ctrl Pts',(0.00152738606777894,-0.0333252451031987,
-0.0147616809253467));
#32369=CARTESIAN_POINT('Ctrl Pts',(0.00164580754532204,-0.0333333934480495,
-0.0146879688496514));
#32370=CARTESIAN_POINT('Ctrl Pts',(0.00185498249976198,-0.0333485631073666,
-0.0145366102096565));
#32371=CARTESIAN_POINT('Ctrl Pts',(0.00194707191897057,-0.0333555622518051,
-0.0144612517746332));
#32372=CARTESIAN_POINT('Ctrl Pts',(0.00209695039410642,-0.0333673462252851,
-0.0143229517386088));
#32373=CARTESIAN_POINT('Ctrl Pts',(0.00215697483423139,-0.0333721903951545,
-0.0142626436339962));
#32374=CARTESIAN_POINT('Ctrl Pts',(0.00225466401188813,-0.0333802691525081,
-0.0141557671987391));
#32375=CARTESIAN_POINT('Ctrl Pts',(0.00229364461872961,-0.0333835522967017,
-0.0141104757181992));
#32376=CARTESIAN_POINT('Ctrl Pts',(0.00234791883705563,-0.0333882133296866,
-0.0140434663717243));
#32377=CARTESIAN_POINT('Ctrl Pts',(0.00236431604857692,-0.0333896342497562,
-0.0140226643717949));
#32378=CARTESIAN_POINT('Ctrl Pts',(0.0023926595887327,-0.0333921138242862,
-0.013985710599464));
#32379=CARTESIAN_POINT('Ctrl Pts',(0.00240472301958964,-0.0333931769662321,
-0.0139696511084833));
#32380=CARTESIAN_POINT('Ctrl Pts',(0.00242958983414122,-0.0333953854682937,
-0.013935845336898));
#32381=CARTESIAN_POINT('Ctrl Pts',(0.00244236219473859,-0.0333965296130096,
-0.0139180776470631));
#32382=CARTESIAN_POINT('Ctrl Pts',(0.00247551106089169,-0.0333995263092527,
-0.0138708830792354));
#32383=CARTESIAN_POINT('Ctrl Pts',(0.00249555760827842,-0.0334013665769486,
-0.0138412281309592));
#32384=CARTESIAN_POINT('Ctrl Pts',(0.00259379487779923,-0.0334105408202969,
-0.0136901467714854));
#32385=CARTESIAN_POINT('Ctrl Pts',(0.00266367878286712,-0.0334175734428608,
-0.0135635411664959));
#32386=CARTESIAN_POINT('Ctrl Pts',(0.00279927504774821,-0.0334330493966487,
-0.0132695664113552));
#32387=CARTESIAN_POINT('Ctrl Pts',(0.00285962265991561,-0.0334413873851521,
-0.0131003539904685));
#32388=CARTESIAN_POINT('Ctrl Pts',(0.00292339910848192,-0.0334538454397706,
-0.0128536725389161));
#32389=CARTESIAN_POINT('Ctrl Pts',(0.00293953111900778,-0.033457612076349,
-0.0127798868024211));
#32390=CARTESIAN_POINT('Ctrl Pts',(0.00295636485685824,-0.0334625383779,
-0.0126860497290093));
#32391=CARTESIAN_POINT('Ctrl Pts',(0.00295967400567624,-0.0334635726975199,
-0.0126664889116386));
#32392=CARTESIAN_POINT('Ctrl Pts',(0.00296469589355574,-0.033465256872757,
-0.0126349020633047));
#32393=CARTESIAN_POINT('Ctrl Pts',(0.00296653006756486,-0.033465900280923,
-0.0126228956433011));
#32394=CARTESIAN_POINT('Ctrl Pts',(0.00296995666212803,-0.0334671600741279,
-0.0125995150956484));
#32395=CARTESIAN_POINT('Ctrl Pts',(0.00297155675805709,-0.0334677760411439,
-0.0125881424124412));
#32396=CARTESIAN_POINT('Ctrl Pts',(0.00297539876266702,-0.0334693267225163,
-0.0125596504977695));
#32397=CARTESIAN_POINT('Ctrl Pts',(0.00297755824133778,-0.0334702657784238,
-0.0125425206941243));
#32398=CARTESIAN_POINT('Ctrl Pts',(0.00298491514385364,-0.0334737261871321,
-0.0124798050174858));
#32399=CARTESIAN_POINT('Ctrl Pts',(0.00298921425821311,-0.0334762898220594,
-0.0124341220556221));
#32400=CARTESIAN_POINT('Ctrl Pts',(0.00300674610335933,-0.0334903128407513,
-0.0121872443109676));
#32401=CARTESIAN_POINT('Ctrl Pts',(0.0030007171964696,-0.033502352356114,
-0.0119852056927177));
#32402=CARTESIAN_POINT('Ctrl Pts',(0.00296081193949715,-0.0335202244195151,
-0.011681283651093));
#32403=CARTESIAN_POINT('Ctrl Pts',(0.00294170641447226,-0.0335262604735305,
-0.0115780467182088));
#32404=CARTESIAN_POINT('Ctrl Pts',(0.00290112723839275,-0.0335360270841346,
-0.0114088947946929));
#32405=CARTESIAN_POINT('Ctrl Pts',(0.0028827124027571,-0.0335398378952589,
-0.0113423457405591));
#32406=CARTESIAN_POINT('Ctrl Pts',(0.00285363918138549,-0.0335450908644545,
-0.0112498271658951));
#32407=CARTESIAN_POINT('Ctrl Pts',(0.00284488913388691,-0.0335465926810205,
-0.0112232847372945));
#32408=CARTESIAN_POINT('Ctrl Pts',(0.00282914100414081,-0.0335491654528002,
-0.0111776680614974));
#32409=CARTESIAN_POINT('Ctrl Pts',(0.00282231779646004,-0.0335502419624426,
-0.0111585358101415));
#32410=CARTESIAN_POINT('Ctrl Pts',(0.00280881402419867,-0.0335523015193921,
-0.0111218531205161));
#32411=CARTESIAN_POINT('Ctrl Pts',(0.00280216197203806,-0.0335532854343438,
-0.011104293266727));
#32412=CARTESIAN_POINT('Ctrl Pts',(0.0027841343290008,-0.0335558735425907,
-0.0110580206559875));
#32413=CARTESIAN_POINT('Ctrl Pts',(0.00277247933953992,-0.0335574685142712,
-0.011029418746871));
#32414=CARTESIAN_POINT('Ctrl Pts',(0.00272736382179645,-0.0335633667010298,
-0.0109234171679631));
#32415=CARTESIAN_POINT('Ctrl Pts',(0.00269108552334449,-0.0335675770946644,
-0.0108472563310091));
#32416=CARTESIAN_POINT('Ctrl Pts',(0.00253966399166702,-0.0335834446059485,
-0.0105610994439099));
#32417=CARTESIAN_POINT('Ctrl Pts',(0.00240276269478221,-0.0335944255477463,
-0.0103636596378104));
#32418=CARTESIAN_POINT('Ctrl Pts',(0.0022060431227533,-0.0336088396303959,
-0.0101419851959459));
#32419=CARTESIAN_POINT('Ctrl Pts',(0.0021670241508855,-0.0336116489773119,
-0.0101004614159256));
#32420=CARTESIAN_POINT('Ctrl Pts',(0.00210013203456061,-0.0336164329165445,
-0.0100332192825171));
#32421=CARTESIAN_POINT('Ctrl Pts',(0.00207291032358271,-0.0336183714553603,
-0.0100068725162208));
#32422=CARTESIAN_POINT('Ctrl Pts',(0.00203378756486346,-0.033621158348103,
-0.0099704165036299));
#32423=CARTESIAN_POINT('Ctrl Pts',(0.00202229436459781,-0.0336219771625735,
-0.0099598729741601));
#32424=CARTESIAN_POINT('Ctrl Pts',(0.00200232348771699,-0.033623401188328,
-0.00994183702763557));
#32425=CARTESIAN_POINT('Ctrl Pts',(0.00199388458581984,-0.0336240033210849,
-0.00993430198201933));
#32426=CARTESIAN_POINT('Ctrl Pts',(0.00197577171573472,-0.0336252968914373,
-0.00991831232699575));
#32427=CARTESIAN_POINT('Ctrl Pts',(0.00196608590752573,-0.0336259892557443,
-0.00990987198721579));
#32428=CARTESIAN_POINT('Ctrl Pts',(0.00193930637832258,-0.0336279045058861,
-0.00988683691036074));
#32429=CARTESIAN_POINT('Ctrl Pts',(0.00192210269609774,-0.0336291359892139,
-0.00987237192864144));
#32430=CARTESIAN_POINT('Ctrl Pts',(0.00180433424706328,-0.0336375638991048,
-0.00977558927594874));
#32431=CARTESIAN_POINT('Ctrl Pts',(0.00169868243732296,-0.0336451082024506,
-0.00969969465232878));
#32432=CARTESIAN_POINT('Ctrl Pts',(0.00143670790868342,-0.0336632129203722,
-0.00953618132325929));
#32433=CARTESIAN_POINT('Ctrl Pts',(0.00127678122121681,-0.0336737864989685,
-0.00945522166658635));
#32434=CARTESIAN_POINT('Ctrl Pts',(0.00105170143166814,-0.0336875887114654,
-0.00936552548481514));
#32435=CARTESIAN_POINT('Ctrl Pts',(0.000992083855422767,-0.0336911516953911,
-0.00934393015321076));
#32436=CARTESIAN_POINT('Ctrl Pts',(0.000886003690370446,-0.0336973235974966,
-0.00930926626875169));
#32437=CARTESIAN_POINT('Ctrl Pts',(0.000839827654198565,-0.0336999557687732,
-0.00929539958195612));
#32438=CARTESIAN_POINT('Ctrl Pts',(0.000769789795029305,-0.03370386807312,
-0.00927619472699345));
#32439=CARTESIAN_POINT('Ctrl Pts',(0.000746165595508288,-0.0337051742124621,
-0.00927002585839427));
#32440=CARTESIAN_POINT('Ctrl Pts',(0.000703177438411757,-0.0337075271116816,
-0.00925935940932528));
#32441=CARTESIAN_POINT('Ctrl Pts',(0.000683839249905239,-0.0337085768828414,
-0.00925476462794435));
#32442=CARTESIAN_POINT('Ctrl Pts',(0.000641900235454159,-0.0337108353247436,
-0.00924523916667989));
#32443=CARTESIAN_POINT('Ctrl Pts',(0.00061928507236787,-0.0337120417901303,
-0.00924037699300135));
#32444=CARTESIAN_POINT('Ctrl Pts',(0.00055680987881161,-0.0337153447562834,
-0.00922769920398575));
#32445=CARTESIAN_POINT('Ctrl Pts',(0.000516843203733572,-0.0337174242612458,
-0.00922043063716578));
#32446=CARTESIAN_POINT('Ctrl Pts',(0.000241871781243092,-0.0337315262754025,
-0.00917617159201931));
#32447=CARTESIAN_POINT('Ctrl Pts',(3.34695343856238E-6,-0.0337426496684483,
-0.00916643671368752));
#32448=CARTESIAN_POINT('Ctrl Pts',(-0.000333825716125148,-0.0337587366901328,
-0.00919279787667365));
#32449=CARTESIAN_POINT('Ctrl Pts',(-0.000433356153499485,-0.0337635446163017,
-0.00920562441907331));
#32450=CARTESIAN_POINT('Ctrl Pts',(-0.000586446892030909,-0.0337712629618868,
-0.00923321246590553));
#32451=CARTESIAN_POINT('Ctrl Pts',(-0.000640558066760292,-0.0337740552886763,
-0.00924451577164478));
#32452=CARTESIAN_POINT('Ctrl Pts',(-0.000711769609780924,-0.0337778511464565,
-0.00926145701357161));
#32453=CARTESIAN_POINT('Ctrl Pts',(-0.000729178299210887,-0.0337787887940389,
-0.00926576383929829));
#32454=CARTESIAN_POINT('Ctrl Pts',(-0.000757912779704372,-0.0337803540745094,
-0.00927314663084856));
#32455=CARTESIAN_POINT('Ctrl Pts',(-0.000769261276142269,-0.0337809768430059,
-0.00927613350812632));
#32456=CARTESIAN_POINT('Ctrl Pts',(-0.000790773216982359,-0.0337821665316029,
-0.00928193053228682));
#32457=CARTESIAN_POINT('Ctrl Pts',(-0.00080093991319622,-0.0337827326834863,
-0.00928472782455402));
#32458=CARTESIAN_POINT('Ctrl Pts',(-0.000828213949647178,-0.0337842615729003,
-0.00929238697802385));
#32459=CARTESIAN_POINT('Ctrl Pts',(-0.000845292902179561,-0.0337852296521758,
-0.00929734739321175));
#32460=CARTESIAN_POINT('Ctrl Pts',(-0.000909809334555627,-0.0337889245323163,
-0.00931670924097599));
#32461=CARTESIAN_POINT('Ctrl Pts',(-0.00095692933637723,-0.0337917010404217,
-0.00933213329153598));
#32462=CARTESIAN_POINT('Ctrl Pts',(-0.0011913284390104,-0.0338058334777848,
-0.00941534575192511));
#32463=CARTESIAN_POINT('Ctrl Pts',(-0.00137190836009119,-0.0338177236633955,
-0.00950049690718562));
#32464=CARTESIAN_POINT('Ctrl Pts',(-0.00163142865392247,-0.0338353566708339,
-0.00965610335911827));
#32465=CARTESIAN_POINT('Ctrl Pts',(-0.00171733566480339,-0.0338413037589557,
-0.0097138500123255));
#32466=CARTESIAN_POINT('Ctrl Pts',(-0.00185479268939082,-0.0338509470172707,
-0.00981695112819509));
#32467=CARTESIAN_POINT('Ctrl Pts',(-0.00190807610539897,-0.0338547208060546,
-0.00985983905829571));
#32468=CARTESIAN_POINT('Ctrl Pts',(-0.00198093519528966,-0.0338599326517222,
-0.00992270630495153));
#32469=CARTESIAN_POINT('Ctrl Pts',(-0.00200176617419573,-0.0338614291184264,
-0.00994119272548116));
#32470=CARTESIAN_POINT('Ctrl Pts',(-0.00203732798046824,-0.033863995664781,
-0.00997364834525282));
#32471=CARTESIAN_POINT('Ctrl Pts',(-0.00205217976855487,-0.0338650712272053,
-0.00998748171660667));
#32472=CARTESIAN_POINT('Ctrl Pts',(-0.00208051597644032,-0.033867130956198,
-0.0100144170309272));
#32473=CARTESIAN_POINT('Ctrl Pts',(-0.00209401981935827,-0.0338681159673373,
-0.0100274970701287));
#32474=CARTESIAN_POINT('Ctrl Pts',(-0.00212946847877434,-0.0338707115076103,
-0.0100624850143133));
#32475=CARTESIAN_POINT('Ctrl Pts',(-0.00215119840209031,-0.0338723127110495,
-0.0100846079680464));
#32476=CARTESIAN_POINT('Ctrl Pts',(-0.00223145296532613,-0.0338782701821735,
-0.0101688889773073));
#32477=CARTESIAN_POINT('Ctrl Pts',(-0.00228766076905602,-0.0338825310445765,
-0.0102332010149176));
#32478=CARTESIAN_POINT('Ctrl Pts',(-0.00249003748671433,-0.033898383086564,
-0.0104857424734329));
#32479=CARTESIAN_POINT('Ctrl Pts',(-0.00261633580989301,-0.0339093124469644,
-0.0106887287250801));
#32480=CARTESIAN_POINT('Ctrl Pts',(-0.00274139680927863,-0.0339236659461116,
-0.0109560259422959));
#32481=CARTESIAN_POINT('Ctrl Pts',(-0.00276402999804866,-0.0339264709775133,
-0.0110082177245521));
#32482=CARTESIAN_POINT('Ctrl Pts',(-0.00279922615419709,-0.0339312483159769,
-0.0110961474561313));
#32483=CARTESIAN_POINT('Ctrl Pts',(-0.0028126208690476,-0.0339331846975033,
-0.0111315375564136));
#32484=CARTESIAN_POINT('Ctrl Pts',(-0.00283058386373906,-0.0339359690065269,
-0.0111818522620625));
#32485=CARTESIAN_POINT('Ctrl Pts',(-0.0028357109981554,-0.0339367874682492,
-0.0111965748987347));
#32486=CARTESIAN_POINT('Ctrl Pts',(-0.00284436007607873,-0.0339382110910635,
-0.0112220484163447));
#32487=CARTESIAN_POINT('Ctrl Pts',(-0.00284793642681659,-0.033938813178737,
-0.0112327806067025));
#32488=CARTESIAN_POINT('Ctrl Pts',(-0.00285544579098707,-0.0339401069030581,
-0.011255747594637));
#32489=CARTESIAN_POINT('Ctrl Pts',(-0.0028593609577176,-0.0339407994694376,
-0.0112679876296553));
#32490=CARTESIAN_POINT('Ctrl Pts',(-0.00286991213315692,-0.0339427158115958,
-0.011301719274122));
#32491=CARTESIAN_POINT('Ctrl Pts',(-0.00287638514432946,-0.0339439482001548,
-0.0113232605548196));
#32492=CARTESIAN_POINT('Ctrl Pts',(-0.00291998431332457,-0.0339526509141746,
-0.0114745029682231));
#32493=CARTESIAN_POINT('Ctrl Pts',(-0.00294856360960901,-0.0339604960759037,
-0.0116064965794291));
#32494=CARTESIAN_POINT('Ctrl Pts',(-0.00299285361193743,-0.0339783784021183,
-0.0119080783278752));
#32495=CARTESIAN_POINT('Ctrl Pts',(-0.00300321674425717,-0.0339884119842963,
-0.0120780118217047));
#32496=CARTESIAN_POINT('Ctrl Pts',(-0.00299756163315046,-0.0340018445421147,
-0.0123133716365926));
#32497=CARTESIAN_POINT('Ctrl Pts',(-0.00299384633835027,-0.0340055299811987,
-0.0123787620566068));
#32498=CARTESIAN_POINT('Ctrl Pts',(-0.00298358001203221,-0.0340118886751861,
-0.0124931688365766));
#32499=CARTESIAN_POINT('Ctrl Pts',(-0.00297795217245256,-0.0340145872062452,
-0.0125422411890859));
#32500=CARTESIAN_POINT('Ctrl Pts',(-0.00296770404967998,-0.0340185768175463,
-0.0126155575365401));
#32501=CARTESIAN_POINT('Ctrl Pts',(-0.00296399238586176,-0.0340198954622457,
-0.0126399183029434));
#32502=CARTESIAN_POINT('Ctrl Pts',(-0.00295674317914521,-0.0340222616794114,
-0.0126838546037975));
#32503=CARTESIAN_POINT('Ctrl Pts',(-0.00295331030968823,-0.0340233124237095,
-0.0127034457484575));
#32504=CARTESIAN_POINT('Ctrl Pts',(-0.00294549598158082,-0.0340255629870533,
-0.0127455728784517));
#32505=CARTESIAN_POINT('Ctrl Pts',(-0.00294105014067019,-0.0340267607318689,
-0.0127680957192668));
#32506=CARTESIAN_POINT('Ctrl Pts',(-0.0029281874507338,-0.0340300144000641,
-0.0128295379599495));
#32507=CARTESIAN_POINT('Ctrl Pts',(-0.00291925347711313,-0.0340320541772108,
-0.0128683449632596));
#32508=CARTESIAN_POINT('Ctrl Pts',(-0.00285012500560406,-0.0340464281526899,
-0.0131434506976239));
#32509=CARTESIAN_POINT('Ctrl Pts',(-0.002762094528966,-0.0340578070819802,
-0.0133718038516003));
#32510=CARTESIAN_POINT('Ctrl Pts',(-0.00260169779295154,-0.0340740405498672,
-0.0136727183546661));
#32511=CARTESIAN_POINT('Ctrl Pts',(-0.00255186997835265,-0.0340787050510572,
-0.0137561678377765));
#32512=CARTESIAN_POINT('Ctrl Pts',(-0.00246807827385146,-0.0340862200455918,
-0.0138821727938511));
#32513=CARTESIAN_POINT('Ctrl Pts',(-0.00243685568229249,-0.0340889597593756,
-0.0139264732776887));
#32514=CARTESIAN_POINT('Ctrl Pts',(-0.00239380159778495,-0.0340926940815064,
-0.0139841760222617));
#32515=CARTESIAN_POINT('Ctrl Pts',(-0.00238302410811179,-0.034093625465097,
-0.0139983552142524));
#32516=CARTESIAN_POINT('Ctrl Pts',(-0.00236495278188501,-0.03409518310916,
-0.0140216960348236));
#32517=CARTESIAN_POINT('Ctrl Pts',(-0.00235773023633278,-0.0340958046034524,
-0.0140309126491647));
#32518=CARTESIAN_POINT('Ctrl Pts',(-0.00234388749453897,-0.0340969942700964,
-0.0140483657900979));
#32519=CARTESIAN_POINT('Ctrl Pts',(-0.00233727740221758,-0.0340975617001701,
-0.0140566100494666));
#32520=CARTESIAN_POINT('Ctrl Pts',(-0.00231934997860591,-0.0340990984959883,
-0.0140787290754456));
#32521=CARTESIAN_POINT('Ctrl Pts',(-0.00230795192820077,-0.0341000732985576,
-0.0140925375217369));
#32522=CARTESIAN_POINT('Ctrl Pts',(-0.00226395465425984,-0.034103824766328,
-0.0141448775882746));
#32523=CARTESIAN_POINT('Ctrl Pts',(-0.00223050998484804,-0.034106653025306,
-0.0141826846258763));
#32524=CARTESIAN_POINT('Ctrl Pts',(-0.00206084248745236,-0.034120812824986,
-0.0143650001362215));
#32525=CARTESIAN_POINT('Ctrl Pts',(-0.00191145882869984,-0.034132667946825,
-0.0144965773114821));
#32526=CARTESIAN_POINT('Ctrl Pts',(-0.00166645299184769,-0.0341502440525831,
-0.0146725630220531));
#32527=CARTESIAN_POINT('Ctrl Pts',(-0.00157968542853716,-0.0341561695176447,
-0.0147283465301897));
#32528=CARTESIAN_POINT('Ctrl Pts',(-0.00143100652823459,-0.0341657827333614,
-0.0148134419433172));
#32529=CARTESIAN_POINT('Ctrl Pts',(-0.0013706592051858,-0.03416954746851,
-0.0148453004125789));
#32530=CARTESIAN_POINT('Ctrl Pts',(-0.00128423907191374,-0.0341747492485911,
-0.0148872190408566));
#32531=CARTESIAN_POINT('Ctrl Pts',(-0.00125903523533144,-0.0341762443998648,
-0.0148990140592912));
#32532=CARTESIAN_POINT('Ctrl Pts',(-0.001215174019169,-0.0341788094166759,
-0.0149188013074119));
#32533=CARTESIAN_POINT('Ctrl Pts',(-0.00119659320688423,-0.034179884747394,
-0.0149269578767765));
#32534=CARTESIAN_POINT('Ctrl Pts',(-0.00116063602620518,-0.0341819445240121,
-0.0149423090770054));
#32535=CARTESIAN_POINT('Ctrl Pts',(-0.00114327200410095,-0.0341829298087768,
-0.0149495300470402));
#32536=CARTESIAN_POINT('Ctrl Pts',(-0.00109707117346208,-0.0341855271998249,
-0.014968235462984));
#32537=CARTESIAN_POINT('Ctrl Pts',(-0.00106812170071878,-0.0341871299544445,
-0.014979436619136));
#32538=CARTESIAN_POINT('Ctrl Pts',(-0.000958664249872616,-0.0341931025270523,
-0.0150198464034051));
#32539=CARTESIAN_POINT('Ctrl Pts',(-0.000877088902219408,-0.0341973762735131,
-0.0150460537379515));
#32540=CARTESIAN_POINT('Ctrl Pts',(-0.000565047458946579,-0.0342132244841497,
-0.0151317525531442));
#32541=CARTESIAN_POINT('Ctrl Pts',(-0.000328931019634678,-0.0342241407562824,
-0.0151672433965715));
#32542=CARTESIAN_POINT('Ctrl Pts',(-3.42820793670757E-5,-0.0342384788764484,
-0.0151761961482578));
#32543=CARTESIAN_POINT('Ctrl Pts',(2.25823401362681E-5,-0.0342412828056937,
-0.0151763069201371));
#32544=CARTESIAN_POINT('Ctrl Pts',(0.000117226831195046,-0.034246058458155,
-0.0151738007129355));
#32545=CARTESIAN_POINT('Ctrl Pts',(0.000155016910013541,-0.0342479942884883,
-0.0151720843213275));
#32546=CARTESIAN_POINT('Ctrl Pts',(0.000208318725397031,-0.0342507779373783,
-0.0151686523609703));
#32547=CARTESIAN_POINT('Ctrl Pts',(0.000223866317502566,-0.0342515963089763,
-0.0151675295462171));
#32548=CARTESIAN_POINT('Ctrl Pts',(0.000250680309804121,-0.0342530198289133,
-0.015165382906679));
#32549=CARTESIAN_POINT('Ctrl Pts',(0.000261951093202847,-0.03425362190514,
-0.0151644164178833));
#32550=CARTESIAN_POINT('Ctrl Pts',(0.000286014821568249,-0.0342549156690621,
-0.0151622157386412));
#32551=CARTESIAN_POINT('Ctrl Pts',(0.000298805506103946,-0.0342556082872627,
-0.0151609630719462));
#32552=CARTESIAN_POINT('Ctrl Pts',(0.000333962716912195,-0.0342575249093787,
-0.015157291700008));
#32553=CARTESIAN_POINT('Ctrl Pts',(0.000356310289424819,-0.0342587575299941,
-0.0151547035728422));
#32554=CARTESIAN_POINT('Ctrl Pts',(0.000513576010346341,-0.0342675228920418,
-0.0151346952853522));
#32555=CARTESIAN_POINT('Ctrl Pts',(0.00064719097540904,-0.0342754367332917,
-0.0151083682128113));
#32556=CARTESIAN_POINT('Ctrl Pts',(0.000946840011479498,-0.0342936420926783,
-0.0150278459720689));
#32557=CARTESIAN_POINT('Ctrl Pts',(0.00111088790677592,-0.0343039287943268,
-0.014968039696976));
#32558=CARTESIAN_POINT('Ctrl Pts',(0.00132555183636874,-0.0343174151433276,
-0.0148678472916823));
#32559=CARTESIAN_POINT('Ctrl Pts',(0.00138144153916055,-0.0343209321186503,
-0.0148395986568057));
#32560=CARTESIAN_POINT('Ctrl Pts',(0.00147833552793655,-0.0343270335771446,
-0.0147867544238806));
#32561=CARTESIAN_POINT('Ctrl Pts',(0.00151971153156067,-0.0343296405749895,
-0.0147628897950129));
#32562=CARTESIAN_POINT('Ctrl Pts',(0.00158127995482397,-0.0343335234940839,
-0.014725391594343));
#32563=CARTESIAN_POINT('Ctrl Pts',(0.00160190379290108,-0.0343348248410766,
-0.0147124841552056));
#32564=CARTESIAN_POINT('Ctrl Pts',(0.00163908390228504,-0.0343371726784623,
-0.0146885806576091));
#32565=CARTESIAN_POINT('Ctrl Pts',(0.00165569211696096,-0.03433822211851,
-0.0146776683315079));
#32566=CARTESIAN_POINT('Ctrl Pts',(0.00169145340477964,-0.0343404837883751,
-0.014653659505954));
#32567=CARTESIAN_POINT('Ctrl Pts',(0.00171056552600858,-0.0343416937605292,
-0.0146405041547294));
#32568=CARTESIAN_POINT('Ctrl Pts',(0.00176297504096698,-0.0343450166098808,
-0.0146035260553021));
#32569=CARTESIAN_POINT('Ctrl Pts',(0.00179594090345443,-0.0343471121430334,
-0.0145792410083115));
#32570=CARTESIAN_POINT('Ctrl Pts',(0.002015006397015,-0.0343610985681317,
-0.0144108363731809));
#32571=CARTESIAN_POINT('Ctrl Pts',(0.00218407892212733,-0.0343721134321571,
-0.014245927362271));
#32572=CARTESIAN_POINT('Ctrl Pts',(0.00239609404274169,-0.0343881404002779,
-0.0139839099219335));
#32573=CARTESIAN_POINT('Ctrl Pts',(0.00245598149570972,-0.0343930104480621,
-0.0139016829958145));
#32574=CARTESIAN_POINT('Ctrl Pts',(0.00254205699614042,-0.0344008165638233,
-0.0137699211504468));
#32575=CARTESIAN_POINT('Ctrl Pts',(0.00257122983607939,-0.0344036313082395,
-0.0137224245093847));
#32576=CARTESIAN_POINT('Ctrl Pts',(0.00260804371731996,-0.0344074533653778,
-0.0136585641292623));
#32577=CARTESIAN_POINT('Ctrl Pts',(0.00261688566483034,-0.0344083936449175,
-0.0136429023181759));
#32578=CARTESIAN_POINT('Ctrl Pts',(0.00263126831706156,-0.0344099621380394,
-0.0136168824354636));
#32579=CARTESIAN_POINT('Ctrl Pts',(0.00263689009826553,-0.0344105854458042,
-0.0136065693895787));
#32580=CARTESIAN_POINT('Ctrl Pts',(0.00264743917073649,-0.0344117751624809,
-0.0135869439400167));
#32581=CARTESIAN_POINT('Ctrl Pts',(0.00265237824260972,-0.0344123407924217,
-0.0135776380940047));
#32582=CARTESIAN_POINT('Ctrl Pts',(0.00266550002957876,-0.0344138664384547,
-0.0135525973212715));
#32583=CARTESIAN_POINT('Ctrl Pts',(0.00267359227826778,-0.0344148317573992,
-0.0135368157563903));
#32584=CARTESIAN_POINT('Ctrl Pts',(0.00270360905272258,-0.0344185036667659,
-0.0134769758389944));
#32585=CARTESIAN_POINT('Ctrl Pts',(0.00272458732103992,-0.0344212592091826,
-0.0134324539443992));
#32586=CARTESIAN_POINT('Ctrl Pts',(0.00284647516087281,-0.0344384026480205,
-0.0131563559827071));
#32587=CARTESIAN_POINT('Ctrl Pts',(0.00291889953234112,-0.034453623836841,
-0.0129133122837938));
#32588=CARTESIAN_POINT('Ctrl Pts',(0.00297765692132849,-0.0344743274315713,
-0.0125570596108822));
#32589=CARTESIAN_POINT('Ctrl Pts',(0.00298949077105853,-0.0344804115792897,
-0.0124491805486363));
#32590=CARTESIAN_POINT('Ctrl Pts',(0.00299724546138588,-0.0344880908989193,
-0.0123084293409625));
#32591=CARTESIAN_POINT('Ctrl Pts',(0.00299850611955335,-0.0344898458974053,
-0.0122759428935426));
#32592=CARTESIAN_POINT('Ctrl Pts',(0.00299971598216001,-0.0344927183440224,
-0.0122222550161421));
#32593=CARTESIAN_POINT('Ctrl Pts',(0.00299996892616627,-0.0344938449683844,
-0.0122010637404368));
#32594=CARTESIAN_POINT('Ctrl Pts',(0.00300002461319226,-0.0344960419371712,
-0.0121594846018045));
#32595=CARTESIAN_POINT('Ctrl Pts',(0.00299984411022637,-0.0344971127343431,
-0.0121390979436702));
#32596=CARTESIAN_POINT('Ctrl Pts',(0.00299891529576274,-0.0344996590735799,
-0.0120903406682142));
#32597=CARTESIAN_POINT('Ctrl Pts',(0.00299797219369084,-0.0345011285952758,
-0.0120619754773406));
#32598=CARTESIAN_POINT('Ctrl Pts',(0.00299321271817669,-0.0345062854345003,
-0.0119616958334017));
#32599=CARTESIAN_POINT('Ctrl Pts',(0.00298720971645073,-0.0345099065214422,
-0.0118899076669784));
#32600=CARTESIAN_POINT('Ctrl Pts',(0.00296529790018503,-0.0345189959594432,
-0.0117073176237771));
#32601=CARTESIAN_POINT('Ctrl Pts',(0.00294576314498241,-0.0345243675747273,
-0.0115970624596732));
#32602=CARTESIAN_POINT('Ctrl Pts',(0.00288173866082887,-0.0345376533955076,
-0.0113252019220437));
#32603=CARTESIAN_POINT('Ctrl Pts',(0.00282979326742278,-0.0345454756227368,
-0.0111657595648701));
#32604=CARTESIAN_POINT('Ctrl Pts',(0.00273982593493822,-0.0345568871223864,
-0.0109521282819776));
#32605=CARTESIAN_POINT('Ctrl Pts',(0.00271292201820517,-0.0345601190442526,
-0.0108935888341284));
#32606=CARTESIAN_POINT('Ctrl Pts',(0.00267545318480082,-0.0345644567784832,
-0.0108185287065842));
#32607=CARTESIAN_POINT('Ctrl Pts',(0.00266658006343966,-0.0345654732865576,
-0.0108011786027092));
#32608=CARTESIAN_POINT('Ctrl Pts',(0.00265193889398139,-0.0345671354871448,
-0.0107732251215521));
#32609=CARTESIAN_POINT('Ctrl Pts',(0.00264627464727293,-0.0345677750349074,
-0.0107625677004703));
#32610=CARTESIAN_POINT('Ctrl Pts',(0.0026350039720529,-0.0345690413360245,
-0.0107416669590874));
#32611=CARTESIAN_POINT('Ctrl Pts',(0.00262940177935275,-0.0345696678410616,
-0.0107314216945453));
#32612=CARTESIAN_POINT('Ctrl Pts',(0.00261518123589728,-0.0345712504016995,
-0.0107057721071383));
#32613=CARTESIAN_POINT('Ctrl Pts',(0.00260648654243604,-0.0345722110228962,
-0.0106904107783884));
#32614=CARTESIAN_POINT('Ctrl Pts',(0.00257122949402419,-0.0345760761453026,
-0.0106293831634086));
#32615=CARTESIAN_POINT('Ctrl Pts',(0.00254359972078884,-0.0345790382761807,
-0.0105843474669341));
#32616=CARTESIAN_POINT('Ctrl Pts',(0.0024639394286114,-0.0345873529935348,
-0.0104618806600705));
#32617=CARTESIAN_POINT('Ctrl Pts',(0.00240946536699408,-0.0345927937015789,
-0.0103861117755327));
#32618=CARTESIAN_POINT('Ctrl Pts',(0.00220654767787301,-0.0346119681278612,
-0.0101299597176363));
#32619=CARTESIAN_POINT('Ctrl Pts',(0.00204064041593849,-0.0346257273955933,
-0.009964439755018));
#32620=CARTESIAN_POINT('Ctrl Pts',(0.00181808388552439,-0.0346414203239254,
-0.00978900365582104));
#32621=CARTESIAN_POINT('Ctrl Pts',(0.00177820983410336,-0.0346441422964082,
-0.00975915091342264));
#32622=CARTESIAN_POINT('Ctrl Pts',(0.00171745851345907,-0.0346481591624086,
-0.00971598595232774));
#32623=CARTESIAN_POINT('Ctrl Pts',(0.00169713111366653,-0.0346494821804487,
-0.00970191774174177));
#32624=CARTESIAN_POINT('Ctrl Pts',(0.00166013453096633,-0.0346518530905548,
-0.00967698371915239));
#32625=CARTESIAN_POINT('Ctrl Pts',(0.00164352688581077,-0.0346529042105308,
-0.00966602955233309));
#32626=CARTESIAN_POINT('Ctrl Pts',(0.00160757221629099,-0.0346551521949152,
-0.00964282429162535));
#32627=CARTESIAN_POINT('Ctrl Pts',(0.00158819133633765,-0.0346563470292288,
-0.00963062782762439));
#32628=CARTESIAN_POINT('Ctrl Pts',(0.00153403817337389,-0.0346596402926559,
-0.00959740844662663));
#32629=CARTESIAN_POINT('Ctrl Pts',(0.00149897498055441,-0.0346617215321998,
-0.00957686788523866));
#32630=CARTESIAN_POINT('Ctrl Pts',(0.00134975892204702,-0.0346703805985349,
-0.00949347943719754));
#32631=CARTESIAN_POINT('Ctrl Pts',(0.00123198693284768,-0.0346767289236711,
-0.00943738819676805));
#32632=CARTESIAN_POINT('Ctrl Pts',(0.00102720088399999,-0.0346872818427046,
-0.00935574979752547));
#32633=CARTESIAN_POINT('Ctrl Pts',(0.000942005841697467,-0.0346915407991256,
-0.00932616021978938));
#32634=CARTESIAN_POINT('Ctrl Pts',(0.000708750964245328,-0.0347030886555901,
-0.0092567526449807));
#32635=CARTESIAN_POINT('Ctrl Pts',(0.000558775451297078,-0.0347103902258542,
-0.00922437269920118));
#32636=CARTESIAN_POINT('Ctrl Pts',(0.000377694610717754,-0.0347196991481665,
-0.00919957680386364));
#32637=CARTESIAN_POINT('Ctrl Pts',(0.000348332311057776,-0.0347212240978858,
-0.00919599768639593));
#32638=CARTESIAN_POINT('Ctrl Pts',(0.000304848400077032,-0.0347235115019578,
-0.00919134866932447));
#32639=CARTESIAN_POINT('Ctrl Pts',(0.000290763648035617,-0.0347242569003196,
-0.0091899435687827));
#32640=CARTESIAN_POINT('Ctrl Pts',(0.000265531238535391,-0.0347256011157826,
-0.00918760659456845));
#32641=CARTESIAN_POINT('Ctrl Pts',(0.000254387584534166,-0.0347261979114213,
-0.00918663732241465));
#32642=CARTESIAN_POINT('Ctrl Pts',(0.000229431710881271,-0.0347275415210618,
-0.00918460722840893));
#32643=CARTESIAN_POINT('Ctrl Pts',(0.000215617521548614,-0.0347282900522575,
-0.00918357974293981));
#32644=CARTESIAN_POINT('Ctrl Pts',(0.000173855539317694,-0.0347305663830886,
-0.00918076421870998));
#32645=CARTESIAN_POINT('Ctrl Pts',(0.000145890049198672,-0.0347321088562114,
-0.00917927185825855));
#32646=CARTESIAN_POINT('Ctrl Pts',(6.24895452250378E-6,-0.0347398879023014,
-0.00917377931081361));
#32647=CARTESIAN_POINT('Ctrl Pts',(-0.000105561046078815,-0.0347463590294455,
-0.00917562991509687));
#32648=CARTESIAN_POINT('Ctrl Pts',(-0.000475559634842973,-0.0347680737263861,
-0.00920246313494406));
#32649=CARTESIAN_POINT('Ctrl Pts',(-0.000730653026213323,-0.0347834157303929,
-0.00925465585206034));
#32650=CARTESIAN_POINT('Ctrl Pts',(-0.00101312983671242,-0.0347998730326235,
-0.00935182773343107));
#32651=CARTESIAN_POINT('Ctrl Pts',(-0.00105013240568794,-0.0348020209309889,
-0.00936537743360993));
#32652=CARTESIAN_POINT('Ctrl Pts',(-0.00111006271315644,-0.0348054876307774,
-0.00938867181549161));
#32653=CARTESIAN_POINT('Ctrl Pts',(-0.00113315415373076,-0.0348068204060212,
-0.00939797973037137));
#32654=CARTESIAN_POINT('Ctrl Pts',(-0.00117449703184685,-0.034809201847736,
-0.0094152459229905));
#32655=CARTESIAN_POINT('Ctrl Pts',(-0.00119278999264321,-0.034810253867157,
-0.00942310041850815));
#32656=CARTESIAN_POINT('Ctrl Pts',(-0.00123183874922494,-0.0348124964043728,
-0.00944032922346036));
#32657=CARTESIAN_POINT('Ctrl Pts',(-0.00125256879173167,-0.0348136849875685,
-0.00944975899928105));
#32658=CARTESIAN_POINT('Ctrl Pts',(-0.00130943538444792,-0.0348169414264154,
-0.00947641236007226));
#32659=CARTESIAN_POINT('Ctrl Pts',(-0.00134533828458003,-0.0348189927399427,
-0.00949412484542092));
#32660=CARTESIAN_POINT('Ctrl Pts',(-0.00153121340017156,-0.0348296051922691,
-0.00959049794414904));
#32661=CARTESIAN_POINT('Ctrl Pts',(-0.00167468894013557,-0.0348377480243278,
-0.00968103847350597));
#32662=CARTESIAN_POINT('Ctrl Pts',(-0.00195526993133758,-0.0348544604459651,
-0.00989326612709907));
#32663=CARTESIAN_POINT('Ctrl Pts',(-0.00209042051034744,-0.0348629835393922,
-0.0100163588671412));
#32664=CARTESIAN_POINT('Ctrl Pts',(-0.00224403055794431,-0.0348743685349453,
-0.010184279248007));
#32665=CARTESIAN_POINT('Ctrl Pts',(-0.00227376053086639,-0.03487666475848,
-0.0102182902741463));
#32666=CARTESIAN_POINT('Ctrl Pts',(-0.00231370946432668,-0.0348799018090744,
-0.0102661300046118));
#32667=CARTESIAN_POINT('Ctrl Pts',(-0.00232459557282121,-0.0348808001937584,
-0.0102793960908996));
#32668=CARTESIAN_POINT('Ctrl Pts',(-0.00234256336751784,-0.0348823118105403,
-0.010301679253244));
#32669=CARTESIAN_POINT('Ctrl Pts',(-0.0023497084346415,-0.0348829207146633,
-0.0103106450658337));
#32670=CARTESIAN_POINT('Ctrl Pts',(-0.00236433667522902,-0.0348841840047522,
-0.010329218405693));
#32671=CARTESIAN_POINT('Ctrl Pts',(-0.00237181299642614,-0.0348848388036065,
-0.0103388308597318));
#32672=CARTESIAN_POINT('Ctrl Pts',(-0.00239140383310954,-0.0348865783659193,
-0.0103643381437399));
#32673=CARTESIAN_POINT('Ctrl Pts',(-0.00240341820997934,-0.0348876695771154,
-0.0103803087253376));
#32674=CARTESIAN_POINT('Ctrl Pts',(-0.00246119335319745,-0.034893032644773,
-0.0104587274714324));
#32675=CARTESIAN_POINT('Ctrl Pts',(-0.00250468172916291,-0.034897429775811,
-0.0105228071672573));
#32676=CARTESIAN_POINT('Ctrl Pts',(-0.00264612979829027,-0.0349128589598591,
-0.0107496463854092));
#32677=CARTESIAN_POINT('Ctrl Pts',(-0.0027310901716194,-0.0349241816136645,
-0.0109199794702632));
#32678=CARTESIAN_POINT('Ctrl Pts',(-0.00284710874499847,-0.034942869468628,
-0.0112210787534907));
#32679=CARTESIAN_POINT('Ctrl Pts',(-0.00288656839361039,-0.0349503877135219,
-0.0113479931833876));
#32680=CARTESIAN_POINT('Ctrl Pts',(-0.00292569159968663,-0.0349595656926304,
-0.0115113477665344));
#32681=CARTESIAN_POINT('Ctrl Pts',(-0.00293328687454053,-0.0349614703302367,
-0.0115457206204964));
#32682=CARTESIAN_POINT('Ctrl Pts',(-0.00294459517957993,-0.0349645216583975,
-0.0116015427964108));
#32683=CARTESIAN_POINT('Ctrl Pts',(-0.00294868265409088,-0.0349656799091502,
-0.0116229121054753));
#32684=CARTESIAN_POINT('Ctrl Pts',(-0.00295610318756234,-0.034967895696436,
-0.0116641316930658));
#32685=CARTESIAN_POINT('Ctrl Pts',(-0.00295946963592129,-0.0349689542178807,
-0.0116839746989232));
#32686=CARTESIAN_POINT('Ctrl Pts',(-0.00296684851618281,-0.0349714065677787,
-0.0117302899625403));
#32687=CARTESIAN_POINT('Ctrl Pts',(-0.00297070678939083,-0.0349727955649953,
-0.0117567852434946));
#32688=CARTESIAN_POINT('Ctrl Pts',(-0.00298225423626283,-0.0349773394749354,
-0.011844281862726));
#32689=CARTESIAN_POINT('Ctrl Pts',(-0.00298842321182215,-0.0349804480173611,
-0.0119054696907493));
#32690=CARTESIAN_POINT('Ctrl Pts',(-0.00299888051881708,-0.0349879193123658,
-0.012055176314337));
#32691=CARTESIAN_POINT('Ctrl Pts',(-0.00300113642909699,-0.0349922263284735,
-0.0121437792915847));
#32692=CARTESIAN_POINT('Ctrl Pts',(-0.0029972755540795,-0.0350020639478382,
-0.0123487355071376));
#32693=CARTESIAN_POINT('Ctrl Pts',(-0.00298831174534155,-0.0350075441243131,
-0.0124648899098138));
#32694=CARTESIAN_POINT('Ctrl Pts',(-0.00295282137540481,-0.0350200664070991,
-0.0127257845928377));
#32695=CARTESIAN_POINT('Ctrl Pts',(-0.00292235874664381,-0.035027124061726,
-0.012869675384374));
#32696=CARTESIAN_POINT('Ctrl Pts',(-0.00287518126323332,-0.0350358393843081,
-0.0130325014184055));
#32697=CARTESIAN_POINT('Ctrl Pts',(-0.00286862991324815,-0.0350370157495548,
-0.0130541901699344));
#32698=CARTESIAN_POINT('Ctrl Pts',(-0.00285796762736313,-0.035038882049868,
-0.0130880962008863));
#32699=CARTESIAN_POINT('Ctrl Pts',(-0.00285402241401679,-0.0350395630211296,
-0.0131003651264354));
#32700=CARTESIAN_POINT('Ctrl Pts',(-0.0028464688720019,-0.0350408498287807,
-0.0131233461494037));
#32701=CARTESIAN_POINT('Ctrl Pts',(-0.00284287889529581,-0.0350414546464236,
-0.0131340637730616));
#32702=CARTESIAN_POINT('Ctrl Pts',(-0.00283421583975468,-0.0350428981197999,
-0.0131594494742046));
#32703=CARTESIAN_POINT('Ctrl Pts',(-0.00282908938235331,-0.0350437397429562,
-0.0131740988138366));
#32704=CARTESIAN_POINT('Ctrl Pts',(-0.00281122113107034,-0.0350466297114517,
-0.0132239157160189));
#32705=CARTESIAN_POINT('Ctrl Pts',(-0.00279793583624809,-0.0350487059158552,
-0.0132588832549685));
#32706=CARTESIAN_POINT('Ctrl Pts',(-0.00276314855281294,-0.0350539544321809,
-0.0133455294954337));
#32707=CARTESIAN_POINT('Ctrl Pts',(-0.00274084780511743,-0.0350571581687624,
-0.0133968713414091));
#32708=CARTESIAN_POINT('Ctrl Pts',(-0.00262084172779812,-0.0350735378706403,
-0.0136532766472321));
#32709=CARTESIAN_POINT('Ctrl Pts',(-0.00250149268052828,-0.0350871224767957,
-0.0138474215552333));
#32710=CARTESIAN_POINT('Ctrl Pts',(-0.00230244058815474,-0.035105529532247,
-0.0141014434232573));
#32711=CARTESIAN_POINT('Ctrl Pts',(-0.00223994197591191,-0.0351108694527583,
-0.0141738003970405));
#32712=CARTESIAN_POINT('Ctrl Pts',(-0.00215196430840077,-0.035117821671529,
-0.0142663270946311));
#32713=CARTESIAN_POINT('Ctrl Pts',(-0.00212946479547153,-0.0351195546247943,
-0.0142892417790271));
#32714=CARTESIAN_POINT('Ctrl Pts',(-0.00209157116994248,-0.0351224007560056,
-0.0143266149368271));
#32715=CARTESIAN_POINT('Ctrl Pts',(-0.00207638494079759,-0.0351235227751405,
-0.0143412796287501));
#32716=CARTESIAN_POINT('Ctrl Pts',(-0.00204619363440947,-0.0351257176947062,
-0.0143698244192038));
#32717=CARTESIAN_POINT('Ctrl Pts',(-0.00203119901204034,-0.0351267909625586,
-0.014383713862132));
#32718=CARTESIAN_POINT('Ctrl Pts',(-0.00199483328704307,-0.0351293545215655,
-0.0144167151856495));
#32719=CARTESIAN_POINT('Ctrl Pts',(-0.00197332768640488,-0.0351308385725719,
-0.0144356762461259));
#32720=CARTESIAN_POINT('Ctrl Pts',(-0.00189529263666527,-0.0351361142235893,
-0.0145025146618048));
#32721=CARTESIAN_POINT('Ctrl Pts',(-0.00183726433942285,-0.0351398352890842,
-0.0145486044655414));
#32722=CARTESIAN_POINT('Ctrl Pts',(-0.00168342624038712,-0.0351492617776901,
-0.0146617614015495));
#32723=CARTESIAN_POINT('Ctrl Pts',(-0.00158529546913449,-0.0351548601216049,
-0.0147254617843674));
#32724=CARTESIAN_POINT('Ctrl Pts',(-0.00132710590219501,-0.0351689745289846,
-0.0148723786877163));
#32725=CARTESIAN_POINT('Ctrl Pts',(-0.00116282155333357,-0.0351773911406822,
-0.0149471878973429));
#32726=CARTESIAN_POINT('Ctrl Pts',(-0.000947635353302538,-0.0351887696077677,
-0.0150226552664496));
#32727=CARTESIAN_POINT('Ctrl Pts',(-0.000902064935518247,-0.0351911996397882,
-0.0150374215037975));
#32728=CARTESIAN_POINT('Ctrl Pts',(-0.000839339166156025,-0.0351945960922051,
-0.0150560994395986));
#32729=CARTESIAN_POINT('Ctrl Pts',(-0.000822472077934371,-0.0351955144467649,
-0.0150609612204881));
#32730=CARTESIAN_POINT('Ctrl Pts',(-0.000795447385743178,-0.0351969952819539,
-0.0150684945966033));
#32731=CARTESIAN_POINT('Ctrl Pts',(-0.000785316496457693,-0.0351975525183222,
-0.0150712614245921));
#32732=CARTESIAN_POINT('Ctrl Pts',(-0.000763784453527056,-0.0351987417253721,
-0.0150770206806381));
#32733=CARTESIAN_POINT('Ctrl Pts',(-0.000752379845245758,-0.0351993744924799,
-0.0150799992018155));
#32734=CARTESIAN_POINT('Ctrl Pts',(-0.000723339335479696,-0.0352009925808031,
-0.0150874011218788));
#32735=CARTESIAN_POINT('Ctrl Pts',(-0.000705680422636967,-0.0352019828778839,
-0.0150917314905322));
#32736=CARTESIAN_POINT('Ctrl Pts',(-0.000631995950186454,-0.0352061383741216,
-0.0151090920681379));
#32737=CARTESIAN_POINT('Ctrl Pts',(-0.000575643687420339,-0.0352093722179058,
-0.015120669439084));
#32738=CARTESIAN_POINT('Ctrl Pts',(-0.000413507845707785,-0.0352187704930593,
-0.0151491481895211));
#32739=CARTESIAN_POINT('Ctrl Pts',(-0.00030710634564027,-0.0352250488796188,
-0.0151620138722155));
#32740=CARTESIAN_POINT('Ctrl Pts',(2.49417841265192E-5,-0.0352446067499424,
-0.0151842276432674));
#32741=CARTESIAN_POINT('Ctrl Pts',(0.000251149750532565,-0.0352578146674948,
-0.0151738344723821));
#32742=CARTESIAN_POINT('Ctrl Pts',(0.000511947896089953,-0.0352723503420026,
-0.0151320976305147));
#32743=CARTESIAN_POINT('Ctrl Pts',(0.000549704449373298,-0.0352744396976675,
-0.015125310265623));
#32744=CARTESIAN_POINT('Ctrl Pts',(0.000611436566119944,-0.0352778319502788,
-0.0151129862474772));
#32745=CARTESIAN_POINT('Ctrl Pts',(0.000635491811659911,-0.0352791478363707,
-0.0151078756109039));
#32746=CARTESIAN_POINT('Ctrl Pts',(0.00067888125731334,-0.0352815111025249,
-0.0150980982590127));
#32747=CARTESIAN_POINT('Ctrl Pts',(0.000698236873399678,-0.0352825616190308,
-0.0150935339981171));
#32748=CARTESIAN_POINT('Ctrl Pts',(0.000739872340052679,-0.035284813854923,
-0.015083277856986));
#32749=CARTESIAN_POINT('Ctrl Pts',(0.000762135105975031,-0.0352860134717941,
-0.0150775215706431));
#32750=CARTESIAN_POINT('Ctrl Pts',(0.000823994324082737,-0.0352893349892275,
-0.015060766118253));
#32751=CARTESIAN_POINT('Ctrl Pts',(0.000863434917108734,-0.0352914391958564,
-0.015049208301472));
#32752=CARTESIAN_POINT('Ctrl Pts',(0.00102997600453913,-0.0353002815883928,
-0.0149966654928808));
#32753=CARTESIAN_POINT('Ctrl Pts',(0.00115450741646375,-0.0353067779285413,
-0.0149480273707974));
#32754=CARTESIAN_POINT('Ctrl Pts',(0.00135818382546414,-0.0353175380028714,
-0.0148523628690619));
#32755=CARTESIAN_POINT('Ctrl Pts',(0.00143915547467117,-0.0353218570361767,
-0.0148097094986222));
#32756=CARTESIAN_POINT('Ctrl Pts',(0.00164533814460637,-0.0353332064572015,
-0.0146887481524998));
#32757=CARTESIAN_POINT('Ctrl Pts',(0.00176692979934277,-0.035340255689866,
-0.0146047891214333));
#32758=CARTESIAN_POINT('Ctrl Pts',(0.00190500854207849,-0.0353492839001866,
-0.0144935736248103));
#32759=CARTESIAN_POINT('Ctrl Pts',(0.00192789860726415,-0.0353508174483709,
-0.0144745685682159));
#32760=CARTESIAN_POINT('Ctrl Pts',(0.00196128070921921,-0.0353531153268114,
-0.0144460028973862));
#32761=CARTESIAN_POINT('Ctrl Pts',(0.00197199422219986,-0.0353538623749409,
-0.0144367026950361));
#32762=CARTESIAN_POINT('Ctrl Pts',(0.00199103683897563,-0.0353552082656566,
-0.0144199338227507));
#32763=CARTESIAN_POINT('Ctrl Pts',(0.00199939069241221,-0.0353558050623468,
-0.0144124940710782));
#32764=CARTESIAN_POINT('Ctrl Pts',(0.00201797375330345,-0.035357147025304,
-0.014395757111758));
#32765=CARTESIAN_POINT('Ctrl Pts',(0.0020281803463914,-0.0353578938856961,
-0.0143864359088202));
#32766=CARTESIAN_POINT('Ctrl Pts',(0.00205875760081152,-0.0353601600735434,
-0.0143581211111652));
#32767=CARTESIAN_POINT('Ctrl Pts',(0.00207892802349295,-0.035361693891269,
-0.014338914515934));
#32768=CARTESIAN_POINT('Ctrl Pts',(0.00217771454033156,-0.0353693883602091,
-0.0142421902929268));
#32769=CARTESIAN_POINT('Ctrl Pts',(0.00225227201902579,-0.0353757783059338,
-0.0141606596484366));
#32770=CARTESIAN_POINT('Ctrl Pts',(0.00248789499352634,-0.0353975562332824,
-0.0138725865777045));
#32771=CARTESIAN_POINT('Ctrl Pts',(0.0026264282681735,-0.0354130553448458,
-0.0136490958475107));
#32772=CARTESIAN_POINT('Ctrl Pts',(0.00275019798843151,-0.0354296164117932,
-0.0133749880325005));
#32773=CARTESIAN_POINT('Ctrl Pts',(0.00276551539659859,-0.0354317361552911,
-0.0133392267850519));
#32774=CARTESIAN_POINT('Ctrl Pts',(0.00278943361497699,-0.0354351670758613,
-0.0132802411859556));
#32775=CARTESIAN_POINT('Ctrl Pts',(0.00279844975250142,-0.0354364917494667,
-0.0132571911417256));
#32776=CARTESIAN_POINT('Ctrl Pts',(0.00281419771968432,-0.0354388644406584,
-0.0132154142773067));
#32777=CARTESIAN_POINT('Ctrl Pts',(0.00282103035834589,-0.035439915707377,
-0.0131967272267249));
#32778=CARTESIAN_POINT('Ctrl Pts',(0.00283531831039913,-0.0354421627381174,
-0.0131564109877264));
#32779=CARTESIAN_POINT('Ctrl Pts',(0.00284271316972503,-0.035443356488532,
-0.0131347616236971));
#32780=CARTESIAN_POINT('Ctrl Pts',(0.00286252006682121,-0.0354466433586039,
-0.0130745308093722));
#32781=CARTESIAN_POINT('Ctrl Pts',(0.00287439926247934,-0.0354487194019013,
-0.0130357785740234));
#32782=CARTESIAN_POINT('Ctrl Pts',(0.00292094883453316,-0.0354573373929622,
-0.0128721639036939));
#32783=CARTESIAN_POINT('Ctrl Pts',(0.00294829760271707,-0.0354636525531688,
-0.0127453583361953));
#32784=CARTESIAN_POINT('Ctrl Pts',(0.00297920596294723,-0.035473712465473,
-0.0125375358704473));
#32785=CARTESIAN_POINT('Ctrl Pts',(0.00298783942475793,-0.0354775228170552,
-0.0124574527700879));
#32786=CARTESIAN_POINT('Ctrl Pts',(0.003004254943023,-0.0354891250148958,
-0.0122133197283107));
#32787=CARTESIAN_POINT('Ctrl Pts',(0.00300180377856027,-0.0354969119081081,
-0.0120489082021016));
#32788=CARTESIAN_POINT('Ctrl Pts',(0.00298308284062134,-0.0355067683900154,
-0.0118563592865642));
#32789=CARTESIAN_POINT('Ctrl Pts',(0.00297981799026124,-0.0355082803582784,
-0.0118272212824298));
#32790=CARTESIAN_POINT('Ctrl Pts',(0.00297435075122108,-0.0355105519412426,
-0.0117841434736861));
#32791=CARTESIAN_POINT('Ctrl Pts',(0.00297247613896369,-0.0355112948386907,
-0.0117701630640507));
#32792=CARTESIAN_POINT('Ctrl Pts',(0.00296893837442253,-0.0355126365285948,
-0.0117451213040687));
#32793=CARTESIAN_POINT('Ctrl Pts',(0.00296731185787311,-0.035513233336693,
-0.0117340553210341));
#32794=CARTESIAN_POINT('Ctrl Pts',(0.00296352543645847,-0.0355145795042095,
-0.0117092590723368));
#32795=CARTESIAN_POINT('Ctrl Pts',(0.00296133199462682,-0.0355153306163834,
-0.0116955346674882));
#32796=CARTESIAN_POINT('Ctrl Pts',(0.00295439247135007,-0.0355176226675588,
-0.0116539694306518));
#32797=CARTESIAN_POINT('Ctrl Pts',(0.00294934865376934,-0.035519178566197,
-0.011626180620626));
#32798=CARTESIAN_POINT('Ctrl Pts',(0.00292200145941928,-0.0355270902140677,
-0.0114867454820147));
#32799=CARTESIAN_POINT('Ctrl Pts',(0.00289374888780714,-0.0355336888710772,
-0.0113763687435723));
#32800=CARTESIAN_POINT('Ctrl Pts',(0.00279882897120363,-0.0355520547175795,
-0.011077458764045));
#32801=CARTESIAN_POINT('Ctrl Pts',(0.00271948512217469,-0.0355638836750979,
-0.010893539523627));
#32802=CARTESIAN_POINT('Ctrl Pts',(0.00258269460608775,-0.0355798341890619,
-0.0106473291393328));
#32803=CARTESIAN_POINT('Ctrl Pts',(0.00254003605500516,-0.0355843828625148,
-0.0105774428116812));
#32804=CARTESIAN_POINT('Ctrl Pts',(0.0024775887225792,-0.0355904929685943,
-0.0104839642136478));
#32805=CARTESIAN_POINT('Ctrl Pts',(0.00246021955942856,-0.035592140334989,
-0.0104588051433091));
#32806=CARTESIAN_POINT('Ctrl Pts',(0.00243159822569542,-0.0355947735420527,
-0.0104186735745273));
#32807=CARTESIAN_POINT('Ctrl Pts',(0.00242058542714945,-0.0355957682274401,
-0.0104035337096179));
#32808=CARTESIAN_POINT('Ctrl Pts',(0.00239730437013557,-0.0355978332217003,
-0.0103721498533602));
#32809=CARTESIAN_POINT('Ctrl Pts',(0.00238501102549321,-0.0355989025012567,
-0.0103559256085253));
#32810=CARTESIAN_POINT('Ctrl Pts',(0.00235529657326915,-0.0356014380629962,
-0.0103175279340267));
#32811=CARTESIAN_POINT('Ctrl Pts',(0.00233772595529563,-0.0356028984619101,
-0.0102954723434859));
#32812=CARTESIAN_POINT('Ctrl Pts',(0.00227499037939574,-0.0356079820961516,
-0.0102189619968596));
#32813=CARTESIAN_POINT('Ctrl Pts',(0.00222821134265425,-0.0356115416780241,
-0.0101658582847115));
#32814=CARTESIAN_POINT('Ctrl Pts',(0.00210477889758045,-0.0356204276361308,
-0.010035348361344));
#32815=CARTESIAN_POINT('Ctrl Pts',(0.00202570772893042,-0.0356256632065451,
-0.0099603701160623));
#32816=CARTESIAN_POINT('Ctrl Pts',(0.00182080313311095,-0.0356384650704474,
-0.00978623413408031));
#32817=CARTESIAN_POINT('Ctrl Pts',(0.00169078563158549,-0.0356459445899314,
-0.00969254034883679));
#32818=CARTESIAN_POINT('Ctrl Pts',(0.00149007106669639,-0.0356574155936249,
-0.00957100002751177));
#32819=CARTESIAN_POINT('Ctrl Pts',(0.00142480103958752,-0.0356611377085898,
-0.0095347336854759));
#32820=CARTESIAN_POINT('Ctrl Pts',(0.00134002046946372,-0.0356660458469634,
-0.00949168428875245));
#32821=CARTESIAN_POINT('Ctrl Pts',(0.00132169574677134,-0.0356671109668186,
-0.00948261390312541));
#32822=CARTESIAN_POINT('Ctrl Pts',(0.00129222102104624,-0.0356688331712479,
-0.00946839772997434));
#32823=CARTESIAN_POINT('Ctrl Pts',(0.00128112936501425,-0.0356694832719174,
-0.00946313171999589));
#32824=CARTESIAN_POINT('Ctrl Pts',(0.00125955000247898,-0.0356707525567307,
-0.00945304830138889));
#32825=CARTESIAN_POINT('Ctrl Pts',(0.00124906634270593,-0.0356713712775203,
-0.00944822309673462));
#32826=CARTESIAN_POINT('Ctrl Pts',(0.00122310909517892,-0.0356729078963964,
-0.00943645704824017));
#32827=CARTESIAN_POINT('Ctrl Pts',(0.0012076040867256,-0.0356738298338929,
-0.00942958673859811));
#32828=CARTESIAN_POINT('Ctrl Pts',(0.00114865157128265,-0.0356773482285946,
-0.00940406049390908));
#32829=CARTESIAN_POINT('Ctrl Pts',(0.00110482522134812,-0.0356799904646111,
-0.00938630198301244));
#32830=CARTESIAN_POINT('Ctrl Pts',(0.000987090500063967,-0.0356871247529926,
-0.00934180532661316));
#32831=CARTESIAN_POINT('Ctrl Pts',(0.000912521190919585,-0.0356916800276548,
-0.00931692352892374));
#32832=CARTESIAN_POINT('Ctrl Pts',(0.000578718474900576,-0.0357120031188721,
-0.00921993332101712));
#32833=CARTESIAN_POINT('Ctrl Pts',(0.000311390463711398,-0.0357279528770105,
-0.00917994576843555));
#32834=CARTESIAN_POINT('Ctrl Pts',(1.2640490683327E-6,-0.0357450060604786,
-0.00917557289780277));
#32835=CARTESIAN_POINT('Ctrl Pts',(-3.97773751530382E-5,-0.0357472374922339,
-0.00917583628752131));
#32836=CARTESIAN_POINT('Ctrl Pts',(-0.00010401540030905,-0.0357506915968563,
-0.00917756710042888));
#32837=CARTESIAN_POINT('Ctrl Pts',(-0.000127221269946943,-0.0357519315240605,
-0.00917846207972079));
#32838=CARTESIAN_POINT('Ctrl Pts',(-0.000170260321233034,-0.0357542171177686,
-0.0091806227014639));
#32839=CARTESIAN_POINT('Ctrl Pts',(-0.000190095700126816,-0.035755264932482,
-0.00918181613165416));
#32840=CARTESIAN_POINT('Ctrl Pts',(-0.000234161614358208,-0.0357575809579381,
-0.00918490711869147));
#32841=CARTESIAN_POINT('Ctrl Pts',(-0.000258384027387859,-0.0357588461088733,
-0.00918690223642446));
#32842=CARTESIAN_POINT('Ctrl Pts',(-0.000329993331741674,-0.0357625645113579,
-0.00919367747865179));
#32843=CARTESIAN_POINT('Ctrl Pts',(-0.000377294606204041,-0.0357649922616427,
-0.00919929197504775));
#32844=CARTESIAN_POINT('Ctrl Pts',(-0.000486192326624026,-0.0357705291573544,
-0.00921485551991437));
#32845=CARTESIAN_POINT('Ctrl Pts',(-0.000547652502143375,-0.0357736149414238,
-0.00922560447311942));
#32846=CARTESIAN_POINT('Ctrl Pts',(-0.00077809403146185,-0.0357851048795045,
-0.00927335716765128));
#32847=CARTESIAN_POINT('Ctrl Pts',(-0.000944098692126996,-0.0357931978196018,
-0.00932303136735014));
#32848=CARTESIAN_POINT('Ctrl Pts',(-0.00123300152870086,-0.0358080037030274,
-0.00943747928173621));
#32849=CARTESIAN_POINT('Ctrl Pts',(-0.0013574418274879,-0.0358146531628978,
-0.00949698614339815));
#32850=CARTESIAN_POINT('Ctrl Pts',(-0.00149692664947124,-0.0358228944549558,
-0.00957590769076583));
#32851=CARTESIAN_POINT('Ctrl Pts',(-0.00151638821710602,-0.03582406319409,
-0.00958721016462689));
#32852=CARTESIAN_POINT('Ctrl Pts',(-0.00154676225157033,-0.0358259200028109,
-0.0096053101999919));
#32853=CARTESIAN_POINT('Ctrl Pts',(-0.00155776167756375,-0.0358265992567676,
-0.00961196097860854));
#32854=CARTESIAN_POINT('Ctrl Pts',(-0.00157836009166009,-0.0358278848432368,
-0.00962459724626502));
#32855=CARTESIAN_POINT('Ctrl Pts',(-0.00158796841316746,-0.0358284901859162,
-0.00963056660996079));
#32856=CARTESIAN_POINT('Ctrl Pts',(-0.00161073364819649,-0.0358299377072133,
-0.00964488904518821));
#32857=CARTESIAN_POINT('Ctrl Pts',(-0.0016238595459862,-0.0358307829006293,
-0.00965329049633871));
#32858=CARTESIAN_POINT('Ctrl Pts',(-0.00166859978259292,-0.0358336985936239,
-0.00968242112911092));
#32859=CARTESIAN_POINT('Ctrl Pts',(-0.00169988635108253,-0.0358357975969619,
-0.00970364469975761));
#32860=CARTESIAN_POINT('Ctrl Pts',(-0.00177716194304706,-0.0358411177276784,
-0.00975822584444497));
#32861=CARTESIAN_POINT('Ctrl Pts',(-0.00182261951791848,-0.0358443712949381,
-0.00979230875885999));
#32862=CARTESIAN_POINT('Ctrl Pts',(-0.00205281636964779,-0.035861395976342,
-0.00997534134104765));
#32863=CARTESIAN_POINT('Ctrl Pts',(-0.00222040102343298,-0.0358755951013135,
-0.0101445613961145));
#32864=CARTESIAN_POINT('Ctrl Pts',(-0.00241927372754666,-0.035893960534741,
-0.0103997496023323));
#32865=CARTESIAN_POINT('Ctrl Pts',(-0.00246930624738904,-0.0358987599965681,
-0.0104699932953441));
#32866=CARTESIAN_POINT('Ctrl Pts',(-0.00253318293974001,-0.0359051400291047,
-0.0105683858663624));
#32867=CARTESIAN_POINT('Ctrl Pts',(-0.0025497120692482,-0.0359068169183037,
-0.0105947347661383));
#32868=CARTESIAN_POINT('Ctrl Pts',(-0.0025755790368098,-0.0359094846237416,
-0.0106374298462313));
#32869=CARTESIAN_POINT('Ctrl Pts',(-0.00258517768870117,-0.0359104847268032,
-0.0106536146731552));
#32870=CARTESIAN_POINT('Ctrl Pts',(-0.00260480559629456,-0.0359125516483981,
-0.0106874315651146));
#32871=CARTESIAN_POINT('Ctrl Pts',(-0.00261480959590133,-0.0359136175368941,
-0.0107050772263566));
#32872=CARTESIAN_POINT('Ctrl Pts',(-0.00263808771232186,-0.035916128349276,
-0.0107471249035681));
#32873=CARTESIAN_POINT('Ctrl Pts',(-0.00265120350205029,-0.0359175677036972,
-0.0107716126991749));
#32874=CARTESIAN_POINT('Ctrl Pts',(-0.00269520022554495,-0.0359224863568711,
-0.0108565710396449));
#32875=CARTESIAN_POINT('Ctrl Pts',(-0.00272436833485895,-0.0359259076037169,
-0.0109179073711483));
#32876=CARTESIAN_POINT('Ctrl Pts',(-0.00279222630517896,-0.035934345868882,
-0.0110740596658006));
#32877=CARTESIAN_POINT('Ctrl Pts',(-0.00282819169515727,-0.0359392843203902,
-0.0111699654192824));
#32878=CARTESIAN_POINT('Ctrl Pts',(-0.0029189285374855,-0.0359535815104554,
-0.0114555821162686));
#32879=CARTESIAN_POINT('Ctrl Pts',(-0.0029599679246924,-0.0359627342564858,
-0.0116490583439944));
#32880=CARTESIAN_POINT('Ctrl Pts',(-0.00298749116615407,-0.0359751427634141,
-0.0118972121940021));
#32881=CARTESIAN_POINT('Ctrl Pts',(-0.00299190092736898,-0.0359777920004475,
-0.0119494188085586));
#32882=CARTESIAN_POINT('Ctrl Pts',(-0.00299599531540426,-0.0359814481546266,
-0.0120198351449709));
#32883=CARTESIAN_POINT('Ctrl Pts',(-0.00299688457985966,-0.0359823970292153,
-0.0120379679209503));
#32884=CARTESIAN_POINT('Ctrl Pts',(-0.0029980328675489,-0.0359839144702652,
-0.0120667130621144));
#32885=CARTESIAN_POINT('Ctrl Pts',(-0.0029984002450903,-0.0359844773066483,
-0.0120773209219052));
#32886=CARTESIAN_POINT('Ctrl Pts',(-0.00299905304236399,-0.0359856650120847,
-0.012099585311108));
#32887=CARTESIAN_POINT('Ctrl Pts',(-0.002999326808685,-0.0359862905408736,
-0.0121112418630132));
#32888=CARTESIAN_POINT('Ctrl Pts',(-0.00299984268902756,-0.035987867465534,
-0.0121404635320267));
#32889=CARTESIAN_POINT('Ctrl Pts',(-0.00299999848009557,-0.0359888233622487,
-0.0121580296009286));
#32890=CARTESIAN_POINT('Ctrl Pts',(-0.00300000446576103,-0.0359926443202545,
-0.0122277151720247));
#32891=CARTESIAN_POINT('Ctrl Pts',(-0.00299865071308026,-0.0359955654232249,
-0.0122798231593143));
#32892=CARTESIAN_POINT('Ctrl Pts',(-0.00299119267042623,-0.0360037233650442,
-0.0124230410351089));
#32893=CARTESIAN_POINT('Ctrl Pts',(-0.00298228539517348,-0.0360090448149082,
-0.0125139473711002));
#32894=CARTESIAN_POINT('Ctrl Pts',(-0.0029369956463546,-0.0360276453175141,
-0.0128278163188737));
#32895=CARTESIAN_POINT('Ctrl Pts',(-0.00287960294277976,-0.036040969330536,
-0.0130470086908784));
#32896=CARTESIAN_POINT('Ctrl Pts',(-0.00277769058637646,-0.036056702744964,
-0.0133106009435901));
#32897=CARTESIAN_POINT('Ctrl Pts',(-0.0027557391732687,-0.0360598149919933,
-0.0133629166525026));
#32898=CARTESIAN_POINT('Ctrl Pts',(-0.00272170725122933,-0.036064266480404,
-0.0134379823683335));
#32899=CARTESIAN_POINT('Ctrl Pts',(-0.00271079755916636,-0.0360656441297542,
-0.0134612469341236));
#32900=CARTESIAN_POINT('Ctrl Pts',(-0.00269085028842581,-0.0360680781725724,
-0.0135024000169851));
#32901=CARTESIAN_POINT('Ctrl Pts',(-0.00268192991378836,-0.0360691384536184,
-0.0135203433260573));
#32902=CARTESIAN_POINT('Ctrl Pts',(-0.00266281773391231,-0.0360713525648563,
-0.013557840208983));
#32903=CARTESIAN_POINT('Ctrl Pts',(-0.00265258875598696,-0.0360725050377761,
-0.0135773735551754));
#32904=CARTESIAN_POINT('Ctrl Pts',(-0.00262481767440084,-0.0360755503132234,
-0.0136290120897287));
#32905=CARTESIAN_POINT('Ctrl Pts',(-0.0026069018317157,-0.0360774300754184,
-0.0136609126516327));
#32906=CARTESIAN_POINT('Ctrl Pts',(-0.00249102456812778,-0.0360890890793787,
-0.0138586790253759));
#32907=CARTESIAN_POINT('Ctrl Pts',(-0.00237786047785913,-0.0360982973943212,
-0.0140151180067865));
#32908=CARTESIAN_POINT('Ctrl Pts',(-0.00212381856825827,-0.0361165180276222,
-0.014303311021787));
#32909=CARTESIAN_POINT('Ctrl Pts',(-0.00198371673595574,-0.0361255015589338,
-0.01443451081625));
#32910=CARTESIAN_POINT('Ctrl Pts',(-0.00181014934738116,-0.0361366927959653,
-0.0145683680477551));
#32911=CARTESIAN_POINT('Ctrl Pts',(-0.00178797848923303,-0.0361381237947136,
-0.0145849818346945));
#32912=CARTESIAN_POINT('Ctrl Pts',(-0.00175442959424053,-0.0361402964925662,
-0.0146094035870066));
#32913=CARTESIAN_POINT('Ctrl Pts',(-0.0017432220614141,-0.0361410235150193,
-0.0146174443858314));
#32914=CARTESIAN_POINT('Ctrl Pts',(-0.00172282466151885,-0.0361423496054179,
-0.0146318663875494));
#32915=CARTESIAN_POINT('Ctrl Pts',(-0.00171365402088759,-0.0361429469267552,
-0.0146382738545781));
#32916=CARTESIAN_POINT('Ctrl Pts',(-0.00169274658924429,-0.0361443112357483,
-0.0146527083813521));
#32917=CARTESIAN_POINT('Ctrl Pts',(-0.00168098847057417,-0.0361450802202468,
-0.0146607033668935));
#32918=CARTESIAN_POINT('Ctrl Pts',(-0.00164431359148961,-0.0361474829283557,
-0.014685261181092));
#32919=CARTESIAN_POINT('Ctrl Pts',(-0.00161920624480304,-0.0361491337014477,
-0.0147015346149449));
#32920=CARTESIAN_POINT('Ctrl Pts',(-0.00148403081831568,-0.036158034850397,
-0.0147863051682421));
#32921=CARTESIAN_POINT('Ctrl Pts',(-0.00136985965557709,-0.0361655945145673,
-0.0148479846532686));
#32922=CARTESIAN_POINT('Ctrl Pts',(-0.0010299371033938,-0.0361875549046775,
-0.0150040999399211));
#32923=CARTESIAN_POINT('Ctrl Pts',(-0.000796130037670471,-0.0362019196288875,
-0.0150786043184217));
#32924=CARTESIAN_POINT('Ctrl Pts',(-0.000516810069068373,-0.0362175284952902,
-0.0151312696220082));
#32925=CARTESIAN_POINT('Ctrl Pts',(-0.000477625799261746,-0.0362196867764967,
-0.0151378546646231));
#32926=CARTESIAN_POINT('Ctrl Pts',(-0.000415630167953753,-0.0362230532810829,
-0.0151470109173127));
#32927=CARTESIAN_POINT('Ctrl Pts',(-0.000392901272377092,-0.0362242773700545,
-0.0151501018862697));
#32928=CARTESIAN_POINT('Ctrl Pts',(-0.000350400163917462,-0.036226547939529,
-0.0151553860281987));
#32929=CARTESIAN_POINT('Ctrl Pts',(-0.000330637378707389,-0.0362275963553301,
-0.0151576437859936));
#32930=CARTESIAN_POINT('Ctrl Pts',(-0.000286319573974246,-0.0362299314524598,
-0.0151622607498318));
#32931=CARTESIAN_POINT('Ctrl Pts',(-0.000261754830036736,-0.0362312148140198,
-0.0151645140051839));
#32932=CARTESIAN_POINT('Ctrl Pts',(-0.000187797776576142,-0.0362350475724103,
-0.0151703790261994));
#32933=CARTESIAN_POINT('Ctrl Pts',(-0.000138339992681926,-0.0362375689594494,
-0.0151730711308622));
#32934=CARTESIAN_POINT('Ctrl Pts',(0.000116250536762689,-0.0362503682636465,
-0.0151806134042614));
#32935=CARTESIAN_POINT('Ctrl Pts',(0.000321419199358098,-0.0362600363131822,
-0.0151656348821813));
#32936=CARTESIAN_POINT('Ctrl Pts',(0.000674690224411421,-0.0362770596895092,
-0.0151030328860211));
#32937=CARTESIAN_POINT('Ctrl Pts',(0.000823621058036811,-0.0362843764791667,
-0.015064663907936));
#32938=CARTESIAN_POINT('Ctrl Pts',(0.000997093887906155,-0.0362937102196635,
-0.0150054625301104));
#32939=CARTESIAN_POINT('Ctrl Pts',(0.00102509814223837,-0.0362952434151831,
-0.0149954380726004));
#32940=CARTESIAN_POINT('Ctrl Pts',(0.00106623107715375,-0.036297540864094,
-0.0149800202802216));
#32941=CARTESIAN_POINT('Ctrl Pts',(0.00107947870708767,-0.036298287844663,
-0.0149749472370169));
#32942=CARTESIAN_POINT('Ctrl Pts',(0.00110310804554624,-0.0362996336666335,
-0.0149657059325244));
#32943=CARTESIAN_POINT('Ctrl Pts',(0.00111350310949635,-0.0363002304631388,
-0.0149615732947957));
#32944=CARTESIAN_POINT('Ctrl Pts',(0.00113669207131603,-0.036301572492908,
-0.0149522038103222));
#32945=CARTESIAN_POINT('Ctrl Pts',(0.0011494729228974,-0.0363023194212357,
-0.0149469366632353));
#32946=CARTESIAN_POINT('Ctrl Pts',(0.00118789914223002,-0.0363045860209889,
-0.0149307891644975));
#32947=CARTESIAN_POINT('Ctrl Pts',(0.00121342916770938,-0.0363061201901037,
-0.0149196400148282));
#32948=CARTESIAN_POINT('Ctrl Pts',(0.00133940120861653,-0.0363138180789388,
-0.0148625251346083));
#32949=CARTESIAN_POINT('Ctrl Pts',(0.00143739996686642,-0.0363202113048059,
-0.0148113947578893));
#32950=CARTESIAN_POINT('Ctrl Pts',(0.00175730887216658,-0.0363419866340859,
-0.0146213260183779));
#32951=CARTESIAN_POINT('Ctrl Pts',(0.00196386152873907,-0.0363574793432828,
-0.014458781871455));
#32952=CARTESIAN_POINT('Ctrl Pts',(0.00217389430384587,-0.0363740361980171,
-0.0142436294527254));
#32953=CARTESIAN_POINT('Ctrl Pts',(0.00220053740300941,-0.0363761570975972,
-0.0142152527195389));
#32954=CARTESIAN_POINT('Ctrl Pts',(0.00224321190486484,-0.0363795894882185,
-0.0141679911262435));
#32955=CARTESIAN_POINT('Ctrl Pts',(0.00225957440740101,-0.0363809144952551,
-0.0141494126014718));
#32956=CARTESIAN_POINT('Ctrl Pts',(0.00228866992933204,-0.0363832875454547,
-0.0141155403310367));
#32957=CARTESIAN_POINT('Ctrl Pts',(0.00230148417241686,-0.036384338842024,
-0.0141003185383934));
#32958=CARTESIAN_POINT('Ctrl Pts',(0.00232870134266448,-0.0363865856821838,
-0.0140673270993386));
#32959=CARTESIAN_POINT('Ctrl Pts',(0.0023430544507531,-0.0363877792154732,
-0.0140495178793561));
#32960=CARTESIAN_POINT('Ctrl Pts',(0.00238225824026796,-0.0363910648052641,
-0.0139997190718823));
#32961=CARTESIAN_POINT('Ctrl Pts',(0.00240666726536358,-0.0363931398080355,
-0.0139673871536493));
#32962=CARTESIAN_POINT('Ctrl Pts',(0.00255034639338418,-0.0364055566190344,
-0.0137688333369805));
#32963=CARTESIAN_POINT('Ctrl Pts',(0.00265301248107068,-0.0364152588639168,
-0.0135912633896652));
#32964=CARTESIAN_POINT('Ctrl Pts',(0.00280657010375567,-0.0364330326520467,
-0.0132492448683431));
#32965=CARTESIAN_POINT('Ctrl Pts',(0.00286296272161191,-0.0364410903712434,
-0.0130882337540886));
#32966=CARTESIAN_POINT('Ctrl Pts',(0.00291262039576375,-0.0364512484975482,
-0.012895217561391));
#32967=CARTESIAN_POINT('Ctrl Pts',(0.00291944394782601,-0.0364527457688092,
-0.0128670041007212));
#32968=CARTESIAN_POINT('Ctrl Pts',(0.00292896107046031,-0.0364549994289248,
-0.0128249945978945));
#32969=CARTESIAN_POINT('Ctrl Pts',(0.00293196896862156,-0.036455739480162,
-0.0128112707447091));
#32970=CARTESIAN_POINT('Ctrl Pts',(0.0029371980543264,-0.0364570783169823,
-0.0127865845601266));
#32971=CARTESIAN_POINT('Ctrl Pts',(0.00293945448876798,-0.0364576751605383,
-0.0127756302445659));
#32972=CARTESIAN_POINT('Ctrl Pts',(0.0029443881296107,-0.0364590243324186,
-0.0127509821567199));
#32973=CARTESIAN_POINT('Ctrl Pts',(0.00294703107634154,-0.0364597784548663,
-0.0127372822624239));
#32974=CARTESIAN_POINT('Ctrl Pts',(0.00295478538395082,-0.0364620889218922,
-0.0126955231591981));
#32975=CARTESIAN_POINT('Ctrl Pts',(0.00295959212610445,-0.0364636605647079,
-0.0126674097665459));
#32976=CARTESIAN_POINT('Ctrl Pts',(0.00298196990773466,-0.0364717299512634,
-0.0125242708731424));
#32977=CARTESIAN_POINT('Ctrl Pts',(0.00299323769398351,-0.0364784807095211,
-0.0124083685500126));
#32978=CARTESIAN_POINT('Ctrl Pts',(0.0030057654876214,-0.0364974208622691,
-0.012085345771044));
#32979=CARTESIAN_POINT('Ctrl Pts',(0.00299237074063453,-0.0365096628881006,
-0.0118782768645188));
#32980=CARTESIAN_POINT('Ctrl Pts',(0.00294535016614654,-0.0365255166214546,
-0.0116010276599633));
#32981=CARTESIAN_POINT('Ctrl Pts',(0.00293022238353103,-0.0365296293113734,
-0.0115283116476631));
#32982=CARTESIAN_POINT('Ctrl Pts',(0.00290533963104305,-0.0365352595648814,
-0.0114276082146904));
#32983=CARTESIAN_POINT('Ctrl Pts',(0.00289784653207465,-0.0365368464537141,
-0.0113990942378676));
#32984=CARTESIAN_POINT('Ctrl Pts',(0.00288446375329487,-0.0365395080808752,
-0.0113510597922487));
#32985=CARTESIAN_POINT('Ctrl Pts',(0.00287879328157979,-0.0365405896676996,
-0.0113314809031983));
#32986=CARTESIAN_POINT('Ctrl Pts',(0.00286691521852962,-0.036542765596481,
-0.0112919797198651));
#32987=CARTESIAN_POINT('Ctrl Pts',(0.00286069843270487,-0.0365438595744673,
-0.011272061353524));
#32988=CARTESIAN_POINT('Ctrl Pts',(0.00284475981024879,-0.0365465575247099,
-0.011222807320906));
#32989=CARTESIAN_POINT('Ctrl Pts',(0.0028347914317321,-0.0365481535001276,
-0.0111935536278561));
#32990=CARTESIAN_POINT('Ctrl Pts',(0.00279329964189367,-0.0365544544545892,
-0.0110776856491529));
#32991=CARTESIAN_POINT('Ctrl Pts',(0.00275824297825931,-0.0365590452878288,
-0.0109923869126421));
#32992=CARTESIAN_POINT('Ctrl Pts',(0.00264740074443722,-0.0365718638606297,
-0.0107544945394076));
#32993=CARTESIAN_POINT('Ctrl Pts',(0.00256248164488157,-0.0365798388836663,
-0.0106065602530943));
#32994=CARTESIAN_POINT('Ctrl Pts',(0.00238494659545061,-0.0365946746051794,
-0.0103504753036083));
#32995=CARTESIAN_POINT('Ctrl Pts',(0.00229632337619972,-0.0366014836238115,
-0.010240170970903));
#32996=CARTESIAN_POINT('Ctrl Pts',(0.00218494895902605,-0.0366099084212479,
-0.0101200065252737));
#32997=CARTESIAN_POINT('Ctrl Pts',(0.00216944445717086,-0.0366110786895943,
-0.0101036519089914));
#32998=CARTESIAN_POINT('Ctrl Pts',(0.00214480495625915,-0.0366129374017226,
-0.0100782410495192));
#32999=CARTESIAN_POINT('Ctrl Pts',(0.00213579317251943,-0.0366136170002465,
-0.0100690659433162));
#33000=CARTESIAN_POINT('Ctrl Pts',(0.00211874570625072,-0.0366149028298883,
-0.0100519313120288));
#33001=CARTESIAN_POINT('Ctrl Pts',(0.00211072364031695,-0.0366155080653574,
-0.010043958912748));
#33002=CARTESIAN_POINT('Ctrl Pts',(0.0020915500342721,-0.0366169547660525,
-0.0100251183128678));
#33003=CARTESIAN_POINT('Ctrl Pts',(0.00208035869424938,-0.0366177992364829,
-0.0100142913153454));
#33004=CARTESIAN_POINT('Ctrl Pts',(0.00204176856454916,-0.0366207097053319,
-0.00997753480300241));
#33005=CARTESIAN_POINT('Ctrl Pts',(0.00201396619849019,-0.0366228040759775,
-0.00995203608989637));
#33006=CARTESIAN_POINT('Ctrl Pts',(0.00194323780956477,-0.0366281096275946,
-0.00988958242850173));
#33007=CARTESIAN_POINT('Ctrl Pts',(0.0018997327068062,-0.0366313530404973,
-0.00985330669503815));
#33008=CARTESIAN_POINT('Ctrl Pts',(0.00167043419294685,-0.0366482420893763,
-0.00967286592462395));
#33009=CARTESIAN_POINT('Ctrl Pts',(0.00146915479416005,-0.0366623117469007,
-0.00954965853702657));
#33010=CARTESIAN_POINT('Ctrl Pts',(0.00117549151968438,-0.0366806854025545,
-0.00941433367250835));
#33011=CARTESIAN_POINT('Ctrl Pts',(0.00109383854871171,-0.0366855976305841,
-0.00938098473124982));
#33012=CARTESIAN_POINT('Ctrl Pts',(0.00098134625636968,-0.0366920973499346,
-0.00934072716949374));
#33013=CARTESIAN_POINT('Ctrl Pts',(0.000951699117684725,-0.0366937860358502,
-0.0093306380988298));
#33014=CARTESIAN_POINT('Ctrl Pts',(0.000901964581640302,-0.0366965793944118,
-0.00931457757477032));
#33015=CARTESIAN_POINT('Ctrl Pts',(0.000881963296006947,-0.0366976922472465,
-0.00930834921859086));
#33016=CARTESIAN_POINT('Ctrl Pts',(0.000842209702367135,-0.036699883800035,
-0.00929642533591894));
#33017=CARTESIAN_POINT('Ctrl Pts',(0.000822460854643503,-0.0367009626895432,
-0.00929072232315037));
#33018=CARTESIAN_POINT('Ctrl Pts',(0.00077441871185937,-0.0367035642101964,
-0.00927738224183657));
#33019=CARTESIAN_POINT('Ctrl Pts',(0.000746068838789926,-0.0367050801130852,
-0.00926995581700696));
#33020=CARTESIAN_POINT('Ctrl Pts',(0.000641096027188231,-0.0367106264794309,
-0.00924409506994982));
#33021=CARTESIAN_POINT('Ctrl Pts',(0.000563861671009458,-0.0367145760332935,
-0.00922826585836568));
#33022=CARTESIAN_POINT('Ctrl Pts',(0.000358759315627147,-0.03672480538856,
-0.00919458815514616));
#33023=CARTESIAN_POINT('Ctrl Pts',(0.000230208683209771,-0.0367309507413409,
-0.00918191668380646));
#33024=CARTESIAN_POINT('Ctrl Pts',(-9.00185525693171E-5,-0.0367461468814493,
-0.00917110414474542));
#33025=CARTESIAN_POINT('Ctrl Pts',(-0.000281433776674939,-0.0367551235167671,
-0.00918296170668082));
#33026=CARTESIAN_POINT('Ctrl Pts',(-0.000497765622491052,-0.0367663070708568,
-0.00921730674930765));
#33027=CARTESIAN_POINT('Ctrl Pts',(-0.000525077258624144,-0.0367677386903863,
-0.00922203169455336));
#33028=CARTESIAN_POINT('Ctrl Pts',(-0.00056587886809098,-0.0367699121477052,
-0.00922967416104993));
#33029=CARTESIAN_POINT('Ctrl Pts',(-0.000579421221987906,-0.0367706392936709,
-0.00923230757331932));
#33030=CARTESIAN_POINT('Ctrl Pts',(-0.000603911681821247,-0.0367719655023004,
-0.00923724547920457));
#33031=CARTESIAN_POINT('Ctrl Pts',(-0.0006148657016026,-0.0367725628164889,
-0.00923951793029843));
#33032=CARTESIAN_POINT('Ctrl Pts',(-0.000639710303475704,-0.0367739269704792,
-0.00924481715111586));
#33033=CARTESIAN_POINT('Ctrl Pts',(-0.00065359220211092,-0.0367746958050904,
-0.00924788140880198));
#33034=CARTESIAN_POINT('Ctrl Pts',(-0.000696607047403286,-0.0367770975716373,
-0.00925769754465249));
#33035=CARTESIAN_POINT('Ctrl Pts',(-0.000725660404111588,-0.0367787475347113,
-0.00926478627289187));
#33036=CARTESIAN_POINT('Ctrl Pts',(-0.000879936119126035,-0.0367876398206301,
-0.00930488095683669));
#33037=CARTESIAN_POINT('Ctrl Pts',(-0.00100302097123913,-0.0367951908062692,
-0.00934553287137309));
#33038=CARTESIAN_POINT('Ctrl Pts',(-0.00134999711134431,-0.0368171583481161,
-0.00948561362835855));
#33039=CARTESIAN_POINT('Ctrl Pts',(-0.0015648898522476,-0.0368315395698085,
-0.00960465929852245));
#33040=CARTESIAN_POINT('Ctrl Pts',(-0.00179504554140822,-0.0368471591859041,
-0.00977181808903299));
#33041=CARTESIAN_POINT('Ctrl Pts',(-0.00182667875586705,-0.0368493142030486,
-0.00979576533585459));
#33042=CARTESIAN_POINT('Ctrl Pts',(-0.00187582820077025,-0.0368526767936784,
-0.00983453013964745));
#33043=CARTESIAN_POINT('Ctrl Pts',(-0.00189366464718435,-0.0368539001719131,
-0.00984893262602421));
#33044=CARTESIAN_POINT('Ctrl Pts',(-0.00192666654807844,-0.0368561700798597,
-0.0098762116423573));
#33045=CARTESIAN_POINT('Ctrl Pts',(-0.00194187230772095,-0.0368572185352222,
-0.00988903723687733));
#33046=CARTESIAN_POINT('Ctrl Pts',(-0.00197565860381956,-0.0368595545506384,
-0.0099181149559936));
#33047=CARTESIAN_POINT('Ctrl Pts',(-0.00199416848711677,-0.0368608387785798,
-0.00993444716980923));
#33048=CARTESIAN_POINT('Ctrl Pts',(-0.00204926890635601,-0.0368646770293317,
-0.00998428799926465));
#33049=CARTESIAN_POINT('Ctrl Pts',(-0.00208523267764469,-0.0368672029188704,
-0.0100184783792989));
#33050=CARTESIAN_POINT('Ctrl Pts',(-0.00226552429857299,-0.0368800087819219,
-0.0101986023311671));
#33051=CARTESIAN_POINT('Ctrl Pts',(-0.00239544736210209,-0.0368896788398055,
-0.0103581733530736));
#33052=CARTESIAN_POINT('Ctrl Pts',(-0.00259220574585257,-0.0369066939174307,
-0.0106579656236349));
#33053=CARTESIAN_POINT('Ctrl Pts',(-0.00266638302995268,-0.0369139999167096,
-0.010792413259548));
#33054=CARTESIAN_POINT('Ctrl Pts',(-0.00274229612521887,-0.0369233223798479,
-0.0109590138959835));
#33055=CARTESIAN_POINT('Ctrl Pts',(-0.00275423495015243,-0.036924856793475,
-0.010986283677699));
#33056=CARTESIAN_POINT('Ctrl Pts',(-0.00277126261280445,-0.0369271557259446,
-0.0110268080745781));
#33057=CARTESIAN_POINT('Ctrl Pts',(-0.00277666664411211,-0.0369279029398237,
-0.0110399291253249));
#33058=CARTESIAN_POINT('Ctrl Pts',(-0.0027861640698091,-0.0369292489992423,
-0.0110634617525319));
#33059=CARTESIAN_POINT('Ctrl Pts',(-0.00279029259871304,-0.0369298457964329,
-0.011073858570028));
#33060=CARTESIAN_POINT('Ctrl Pts',(-0.00279939131751406,-0.0369311875956844,
-0.0110971507181222));
#33061=CARTESIAN_POINT('Ctrl Pts',(-0.00280433057080931,-0.0369319342895694,
-0.0111100573330409));
#33062=CARTESIAN_POINT('Ctrl Pts',(-0.00281894963931801,-0.0369341994680632,
-0.0111490632400563));
#33063=CARTESIAN_POINT('Ctrl Pts',(-0.00282835530145968,-0.0369357324247709,
-0.0111752629362362));
#33064=CARTESIAN_POINT('Ctrl Pts',(-0.00287320611079789,-0.0369434185187938,
-0.0113058839811864));
#33065=CARTESIAN_POINT('Ctrl Pts',(-0.00290323726482158,-0.0369498004327213,
-0.0114120669032405));
#33066=CARTESIAN_POINT('Ctrl Pts',(-0.00297553762605092,-0.03696914222798,
-0.0117346034232676));
#33067=CARTESIAN_POINT('Ctrl Pts',(-0.00299990468521026,-0.0369821981326441,
-0.0119542272990632));
#33068=CARTESIAN_POINT('Ctrl Pts',(-0.00299999972093215,-0.0369945846061161,
-0.0121745592977555));
#33069=CARTESIAN_POINT('',(-0.0029999998192441,-0.0399949849792216,-0.0121748118762893));
#33070=CARTESIAN_POINT('Ctrl Pts',(-0.00299999972093215,-0.0369945846061161,
-0.0121745592977554));
#33071=CARTESIAN_POINT('Ctrl Pts',(-0.00300002044309324,-0.0369972854273804,
-0.0122226018135391));
#33072=CARTESIAN_POINT('Ctrl Pts',(-0.00299888744122127,-0.036999954978733,
-0.0122706295676167));
#33073=CARTESIAN_POINT('Ctrl Pts',(-0.00299499082230191,-0.0370044480830774,
-0.012352416913827));
#33074=CARTESIAN_POINT('Ctrl Pts',(-0.00299280903808429,-0.0370062877432467,
-0.0123861838072021));
#33075=CARTESIAN_POINT('Ctrl Pts',(-0.00298845331848487,-0.0370091714159223,
-0.0124395483674484));
#33076=CARTESIAN_POINT('Ctrl Pts',(-0.00298665668657259,-0.0370102268141541,
-0.0124591732365225));
#33077=CARTESIAN_POINT('Ctrl Pts',(-0.00298274368844551,-0.0370122905234387,
-0.0124977271901588));
#33078=CARTESIAN_POINT('Ctrl Pts',(-0.0029806401715497,-0.0370132991780978,
-0.0125166566183005));
#33079=CARTESIAN_POINT('Ctrl Pts',(-0.00297578076485031,-0.0370154337400218,
-0.0125568917393376));
#33080=CARTESIAN_POINT('Ctrl Pts',(-0.00297297599174496,-0.0370165580796817,
-0.012578190516932));
#33081=CARTESIAN_POINT('Ctrl Pts',(-0.0029651561954335,-0.0370194387258182,
-0.012633016070175));
#33082=CARTESIAN_POINT('Ctrl Pts',(-0.00295980119818566,-0.0370211844854742,
-0.0126664917065591));
#33083=CARTESIAN_POINT('Ctrl Pts',(-0.00293371205169528,-0.0370288041114952,
-0.0128135560272379));
#33084=CARTESIAN_POINT('Ctrl Pts',(-0.00290699715426476,-0.0370344929313124,
-0.0129259880337695));
#33085=CARTESIAN_POINT('Ctrl Pts',(-0.00282859361209651,-0.0370476857028708,
-0.0131877595939289));
#33086=CARTESIAN_POINT('Ctrl Pts',(-0.00277146896525616,-0.0370550638819975,
-0.013335101189664));
#33087=CARTESIAN_POINT('Ctrl Pts',(-0.00265315300429085,-0.037068102831315,
-0.0135808422605973));
#33088=CARTESIAN_POINT('Ctrl Pts',(-0.00259737631624408,-0.0370736802610889,
-0.0136814584216503));
#33089=CARTESIAN_POINT('Ctrl Pts',(-0.00252081613852199,-0.0370809905291002,
-0.013802595614908));
#33090=CARTESIAN_POINT('Ctrl Pts',(-0.00250532288371242,-0.0370824546846683,
-0.0138263567689643));
#33091=CARTESIAN_POINT('Ctrl Pts',(-0.00248172659690742,-0.0370846679180651,
-0.0138614472282185));
#33092=CARTESIAN_POINT('Ctrl Pts',(-0.00247387743128668,-0.0370854014986492,
-0.0138729461767796));
#33093=CARTESIAN_POINT('Ctrl Pts',(-0.00245957864348211,-0.0370867339378084,
-0.013893583766505));
#33094=CARTESIAN_POINT('Ctrl Pts',(-0.00245315757200238,-0.0370873309510449,
-0.0139027415352423));
#33095=CARTESIAN_POINT('Ctrl Pts',(-0.00243853728434795,-0.0370886873438808,
-0.0139233469712934));
#33096=CARTESIAN_POINT('Ctrl Pts',(-0.00243030863270394,-0.0370894486154127,
-0.013934772898004));
#33097=CARTESIAN_POINT('Ctrl Pts',(-0.00240477593244303,-0.0370918031743114,
-0.0139697052009798));
#33098=CARTESIAN_POINT('Ctrl Pts',(-0.00238720946407241,-0.0370934125854988,
-0.0139930166878927));
#33099=CARTESIAN_POINT('Ctrl Pts',(-0.00223219197604203,-0.0371074991872236,
-0.0141926042982427));
#33100=CARTESIAN_POINT('Ctrl Pts',(-0.00207578302806841,-0.0371208839489748,
-0.0143532566941638));
#33101=CARTESIAN_POINT('Ctrl Pts',(-0.0018205562500794,-0.0371401449311814,
-0.0145626807052035));
#33102=CARTESIAN_POINT('Ctrl Pts',(-0.00173457132032445,-0.0371462847788871,
-0.0146258809382894));
#33103=CARTESIAN_POINT('Ctrl Pts',(-0.00160560038026694,-0.0371549488219101,
-0.0147104760708857));
#33104=CARTESIAN_POINT('Ctrl Pts',(-0.00156518619011357,-0.0371575920287867,
-0.014735630184333));
#33105=CARTESIAN_POINT('Ctrl Pts',(-0.00149081407952689,-0.0371623270430561,
-0.0147794997362258));
#33106=CARTESIAN_POINT('Ctrl Pts',(-0.00145705986625813,-0.0371644295871248,
-0.014798538588036));
#33107=CARTESIAN_POINT('Ctrl Pts',(-0.00140313272875679,-0.0371677171758412,
-0.0148275932857108));
#33108=CARTESIAN_POINT('Ctrl Pts',(-0.00138320044839812,-0.0371689172351352,
-0.0148380446835801));
#33109=CARTESIAN_POINT('Ctrl Pts',(-0.00134538638621148,-0.0371711661406242,
-0.0148573329546732));
#33110=CARTESIAN_POINT('Ctrl Pts',(-0.00132753050291453,-0.0371722165903185,
-0.0148662176722987));
#33111=CARTESIAN_POINT('Ctrl Pts',(-0.00128682026186918,-0.0371745861967653,
-0.0148859702516155));
#33112=CARTESIAN_POINT('Ctrl Pts',(-0.00126391418380141,-0.0371759015780273,
-0.0148967283915958));
#33113=CARTESIAN_POINT('Ctrl Pts',(-0.00119265434133246,-0.0371799406994135,
-0.0149291024015441));
#33114=CARTESIAN_POINT('Ctrl Pts',(-0.00114386112634324,-0.037182631598501,
-0.0149497291333713));
#33115=CARTESIAN_POINT('Ctrl Pts',(-0.000880427758573214,-0.0371968095614718,
-0.0150529583010294));
#33116=CARTESIAN_POINT('Ctrl Pts',(-0.000657379722192128,-0.0372075190551629,
-0.0151119633160031));
#33117=CARTESIAN_POINT('Ctrl Pts',(-0.000338363856336814,-0.0372228871702796,
-0.0151581411054175));
#33118=CARTESIAN_POINT('Ctrl Pts',(-0.000246396792648505,-0.0372273338265884,
-0.0151671435738797));
#33119=CARTESIAN_POINT('Ctrl Pts',(-0.000101732598820027,-0.0372345380187635,
-0.0151745875303708));
#33120=CARTESIAN_POINT('Ctrl Pts',(-4.9239780400128E-5,-0.0372371954855935,
-0.0151759085239918));
#33121=CARTESIAN_POINT('Ctrl Pts',(2.08703028142546E-5,-0.0372408334751768,
-0.0151758323925362));
#33122=CARTESIAN_POINT('Ctrl Pts',(3.84820360315202E-5,-0.0372417548179085,
-0.0151756581652024));
#33123=CARTESIAN_POINT('Ctrl Pts',(6.77578217498163E-5,-0.0372433002521556,
-0.0151751107020802));
#33124=CARTESIAN_POINT('Ctrl Pts',(7.94233512608195E-5,-0.037243919733841,
-0.0151748244590345));
#33125=CARTESIAN_POINT('Ctrl Pts',(0.000103161117889949,-0.0372451882798842,
-0.0151741033940211));
#33126=CARTESIAN_POINT('Ctrl Pts',(0.000115232879814928,-0.0372458375703076,
-0.0151736637035798));
#33127=CARTESIAN_POINT('Ctrl Pts',(0.000146820030051706,-0.0372475468571941,
-0.0151723221319126));
#33128=CARTESIAN_POINT('Ctrl Pts',(0.000166329551303206,-0.0372486129221587,
-0.0151713025188336));
#33129=CARTESIAN_POINT('Ctrl Pts',(0.000250631803590922,-0.0372532601648237,
-0.0151660705880903));
#33130=CARTESIAN_POINT('Ctrl Pts',(0.000315284714862968,-0.0372569279704126,
-0.0151599461572649));
#33131=CARTESIAN_POINT('Ctrl Pts',(0.000545366834080181,-0.0372702371484968,
-0.0151305906431541));
#33132=CARTESIAN_POINT('Ctrl Pts',(0.000708992075988477,-0.0372801612482176,
-0.0150956524265341));
#33133=CARTESIAN_POINT('Ctrl Pts',(0.00102219420103656,-0.0372992835294335,
-0.0150008814363621));
#33134=CARTESIAN_POINT('Ctrl Pts',(0.00117158357947138,-0.0373084634288394,
-0.0149422712382416));
#33135=CARTESIAN_POINT('Ctrl Pts',(0.00135146440412296,-0.0373194516452926,
-0.014854497933067));
#33136=CARTESIAN_POINT('Ctrl Pts',(0.00138698451412708,-0.0373216193006787,
-0.0148362794446832));
#33137=CARTESIAN_POINT('Ctrl Pts',(0.0014421622064965,-0.0373249843645516,
-0.0148065729005021));
#33138=CARTESIAN_POINT('Ctrl Pts',(0.00146206977513875,-0.0373261980010782,
-0.0147955611954879));
#33139=CARTESIAN_POINT('Ctrl Pts',(0.00149916198486166,-0.0373284589626624,
-0.0147744894185091));
#33140=CARTESIAN_POINT('Ctrl Pts',(0.00151637536302494,-0.0373295080801955,
-0.0147644826897266));
#33141=CARTESIAN_POINT('Ctrl Pts',(0.00155491507616576,-0.037331857277806,
-0.0147415618848708));
#33142=CARTESIAN_POINT('Ctrl Pts',(0.00157618274298463,-0.0373331538500317,
-0.0147285517636009));
#33143=CARTESIAN_POINT('Ctrl Pts',(0.00163073857920877,-0.03733648197205,
-0.0146942363965434));
#33144=CARTESIAN_POINT('Ctrl Pts',(0.00166377281675525,-0.0373384992548174,
-0.0146725354843417));
#33145=CARTESIAN_POINT('Ctrl Pts',(0.00190972404152861,-0.0373535592438023,
-0.014503914698254));
#33146=CARTESIAN_POINT('Ctrl Pts',(0.00210325364473563,-0.0373655228288524,
-0.0143306715972191));
#33147=CARTESIAN_POINT('Ctrl Pts',(0.0023453447593637,-0.0373832651392373,
-0.0140498645242398));
#33148=CARTESIAN_POINT('Ctrl Pts',(0.00241370426447676,-0.037388711233053,
-0.0139609549110292));
#33149=CARTESIAN_POINT('Ctrl Pts',(0.0024927455841174,-0.0373958609720388,
-0.0138452860628398));
#33150=CARTESIAN_POINT('Ctrl Pts',(0.00250824069277282,-0.037397308889097,
-0.0138219136931857));
#33151=CARTESIAN_POINT('Ctrl Pts',(0.00253090100950291,-0.0373995022775469,
-0.0137866705232363));
#33152=CARTESIAN_POINT('Ctrl Pts',(0.00253831563468918,-0.037400232656178,
-0.0137749611046467));
#33153=CARTESIAN_POINT('Ctrl Pts',(0.00255156743641552,-0.0374015619777372,
-0.0137537090294394));
#33154=CARTESIAN_POINT('Ctrl Pts',(0.00255743273512644,-0.0374021591234302,
-0.0137441845411578));
#33155=CARTESIAN_POINT('Ctrl Pts',(0.00257059538114897,-0.0374035193023665,
-0.013722539914486));
#33156=CARTESIAN_POINT('Ctrl Pts',(0.00257786032128642,-0.0374042842779993,
-0.0137104008702787));
#33157=CARTESIAN_POINT('Ctrl Pts',(0.00260002822468843,-0.0374066618840454,
-0.0136727586730617));
#33158=CARTESIAN_POINT('Ctrl Pts',(0.00261464019585624,-0.0374082910782125,
-0.0136470871305454));
#33159=CARTESIAN_POINT('Ctrl Pts',(0.00270220658746547,-0.0374184262177816,
-0.0134878174700126));
#33160=CARTESIAN_POINT('Ctrl Pts',(0.00276527951816509,-0.0374273627007037,
-0.0133490510875615));
#33161=CARTESIAN_POINT('Ctrl Pts',(0.00288458392718222,-0.0374477836794666,
-0.0130227774474267));
#33162=CARTESIAN_POINT('Ctrl Pts',(0.002933575167356,-0.0374592043657586,
-0.0128333172933975));
#33163=CARTESIAN_POINT('Ctrl Pts',(0.00297266017997057,-0.037473260151968,
-0.0125839673303088));
#33164=CARTESIAN_POINT('Ctrl Pts',(0.00297989501878687,-0.037476396424312,
-0.0125272674231773));
#33165=CARTESIAN_POINT('Ctrl Pts',(0.00298806324686612,-0.0374808903773776,
-0.0124444727489461));
#33166=CARTESIAN_POINT('Ctrl Pts',(0.00299028280805924,-0.0374822869104341,
-0.0124185200714889));
#33167=CARTESIAN_POINT('Ctrl Pts',(0.00299361066697225,-0.0374847388873987,
-0.0123725668869731));
#33168=CARTESIAN_POINT('Ctrl Pts',(0.00299485715402919,-0.0374857985029798,
-0.0123525782677314));
#33169=CARTESIAN_POINT('Ctrl Pts',(0.00299705750808612,-0.0374880141205574,
-0.0123105170379525));
#33170=CARTESIAN_POINT('Ctrl Pts',(0.00299796790448567,-0.0374891687295452,
-0.0122884432973145));
#33171=CARTESIAN_POINT('Ctrl Pts',(0.00299974422656263,-0.0374922264601912,
-0.0122295915892838));
#33172=CARTESIAN_POINT('Ctrl Pts',(0.00300017767121487,-0.0374941163446732,
-0.0121928038145459));
#33173=CARTESIAN_POINT('Ctrl Pts',(0.00299880250555736,-0.037504692502762,
-0.0119848382545637));
#33174=CARTESIAN_POINT('Ctrl Pts',(0.00298302146881439,-0.0375129412064582,
-0.0118140605827843));
#33175=CARTESIAN_POINT('Ctrl Pts',(0.00292980333788672,-0.0375272513084608,
-0.0115177380114177));
#33176=CARTESIAN_POINT('Ctrl Pts',(0.00289857466076249,-0.0375333522074619,
-0.011391553369944));
#33177=CARTESIAN_POINT('Ctrl Pts',(0.00283083713085173,-0.037544181788,
-0.0111782636316869));
#33178=CARTESIAN_POINT('Ctrl Pts',(0.00279821676528967,-0.0375488192113112,
-0.0110901258412438));
#33179=CARTESIAN_POINT('Ctrl Pts',(0.00275329122241311,-0.0375547481661455,
-0.0109842867149117));
#33180=CARTESIAN_POINT('Ctrl Pts',(0.00274485953352157,-0.0375558442465599,
-0.0109649901466173));
#33181=CARTESIAN_POINT('Ctrl Pts',(0.00273113664496737,-0.0375576046980961,
-0.0109344642778422));
#33182=CARTESIAN_POINT('Ctrl Pts',(0.00272597754827251,-0.0375582615292014,
-0.0109231759777802));
#33183=CARTESIAN_POINT('Ctrl Pts',(0.002715970479512,-0.0375595267206954,
-0.0109016347115573));
#33184=CARTESIAN_POINT('Ctrl Pts',(0.00271113419474063,-0.0375601344054861,
-0.0108913767451032));
#33185=CARTESIAN_POINT('Ctrl Pts',(0.00269912675937915,-0.0375616336472831,
-0.0108662783933782));
#33186=CARTESIAN_POINT('Ctrl Pts',(0.00269189128805988,-0.0375625289554351,
-0.0108514693041431));
#33187=CARTESIAN_POINT('Ctrl Pts',(0.00266630623366604,-0.0375656651415887,
-0.0108001794102768));
#33188=CARTESIAN_POINT('Ctrl Pts',(0.00264733478122021,-0.0375679390852926,
-0.0107640155522906));
#33189=CARTESIAN_POINT('Ctrl Pts',(0.00250100657200337,-0.0375850491183667,
-0.0104984060320765));
#33190=CARTESIAN_POINT('Ctrl Pts',(0.00234477208838719,-0.0376008994558459,
-0.0102861651716031));
#33191=CARTESIAN_POINT('Ctrl Pts',(0.00208695424460772,-0.037622243702121,
-0.0100179295092302));
#33192=CARTESIAN_POINT('Ctrl Pts',(0.00200672343028683,-0.0376283958452394,
-0.00994312444017302));
#33193=CARTESIAN_POINT('Ctrl Pts',(0.00189753733051129,-0.037636145131618,
-0.00985197387956283));
#33194=CARTESIAN_POINT('Ctrl Pts',(0.00187216413263985,-0.0376379058075873,
-0.0098314845030936));
#33195=CARTESIAN_POINT('Ctrl Pts',(0.00182974225931127,-0.0376407850343264,
-0.00979835601947079));
#33196=CARTESIAN_POINT('Ctrl Pts',(0.00181288502435536,-0.0376419128484175,
-0.00978547718433662));
#33197=CARTESIAN_POINT('Ctrl Pts',(0.00177975583463052,-0.0376440982712655,
-0.00976071871862555));
#33198=CARTESIAN_POINT('Ctrl Pts',(0.00176349805428186,-0.0376451564975836,
-0.00974882208551559));
#33199=CARTESIAN_POINT('Ctrl Pts',(0.00172423940507011,-0.0376476786356387,
-0.00972069732877153));
#33200=CARTESIAN_POINT('Ctrl Pts',(0.00170112735470768,-0.0376491365779514,
-0.0097046272558229));
#33201=CARTESIAN_POINT('Ctrl Pts',(0.00162377641072108,-0.0376539310241366,
-0.00965244373114894));
#33202=CARTESIAN_POINT('Ctrl Pts',(0.00156858583977075,-0.0376572154170436,
-0.00961777103012518));
#33203=CARTESIAN_POINT('Ctrl Pts',(0.00132601850555366,-0.0376711479922775,
-0.00947618631205751));
#33204=CARTESIAN_POINT('Ctrl Pts',(0.00112855205184552,-0.0376811848038427,
-0.00938786133563327));
#33205=CARTESIAN_POINT('Ctrl Pts',(0.000839021764853071,-0.0376957123064264,
-0.00929420590120984));
#33206=CARTESIAN_POINT('Ctrl Pts',(0.000753564249706857,-0.0376999868228641,
-0.00927068746040749));
#33207=CARTESIAN_POINT('Ctrl Pts',(0.00061734691175093,-0.0377069437191662,
-0.00923961469493174));
#33208=CARTESIAN_POINT('Ctrl Pts',(0.000567217490811083,-0.0377095341475461,
-0.00922952030581138));
#33209=CARTESIAN_POINT('Ctrl Pts',(0.000499671268170587,-0.0377130934865716,
-0.00921770639638369));
#33210=CARTESIAN_POINT('Ctrl Pts',(0.000482459589042077,-0.0377140064137885,
-0.00921485056501733));
#33211=CARTESIAN_POINT('Ctrl Pts',(0.000453729411853558,-0.0377155416462878,
-0.00921034068145948));
#33212=CARTESIAN_POINT('Ctrl Pts',(0.000442224153176486,-0.0377161594717798,
-0.00920860318178661));
#33213=CARTESIAN_POINT('Ctrl Pts',(0.000418708128923782,-0.0377174289485115,
-0.00920519165008405));
#33214=CARTESIAN_POINT('Ctrl Pts',(0.000406696870285474,-0.0377180808731861,
-0.00920352344263359));
#33215=CARTESIAN_POINT('Ctrl Pts',(0.000375096833428594,-0.037719804637521,
-0.00919932973339328));
#33216=CARTESIAN_POINT('Ctrl Pts',(0.00035549295112039,-0.0377208827259958,
-0.0091969248184984));
#33217=CARTESIAN_POINT('Ctrl Pts',(0.000269027170829223,-0.0377256718604464,
-0.00918718323297989));
#33218=CARTESIAN_POINT('Ctrl Pts',(0.000201956959841878,-0.0377294759985951,
-0.00918190330559078));
#33219=CARTESIAN_POINT('Ctrl Pts',(-3.0407849027876E-5,-0.0377428396741294,
-0.00917145408906216));
#33220=CARTESIAN_POINT('Ctrl Pts',(-0.000195914849611807,-0.0377526626329514,
-0.00917769456514838));
#33221=CARTESIAN_POINT('Ctrl Pts',(-0.000470297970778056,-0.0377688102072291,
-0.00921086606483261));
#33222=CARTESIAN_POINT('Ctrl Pts',(-0.000579714920712568,-0.0377752165082834,
-0.00923030354177732));
#33223=CARTESIAN_POINT('Ctrl Pts',(-0.00075755950619684,-0.0377854921212332,
-0.00927219377045805));
#33224=CARTESIAN_POINT('Ctrl Pts',(-0.000826702041539106,-0.0377894531243794,
-0.00929111761568895));
#33225=CARTESIAN_POINT('Ctrl Pts',(-0.000922142781441596,-0.0377948723204791,
-0.00932095307942868));
#33226=CARTESIAN_POINT('Ctrl Pts',(-0.000949060428788879,-0.0377963953640786,
-0.00932978812936573));
#33227=CARTESIAN_POINT('Ctrl Pts',(-0.000995119084197374,-0.0377989929058438,
-0.00934563187099686));
#33228=CARTESIAN_POINT('Ctrl Pts',(-0.00101432089647831,-0.0378000732444643,
-0.00935245667976048));
#33229=CARTESIAN_POINT('Ctrl Pts',(-0.0010510007034363,-0.0378021324395794,
-0.00936591610863203));
#33230=CARTESIAN_POINT('Ctrl Pts',(-0.00106848908562557,-0.0378031122532645,
-0.0093725194646185));
#33231=CARTESIAN_POINT('Ctrl Pts',(-0.00111426458223233,-0.0378056722919803,
-0.00939029421720802));
#33232=CARTESIAN_POINT('Ctrl Pts',(-0.00114244588364151,-0.0378072436855356,
-0.00940173317791727));
#33233=CARTESIAN_POINT('Ctrl Pts',(-0.00124471550365131,-0.0378129337398839,
-0.00944506784794806));
#33234=CARTESIAN_POINT('Ctrl Pts',(-0.00131768583698017,-0.0378169682643452,
-0.00947952037346398));
#33235=CARTESIAN_POINT('Ctrl Pts',(-0.00156723723700532,-0.0378307971921275,
-0.00960989843765308));
#33236=CARTESIAN_POINT('Ctrl Pts',(-0.00173549288162418,-0.0378401429586102,
-0.00972056882622447));
#33237=CARTESIAN_POINT('Ctrl Pts',(-0.00198009706791911,-0.0378552118975698,
-0.00991924846681959));
#33238=CARTESIAN_POINT('Ctrl Pts',(-0.00206457454301919,-0.0378607565391,
-0.00999627135374706));
#33239=CARTESIAN_POINT('Ctrl Pts',(-0.00216422795614718,-0.0378680267272226,
-0.0100981340055179));
#33240=CARTESIAN_POINT('Ctrl Pts',(-0.00218372060427283,-0.0378694868556049,
-0.0101186308215999));
#33241=CARTESIAN_POINT('Ctrl Pts',(-0.00221236016960907,-0.0378716951686239,
-0.0101496114736076));
#33242=CARTESIAN_POINT('Ctrl Pts',(-0.00222172918579084,-0.0378724279567887,
-0.0101598887990773));
#33243=CARTESIAN_POINT('Ctrl Pts',(-0.00223850401260117,-0.037873759621071,
-0.0101785488793524));
#33244=CARTESIAN_POINT('Ctrl Pts',(-0.0022459348551604,-0.0378743566637337,
-0.0101869084087238));
#33245=CARTESIAN_POINT('Ctrl Pts',(-0.00226262538298555,-0.0378757139789977,
-0.0102058976782667));
#33246=CARTESIAN_POINT('Ctrl Pts',(-0.00227185695899828,-0.0378764761558808,
-0.01021655120047));
#33247=CARTESIAN_POINT('Ctrl Pts',(-0.00230002711983631,-0.0378788363362719,
-0.0102495271960145));
#33248=CARTESIAN_POINT('Ctrl Pts',(-0.00231871382895359,-0.0378804505703915,
-0.0102720615401041));
#33249=CARTESIAN_POINT('Ctrl Pts',(-0.00243922423081966,-0.037891165131394,
-0.0104217918058745));
#33250=CARTESIAN_POINT('Ctrl Pts',(-0.00253086451726537,-0.0379007601187622,
-0.0105568214346169));
#33251=CARTESIAN_POINT('Ctrl Pts',(-0.0026513271363398,-0.0379151398042545,
-0.0107697438117327));
#33252=CARTESIAN_POINT('Ctrl Pts',(-0.00268864846269303,-0.0379199360982675,
-0.0108424930478021));
#33253=CARTESIAN_POINT('Ctrl Pts',(-0.00277736852592235,-0.0379322019982186,
-0.0110343490997371));
#33254=CARTESIAN_POINT('Ctrl Pts',(-0.00282410316489579,-0.037939572177499,
-0.0111554341335098));
#33255=CARTESIAN_POINT('Ctrl Pts',(-0.00287497631173254,-0.0379489218076826,
-0.0113178588574153));
#33256=CARTESIAN_POINT('Ctrl Pts',(-0.00288630754296669,-0.0379511242289986,
-0.0113567853906999));
#33257=CARTESIAN_POINT('Ctrl Pts',(-0.00290279455745963,-0.0379545305932805,
-0.0114180227124528));
#33258=CARTESIAN_POINT('Ctrl Pts',(-0.0029084895529716,-0.0379557514279185,
-0.0114401821771386));
#33259=CARTESIAN_POINT('Ctrl Pts',(-0.00291866219870402,-0.0379580189776256,
-0.0114817302279686));
#33260=CARTESIAN_POINT('Ctrl Pts',(-0.00292320149540094,-0.0379590675837491,
-0.011501102300451));
#33261=CARTESIAN_POINT('Ctrl Pts',(-0.00293295352853091,-0.0379614069315476,
-0.0115446671166774));
#33262=CARTESIAN_POINT('Ctrl Pts',(-0.00293806033987555,-0.0379626942964263,
-0.0115688822261031));
#33263=CARTESIAN_POINT('Ctrl Pts',(-0.00295042051231099,-0.0379659814071533,
-0.0116313065490464));
#33264=CARTESIAN_POINT('Ctrl Pts',(-0.00295723168769888,-0.0379679674894826,
-0.0116695991348617));
#33265=CARTESIAN_POINT('Ctrl Pts',(-0.00300413471564091,-0.0379831666217663,
-0.0119666834664119));
#33266=CARTESIAN_POINT('Ctrl Pts',(-0.00301092898457304,-0.0379952659165436,
-0.0122295706366045));
#33267=CARTESIAN_POINT('Ctrl Pts',(-0.00297194724054524,-0.0380130907312578,
-0.0125997792812104));
#33268=CARTESIAN_POINT('Ctrl Pts',(-0.0029543398689143,-0.0380184595843295,
-0.0127088220121337));
#33269=CARTESIAN_POINT('Ctrl Pts',(-0.00292481886294813,-0.0380255149297125,
-0.0128438429341274));
#33270=CARTESIAN_POINT('Ctrl Pts',(-0.00291849219275542,-0.0380269531610892,
-0.0128709639012601));
#33271=CARTESIAN_POINT('Ctrl Pts',(-0.00290846198336515,-0.0380291347061286,
-0.0129114074567973));
#33272=CARTESIAN_POINT('Ctrl Pts',(-0.00290504225315914,-0.0380298631659172,
-0.012924799572219));
#33273=CARTESIAN_POINT('Ctrl Pts',(-0.00289868750565138,-0.0380311906359535,
-0.0129489870996352));
#33274=CARTESIAN_POINT('Ctrl Pts',(-0.00289578448739946,-0.0380317878778922,
-0.0129597903641244));
#33275=CARTESIAN_POINT('Ctrl Pts',(-0.00288906260805417,-0.0380331503993545,
-0.0129842582231015));
#33276=CARTESIAN_POINT('Ctrl Pts',(-0.0028852072065392,-0.0380339176522124,
-0.0129979120764626));
#33277=CARTESIAN_POINT('Ctrl Pts',(-0.00287296677832843,-0.0380363094934002,
-0.0130401143631185));
#33278=CARTESIAN_POINT('Ctrl Pts',(-0.00286425399823239,-0.0380379509200457,
-0.013068565009904));
#33279=CARTESIAN_POINT('Ctrl Pts',(-0.00280996833975091,-0.0380478133513822,
-0.0132368467884605));
#33280=CARTESIAN_POINT('Ctrl Pts',(-0.00275458874533698,-0.038056434931989,
-0.01337329385379));
#33281=CARTESIAN_POINT('Ctrl Pts',(-0.00264728509805603,-0.0380706686341365,
-0.0135903956917944));
#33282=CARTESIAN_POINT('Ctrl Pts',(-0.00260110350078717,-0.0380762629662318,
-0.0136736216504018));
#33283=CARTESIAN_POINT('Ctrl Pts',(-0.00248210666811348,-0.0380893915027212,
-0.0138659151507224));
#33284=CARTESIAN_POINT('Ctrl Pts',(-0.00240594005634628,-0.0380968430181555,
-0.0139726897951731));
#33285=CARTESIAN_POINT('Ctrl Pts',(-0.00229725377369942,-0.0381062799918662,
-0.0141056937700087));
#33286=CARTESIAN_POINT('Ctrl Pts',(-0.00227083867429439,-0.038108493388957,
-0.014136707979788));
#33287=CARTESIAN_POINT('Ctrl Pts',(-0.00222858609876653,-0.0381119127829061,
-0.0141843176970745));
#33288=CARTESIAN_POINT('Ctrl Pts',(-0.00221317673944085,-0.0381131358831869,
-0.0142012851040353));
#33289=CARTESIAN_POINT('Ctrl Pts',(-0.00218403275149779,-0.0381154055340991,
-0.0142326460906157));
#33290=CARTESIAN_POINT('Ctrl Pts',(-0.00217034654364241,-0.0381164540065879,
-0.0142470827775327));
#33291=CARTESIAN_POINT('Ctrl Pts',(-0.00213935320174369,-0.0381187903874408,
-0.0142791310866967));
#33292=CARTESIAN_POINT('Ctrl Pts',(-0.00212197009664199,-0.0381200749588172,
-0.0142966674185424));
#33293=CARTESIAN_POINT('Ctrl Pts',(-0.00207679152586123,-0.0381233496544202,
-0.0143411325998502));
#33294=CARTESIAN_POINT('Ctrl Pts',(-0.00204868754421004,-0.0381253262954874,
-0.014367742212188));
#33295=CARTESIAN_POINT('Ctrl Pts',(-0.00185590655526666,-0.0381385062048197,
-0.0145433244082964));
#33296=CARTESIAN_POINT('Ctrl Pts',(-0.00167564669943691,-0.0381489445459278,
-0.0146741576283947));
#33297=CARTESIAN_POINT('Ctrl Pts',(-0.00138759235799904,-0.0381646762826408,
-0.0148379065620802));
#33298=CARTESIAN_POINT('Ctrl Pts',(-0.00128972269425873,-0.038169890963357,
-0.0148866747598141));
#33299=CARTESIAN_POINT('Ctrl Pts',(-0.00113597550791388,-0.0381781807261722,
-0.014953072817688));
#33300=CARTESIAN_POINT('Ctrl Pts',(-0.00108187647986248,-0.0381811158805767,
-0.0149745907096343));
#33301=CARTESIAN_POINT('Ctrl Pts',(-0.00101003612252503,-0.0381850784681157,
-0.0150007710434108));
#33302=CARTESIAN_POINT('Ctrl Pts',(-0.000992826780230872,-0.038186032518885,
-0.0150068651647332));
#33303=CARTESIAN_POINT('Ctrl Pts',(-0.000964401817901725,-0.0381876178596878,
-0.015016639875531));
#33304=CARTESIAN_POINT('Ctrl Pts',(-0.00095321793925728,-0.0381882440256238,
-0.0150204121034411));
#33305=CARTESIAN_POINT('Ctrl Pts',(-0.000930697826041185,-0.0381895102537011,
-0.0150278602247926));
#33306=CARTESIAN_POINT('Ctrl Pts',(-0.00091936139598845,-0.0381901503697621,
-0.0150315347521498));
#33307=CARTESIAN_POINT('Ctrl Pts',(-0.000890097351650106,-0.0381918091841625,
-0.0150408279237655));
#33308=CARTESIAN_POINT('Ctrl Pts',(-0.000872138556095567,-0.0381928333369005,
-0.0150463458001818));
#33309=CARTESIAN_POINT('Ctrl Pts',(-0.000798881986234456,-0.0381970326494137,
-0.0150681031221734));
#33310=CARTESIAN_POINT('Ctrl Pts',(-0.000743176224571877,-0.0382002756647244,
-0.015082915349514));
#33311=CARTESIAN_POINT('Ctrl Pts',(-0.000519219071816896,-0.0382134201201707,
-0.0151356082420127));
#33312=CARTESIAN_POINT('Ctrl Pts',(-0.000348267692692032,-0.0382236699510084,
-0.0151605552173447));
#33313=CARTESIAN_POINT('Ctrl Pts',(-1.28885291828755E-5,-0.0382433151825151,
-0.0151802786561979));
#33314=CARTESIAN_POINT('Ctrl Pts',(0.000150874798862594,-0.0382526940326813,
-0.0151765176658144));
#33315=CARTESIAN_POINT('Ctrl Pts',(0.000353269772085546,-0.0382638669440909,
-0.0151552486787805));
#33316=CARTESIAN_POINT('Ctrl Pts',(0.000392920194550312,-0.0382660368777107,
-0.0151502793427568));
#33317=CARTESIAN_POINT('Ctrl Pts',(0.000454980648122617,-0.0382694046483831,
-0.0151412386768143));
#33318=CARTESIAN_POINT('Ctrl Pts',(0.000477462777156135,-0.0382706187566624,
-0.0151377019048761));
#33319=CARTESIAN_POINT('Ctrl Pts',(0.000519533418745883,-0.03827288014437,
-0.0151305920887756));
#33320=CARTESIAN_POINT('Ctrl Pts',(0.00053913071657834,-0.0382739292227878,
-0.0151270792112145));
#33321=CARTESIAN_POINT('Ctrl Pts',(0.000583173594536535,-0.0382762777493693,
-0.0151187310354264));
#33322=CARTESIAN_POINT('Ctrl Pts',(0.000607596965225421,-0.0382775736985255,
-0.0151137856993893));
#33323=CARTESIAN_POINT('Ctrl Pts',(0.000670547487576641,-0.0382808990435796,
-0.0151002206531614));
#33324=CARTESIAN_POINT('Ctrl Pts',(0.000708971722641221,-0.0382829142136489,
-0.0150911436158416));
#33325=CARTESIAN_POINT('Ctrl Pts',(0.000997947248644278,-0.0382979837337265,
-0.0150168267535087));
#33326=CARTESIAN_POINT('Ctrl Pts',(0.00123927253768217,-0.0383099566142507,
-0.0149201627607569));
#33327=CARTESIAN_POINT('Ctrl Pts',(0.00156289130452094,-0.0383277045138112,
-0.0147390358303782));
#33328=CARTESIAN_POINT('Ctrl Pts',(0.00165744085573282,-0.0383331452782901,
-0.0146789353326539));
#33329=CARTESIAN_POINT('Ctrl Pts',(0.00177117902580598,-0.038340288503813,
-0.0145973632402221));
#33330=CARTESIAN_POINT('Ctrl Pts',(0.00179372460252557,-0.0383417357548207,
-0.0145807103594571));
#33331=CARTESIAN_POINT('Ctrl Pts',(0.00182706247315057,-0.0383439283282149,
-0.0145553563306604));
#33332=CARTESIAN_POINT('Ctrl Pts',(0.00183803371714259,-0.0383446585742784,
-0.0145468918897105));
#33333=CARTESIAN_POINT('Ctrl Pts',(0.00185775475092044,-0.0383459877658143,
-0.0145314577554535));
#33334=CARTESIAN_POINT('Ctrl Pts',(0.00186652472745447,-0.0383465849160221,
-0.0145245147268607));
#33335=CARTESIAN_POINT('Ctrl Pts',(0.00188630045166375,-0.0383479452485527,
-0.0145086779308926));
#33336=CARTESIAN_POINT('Ctrl Pts',(0.00189728219272437,-0.0383487103753437,
-0.0144997552811555));
#33337=CARTESIAN_POINT('Ctrl Pts',(0.00193100401168371,-0.0383510889321497,
-0.0144719580023355));
#33338=CARTESIAN_POINT('Ctrl Pts',(0.00195352801886612,-0.0383527189442987,
-0.0144528252913142));
#33339=CARTESIAN_POINT('Ctrl Pts',(0.00208997361415517,-0.0383628301454171,
-0.014333408604781));
#33340=CARTESIAN_POINT('Ctrl Pts',(0.00219642458859821,-0.038371739263382,
-0.0142249377524926));
#33341=CARTESIAN_POINT('Ctrl Pts',(0.00235312967283044,-0.0383860349905313,
-0.0140389539007192));
#33342=CARTESIAN_POINT('Ctrl Pts',(0.00240882810348608,-0.0383914099590158,
-0.0139663591219473));
#33343=CARTESIAN_POINT('Ctrl Pts',(0.00253571217344898,-0.0384042896785454,
-0.013784323934531));
#33344=CARTESIAN_POINT('Ctrl Pts',(0.00260324776088318,-0.038411707240564,
-0.0136725568138752));
#33345=CARTESIAN_POINT('Ctrl Pts',(0.00268201036428155,-0.0384211077693719,
-0.0135206480449679));
#33346=CARTESIAN_POINT('Ctrl Pts',(0.00269998709514019,-0.0384233165952397,
-0.0134841813957939));
#33347=CARTESIAN_POINT('Ctrl Pts',(0.00272692448824798,-0.0384267305617329,
-0.0134266159918156));
#33348=CARTESIAN_POINT('Ctrl Pts',(0.00273639356015427,-0.0384279527175141,
-0.01340576175171));
#33349=CARTESIAN_POINT('Ctrl Pts',(0.00275363988920776,-0.0384302214888551,
-0.0133665938626722));
#33350=CARTESIAN_POINT('Ctrl Pts',(0.00276147552375389,-0.0384312700134707,
-0.0133483074289872));
#33351=CARTESIAN_POINT('Ctrl Pts',(0.00277863606857027,-0.0384336076164033,
-0.0133071323687479));
#33352=CARTESIAN_POINT('Ctrl Pts',(0.00278786125751644,-0.0384348933412666,
-0.0132842036009561));
#33353=CARTESIAN_POINT('Ctrl Pts',(0.00281083059315546,-0.0384381731661011,
-0.0132250124882865));
#33354=CARTESIAN_POINT('Ctrl Pts',(0.00282415708452435,-0.0384401537084813,
-0.0131885924368582));
#33355=CARTESIAN_POINT('Ctrl Pts',(0.0029087266652231,-0.0384532907482815,
-0.0129428059397929));
#33356=CARTESIAN_POINT('Ctrl Pts',(0.00295733651518357,-0.0384636897262207,
-0.01272637643387));
#33357=CARTESIAN_POINT('Ctrl Pts',(0.00299382221118458,-0.0384794029121674,
-0.0123974111947451));
#33358=CARTESIAN_POINT('Ctrl Pts',(0.00299992494541448,-0.0384846421759763,
-0.0122876885680689));
#33359=CARTESIAN_POINT('Ctrl Pts',(0.00300003817796209,-0.0384929168377875,
-0.0121204987763927));
#33360=CARTESIAN_POINT('Ctrl Pts',(0.00299843043573469,-0.038495809124339,
-0.012063126393098));
#33361=CARTESIAN_POINT('Ctrl Pts',(0.00299411551288363,-0.0384997512260852,
-0.0119871095017452));
#33362=CARTESIAN_POINT('Ctrl Pts',(0.00299287675335369,-0.0385007308112597,
-0.0119683909390974));
#33363=CARTESIAN_POINT('Ctrl Pts',(0.00299056458162604,-0.0385023475237244,
-0.0119378084189421));
#33364=CARTESIAN_POINT('Ctrl Pts',(0.00298959589558238,-0.0385029791164709,
-0.0119259368058963));
#33365=CARTESIAN_POINT('Ctrl Pts',(0.00298752611668686,-0.0385042447654798,
-0.0119023077716062));
#33366=CARTESIAN_POINT('Ctrl Pts',(0.00298642624939588,-0.0385048787493831,
-0.0118905504776998));
#33367=CARTESIAN_POINT('Ctrl Pts',(0.00298344667560644,-0.038506503615628,
-0.0118606070286782));
#33368=CARTESIAN_POINT('Ctrl Pts',(0.00298147010031703,-0.0385074995524286,
-0.0118424312156196));
#33369=CARTESIAN_POINT('Ctrl Pts',(0.00297247650210088,-0.038511712887228,
-0.0117662180915147));
#33370=CARTESIAN_POINT('Ctrl Pts',(0.00296393030013996,-0.0385150012420553,
-0.0117083772068289));
#33371=CARTESIAN_POINT('Ctrl Pts',(0.0029344403410876,-0.0385246272079108,
-0.0115424722609411));
#33372=CARTESIAN_POINT('Ctrl Pts',(0.00290923312333203,-0.0385310845282925,
-0.0114352641599816));
#33373=CARTESIAN_POINT('Ctrl Pts',(0.00281593822788839,-0.0385505263554746,
-0.0111179254418827));
#33374=CARTESIAN_POINT('Ctrl Pts',(0.00273049172443464,-0.0385634283098509,
-0.0109136482570906));
#33375=CARTESIAN_POINT('Ctrl Pts',(0.00260456342050484,-0.0385777217191394,
-0.0106866401861755));
#33376=CARTESIAN_POINT('Ctrl Pts',(0.0025850793150576,-0.0385798365196836,
-0.010653069193299));
#33377=CARTESIAN_POINT('Ctrl Pts',(0.0025521255816362,-0.0385832611598833,
-0.0105987463552682));
#33378=CARTESIAN_POINT('Ctrl Pts',(0.00253904146004677,-0.0385845844127943,
-0.0105777670026649));
#33379=CARTESIAN_POINT('Ctrl Pts',(0.00251496343622294,-0.0385869555834838,
-0.010540202129362));
#33380=CARTESIAN_POINT('Ctrl Pts',(0.00250406114513512,-0.0385880067320656,
-0.0105235598500129));
#33381=CARTESIAN_POINT('Ctrl Pts',(0.00248025784800593,-0.0385902546063497,
-0.0104880010413813));
#33382=CARTESIAN_POINT('Ctrl Pts',(0.00246730415786335,-0.0385914493041666,
-0.010469121197277));
#33383=CARTESIAN_POINT('Ctrl Pts',(0.00243077399012196,-0.0385947417312756,
-0.0104171641161299));
#33384=CARTESIAN_POINT('Ctrl Pts',(0.00240673957702643,-0.0385968222861442,
-0.0103844140338685));
#33385=CARTESIAN_POINT('Ctrl Pts',(0.00230289525315512,-0.0386054758775297,
-0.0102487759939204));
#33386=CARTESIAN_POINT('Ctrl Pts',(0.00221709284449092,-0.0386118197773989,
-0.0101506478682194));
#33387=CARTESIAN_POINT('Ctrl Pts',(0.00206224495969223,-0.0386223217727025,
-0.00999523494514102));
#33388=CARTESIAN_POINT('Ctrl Pts',(0.00199652444888733,-0.0386265354076054,
-0.00993490683747034));
#33389=CARTESIAN_POINT('Ctrl Pts',(0.00181013109120773,-0.0386380794596843,
-0.00977852475355941));
#33390=CARTESIAN_POINT('Ctrl Pts',(0.00168459870079932,-0.0386454212204768,
-0.00968871096250319));
#33391=CARTESIAN_POINT('Ctrl Pts',(0.00152732877733873,-0.0386547814237194,
-0.00959357742562413));
#33392=CARTESIAN_POINT('Ctrl Pts',(0.00150169444234515,-0.0386563121970781,
-0.00957858635902542));
#33393=CARTESIAN_POINT('Ctrl Pts',(0.00146350008988871,-0.0386586066976584,
-0.0095570045953262));
#33394=CARTESIAN_POINT('Ctrl Pts',(0.00145110840548118,-0.0386593532160095,
-0.00955011808274345));
#33395=CARTESIAN_POINT('Ctrl Pts',(0.00142885222449578,-0.0386606985661463,
-0.00953795517227716));
#33396=CARTESIAN_POINT('Ctrl Pts',(0.00141900638169355,-0.038661295359854,
-0.0095326457611751));
#33397=CARTESIAN_POINT('Ctrl Pts',(0.00139691971816581,-0.0386626378407869,
-0.0095208944121656));
#33398=CARTESIAN_POINT('Ctrl Pts',(0.00138466400744241,-0.0386633852294527,
-0.00951448204312785));
#33399=CARTESIAN_POINT('Ctrl Pts',(0.00134755456317872,-0.0386656546466079,
-0.0094953915466785));
#33400=CARTESIAN_POINT('Ctrl Pts',(0.0013225685018813,-0.038667191223888,
-0.00948297547858484));
#33401=CARTESIAN_POINT('Ctrl Pts',(0.00119748217814813,-0.0386749126413374,
-0.00942297838613298));
#33402=CARTESIAN_POINT('Ctrl Pts',(0.00109497828094512,-0.0386813284494651,
-0.00938062474162731));
#33403=CARTESIAN_POINT('Ctrl Pts',(0.000744042790804974,-0.0387030860675511,
-0.00925789132101391));
#33404=CARTESIAN_POINT('Ctrl Pts',(0.000487470579661229,-0.0387185349053377,
-0.00920423463305956));
#33405=CARTESIAN_POINT('Ctrl Pts',(0.00018822610378376,-0.0387350628504217,
-0.00918150917919925));
#33406=CARTESIAN_POINT('Ctrl Pts',(0.000149222848675907,-0.0387371916534693,
-0.0091793122081576));
#33407=CARTESIAN_POINT('Ctrl Pts',(8.54070832880134E-5,-0.0387406340826542,
-0.00917696674648536));
#33408=CARTESIAN_POINT('Ctrl Pts',(6.06168239286941E-5,-0.0387419613584356,
-0.00917636324646113));
#33409=CARTESIAN_POINT('Ctrl Pts',(1.59234775696302E-5,-0.0387443368416078,
-0.00917582954878122));
#33410=CARTESIAN_POINT('Ctrl Pts',(-3.97663950225589E-6,-0.0387453883316623,
-0.00917578992119837));
#33411=CARTESIAN_POINT('Ctrl Pts',(-4.67173719602617E-5,-0.0387476338483137,
-0.00917613009128741));
#33412=CARTESIAN_POINT('Ctrl Pts',(-6.95563115034423E-5,-0.038748825887186,
-0.00917657275312798));
#33413=CARTESIAN_POINT('Ctrl Pts',(-0.000132732048396999,-0.0387521027168052,
-0.00917851924458077));
#33414=CARTESIAN_POINT('Ctrl Pts',(-0.000173047625683019,-0.0387541706077786,
-0.00918057635945556));
#33415=CARTESIAN_POINT('Ctrl Pts',(-0.000406993128765488,-0.0387660547152393,
-0.00919725292670068));
#33416=CARTESIAN_POINT('Ctrl Pts',(-0.000598880785348187,-0.0387753021225477,
-0.00922982987934081));
#33417=CARTESIAN_POINT('Ctrl Pts',(-0.000962051909960035,-0.0387931437202054,
-0.00932846365032878));
#33418=CARTESIAN_POINT('Ctrl Pts',(-0.00113308553822213,-0.0388017195433591,
-0.00939210132974085));
#33419=CARTESIAN_POINT('Ctrl Pts',(-0.00132277308792866,-0.0388124524766794,
-0.00948307198145786));
#33420=CARTESIAN_POINT('Ctrl Pts',(-0.00134809790753585,-0.0388139123763085,
-0.00949566080804657));
#33421=CARTESIAN_POINT('Ctrl Pts',(-0.00138560366985646,-0.038816120403891,
-0.0095149707550036));
#33422=CARTESIAN_POINT('Ctrl Pts',(-0.00139792260213483,-0.0388168531407309,
-0.00952142194251254));
#33423=CARTESIAN_POINT('Ctrl Pts',(-0.00142006828334926,-0.0388181847446295,
-0.00953321612340705));
#33424=CARTESIAN_POINT('Ctrl Pts',(-0.00142991060176433,-0.0388187817788467,
-0.0095385287392919));
#33425=CARTESIAN_POINT('Ctrl Pts',(-0.00145209104366136,-0.038820139114881,
-0.00955066180060661));
#33426=CARTESIAN_POINT('Ctrl Pts',(-0.00146441088651729,-0.038820901321531,
-0.00955751421822301));
#33427=CARTESIAN_POINT('Ctrl Pts',(-0.00150216668415699,-0.0388232617255935,
-0.00957886418071039));
#33428=CARTESIAN_POINT('Ctrl Pts',(-0.00152743840433289,-0.0388248761584615,
-0.00959364706722501));
#33429=CARTESIAN_POINT('Ctrl Pts',(-0.00165807674838472,-0.0388333870204492,
-0.00967265373142536));
#33430=CARTESIAN_POINT('Ctrl Pts',(-0.00175961675864719,-0.0388405657251032,
-0.00974295978235645));
#33431=CARTESIAN_POINT('Ctrl Pts',(-0.00203544054951817,-0.0388611635934932,
-0.0099602593015319));
#33432=CARTESIAN_POINT('Ctrl Pts',(-0.00219774383051521,-0.0388745971795189,
-0.0101211456020383));
#33433=CARTESIAN_POINT('Ctrl Pts',(-0.00237422535755924,-0.0388902799717701,
-0.0103411878523124));
#33434=CARTESIAN_POINT('Ctrl Pts',(-0.00240701601816053,-0.0388932544580106,
-0.0103844243298767));
#33435=CARTESIAN_POINT('Ctrl Pts',(-0.00245354594362036,-0.0388975687565241,
-0.0104493628472223));
#33436=CARTESIAN_POINT('Ctrl Pts',(-0.00246820703516177,-0.0388989429010993,
-0.0104703882411029));
#33437=CARTESIAN_POINT('Ctrl Pts',(-0.00249384189615975,-0.0389013729704397,
-0.0105081741320989));
#33438=CARTESIAN_POINT('Ctrl Pts',(-0.00250492050365629,-0.0389024327386065,
-0.0105248613236326));
#33439=CARTESIAN_POINT('Ctrl Pts',(-0.00252785961587549,-0.0389046479843788,
-0.0105601759248636));
#33440=CARTESIAN_POINT('Ctrl Pts',(-0.0025396832775329,-0.0389058020775142,
-0.0105788259046472));
#33441=CARTESIAN_POINT('Ctrl Pts',(-0.00257062713357922,-0.0389088568147299,
-0.0106288478617212));
#33442=CARTESIAN_POINT('Ctrl Pts',(-0.00258937907631898,-0.0389107442689742,
-0.0106604438395106));
#33443=CARTESIAN_POINT('Ctrl Pts',(-0.00271078419993422,-0.0389232303810811,
-0.0108738409426379));
#33444=CARTESIAN_POINT('Ctrl Pts',(-0.00279479958166486,-0.0389331454946652,
-0.011065586539442));
#33445=CARTESIAN_POINT('Ctrl Pts',(-0.00291087670828539,-0.0389512600979821,
-0.0114296402026054));
#33446=CARTESIAN_POINT('Ctrl Pts',(-0.00294911221939567,-0.0389594500161003,
-0.0115989978677757));
#33447=CARTESIAN_POINT('Ctrl Pts',(-0.00297640784128063,-0.0389697537799309,
-0.0117992533425694));
#33448=CARTESIAN_POINT('Ctrl Pts',(-0.00297988934446562,-0.0389712412015348,
-0.011827872633229));
#33449=CARTESIAN_POINT('Ctrl Pts',(-0.00298444918056285,-0.0389734828493506,
-0.0118704692173335));
#33450=CARTESIAN_POINT('Ctrl Pts',(-0.00298584296106661,-0.0389742209904355,
-0.0118844118039434));
#33451=CARTESIAN_POINT('Ctrl Pts',(-0.00298817358054488,-0.0389755579552331,
-0.0119095005871635));
#33452=CARTESIAN_POINT('Ctrl Pts',(-0.00298914582883364,-0.0389761548658353,
-0.0119206429542594));
#33453=CARTESIAN_POINT('Ctrl Pts',(-0.00299119399647987,-0.0389775062239053,
-0.0119457354316928));
#33454=CARTESIAN_POINT('Ctrl Pts',(-0.00299223464617144,-0.0389782624945639,
-0.0119596877050776));
#33455=CARTESIAN_POINT('Ctrl Pts',(-0.00299511325906131,-0.0389805859756623,
-0.0120022985324384));
#33456=CARTESIAN_POINT('Ctrl Pts',(-0.00299663730093455,-0.038982168723352,
-0.0120309759044117));
#33457=CARTESIAN_POINT('Ctrl Pts',(-0.00300232497431783,-0.038990350493258,
-0.0121777282662941));
#33458=CARTESIAN_POINT('Ctrl Pts',(-0.00299992206141389,-0.0389972098103454,
-0.0122959456158238));
#33459=CARTESIAN_POINT('Ctrl Pts',(-0.00297374028262983,-0.0390165642481569,
-0.0126251368941267));
#33460=CARTESIAN_POINT('Ctrl Pts',(-0.00293454618453088,-0.0390291041056367,
-0.0128342183540017));
#33461=CARTESIAN_POINT('Ctrl Pts',(-0.00285381195661623,-0.039044899389337,
-0.0131034923703898));
#33462=CARTESIAN_POINT('Ctrl Pts',(-0.00283173084692017,-0.0390487104256614,
-0.0131688580216957));
#33463=CARTESIAN_POINT('Ctrl Pts',(-0.00279732358097167,-0.0390540021401096,
-0.0132601965120349));
#33464=CARTESIAN_POINT('Ctrl Pts',(-0.0027868492676536,-0.0390555416770672,
-0.0132868396426793));
#33465=CARTESIAN_POINT('Ctrl Pts',(-0.00276832514389438,-0.0390581477582604,
-0.0133320475137219));
#33466=CARTESIAN_POINT('Ctrl Pts',(-0.00276046607754844,-0.0390592204936834,
-0.0133506878514358));
#33467=CARTESIAN_POINT('Ctrl Pts',(-0.00274403413157239,-0.0390613982542113,
-0.0133885861381884));
#33468=CARTESIAN_POINT('Ctrl Pts',(-0.0027354456072213,-0.0390625026825667,
-0.0134078360966683));
#33469=CARTESIAN_POINT('Ctrl Pts',(-0.00271332968509638,-0.0390652644042006,
-0.0134560340897733));
#33470=CARTESIAN_POINT('Ctrl Pts',(-0.00269954122029,-0.0390669128358835,
-0.0134848598443316));
#33471=CARTESIAN_POINT('Ctrl Pts',(-0.0026396470821944,-0.0390737813662494,
-0.0136050994738884));
#33472=CARTESIAN_POINT('Ctrl Pts',(-0.00258933654992385,-0.039078857944528,
-0.0136943460116615));
#33473=CARTESIAN_POINT('Ctrl Pts',(-0.00241999263689838,-0.0390942384668816,
-0.0139617680625989));
#33474=CARTESIAN_POINT('Ctrl Pts',(-0.00228639399007479,-0.0391041170316073,
-0.0141298882182757));
#33475=CARTESIAN_POINT('Ctrl Pts',(-0.00207441824598657,-0.0391187646997157,
-0.014344837198527));
#33476=CARTESIAN_POINT('Ctrl Pts',(-0.00201008653344285,-0.0391231087231494,
-0.0144045865696192));
#33477=CARTESIAN_POINT('Ctrl Pts',(-0.0019270058287337,-0.0391287296770877,
-0.0144752232587987));
#33478=CARTESIAN_POINT('Ctrl Pts',(-0.00191063143912187,-0.0391298380409864,
-0.0144888472744108));
#33479=CARTESIAN_POINT('Ctrl Pts',(-0.00188444792794975,-0.0391316136790795,
-0.0145101650411146));
#33480=CARTESIAN_POINT('Ctrl Pts',(-0.00187473326568934,-0.0391322731882558,
-0.0145179742339421));
#33481=CARTESIAN_POINT('Ctrl Pts',(-0.00185600428031605,-0.0391335466151013,
-0.0145328384666745));
#33482=CARTESIAN_POINT('Ctrl Pts',(-0.0018469978403904,-0.039134159890283,
-0.0145399027762784));
#33483=CARTESIAN_POINT('Ctrl Pts',(-0.00182495514277333,-0.0391356626648682,
-0.0145569893848625));
#33484=CARTESIAN_POINT('Ctrl Pts',(-0.00181187656359613,-0.0391365558177641,
-0.0145669563135732));
#33485=CARTESIAN_POINT('Ctrl Pts',(-0.00176388642718363,-0.0391398365684443,
-0.0146029088547011));
#33486=CARTESIAN_POINT('Ctrl Pts',(-0.00172849383643636,-0.0391422626399744,
-0.0146282404378204));
#33487=CARTESIAN_POINT('Ctrl Pts',(-0.00163519224018046,-0.0391486490110194,
-0.0146919961484998));
#33488=CARTESIAN_POINT('Ctrl Pts',(-0.00157647771028428,-0.0391526586969372,
-0.0147291933836279));
#33489=CARTESIAN_POINT('Ctrl Pts',(-0.00140528564537905,-0.0391642196998403,
-0.0148294913241597));
#33490=CARTESIAN_POINT('Ctrl Pts',(-0.0012899578316361,-0.0391718488368925,
-0.0148874269556516));
#33491=CARTESIAN_POINT('Ctrl Pts',(-0.00102070520665153,-0.0391889279319041,
-0.0150016105366168));
#33492=CARTESIAN_POINT('Ctrl Pts',(-0.000865166701356852,-0.0391982789183774,
-0.0150530467161435));
#33493=CARTESIAN_POINT('Ctrl Pts',(-0.00067097495634809,-0.0392092081008345,
-0.0151000806411456));
#33494=CARTESIAN_POINT('Ctrl Pts',(-0.000635605052469569,-0.0392111705041494,
-0.0151079718697894));
#33495=CARTESIAN_POINT('Ctrl Pts',(-0.000578570366755936,-0.0392142907984768,
-0.0151196160429682));
#33496=CARTESIAN_POINT('Ctrl Pts',(-0.000556992945057825,-0.0392154612242389,
-0.0151237748813571));
#33497=CARTESIAN_POINT('Ctrl Pts',(-0.000515638383835819,-0.0392176857541131,
-0.0151312752965544));
#33498=CARTESIAN_POINT('Ctrl Pts',(-0.000495869688292898,-0.0392187410324173,
-0.0151346563347835));
#33499=CARTESIAN_POINT('Ctrl Pts',(-0.000450122735577565,-0.039221164972726,
-0.0151420090617193));
#33500=CARTESIAN_POINT('Ctrl Pts',(-0.000424123045263789,-0.0392225291600631,
-0.0151458381785259));
#33501=CARTESIAN_POINT('Ctrl Pts',(-0.000340076528525251,-0.0392268982572724,
-0.0151570899707118));
#33502=CARTESIAN_POINT('Ctrl Pts',(-0.00028186034272584,-0.0392298617549315,
-0.0151631563377064));
#33503=CARTESIAN_POINT('Ctrl Pts',(-0.000141124136975081,-0.0392369031773296,
-0.0151736704707532));
#33504=CARTESIAN_POINT('Ctrl Pts',(-5.85247863529789E-5,-0.0392409340142681,
-0.0151764198772384));
#33505=CARTESIAN_POINT('Ctrl Pts',(0.000145908966180293,-0.0392507765552011,
-0.015174778479957));
#33506=CARTESIAN_POINT('Ctrl Pts',(0.000267560614603388,-0.0392565132968298,
-0.0151663805902251));
#33507=CARTESIAN_POINT('Ctrl Pts',(0.000527771718355039,-0.0392689839189267,
-0.0151324091744021));
#33508=CARTESIAN_POINT('Ctrl Pts',(0.000665715536189162,-0.0392757203222382,
-0.0151044333918121));
#33509=CARTESIAN_POINT('Ctrl Pts',(0.000829825185483897,-0.0392843921204166,
-0.0150589547412073));
#33510=CARTESIAN_POINT('Ctrl Pts',(0.000858354197409255,-0.0392859245929285,
-0.0150505901062668));
#33511=CARTESIAN_POINT('Ctrl Pts',(0.000900301656824832,-0.0392882211165156,
-0.0150376111487432));
#33512=CARTESIAN_POINT('Ctrl Pts',(0.000913819996949949,-0.039288967910889,
-0.0150333231696109));
#33513=CARTESIAN_POINT('Ctrl Pts',(0.0009379450740193,-0.0392903134851821,
-0.0150254820619961));
#33514=CARTESIAN_POINT('Ctrl Pts',(0.000948563046926292,-0.0392909102220226,
-0.0150219652412202));
#33515=CARTESIAN_POINT('Ctrl Pts',(0.000972259805630739,-0.039292252215025,
-0.0150139692066333));
#33516=CARTESIAN_POINT('Ctrl Pts',(0.000985327335711489,-0.0392929991675005,
-0.0150094589634474));
#33517=CARTESIAN_POINT('Ctrl Pts',(0.00102463790398862,-0.0392952660846629,
-0.014995586166974));
#33518=CARTESIAN_POINT('Ctrl Pts',(0.00105078148140545,-0.0392968005553837,
-0.0149859483954579));
#33519=CARTESIAN_POINT('Ctrl Pts',(0.0011799303674384,-0.0393045015598309,
-0.0149362837497199));
#33520=CARTESIAN_POINT('Ctrl Pts',(0.00128079683873615,-0.0393108978285933,
-0.0148909532409753));
#33521=CARTESIAN_POINT('Ctrl Pts',(0.001611300749046,-0.0393326757371569,
-0.0147198998180659));
#33522=CARTESIAN_POINT('Ctrl Pts',(0.00182699172161334,-0.0393481677114533,
-0.0145697220746977));
#33523=CARTESIAN_POINT('Ctrl Pts',(0.00204924915412847,-0.0393647249737159,
-0.0143672213436977));
#33524=CARTESIAN_POINT('Ctrl Pts',(0.00207751856400366,-0.0393668468467883,
-0.0143404393591483));
#33525=CARTESIAN_POINT('Ctrl Pts',(0.00212289938237204,-0.0393702804875151,
-0.0142957380223536));
#33526=CARTESIAN_POINT('Ctrl Pts',(0.00214032378805177,-0.0393716057876214,
-0.0142781442304326));
#33527=CARTESIAN_POINT('Ctrl Pts',(0.00217135386096708,-0.0393739791661016,
-0.0142460267837763));
#33528=CARTESIAN_POINT('Ctrl Pts',(0.00218503649062956,-0.0393750305014769,
-0.0142315797903034));
#33529=CARTESIAN_POINT('Ctrl Pts',(0.00221413398877599,-0.0393772772141166,
-0.0142002380458476));
#33530=CARTESIAN_POINT('Ctrl Pts',(0.00222950150161526,-0.0393784705838083,
-0.014183300936165));
#33531=CARTESIAN_POINT('Ctrl Pts',(0.00227153637598166,-0.0393817551613423,
-0.0141358945749736));
#33532=CARTESIAN_POINT('Ctrl Pts',(0.00229778330847261,-0.0393838293344136,
-0.0141050581548049));
#33533=CARTESIAN_POINT('Ctrl Pts',(0.00245209062998006,-0.0393961873073987,
-0.0139161505622354));
#33534=CARTESIAN_POINT('Ctrl Pts',(0.00256442601590134,-0.0394058396432739,
-0.01374592050761));
#33535=CARTESIAN_POINT('Ctrl Pts',(0.00273815972245396,-0.0394236191171213,
-0.0134135610356391));
#33536=CARTESIAN_POINT('Ctrl Pts',(0.00280444514595227,-0.0394317328632308,
-0.0132549801383261));
#33537=CARTESIAN_POINT('Ctrl Pts',(0.00286564618576958,-0.0394419526798934,
-0.0130640592459295));
#33538=CARTESIAN_POINT('Ctrl Pts',(0.00287408252761063,-0.0394434459431049,
-0.0130363690600189));
#33539=CARTESIAN_POINT('Ctrl Pts',(0.00288601241832093,-0.0394456947683726,
-0.0129950781136299));
#33540=CARTESIAN_POINT('Ctrl Pts',(0.00288981350310425,-0.0394464340991057,
-0.0129815671923847));
#33541=CARTESIAN_POINT('Ctrl Pts',(0.00289647407954364,-0.0394477724375182,
-0.0129572386566017));
#33542=CARTESIAN_POINT('Ctrl Pts',(0.00289936805307299,-0.0394483695172106,
-0.0129464310403337));
#33543=CARTESIAN_POINT('Ctrl Pts',(0.00290574146158099,-0.0394497203007062,
-0.01292208511333));
#33544=CARTESIAN_POINT('Ctrl Pts',(0.00290918675807305,-0.039450475814798,
-0.012908538602502));
#33545=CARTESIAN_POINT('Ctrl Pts',(0.00291939934681311,-0.0394527935443473,
-0.0128671759216941));
#33546=CARTESIAN_POINT('Ctrl Pts',(0.00292586308743801,-0.0394543711750504,
-0.0128392872385315));
#33547=CARTESIAN_POINT('Ctrl Pts',(0.00295676936123018,-0.0394624987347242,
-0.0126966894374659));
#33548=CARTESIAN_POINT('Ctrl Pts',(0.00297486741668729,-0.0394693052259971,
-0.0125807175142311));
#33549=CARTESIAN_POINT('Ctrl Pts',(0.00300626841307121,-0.0394884620701573,
-0.0122552952313297));
#33550=CARTESIAN_POINT('Ctrl Pts',(0.00300447414339993,-0.0395008608299876,
-0.0120450340041819));
#33551=CARTESIAN_POINT('Ctrl Pts',(0.00297270405076887,-0.0395166729678301,
-0.0117658380842074));
#33552=CARTESIAN_POINT('Ctrl Pts',(0.00296212176763812,-0.0395206163921595,
-0.0116953144040078));
#33553=CARTESIAN_POINT('Ctrl Pts',(0.00294370913985941,-0.0395260580939518,
-0.0115966996928226));
#33554=CARTESIAN_POINT('Ctrl Pts',(0.00293796819512319,-0.0395276196805869,
-0.0115682470409497));
#33555=CARTESIAN_POINT('Ctrl Pts',(0.00292751073052948,-0.0395302518617929,
-0.0115200383741477));
#33556=CARTESIAN_POINT('Ctrl Pts',(0.00292300493616394,-0.0395313289461742,
-0.0115002391607041));
#33557=CARTESIAN_POINT('Ctrl Pts',(0.00291343451724971,-0.0395335063590285,
-0.0114600742373949));
#33558=CARTESIAN_POINT('Ctrl Pts',(0.00290835651715466,-0.0395346061986208,
-0.0114397128569683));
#33559=CARTESIAN_POINT('Ctrl Pts',(0.0028951308664012,-0.0395373387166609,
-0.0113889559416659));
#33560=CARTESIAN_POINT('Ctrl Pts',(0.00288671774743782,-0.0395389629419467,
-0.011358631831447));
#33561=CARTESIAN_POINT('Ctrl Pts',(0.00285030885504014,-0.0395455574706666,
-0.0112349859373537));
#33562=CARTESIAN_POINT('Ctrl Pts',(0.00281825126161172,-0.0395503989741523,
-0.011142918631392));
#33563=CARTESIAN_POINT('Ctrl Pts',(0.00271851747211837,-0.0395633735513514,
-0.0108959320556279));
#33564=CARTESIAN_POINT('Ctrl Pts',(0.00264215149722873,-0.0395712782327611,
-0.0107449193280151));
#33565=CARTESIAN_POINT('Ctrl Pts',(0.00248193095408904,-0.0395858265197355,
-0.0104851141351942));
#33566=CARTESIAN_POINT('Ctrl Pts',(0.00240256396271854,-0.0395924094033827,
-0.010374115438874));
#33567=CARTESIAN_POINT('Ctrl Pts',(0.00230163406931255,-0.0396005745914476,
-0.0102515386359574));
#33568=CARTESIAN_POINT('Ctrl Pts',(0.00228713723402088,-0.039601743072216,
-0.010234330822341));
#33569=CARTESIAN_POINT('Ctrl Pts',(0.00226405701431732,-0.039603599607838,
-0.0102075517207339));
#33570=CARTESIAN_POINT('Ctrl Pts',(0.00225560306191441,-0.0396042788539704,
-0.0101978694561736));
#33571=CARTESIAN_POINT('Ctrl Pts',(0.00223959729801393,-0.0396055640606734,
-0.010179774193298));
#33572=CARTESIAN_POINT('Ctrl Pts',(0.00223205981432771,-0.0396061690273814,
-0.0101713491647288));
#33573=CARTESIAN_POINT('Ctrl Pts',(0.00221402705030322,-0.0396076154805386,
-0.0101514208487962));
#33574=CARTESIAN_POINT('Ctrl Pts',(0.00220348958532341,-0.0396084599764574,
-0.0101399564077591));
#33575=CARTESIAN_POINT('Ctrl Pts',(0.00216708456251237,-0.0396113734112116,
-0.0101009625689168));
#33576=CARTESIAN_POINT('Ctrl Pts',(0.0021407874339902,-0.0396134708419514,
-0.0100738409414576));
#33577=CARTESIAN_POINT('Ctrl Pts',(0.00207371457127198,-0.0396187866753922,
-0.010007229462345));
#33578=CARTESIAN_POINT('Ctrl Pts',(0.00203231757378688,-0.0396220375036569,
-0.00996838729685674));
#33579=CARTESIAN_POINT('Ctrl Pts',(0.00181272409183881,-0.0396390244275337,
-0.00977376100081102));
#33580=CARTESIAN_POINT('Ctrl Pts',(0.00161762034693136,-0.0396531882096877,
-0.009638267884226));
#33581=CARTESIAN_POINT('Ctrl Pts',(0.00133189107574234,-0.0396715664798037,
-0.00948631457592746));
#33582=CARTESIAN_POINT('Ctrl Pts',(0.00125342120706623,-0.0396764068472325,
-0.00944886050546996));
#33583=CARTESIAN_POINT('Ctrl Pts',(0.00114474767397187,-0.0396828294802495,
-0.00940267387661836));
#33584=CARTESIAN_POINT('Ctrl Pts',(0.00111587640407197,-0.0396845099174429,
-0.00939093116434264));
#33585=CARTESIAN_POINT('Ctrl Pts',(0.00106928810481684,-0.0396871811612268,
-0.0093728233155729));
#33586=CARTESIAN_POINT('Ctrl Pts',(0.00105168556853572,-0.039688181322305,
-0.0093661715330512));
#33587=CARTESIAN_POINT('Ctrl Pts',(0.0010150080638223,-0.0396902468043696,
-0.00935270453531472));
#33588=CARTESIAN_POINT('Ctrl Pts',(0.000995924280322381,-0.0396913112129239,
-0.00934591599117993));
#33589=CARTESIAN_POINT('Ctrl Pts',(0.000950597863230456,-0.0396938157262249,
-0.00933030763103566));
#33590=CARTESIAN_POINT('Ctrl Pts',(0.000924298793233889,-0.0396952503187625,
-0.00932165669526648));
#33591=CARTESIAN_POINT('Ctrl Pts',(0.000833605375945967,-0.0397001372874357,
-0.00929320862828096));
#33592=CARTESIAN_POINT('Ctrl Pts',(0.000768664168127061,-0.0397035325723301,
-0.00927521639528295));
#33593=CARTESIAN_POINT('Ctrl Pts',(0.000604795754938369,-0.0397118893254924,
-0.00923570669867853));
#33594=CARTESIAN_POINT('Ctrl Pts',(0.000505281739059318,-0.0397167742408331,
-0.00921697986296786));
#33595=CARTESIAN_POINT('Ctrl Pts',(0.000211278876579293,-0.0397309347067533,
-0.00917692201730842));
#33596=CARTESIAN_POINT('Ctrl Pts',(1.54489283979635E-5,-0.0397400035473488,
-0.00916953023161437));
#33597=CARTESIAN_POINT('Ctrl Pts',(-0.000234939306648998,-0.0397524382447527,
-0.00918455477104413));
#33598=CARTESIAN_POINT('Ctrl Pts',(-0.000290081535653657,-0.0397552314741943,
-0.00918939797984695));
#33599=CARTESIAN_POINT('Ctrl Pts',(-0.000363445185181044,-0.0397590569618281,
-0.00919789251939113));
#33600=CARTESIAN_POINT('Ctrl Pts',(-0.000381814833243012,-0.0397600240287658,
-0.00920019199310643));
#33601=CARTESIAN_POINT('Ctrl Pts',(-0.00041074397304167,-0.039761563132472,
-0.00920408556273013));
#33602=CARTESIAN_POINT('Ctrl Pts',(-0.000421318531893806,-0.0397621291344292,
-0.0092055663133028));
#33603=CARTESIAN_POINT('Ctrl Pts',(-0.000443353371492702,-0.0397633160708654,
-0.0092087718755136));
#33604=CARTESIAN_POINT('Ctrl Pts',(-0.000454811848787681,-0.0397639375868941,
-0.00921050668293932));
#33605=CARTESIAN_POINT('Ctrl Pts',(-0.00048327371581384,-0.0397654915894961,
-0.00921498463737923));
#33606=CARTESIAN_POINT('Ctrl Pts',(-0.000500263966787123,-0.0397664283187391,
-0.00921780788834041));
#33607=CARTESIAN_POINT('Ctrl Pts',(-0.000565834052410495,-0.039770076043224,
-0.00922928465586122));
#33608=CARTESIAN_POINT('Ctrl Pts',(-0.000614219683179988,-0.0397728370995543,
-0.00923898956491019));
#33609=CARTESIAN_POINT('Ctrl Pts',(-0.000744113699894974,-0.0397803982986722,
-0.00926839319478653));
#33610=CARTESIAN_POINT('Ctrl Pts',(-0.000825070500280015,-0.0397852702984067,
-0.00929032271465621));
#33611=CARTESIAN_POINT('Ctrl Pts',(-0.00109410228534698,-0.0398017949266034,
-0.00937544606675465));
#33612=CARTESIAN_POINT('Ctrl Pts',(-0.00127682639303939,-0.0398135420009456,
-0.00945389296504211));
#33613=CARTESIAN_POINT('Ctrl Pts',(-0.00152376337572712,-0.0398295349814844,
-0.00959028664832621));
#33614=CARTESIAN_POINT('Ctrl Pts',(-0.00159532836875495,-0.0398341922533159,
-0.00963381888695232));
#33615=CARTESIAN_POINT('Ctrl Pts',(-0.00169062013624761,-0.0398404204088989,
-0.00969739542851158));
#33616=CARTESIAN_POINT('Ctrl Pts',(-0.00171599241279145,-0.0398420816261606,
-0.00971489413730863));
#33617=CARTESIAN_POINT('Ctrl Pts',(-0.00175637707271845,-0.0398447312993771,
-0.00974367485790911));
#33618=CARTESIAN_POINT('Ctrl Pts',(-0.00177156058830689,-0.0398457288010343,
-0.00975471193714494));
#33619=CARTESIAN_POINT('Ctrl Pts',(-0.00180297103271198,-0.0398477954422173,
-0.00977799825500174));
#33620=CARTESIAN_POINT('Ctrl Pts',(-0.00181917907705367,-0.0398488635967568,
-0.00979027142678888));
#33621=CARTESIAN_POINT('Ctrl Pts',(-0.00185742377422857,-0.0398513889086865,
-0.00981984780132442));
#33622=CARTESIAN_POINT('Ctrl Pts',(-0.00187934544332701,-0.0398528403243052,
-0.00983729695923238));
#33623=CARTESIAN_POINT('Ctrl Pts',(-0.00195475984832837,-0.0398578505814981,
-0.00989907054993767));
#33624=CARTESIAN_POINT('Ctrl Pts',(-0.00200695674159328,-0.0398613483559867,
-0.00994494512315154));
#33625=CARTESIAN_POINT('Ctrl Pts',(-0.00213461105148626,-0.0398700332804864,
-0.0100652472391694));
#33626=CARTESIAN_POINT('Ctrl Pts',(-0.00220780609729937,-0.0398751353458972,
-0.0101419367900389));
#33627=CARTESIAN_POINT('Ctrl Pts',(-0.00242320606735126,-0.039890899785197,
-0.010392982674363));
#33628=CARTESIAN_POINT('Ctrl Pts',(-0.00254995311452363,-0.0399012893600811,
-0.0105795227271284));
#33629=CARTESIAN_POINT('Ctrl Pts',(-0.00266813542260465,-0.0399142231334858,
-0.0108040333618264));
#33630=CARTESIAN_POINT('Ctrl Pts',(-0.00268123659104808,-0.0399157152516365,
-0.0108298195700061));
#33631=CARTESIAN_POINT('Ctrl Pts',(-0.00270014029017881,-0.0399179631098428,
-0.0108683979211079));
#33632=CARTESIAN_POINT('Ctrl Pts',(-0.00270622944840316,-0.0399187026749469,
-0.0108810485612566));
#33633=CARTESIAN_POINT('Ctrl Pts',(-0.00271702252410573,-0.0399200426439551,
-0.0109038806513336));
#33634=CARTESIAN_POINT('Ctrl Pts',(-0.00272175845410706,-0.0399206411373407,
-0.0109140463719535));
#33635=CARTESIAN_POINT('Ctrl Pts',(-0.00273229686775892,-0.0399219969193233,
-0.0109370025767652));
#33636=CARTESIAN_POINT('Ctrl Pts',(-0.00273806658244795,-0.0399227560490853,
-0.0109498073537495));
#33637=CARTESIAN_POINT('Ctrl Pts',(-0.00275540544741321,-0.0399250885108314,
-0.0109890204997561));
#33638=CARTESIAN_POINT('Ctrl Pts',(-0.00276668370052161,-0.0399266774278223,
-0.0110155548654924));
#33639=CARTESIAN_POINT('Ctrl Pts',(-0.00282250314421805,-0.0399349062873632,
-0.0111523243778234));
#33640=CARTESIAN_POINT('Ctrl Pts',(-0.0028608422701259,-0.0399418080382577,
-0.0112649676206232));
#33641=CARTESIAN_POINT('Ctrl Pts',(-0.00294966047371335,-0.0399614114238219,
-0.0115875915182237));
#33642=CARTESIAN_POINT('Ctrl Pts',(-0.00298432685081978,-0.0399741518488867,
-0.0118012033774357));
#33643=CARTESIAN_POINT('Ctrl Pts',(-0.00299857292497328,-0.0399891941625337,
-0.0120693580166509));
#33644=CARTESIAN_POINT('Ctrl Pts',(-0.00299998151196683,-0.0399921098222384,
-0.0121220739398953));
#33645=CARTESIAN_POINT('Ctrl Pts',(-0.0029999998192441,-0.0399949849792216,
-0.0121748118762894));
#33646=CARTESIAN_POINT('Ctrl Pts',(0.00256965295416722,-0.0405776976452009,
-0.0106276660578484));
#33647=CARTESIAN_POINT('Ctrl Pts',(0.00261879861117561,-0.0405720710453063,
-0.0107092371239148));
#33648=CARTESIAN_POINT('Ctrl Pts',(0.00266403531987886,-0.0405664894762788,
-0.0107931070827784));
#33649=CARTESIAN_POINT('Ctrl Pts',(0.00272274854087895,-0.0405587562280604,
-0.0109155807532141));
#33650=CARTESIAN_POINT('Ctrl Pts',(0.00273954608364068,-0.0405564757033417,
-0.0109525242035279));
#33651=CARTESIAN_POINT('Ctrl Pts',(0.00276145282245608,-0.0405534158610409,
-0.0110034206692555));
#33652=CARTESIAN_POINT('Ctrl Pts',(0.00276721497095573,-0.0405526022603544,
-0.011017086159205));
#33653=CARTESIAN_POINT('Ctrl Pts',(0.00277696563795014,-0.0405512108519496,
-0.0110406983771469));
#33654=CARTESIAN_POINT('Ctrl Pts',(0.00278100258354374,-0.0405506302687271,
-0.011050624660749));
#33655=CARTESIAN_POINT('Ctrl Pts',(0.00278905317772386,-0.0405494635330612,
-0.0110707279345512));
#33656=CARTESIAN_POINT('Ctrl Pts',(0.00279306442155231,-0.040548877595032,
-0.0110809054290569));
#33657=CARTESIAN_POINT('Ctrl Pts',(0.00280147737259189,-0.0405476384279538,
-0.0111025981923252));
#33658=CARTESIAN_POINT('Ctrl Pts',(0.00280586396624662,-0.0405469860823097,
-0.0111141191484769));
#33659=CARTESIAN_POINT('Ctrl Pts',(0.00281753865299263,-0.0405452319461826,
-0.0111453592877216));
#33660=CARTESIAN_POINT('Ctrl Pts',(0.00282469081541642,-0.0405441377088638,
-0.0111651288990728));
#33661=CARTESIAN_POINT('Ctrl Pts',(0.00285966167485715,-0.0405386781683054,
-0.0112650649466885));
#33662=CARTESIAN_POINT('Ctrl Pts',(0.00288428004607311,-0.0405344704922299,
-0.0113463166276499));
#33663=CARTESIAN_POINT('Ctrl Pts',(0.0029409825100946,-0.0405234096535795,
-0.0115667564360639));
#33664=CARTESIAN_POINT('Ctrl Pts',(0.00296663176830873,-0.0405167172989409,
-0.011707370721134));
#33665=CARTESIAN_POINT('Ctrl Pts',(0.00299405510528987,-0.0405047420096543,
-0.0119577932318347));
#33666=CARTESIAN_POINT('Ctrl Pts',(0.0030000061268486,-0.0404995086955379,
-0.0120668689222672));
#33667=CARTESIAN_POINT('Ctrl Pts',(0.00299999565021975,-0.040490317626161,
-0.0122533712474678));
#33668=CARTESIAN_POINT('Ctrl Pts',(0.0029969998723812,-0.0404864369948116,
-0.0123306870493325));
#33669=CARTESIAN_POINT('Ctrl Pts',(0.00298876169002086,-0.040480967829138,
-0.0124369220926438));
#33670=CARTESIAN_POINT('Ctrl Pts',(0.00298607791883728,-0.0404794561517935,
-0.0124660117742412));
#33671=CARTESIAN_POINT('Ctrl Pts',(0.00298077556634881,-0.0404768553253285,
-0.0125155624431293));
#33672=CARTESIAN_POINT('Ctrl Pts',(0.00297836996422824,-0.0404757727012125,
-0.0125360443699115));
#33673=CARTESIAN_POINT('Ctrl Pts',(0.00297338539539684,-0.0404736979990825,
-0.0125750119088238));
#33674=CARTESIAN_POINT('Ctrl Pts',(0.00297084470699352,-0.0404727071347163,
-0.0125935014894876));
#33675=CARTESIAN_POINT('Ctrl Pts',(0.00296448897942972,-0.0404703735081709,
-0.0126367578327425));
#33676=CARTESIAN_POINT('Ctrl Pts',(0.00296053585755001,-0.0404690266053592,
-0.0126615026409925));
#33677=CARTESIAN_POINT('Ctrl Pts',(0.00294559992202271,-0.0404642743089021,
-0.0127480226059367));
#33678=CARTESIAN_POINT('Ctrl Pts',(0.00293299013605131,-0.040460820385791,
-0.0128094972915569));
#33679=CARTESIAN_POINT('Ctrl Pts',(0.00286956058495486,-0.0404455098138617,
-0.0130759768735808));
#33680=CARTESIAN_POINT('Ctrl Pts',(0.00279910450280392,-0.040433095513478,
-0.0132756695412901));
#33681=CARTESIAN_POINT('Ctrl Pts',(0.00265818961569454,-0.0404139799100914,
-0.013571414100777));
#33682=CARTESIAN_POINT('Ctrl Pts',(0.00260201391340249,-0.0404072425115315,
-0.0136735480038217));
#33683=CARTESIAN_POINT('Ctrl Pts',(0.00252480006973463,-0.0403991722025544,
-0.0137964102106676));
#33684=CARTESIAN_POINT('Ctrl Pts',(0.00250921473316229,-0.040397595812251,
-0.0138204388490633));
#33685=CARTESIAN_POINT('Ctrl Pts',(0.00248543905272108,-0.0403952720352007,
-0.0138559699092001));
#33686=CARTESIAN_POINT('Ctrl Pts',(0.0024775081064065,-0.0403945097821374,
-0.0138676430927767));
#33687=CARTESIAN_POINT('Ctrl Pts',(0.00246308087557972,-0.040393146780609,
-0.0138885588089788));
#33688=CARTESIAN_POINT('Ctrl Pts',(0.00245661433980383,-0.0403925442145641,
-0.0138978212316271));
#33689=CARTESIAN_POINT('Ctrl Pts',(0.00244191226338605,-0.0403911930484467,
-0.0139186285402674));
#33690=CARTESIAN_POINT('Ctrl Pts',(0.00243364702012821,-0.0403904463853412,
-0.0139301518027545));
#33691=CARTESIAN_POINT('Ctrl Pts',(0.00240780591699792,-0.0403881502051173,
-0.0139656449207905));
#33692=CARTESIAN_POINT('Ctrl Pts',(0.00238995486302466,-0.0403866177372581,
-0.0139894131296663));
#33693=CARTESIAN_POINT('Ctrl Pts',(0.00228766265239588,-0.0403781086559713,
-0.0141214784378251));
#33694=CARTESIAN_POINT('Ctrl Pts',(0.00219620949879302,-0.0403715113958629,
-0.0142241521112112));
#33695=CARTESIAN_POINT('Ctrl Pts',(0.00201370293991924,-0.0403593556999734,
-0.0144027167035425));
#33696=CARTESIAN_POINT('Ctrl Pts',(0.00192457595399876,-0.0403537923047462,
-0.0144801812288325));
#33697=CARTESIAN_POINT('Ctrl Pts',(0.00176300407091633,-0.0403439796037956,
-0.0146046825232077));
#33698=CARTESIAN_POINT('Ctrl Pts',(0.001692665572248,-0.0403397886847267,
-0.0146542150151867));
#33699=CARTESIAN_POINT('Ctrl Pts',(0.00156970597375033,-0.0403325030016915,
-0.014733124701304));
#33700=CARTESIAN_POINT('Ctrl Pts',(0.00151815014602399,-0.0403294598911116,
-0.0147640637623415));
#33701=CARTESIAN_POINT('Ctrl Pts',(0.00144261009357475,-0.0403249991113226,
-0.0148063620828304));
#33702=CARTESIAN_POINT('Ctrl Pts',(0.00141934887838025,-0.040323625294301,
-0.0148189857299882));
#33703=CARTESIAN_POINT('Ctrl Pts',(0.00137822418399705,-0.0403211947113337,
-0.0148406042998392));
#33704=CARTESIAN_POINT('Ctrl Pts',(0.00136043192009853,-0.0403201425808426,
-0.0148497315241323));
#33705=CARTESIAN_POINT('Ctrl Pts',(0.00132313367568664,-0.0403179352565859,
-0.0148683964485055));
#33706=CARTESIAN_POINT('Ctrl Pts',(0.00130361278204073,-0.0403167790319272,
-0.0148779015992171));
#33707=CARTESIAN_POINT('Ctrl Pts',(0.00125205471136081,-0.0403137220116079,
-0.0149023175975434));
#33708=CARTESIAN_POINT('Ctrl Pts',(0.00121985491628539,-0.0403118095254279,
-0.0149168754460356));
#33709=CARTESIAN_POINT('Ctrl Pts',(0.00106230148050335,-0.0403024328539316,
-0.0149847808724365));
#33710=CARTESIAN_POINT('Ctrl Pts',(0.000933683416954394,-0.0402947104725204,
-0.0150301109051748));
#33711=CARTESIAN_POINT('Ctrl Pts',(0.000626722277476678,-0.0402762373237819,
-0.0151153220215603));
#33712=CARTESIAN_POINT('Ctrl Pts',(0.000446927347611358,-0.0402653734004754,
-0.0151479754470612));
#33713=CARTESIAN_POINT('Ctrl Pts',(0.000183769610370934,-0.0402500847053172,
-0.0151713375144694));
#33714=CARTESIAN_POINT('Ctrl Pts',(0.000101986409596025,-0.0402454227535879,
-0.0151752361904458));
#33715=CARTESIAN_POINT('Ctrl Pts',(-7.10287049814954E-7,-0.0402397593314459,
-0.0151759256650622));
#33716=CARTESIAN_POINT('Ctrl Pts',(-2.15626867610429E-5,-0.040238619285167,
-0.0151758482663919));
#33717=CARTESIAN_POINT('Ctrl Pts',(-5.47104820396596E-5,-0.0402368245539899,
-0.0151753795854766));
#33718=CARTESIAN_POINT('Ctrl Pts',(-6.70068523135331E-5,-0.0402361626246399,
-0.0151751300905804));
#33719=CARTESIAN_POINT('Ctrl Pts',(-9.05986260739049E-5,-0.0402349004628171,
-0.0151745062511431));
#33720=CARTESIAN_POINT('Ctrl Pts',(-0.00010189384314063,-0.0402342996626474,
-0.0151741436926928));
#33721=CARTESIAN_POINT('Ctrl Pts',(-0.000129456880718558,-0.0402328416536381,
-0.0151731030268803));
#33722=CARTESIAN_POINT('Ctrl Pts',(-0.000145721954295245,-0.0402319881214045,
-0.0151723562859015));
#33723=CARTESIAN_POINT('Ctrl Pts',(-0.000205350289779144,-0.0402288815833001,
-0.0151691320402153));
#33724=CARTESIAN_POINT('Ctrl Pts',(-0.000248666154669872,-0.0402266686303352,
-0.015165845250389));
#33725=CARTESIAN_POINT('Ctrl Pts',(-0.000361145506699171,-0.0402210018226433,
-0.0151548489326624));
#33726=CARTESIAN_POINT('Ctrl Pts',(-0.0004301407063033,-0.0402176042235468,
-0.0151456716407745));
#33727=CARTESIAN_POINT('Ctrl Pts',(-0.000625350959277983,-0.0402080676315979,
-0.0151127594231186));
#33728=CARTESIAN_POINT('Ctrl Pts',(-0.000750446269556413,-0.04020204348561,
-0.0150833115107572));
#33729=CARTESIAN_POINT('Ctrl Pts',(-0.00103110949125309,-0.0401880903968969,
-0.0149979149648303));
#33730=CARTESIAN_POINT('Ctrl Pts',(-0.00118470396521038,-0.0401801212133555,
-0.0149369559532378));
#33731=CARTESIAN_POINT('Ctrl Pts',(-0.0013645136149081,-0.0401699078832326,
-0.0148478150214952));
#33732=CARTESIAN_POINT('Ctrl Pts',(-0.00139624222860681,-0.0401680712270034,
-0.0148313729003655));
#33733=CARTESIAN_POINT('Ctrl Pts',(-0.00144669697266912,-0.040165091209939,
-0.0148040724457243));
#33734=CARTESIAN_POINT('Ctrl Pts',(-0.00146561291330338,-0.0401639602988138,
-0.0147935711543631));
#33735=CARTESIAN_POINT('Ctrl Pts',(-0.00150154481459948,-0.0401617850485254,
-0.0147731118046841));
#33736=CARTESIAN_POINT('Ctrl Pts',(-0.0015185794801785,-0.0401607419912673,
-0.0147631887842549));
#33737=CARTESIAN_POINT('Ctrl Pts',(-0.00155765497805228,-0.0401583214147595,
-0.0147399077239977));
#33738=CARTESIAN_POINT('Ctrl Pts',(-0.00157962372534291,-0.040156939721628,
-0.0147264322441178));
#33739=CARTESIAN_POINT('Ctrl Pts',(-0.00164963526617186,-0.0401524679235596,
-0.0146822361743953));
#33740=CARTESIAN_POINT('Ctrl Pts',(-0.001696974727142,-0.0401493386928709,
-0.0146504295869694));
#33741=CARTESIAN_POINT('Ctrl Pts',(-0.00180844172346869,-0.0401417103717177,
-0.0145708335762152));
#33742=CARTESIAN_POINT('Ctrl Pts',(-0.00187161906712831,-0.0401371689255701,
-0.0145217929038094));
#33743=CARTESIAN_POINT('Ctrl Pts',(-0.00202926132435129,-0.0401252883990066,
-0.014389000195465));
#33744=CARTESIAN_POINT('Ctrl Pts',(-0.00212053496248324,-0.0401178575547624,
-0.0143017059476906));
#33745=CARTESIAN_POINT('Ctrl Pts',(-0.0022174373159377,-0.0401094469106787,
-0.0141965597787505));
#33746=CARTESIAN_POINT('Ctrl Pts',(-0.00222873319655102,-0.0401084578831224,
-0.0141840941384101));
#33747=CARTESIAN_POINT('Ctrl Pts',(-0.00233152887545786,-0.040099381494069,
-0.0140687177369802));
#33748=CARTESIAN_POINT('Ctrl Pts',(-0.00241595464481703,-0.0400913599467195,
-0.0139597065533433));
#33749=CARTESIAN_POINT('Ctrl Pts',(-0.00250500095086284,-0.0400825120918266,
-0.0138267521562276));
#33750=CARTESIAN_POINT('Ctrl Pts',(-0.00251719828008138,-0.040081290702434,
-0.013808093991366));
#33751=CARTESIAN_POINT('Ctrl Pts',(-0.00253600131703588,-0.0400793949696446,
-0.013778618978742));
#33752=CARTESIAN_POINT('Ctrl Pts',(-0.0025427481482677,-0.0400787120524843,
-0.0137678936158807));
#33753=CARTESIAN_POINT('Ctrl Pts',(-0.00255530963138453,-0.0400774359357042,
-0.0137476412010889));
#33754=CARTESIAN_POINT('Ctrl Pts',(-0.00256113930954321,-0.0400768418216707,
-0.0137381240695144));
#33755=CARTESIAN_POINT('Ctrl Pts',(-0.00257483634965178,-0.0400754410128577,
-0.0137154805012945));
#33756=CARTESIAN_POINT('Ctrl Pts',(-0.0025826567407554,-0.0400746372526873,
-0.013702325810599));
#33757=CARTESIAN_POINT('Ctrl Pts',(-0.00260884008133195,-0.040071930617449,
-0.0136575055015148));
#33758=CARTESIAN_POINT('Ctrl Pts',(-0.00262672465101543,-0.0400700552214901,
-0.0136255628049344));
#33759=CARTESIAN_POINT('Ctrl Pts',(-0.00273586123447575,-0.040058387866461,
-0.0134219858358367));
#33760=CARTESIAN_POINT('Ctrl Pts',(-0.00281084316255062,-0.0400493172240128,
-0.013242135644124));
#33761=CARTESIAN_POINT('Ctrl Pts',(-0.00289558616303424,-0.0400356016518335,
-0.0129660943663709));
#33762=CARTESIAN_POINT('Ctrl Pts',(-0.00291900253868639,-0.0400310943487473,
-0.0128746546558181));
#33763=CARTESIAN_POINT('Ctrl Pts',(-0.00295676732285468,-0.0400219758964842,
-0.0126916843449128));
#33764=CARTESIAN_POINT('Ctrl Pts',(-0.00297126309730216,-0.0400173734528224,
-0.0126002921505042));
#33765=CARTESIAN_POINT('Ctrl Pts',(-0.00298501596369903,-0.040011026572921,
-0.0124769810296456));
#33766=CARTESIAN_POINT('Ctrl Pts',(-0.0029880216525534,-0.0400093960774991,
-0.0124455285153653));
#33767=CARTESIAN_POINT('Ctrl Pts',(-0.00299218877698966,-0.0400066620897498,
-0.0123932075219325));
#33768=CARTESIAN_POINT('Ctrl Pts',(-0.00299362994397026,-0.0400055672142554,
-0.0123723635162052));
#33769=CARTESIAN_POINT('Ctrl Pts',(-0.00299594895766515,-0.0400034789638127,
-0.0123328247810819));
#33770=CARTESIAN_POINT('Ctrl Pts',(-0.00299686982764377,-0.0400024869604999,
-0.0123141335163856));
#33771=CARTESIAN_POINT('Ctrl Pts',(-0.00299836853126886,-0.0400004830281664,
-0.0122765647918212));
#33772=CARTESIAN_POINT('Ctrl Pts',(-0.00299894309789592,-0.03999947104557,
-0.012257688060272));
#33773=CARTESIAN_POINT('Ctrl Pts',(-0.00299978707736779,-0.0399973042605326,
-0.0122174781542378));
#33774=CARTESIAN_POINT('Ctrl Pts',(-0.00300000722478825,-0.0399961480195609,
-0.0121961450931526));
#33775=CARTESIAN_POINT('Ctrl Pts',(-0.0029999998192441,-0.0399949849792216,
-0.0121748118762893));
#33776=CARTESIAN_POINT('Origin',(1.7347234759768E-18,-0.0298787743898723,
-0.0121758532865581));
#33777=CARTESIAN_POINT('',(-0.00250000000000292,-0.0304787743898694,-0.0121758532865581));
#33778=CARTESIAN_POINT('Origin',(1.00024155624823E-14,-0.0304787743898623,
-0.0121758532865681));
#33779=CARTESIAN_POINT('',(-0.0031,-0.0298787743898723,-0.0121758532865581));
#33780=CARTESIAN_POINT('Origin',(1.00024155624823E-14,-0.0304787743898623,
-0.0121758532865681));
#33781=CARTESIAN_POINT('Origin',(0.,-0.0424924495244671,-0.0121758532865581));
#33782=CARTESIAN_POINT('Origin',(1.00024155624823E-14,-0.0304787743898623,
-0.0121758532865681));
#33783=CARTESIAN_POINT('Ctrl Pts',(0.00667266361729431,-0.0408411507555838,
-0.0135686213491869));
#33784=CARTESIAN_POINT('Ctrl Pts',(0.00621453914932291,-0.0408149751823628,
-0.0137898879259038));
#33785=CARTESIAN_POINT('Ctrl Pts',(0.00507072224427489,-0.040762628119428,
-0.0137417506490211));
#33786=CARTESIAN_POINT('Ctrl Pts',(0.00417951551514757,-0.0406841095667795,
-0.0122616719912261));
#33787=CARTESIAN_POINT('Ctrl Pts',(0.00492533652721776,-0.0406055950976381,
-0.0107057736276615));
#33788=CARTESIAN_POINT('Ctrl Pts',(0.00663317335312316,-0.0405270806284968,
-0.0104680447707994));
#33789=CARTESIAN_POINT('Ctrl Pts',(0.00777404656683587,-0.0404485661593554,
-0.011762495846534));
#33790=CARTESIAN_POINT('Ctrl Pts',(0.00732306899069569,-0.0403700516902141,
-0.0134276029751788));
#33791=CARTESIAN_POINT('Ctrl Pts',(0.0056855439467377,-0.0402915372210728,
-0.0139699426948976));
#33792=CARTESIAN_POINT('Ctrl Pts',(0.00432995641023964,-0.0402130227519315,
-0.0129029294162582));
#33793=CARTESIAN_POINT('Ctrl Pts',(0.00447248538985062,-0.0401345082827901,
-0.0111837377979531));
#33794=CARTESIAN_POINT('Ctrl Pts',(0.0059851779029977,-0.0400559938136489,
-0.0103544763934777));
#33795=CARTESIAN_POINT('Ctrl Pts',(0.00751118377554786,-0.0399774793445075,
-0.0111590157052924));
#33796=CARTESIAN_POINT('Ctrl Pts',(0.00768163121117975,-0.0398989648753662,
-0.0128756677943404));
#33797=CARTESIAN_POINT('Ctrl Pts',(0.00634364059981585,-0.0398204504062249,
-0.013964579343715));
#33798=CARTESIAN_POINT('Ctrl Pts',(0.0046973980185026,-0.0397419359370836,
-0.0134489822855388));
#33799=CARTESIAN_POINT('Ctrl Pts',(0.00421960572095684,-0.0396634214679422,
-0.0117913740701257));
#33800=CARTESIAN_POINT('Ctrl Pts',(0.0053388471060399,-0.0395849069988008,
-0.0104786480096583));
#33801=CARTESIAN_POINT('Ctrl Pts',(0.00705115061506779,-0.0395063925296596,
-0.0106883348320183));
#33802=CARTESIAN_POINT('Ctrl Pts',(0.00782055967922068,-0.0394278780605182,
-0.0122323429056206));
#33803=CARTESIAN_POINT('Ctrl Pts',(0.00695690569528211,-0.0393493635913769,
-0.0137256791573249));
#33804=CARTESIAN_POINT('Ctrl Pts',(0.00523489617102149,-0.0392708491222356,
-0.0138288036313886));
#33805=CARTESIAN_POINT('Ctrl Pts',(0.00419919366962196,-0.0391923346530943,
-0.0124492124957124));
#33806=CARTESIAN_POINT('Ctrl Pts',(0.00477883530496066,-0.0391138201839529,
-0.010824414978702));
#33807=CARTESIAN_POINT('Ctrl Pts',(0.00645387582937621,-0.0390353057148116,
-0.010411873286939));
#33808=CARTESIAN_POINT('Ctrl Pts',(0.00772178447199111,-0.0389567912456703,
-0.0115816420968184));
#33809=CARTESIAN_POINT('Ctrl Pts',(0.00744523249116456,-0.0388782767765289,
-0.0132844252303561));
#33810=CARTESIAN_POINT('Ctrl Pts',(0.00587229021614751,-0.0387997623073876,
-0.0139928064833142));
#33811=CARTESIAN_POINT('Ctrl Pts',(0.00441390509800126,-0.0387212478382463,
-0.0130713596616639));
#33812=CARTESIAN_POINT('Ctrl Pts',(0.00437826548718945,-0.038642733369105,
-0.0113466332448878));
#33813=CARTESIAN_POINT('Ctrl Pts',(0.00579734052997675,-0.0385642188999636,
-0.010365726812645));
#33814=CARTESIAN_POINT('Ctrl Pts',(0.00739820346327778,-0.0384857044308223,
-0.0110085248100627));
#33815=CARTESIAN_POINT('Ctrl Pts',(0.00774486169156298,-0.038407189961681,
-0.0126984299688818));
#33816=CARTESIAN_POINT('Ctrl Pts',(0.00652635875128295,-0.0383286754925397,
-0.0139195778073208));
#33817=CARTESIAN_POINT('Ctrl Pts',(0.00483570593105475,-0.0382501610233984,
-0.0135765845040604));
#33818=CARTESIAN_POINT('Ctrl Pts',(0.00418943834467669,-0.038171646554257,
-0.0119771191414636));
#33819=CARTESIAN_POINT('Ctrl Pts',(0.00516726562172514,-0.0380931320851157,
-0.0105559204619115));
#33820=CARTESIAN_POINT('Ctrl Pts',(0.00689206513754615,-0.0380146176159744,
-0.0105878205894473));
#33821=CARTESIAN_POINT('Ctrl Pts',(0.00781667217861196,-0.037936103146833,
-0.012044203882063));
#33822=CARTESIAN_POINT('Ctrl Pts',(0.00711170265126494,-0.0378575886776917,
-0.01361867932755));
#33823=CARTESIAN_POINT('Ctrl Pts',(0.00540952407975407,-0.0377790742085504,
-0.0138989209182331));
#33824=CARTESIAN_POINT('Ctrl Pts',(0.00423700706452516,-0.0377005597394091,
-0.0126335551323258));
#33825=CARTESIAN_POINT('Ctrl Pts',(0.00464591942445379,-0.0376220452702677,
-0.0109576171533986));
#33826=CARTESIAN_POINT('Ctrl Pts',(0.00626944937421679,-0.0375435308011264,
-0.0103744674140466));
#33827=CARTESIAN_POINT('Ctrl Pts',(0.0076512965121535,-0.0374650163319851,
-0.0114071497552607));
#33828=CARTESIAN_POINT('Ctrl Pts',(0.007551879443792,-0.0373865018628437,
-0.013129430554788));
#33829=CARTESIAN_POINT('Ctrl Pts',(0.006060471354512,-0.0373079873937024,
-0.0139962191982324));
#33830=CARTESIAN_POINT('Ctrl Pts',(0.00451469679310158,-0.0372294729245611,
-0.0132303578992094));
#33831=CARTESIAN_POINT('Ctrl Pts',(0.0043014971156851,-0.0371509584554198,
-0.0115181250952989));
#33832=CARTESIAN_POINT('Ctrl Pts',(0.00561140292832371,-0.0370724439862784,
-0.0103968007018607));
#33833=CARTESIAN_POINT('Ctrl Pts',(0.00727080916413441,-0.0369939295171371,
-0.0108694947301078));
#33834=CARTESIAN_POINT('Ctrl Pts',(0.00778849486716388,-0.0369154089680987,
-0.0125178380097699));
#33835=CARTESIAN_POINT('Ctrl Pts',(0.00706639652799099,-0.036863059908774,
-0.013406293288968));
#33836=CARTESIAN_POINT('Ctrl Pts',(0.0065970260151864,-0.0368368823391631,
-0.0136026816399946));
#33837=CARTESIAN_POINT('Ctrl Pts',(0.00663125973307481,-0.0408961160367515,
-0.0134828934963237));
#33838=CARTESIAN_POINT('Ctrl Pts',(0.00620133380586334,-0.0408699404635307,
-0.0136905406420376));
#33839=CARTESIAN_POINT('Ctrl Pts',(0.00512792127751624,-0.0408175934005959,
-0.0136453663174946));
#33840=CARTESIAN_POINT('Ctrl Pts',(0.00429157022852352,-0.0407390748479473,
-0.0122563896664198));
#33841=CARTESIAN_POINT('Ctrl Pts',(0.00499148436226952,-0.040660560378806,
-0.0107962601746154));
#33842=CARTESIAN_POINT('Ctrl Pts',(0.00659420017911819,-0.0405820459096646,
-0.010573164037306));
#33843=CARTESIAN_POINT('Ctrl Pts',(0.00766485020662715,-0.0405035314405233,
-0.011787938880984));
#33844=CARTESIAN_POINT('Ctrl Pts',(0.00724163126477025,-0.040425016971382,
-0.0133505551048212));
#33845=CARTESIAN_POINT('Ctrl Pts',(0.00570489938931959,-0.0403465025022407,
-0.0138595126549301));
#33846=CARTESIAN_POINT('Ctrl Pts',(0.00443275116478599,-0.0402679880330993,
-0.0128581763255321));
#33847=CARTESIAN_POINT('Ctrl Pts',(0.00456650718088586,-0.0401894735639581,
-0.0112448046280396));
#33848=CARTESIAN_POINT('Ctrl Pts',(0.00598609023476707,-0.0401109590948166,
-0.0104665860364886));
#33849=CARTESIAN_POINT('Ctrl Pts',(0.00741816718230774,-0.0400324446256754,
-0.0112216042330534));
#33850=CARTESIAN_POINT('Ctrl Pts',(0.00757812321375344,-0.0399539301565341,
-0.0128325927147457));
#33851=CARTESIAN_POINT('Ctrl Pts',(0.00632248878597894,-0.0398754156873926,
-0.0138544794294832));
#33852=CARTESIAN_POINT('Ctrl Pts',(0.00477757595624066,-0.0397969012182514,
-0.0133706184729063));
#33853=CARTESIAN_POINT('Ctrl Pts',(0.00432919279642726,-0.0397183867491099,
-0.011815039588154));
#33854=CARTESIAN_POINT('Ctrl Pts',(0.0053795424806211,-0.0396398722799688,
-0.0105831146241368));
#33855=CARTESIAN_POINT('Ctrl Pts',(0.00698645004669358,-0.0395613578108274,
-0.0107798947741392));
#33856=CARTESIAN_POINT('Ctrl Pts',(0.00770850033747063,-0.0394828433416861,
-0.0122288658487573));
#33857=CARTESIAN_POINT('Ctrl Pts',(0.00689800610327526,-0.0394043288725447,
-0.0136302840604831));
#33858=CARTESIAN_POINT('Ctrl Pts',(0.00528198994796513,-0.0393258144034035,
-0.0137270610026236));
#33859=CARTESIAN_POINT('Ctrl Pts',(0.00431003715050586,-0.0392472999342621,
-0.0124323866517762));
#33860=CARTESIAN_POINT('Ctrl Pts',(0.00485400060355347,-0.0391687854651208,
-0.01090759889677));
#33861=CARTESIAN_POINT('Ctrl Pts',(0.00642593880140802,-0.0390902709959795,
-0.0105204500284067));
#33862=CARTESIAN_POINT('Ctrl Pts',(0.00761580495548908,-0.0390117565268381,
-0.0116182170663417));
#33863=CARTESIAN_POINT('Ctrl Pts',(0.00735627534052331,-0.0389332420576968,
-0.0132161902563959));
#33864=CARTESIAN_POINT('Ctrl Pts',(0.00588015102646683,-0.0388547275885554,
-0.0138809691282728));
#33865=CARTESIAN_POINT('Ctrl Pts',(0.00451153263128116,-0.0387762131194141,
-0.013016239329124));
#33866=CARTESIAN_POINT('Ctrl Pts',(0.00447808671473453,-0.0386976986502728,
-0.0113976735118431));
#33867=CARTESIAN_POINT('Ctrl Pts',(0.00580981465376934,-0.0386191841811315,
-0.0104771439682956));
#33868=CARTESIAN_POINT('Ctrl Pts',(0.00731214104988036,-0.0385406697119902,
-0.0110803763742686));
#33869=CARTESIAN_POINT('Ctrl Pts',(0.00763746172284284,-0.0384621552428488,
-0.0126662642564893));
#33870=CARTESIAN_POINT('Ctrl Pts',(0.00649396024445763,-0.0383836407737075,
-0.0138122478338953));
#33871=CARTESIAN_POINT('Ctrl Pts',(0.00490737072098658,-0.0383051263045662,
-0.0134903665019845));
#33872=CARTESIAN_POINT('Ctrl Pts',(0.00430088228667392,-0.0382266118354249,
-0.0119893516531119));
#33873=CARTESIAN_POINT('Ctrl Pts',(0.0052185222036143,-0.0381480973662836,
-0.010655630791697));
#33874=CARTESIAN_POINT('Ctrl Pts',(0.00683715662053758,-0.0380695828971422,
-0.0106855673981607));
#33875=CARTESIAN_POINT('Ctrl Pts',(0.00770485212083813,-0.0379910684280009,
-0.0120523071844584));
#33876=CARTESIAN_POINT('Ctrl Pts',(0.00704327497556473,-0.0379125539588594,
-0.0135298702990634));
#33877=CARTESIAN_POINT('Ctrl Pts',(0.00544586913545169,-0.0378340394897182,
-0.0137928624205084));
#33878=CARTESIAN_POINT('Ctrl Pts',(0.00434552305008409,-0.0377555250205769,
-0.0126053826048663));
#33879=CARTESIAN_POINT('Ctrl Pts',(0.00472926597974898,-0.0376770105514356,
-0.0110326021927446));
#33880=CARTESIAN_POINT('Ctrl Pts',(0.00625286418898258,-0.0375984960822943,
-0.0104853465669882));
#33881=CARTESIAN_POINT('Ctrl Pts',(0.00754965568032684,-0.0375199816131529,
-0.0114544651015805));
#33882=CARTESIAN_POINT('Ctrl Pts',(0.00745635794513875,-0.0374414671440116,
-0.0130707358345845));
#33883=CARTESIAN_POINT('Ctrl Pts',(0.0060567492133162,-0.0373629526748703,
-0.0138841717832892));
#33884=CARTESIAN_POINT('Ctrl Pts',(0.00460612038199239,-0.037284438205729,
-0.0131654508851109));
#33885=CARTESIAN_POINT('Ctrl Pts',(0.0044060436006751,-0.0372059237365876,
-0.0115586096721047));
#33886=CARTESIAN_POINT('Ctrl Pts',(0.00563532190914864,-0.0371274092674463,
-0.0105063051931748));
#33887=CARTESIAN_POINT('Ctrl Pts',(0.00719258814229796,-0.037048894798305,
-0.010949903893068));
#33888=CARTESIAN_POINT('Ctrl Pts',(0.00767840918317049,-0.0369703742492665,
-0.0124967881186791));
#33889=CARTESIAN_POINT('Ctrl Pts',(0.007000757541071,-0.0369180251899419,
-0.0133305570753701));
#33890=CARTESIAN_POINT('Ctrl Pts',(0.006560277787137,-0.0368918476203311,
-0.01351485730339));
#33891=CARTESIAN_POINT('Ctrl Pts',(0.0065898558488552,-0.0409510813179196,
-0.0133971656434607));
#33892=CARTESIAN_POINT('Ctrl Pts',(0.00618812846240375,-0.0409249057446983,
-0.0135911933581714));
#33893=CARTESIAN_POINT('Ctrl Pts',(0.00518512031075758,-0.0408725586817636,
-0.0135489819859681));
#33894=CARTESIAN_POINT('Ctrl Pts',(0.00440362494189948,-0.0407940401291151,
-0.0122511073416135));
#33895=CARTESIAN_POINT('Ctrl Pts',(0.00505763219732118,-0.0407155256599738,
-0.0108867467215694));
#33896=CARTESIAN_POINT('Ctrl Pts',(0.00655522700511323,-0.0406370111908325,
-0.0106782833038126));
#33897=CARTESIAN_POINT('Ctrl Pts',(0.00755565384641844,-0.0405584967216911,
-0.0118133819154339));
#33898=CARTESIAN_POINT('Ctrl Pts',(0.00716019353884481,-0.0404799822525498,
-0.0132735072344637));
#33899=CARTESIAN_POINT('Ctrl Pts',(0.00572425483190137,-0.0404014677834084,
-0.0137490826149629));
#33900=CARTESIAN_POINT('Ctrl Pts',(0.00453554591933244,-0.0403229533142671,
-0.0128134232348059));
#33901=CARTESIAN_POINT('Ctrl Pts',(0.00466052897192121,-0.0402444388451258,
-0.0113058714581259));
#33902=CARTESIAN_POINT('Ctrl Pts',(0.00598700256653645,-0.0401659243759845,
-0.0105786956794995));
#33903=CARTESIAN_POINT('Ctrl Pts',(0.00732515058906774,-0.0400874099068432,
-0.0112841927608144));
#33904=CARTESIAN_POINT('Ctrl Pts',(0.00747461521632705,-0.0400088954377018,
-0.0127895176351511));
#33905=CARTESIAN_POINT('Ctrl Pts',(0.00630133697214193,-0.0399303809685605,
-0.0137443795152512));
#33906=CARTESIAN_POINT('Ctrl Pts',(0.00485775389397871,-0.0398518664994192,
-0.0132922546602737));
#33907=CARTESIAN_POINT('Ctrl Pts',(0.00443877987189778,-0.0397733520302779,
-0.0118387051061822));
#33908=CARTESIAN_POINT('Ctrl Pts',(0.0054202378552023,-0.0396948375611365,
-0.0106875812386152));
#33909=CARTESIAN_POINT('Ctrl Pts',(0.00692174947831937,-0.0396163230919952,
-0.01087145471626));
#33910=CARTESIAN_POINT('Ctrl Pts',(0.00759644099572046,-0.0395378086228539,
-0.0122253887918938));
#33911=CARTESIAN_POINT('Ctrl Pts',(0.00683910651126841,-0.0394592941537125,
-0.0135348889636414));
#33912=CARTESIAN_POINT('Ctrl Pts',(0.00532908372490877,-0.0393807796845712,
-0.0136253183738586));
#33913=CARTESIAN_POINT('Ctrl Pts',(0.00442088063138974,-0.0393022652154299,
-0.01241556080784));
#33914=CARTESIAN_POINT('Ctrl Pts',(0.00492916590214617,-0.0392237507462886,
-0.010990782814838));
#33915=CARTESIAN_POINT('Ctrl Pts',(0.00639800177343982,-0.0391452362771472,
-0.0106290267698747));
#33916=CARTESIAN_POINT('Ctrl Pts',(0.00750982543898704,-0.0390667218080059,
-0.0116547920358649));
#33917=CARTESIAN_POINT('Ctrl Pts',(0.00726731818988206,-0.0389882073388646,
-0.0131479552824357));
#33918=CARTESIAN_POINT('Ctrl Pts',(0.00588801183678637,-0.0389096928697233,
-0.0137691317732312));
#33919=CARTESIAN_POINT('Ctrl Pts',(0.00460916016456105,-0.038831178400582,
-0.012961118996584));
#33920=CARTESIAN_POINT('Ctrl Pts',(0.00457790794227973,-0.0387526639314406,
-0.0114487137787985));
#33921=CARTESIAN_POINT('Ctrl Pts',(0.00582228877756173,-0.0386741494622993,
-0.0105885611239463));
#33922=CARTESIAN_POINT('Ctrl Pts',(0.00722607863648303,-0.038595634993158,
-0.0111522279384746));
#33923=CARTESIAN_POINT('Ctrl Pts',(0.00753006175412259,-0.0385171205240167,
-0.0126340985440969));
#33924=CARTESIAN_POINT('Ctrl Pts',(0.0064615617376323,-0.0384386060548753,
-0.01370491786047));
#33925=CARTESIAN_POINT('Ctrl Pts',(0.00497903551091831,-0.038360091585734,
-0.0134041484999088));
#33926=CARTESIAN_POINT('Ctrl Pts',(0.00441232622867113,-0.0382815771165927,
-0.0120015841647602));
#33927=CARTESIAN_POINT('Ctrl Pts',(0.00526977878550357,-0.0382030626474514,
-0.0107553411214825));
#33928=CARTESIAN_POINT('Ctrl Pts',(0.006782248103529,-0.03812454817831,
-0.0107833142068739));
#33929=CARTESIAN_POINT('Ctrl Pts',(0.0075930320630644,-0.0380460337091687,
-0.0120604104868537));
#33930=CARTESIAN_POINT('Ctrl Pts',(0.00697484729986451,-0.0379675192400273,
-0.0134410612705769));
#33931=CARTESIAN_POINT('Ctrl Pts',(0.00548221419114921,-0.037889004770886,
-0.0136868039227835));
#33932=CARTESIAN_POINT('Ctrl Pts',(0.00445403903564292,-0.0378104903017447,
-0.0125772100774068));
#33933=CARTESIAN_POINT('Ctrl Pts',(0.00481261253504416,-0.0377319758326034,
-0.0111075872320905));
#33934=CARTESIAN_POINT('Ctrl Pts',(0.00623627900374848,-0.037653461363462,
-0.0105962257199298));
#33935=CARTESIAN_POINT('Ctrl Pts',(0.00744801484850009,-0.0375749468943207,
-0.0115017804479003));
#33936=CARTESIAN_POINT('Ctrl Pts',(0.00736083644648552,-0.0374964324251795,
-0.0130120411143809));
#33937=CARTESIAN_POINT('Ctrl Pts',(0.0060530270721205,-0.037417917956038,
-0.013772124368346));
#33938=CARTESIAN_POINT('Ctrl Pts',(0.00469754397088331,-0.0373394034868968,
-0.0131005438710126));
#33939=CARTESIAN_POINT('Ctrl Pts',(0.0045105900856651,-0.0372608890177554,
-0.0115990942489104));
#33940=CARTESIAN_POINT('Ctrl Pts',(0.00565924088997368,-0.0371823745486141,
-0.010615809684489));
#33941=CARTESIAN_POINT('Ctrl Pts',(0.00711436712046152,-0.0371038600794727,
-0.0110303130560284));
#33942=CARTESIAN_POINT('Ctrl Pts',(0.0075683234991771,-0.0370253395304344,
-0.0124757382275885));
#33943=CARTESIAN_POINT('Ctrl Pts',(0.00693511855415113,-0.0369729904711097,
-0.0132548208617724));
#33944=CARTESIAN_POINT('Ctrl Pts',(0.00652352955908771,-0.0369468129014988,
-0.0134270329667855));
#33945=CARTESIAN_POINT('Ctrl Pts',(0.0065484519646357,-0.0410060465990872,
-0.0133114377905975));
#33946=CARTESIAN_POINT('Ctrl Pts',(0.00617492311894418,-0.0409798710258663,
-0.0134918460743052));
#33947=CARTESIAN_POINT('Ctrl Pts',(0.00524231934399881,-0.0409275239629315,
-0.0134525976544415));
#33948=CARTESIAN_POINT('Ctrl Pts',(0.00451567965527543,-0.0408490054102829,
-0.0122458250168071));
#33949=CARTESIAN_POINT('Ctrl Pts',(0.00512378003237285,-0.0407704909411417,
-0.0109772332685232));
#33950=CARTESIAN_POINT('Ctrl Pts',(0.00651625383110827,-0.0406919764720003,
-0.0107834025703192));
#33951=CARTESIAN_POINT('Ctrl Pts',(0.00744645748620972,-0.0406134620028589,
-0.0118388249498838));
#33952=CARTESIAN_POINT('Ctrl Pts',(0.00707875581291927,-0.0405349475337177,
-0.0131964593641061));
#33953=CARTESIAN_POINT('Ctrl Pts',(0.00574361027448316,-0.0404564330645763,
-0.0136386525749953));
#33954=CARTESIAN_POINT('Ctrl Pts',(0.00463834067387879,-0.040377918595435,
-0.01276867014408));
#33955=CARTESIAN_POINT('Ctrl Pts',(0.00475455076295656,-0.0402994041262936,
-0.0113669382882124));
#33956=CARTESIAN_POINT('Ctrl Pts',(0.00598791489830592,-0.0402208896571524,
-0.0106908053225104));
#33957=CARTESIAN_POINT('Ctrl Pts',(0.00723213399582761,-0.040142375188011,
-0.0113467812885753));
#33958=CARTESIAN_POINT('Ctrl Pts',(0.00737110721890075,-0.0400638607188697,
-0.0127464425555564));
#33959=CARTESIAN_POINT('Ctrl Pts',(0.00628018515830493,-0.0399853462497283,
-0.0136342796010194));
#33960=CARTESIAN_POINT('Ctrl Pts',(0.00493793183171677,-0.0399068317805871,
-0.0132138908476413));
#33961=CARTESIAN_POINT('Ctrl Pts',(0.0045483669473682,-0.0398283173114457,
-0.0118623706242104));
#33962=CARTESIAN_POINT('Ctrl Pts',(0.0054609332297836,-0.0397498028423044,
-0.0107920478530937));
#33963=CARTESIAN_POINT('Ctrl Pts',(0.00685704890994516,-0.0396712883731631,
-0.0109630146583807));
#33964=CARTESIAN_POINT('Ctrl Pts',(0.00748438165397041,-0.0395927739040217,
-0.0122219117350304));
#33965=CARTESIAN_POINT('Ctrl Pts',(0.00678020691926156,-0.0395142594348804,
-0.0134394938667997));
#33966=CARTESIAN_POINT('Ctrl Pts',(0.00537617750185241,-0.0394357449657391,
-0.0135235757450938));
#33967=CARTESIAN_POINT('Ctrl Pts',(0.00453172411227353,-0.0393572304965978,
-0.0123987349639038));
#33968=CARTESIAN_POINT('Ctrl Pts',(0.00500433120073897,-0.0392787160274565,
-0.0110739667329061));
#33969=CARTESIAN_POINT('Ctrl Pts',(0.00637006474547161,-0.0392002015583151,
-0.0107376035113427));
#33970=CARTESIAN_POINT('Ctrl Pts',(0.00740384592248502,-0.0391216870891738,
-0.0116913670053881));
#33971=CARTESIAN_POINT('Ctrl Pts',(0.00717836103924093,-0.0390431726200324,
-0.0130797203084755));
#33972=CARTESIAN_POINT('Ctrl Pts',(0.00589587264710569,-0.0389646581508911,
-0.0136572944181898));
#33973=CARTESIAN_POINT('Ctrl Pts',(0.00470678769784105,-0.0388861436817498,
-0.0129059986640441));
#33974=CARTESIAN_POINT('Ctrl Pts',(0.0046777291698248,-0.0388076292126085,
-0.0114997540457538));
#33975=CARTESIAN_POINT('Ctrl Pts',(0.00583476290135422,-0.0387291147434672,
-0.0106999782795971));
#33976=CARTESIAN_POINT('Ctrl Pts',(0.00714001622308571,-0.0386506002743258,
-0.0112240795026805));
#33977=CARTESIAN_POINT('Ctrl Pts',(0.00742266178540245,-0.0385720858051845,
-0.0126019328317044));
#33978=CARTESIAN_POINT('Ctrl Pts',(0.00642916323080688,-0.0384935713360431,
-0.0135975878870446));
#33979=CARTESIAN_POINT('Ctrl Pts',(0.00505070030085003,-0.0384150568669019,
-0.013317930497833));
#33980=CARTESIAN_POINT('Ctrl Pts',(0.00452377017066826,-0.0383365423977605,
-0.0120138166764086));
#33981=CARTESIAN_POINT('Ctrl Pts',(0.00532103536739272,-0.0382580279286192,
-0.010855051451268));
#33982=CARTESIAN_POINT('Ctrl Pts',(0.00672733958652042,-0.0381795134594779,
-0.0108810610155872));
#33983=CARTESIAN_POINT('Ctrl Pts',(0.00748121200529069,-0.0381009989903365,
-0.0120685137892491));
#33984=CARTESIAN_POINT('Ctrl Pts',(0.00690641962416429,-0.0380224845211952,
-0.0133522522420902));
#33985=CARTESIAN_POINT('Ctrl Pts',(0.00551855924684682,-0.0379439700520539,
-0.0135807454250589));
#33986=CARTESIAN_POINT('Ctrl Pts',(0.00456255502120176,-0.0378654555829126,
-0.0125490375499473));
#33987=CARTESIAN_POINT('Ctrl Pts',(0.00489595909033924,-0.0377869411137712,
-0.0111825722714365));
#33988=CARTESIAN_POINT('Ctrl Pts',(0.00621969381851428,-0.0377084266446299,
-0.0107071048728713));
#33989=CARTESIAN_POINT('Ctrl Pts',(0.00734637401667343,-0.0376299121754886,
-0.0115490957942202));
#33990=CARTESIAN_POINT('Ctrl Pts',(0.00726531494783229,-0.0375513977063472,
-0.0129533463941774));
#33991=CARTESIAN_POINT('Ctrl Pts',(0.0060493049309247,-0.037472883237206,
-0.0136600769534027));
#33992=CARTESIAN_POINT('Ctrl Pts',(0.00478896755977412,-0.0373943687680646,
-0.0130356368569142));
#33993=CARTESIAN_POINT('Ctrl Pts',(0.00461513657065499,-0.0373158542989233,
-0.0116395788257163));
#33994=CARTESIAN_POINT('Ctrl Pts',(0.00568315987079862,-0.0372373398297819,
-0.010725314175803));
#33995=CARTESIAN_POINT('Ctrl Pts',(0.00703614609862507,-0.0371588253606407,
-0.0111107222189887));
#33996=CARTESIAN_POINT('Ctrl Pts',(0.00745823781518362,-0.0370803048116022,
-0.0124546883364978));
#33997=CARTESIAN_POINT('Ctrl Pts',(0.00686947956723124,-0.0370279557522776,
-0.0131790846481745));
#33998=CARTESIAN_POINT('Ctrl Pts',(0.00648678133103831,-0.0370017781826666,
-0.0133392086301809));
#33999=CARTESIAN_POINT('Ctrl Pts',(0.00680869722628235,-0.0368513852118003,
-0.0134899528977776));
#34000=CARTESIAN_POINT('Ctrl Pts',(0.00706735492668958,-0.0368670469798486,
-0.0133307713422738));
#34001=CARTESIAN_POINT('Ctrl Pts',(0.00748740299124012,-0.0368983794779675,
-0.0128554401592746));
#34002=CARTESIAN_POINT('Ctrl Pts',(0.00761399556669309,-0.036945382706157,
-0.0119117220579786));
#34003=CARTESIAN_POINT('Ctrl Pts',(0.00719343876865978,-0.0369923574079242,
-0.0110581054138011));
#34004=CARTESIAN_POINT('Ctrl Pts',(0.00664452962814855,-0.0370236613796206,
-0.0107415249439345));
#34005=CARTESIAN_POINT('Ctrl Pts',(0.00634923972919489,-0.0370392946212466,
-0.010672896044278));
#34006=CARTESIAN_POINT('Ctrl Pts',(0.00445700002442818,-0.0406839559076129,
-0.0121761278505149));
#34007=CARTESIAN_POINT('Ctrl Pts',(0.00445699610157866,-0.0406827676486519,
-0.0121540821429041));
#34008=CARTESIAN_POINT('Ctrl Pts',(0.00445746464932956,-0.0406815592236051,
-0.0121320397232979));
#34009=CARTESIAN_POINT('Ctrl Pts',(0.00446156087853884,-0.0406762331732241,
-0.0120361258433312));
#34010=CARTESIAN_POINT('Ctrl Pts',(0.00447002471206943,-0.0406719777460916,
-0.0119625611665503));
#34011=CARTESIAN_POINT('Ctrl Pts',(0.00450200642077586,-0.0406621029460487,
-0.0117929836898513));
#34012=CARTESIAN_POINT('Ctrl Pts',(0.00452953269981767,-0.0406565356122923,
-0.0116980411010296));
#34013=CARTESIAN_POINT('Ctrl Pts',(0.00457463140256198,-0.0406499852539944,
-0.0115844750880577));
#34014=CARTESIAN_POINT('Ctrl Pts',(0.00458382523766999,-0.0406487381886269,
-0.0115627848288545));
#34015=CARTESIAN_POINT('Ctrl Pts',(0.00459988476268503,-0.0406466973971073,
-0.0115271881703461));
#34016=CARTESIAN_POINT('Ctrl Pts',(0.00460646965420429,-0.0406458946660406,
-0.0115131600629839));
#34017=CARTESIAN_POINT('Ctrl Pts',(0.00461987221006823,-0.040644325122731,
-0.0114856914810224));
#34018=CARTESIAN_POINT('Ctrl Pts',(0.00462667765992274,-0.0406435580169627,
-0.0114722470012902));
#34019=CARTESIAN_POINT('Ctrl Pts',(0.00464393981669878,-0.0406416825463828,
-0.0114393497688382));
#34020=CARTESIAN_POINT('Ctrl Pts',(0.00465461941167596,-0.0406405818082087,
-0.0114200174686332));
#34021=CARTESIAN_POINT('Ctrl Pts',(0.0047003606599803,-0.0406360947328233,
-0.0113412595959409));
#34022=CARTESIAN_POINT('Ctrl Pts',(0.0047389748587225,-0.0406328295109826,
-0.0112839868539343));
#34023=CARTESIAN_POINT('Ctrl Pts',(0.00483288730224696,-0.0406256990940078,
-0.01116304883702));
#34024=CARTESIAN_POINT('Ctrl Pts',(0.00488982378172016,-0.0406218727514404,
-0.0111009427466056));
#34025=CARTESIAN_POINT('Ctrl Pts',(0.00498023015181734,-0.0406160276615646,
-0.0110172126458984));
#34026=CARTESIAN_POINT('Ctrl Pts',(0.0050099234258388,-0.0406141378072767,
-0.0109917389892215));
#34027=CARTESIAN_POINT('Ctrl Pts',(0.00505052177962872,-0.0406115456802015,
-0.0109595053832507));
#34028=CARTESIAN_POINT('Ctrl Pts',(0.0050605906932869,-0.0406109021456263,
-0.0109517122619234));
#34029=CARTESIAN_POINT('Ctrl Pts',(0.00507760783578008,-0.0406098113526726,
-0.0109388749559681));
#34030=CARTESIAN_POINT('Ctrl Pts',(0.00508450402403877,-0.0406093684477241,
-0.0109337623838509));
#34031=CARTESIAN_POINT('Ctrl Pts',(0.00509908128073857,-0.0406084296674785,
-0.0109231427130448));
#34032=CARTESIAN_POINT('Ctrl Pts',(0.00510677085686588,-0.0406079330586185,
-0.0109176482123518));
#34033=CARTESIAN_POINT('Ctrl Pts',(0.0051287495830447,-0.0406065108169485,
-0.0109022465828717));
#34034=CARTESIAN_POINT('Ctrl Pts',(0.00514315603632636,-0.0406055752556271,
-0.0108925101137455));
#34035=CARTESIAN_POINT('Ctrl Pts',(0.00521103014543226,-0.0406011634196553,
-0.0108482903692046));
#34036=CARTESIAN_POINT('Ctrl Pts',(0.0052664305215898,-0.0405975531958185,
-0.0108168935806533));
#34037=CARTESIAN_POINT('Ctrl Pts',(0.00539748420550416,-0.0405892245417142,
-0.0107529759235915));
#34038=CARTESIAN_POINT('Ctrl Pts',(0.00547412838128347,-0.0405845083626427,
-0.0107229025251984));
#34039=CARTESIAN_POINT('Ctrl Pts',(0.00559877509581852,-0.0405772712952236,
-0.0106851573210044));
#34040=CARTESIAN_POINT('Ctrl Pts',(0.00564537132426037,-0.0405746545509841,
-0.0106733903033605));
#34041=CARTESIAN_POINT('Ctrl Pts',(0.00571161381318462,-0.0405710645317597,
-0.0106599162518569));
#34042=CARTESIAN_POINT('Ctrl Pts',(0.00573085658234744,-0.0405700366596072,
-0.0106563818151584));
#34043=CARTESIAN_POINT('Ctrl Pts',(0.00576466437083863,-0.0405682562475722,
-0.0106508345574724));
#34044=CARTESIAN_POINT('Ctrl Pts',(0.00577920034588751,-0.0405674989135889,
-0.0106486622328876));
#34045=CARTESIAN_POINT('Ctrl Pts',(0.00580971851370332,-0.0405659253011414,
-0.0106445463007741));
#34046=CARTESIAN_POINT('Ctrl Pts',(0.00582570460195273,-0.0405651103844024,
-0.0106426444725222));
#34047=CARTESIAN_POINT('Ctrl Pts',(0.00586874362620771,-0.0405629399170064,
-0.0106382060835627));
#34048=CARTESIAN_POINT('Ctrl Pts',(0.00589583910960418,-0.0405615984467416,
-0.0106361332559867));
#34049=CARTESIAN_POINT('Ctrl Pts',(0.00604250753895965,-0.0405544492504777,
-0.0106288026954927));
#34050=CARTESIAN_POINT('Ctrl Pts',(0.00616232398331993,-0.040549050050643,
-0.0106367547653879));
#34051=CARTESIAN_POINT('Ctrl Pts',(0.00634446625848518,-0.040540483688935,
-0.0106703677706405));
#34052=CARTESIAN_POINT('Ctrl Pts',(0.00640808321580915,-0.0405374112501371,
-0.010686353286068));
#34053=CARTESIAN_POINT('Ctrl Pts',(0.00648405816422829,-0.0405334481924993,
-0.0107106775967714));
#34054=CARTESIAN_POINT('Ctrl Pts',(0.00649756980070762,-0.0405327316741058,
-0.010715210833702));
#34055=CARTESIAN_POINT('Ctrl Pts',(0.00651927400125313,-0.0405315588967731,
-0.0107228288192166));
#34056=CARTESIAN_POINT('Ctrl Pts',(0.00652750674736777,-0.0405311089228818,
-0.0107257973512768));
#34057=CARTESIAN_POINT('Ctrl Pts',(0.00654388351128701,-0.0405302027661414,
-0.0107318603426371));
#34058=CARTESIAN_POINT('Ctrl Pts',(0.00655202741224689,-0.0405297466170746,
-0.0107349540454444));
#34059=CARTESIAN_POINT('Ctrl Pts',(0.00657340879416736,-0.0405285352403709,
-0.0107432842640634));
#34060=CARTESIAN_POINT('Ctrl Pts',(0.00658660055445618,-0.0405277738395995,
-0.0107486352193798));
#34061=CARTESIAN_POINT('Ctrl Pts',(0.00666077149675907,-0.0405234208719857,
-0.0107799230772966));
#34062=CARTESIAN_POINT('Ctrl Pts',(0.00672010007344723,-0.0405196643354348,
-0.0108095829422025));
#34063=CARTESIAN_POINT('Ctrl Pts',(0.00685064442419358,-0.0405110244120001,
-0.0108857155068935));
#34064=CARTESIAN_POINT('Ctrl Pts',(0.00692030822830832,-0.0405061408877977,
-0.0109344484631835));
#34065=CARTESIAN_POINT('Ctrl Pts',(0.00702316218686836,-0.0404987009356184,
-0.011019838640222));
#34066=CARTESIAN_POINT('Ctrl Pts',(0.00705921345389497,-0.040496039235344,
-0.0110527779329401));
#34067=CARTESIAN_POINT('Ctrl Pts',(0.0071074299575915,-0.0404924080911202,
-0.0111012232446214));
#34068=CARTESIAN_POINT('Ctrl Pts',(0.00712095060435605,-0.0404913811374663,
-0.0111153342500687));
#34069=CARTESIAN_POINT('Ctrl Pts',(0.00714407125483256,-0.0404896087988136,
-0.0111404007577633));
#34070=CARTESIAN_POINT('Ctrl Pts',(0.00715379076095117,-0.0404888584651087,
-0.0111512422020941));
#34071=CARTESIAN_POINT('Ctrl Pts',(0.00717374921729286,-0.0404873058563317,
-0.0111741486894487));
#34072=CARTESIAN_POINT('Ctrl Pts',(0.00718395898396545,-0.0404865048110825,
-0.0111862369605131));
#34073=CARTESIAN_POINT('Ctrl Pts',(0.00721067848335506,-0.0404843884115581,
-0.0112188781181165));
#34074=CARTESIAN_POINT('Ctrl Pts',(0.00722685078702089,-0.0404830862719446,
-0.0112397009972574));
#34075=CARTESIAN_POINT('Ctrl Pts',(0.00731389407794713,-0.0404759351358193,
-0.0113579071945071));
#34076=CARTESIAN_POINT('Ctrl Pts',(0.00737370471020973,-0.0404705085761867,
-0.0114629088327208));
#34077=CARTESIAN_POINT('Ctrl Pts',(0.00744447072214441,-0.0404621319215776,
-0.0116298995096336));
#34078=CARTESIAN_POINT('Ctrl Pts',(0.00746489839236045,-0.0404592819162149,
-0.0116873527649018));
#34079=CARTESIAN_POINT('Ctrl Pts',(0.00748659493362031,-0.0404554479791744,
-0.0117621246470168));
#34080=CARTESIAN_POINT('Ctrl Pts',(0.00749104669321343,-0.0404546024919145,
-0.0117784673287728));
#34081=CARTESIAN_POINT('Ctrl Pts',(0.00749751571499807,-0.0404532728482512,
-0.0118038566373665));
#34082=CARTESIAN_POINT('Ctrl Pts',(0.00749972211588009,-0.0404527985405521,
-0.0118128541260811));
#34083=CARTESIAN_POINT('Ctrl Pts',(0.00750374374615377,-0.040451892289061,
-0.0118299167589125));
#34084=CARTESIAN_POINT('Ctrl Pts',(0.0075055754037722,-0.0404514612376108,
-0.0118379775285717));
#34085=CARTESIAN_POINT('Ctrl Pts',(0.00750995898399796,-0.0404503832093031,
-0.0118580125093438));
#34086=CARTESIAN_POINT('Ctrl Pts',(0.00751243330170728,-0.0404497321888876,
-0.011870003024546));
#34087=CARTESIAN_POINT('Ctrl Pts',(0.00752110556584302,-0.040447286361925,
-0.011914710344225));
#34088=CARTESIAN_POINT('Ctrl Pts',(0.00752638634419614,-0.0404454508780432,
-0.0119475941422348));
#34089=CARTESIAN_POINT('Ctrl Pts',(0.00754497888917948,-0.040437226605193,
-0.012093357462402));
#34090=CARTESIAN_POINT('Ctrl Pts',(0.00754686015598122,-0.0404305949312341,
-0.0122073390250365));
#34091=CARTESIAN_POINT('Ctrl Pts',(0.00753100969887862,-0.0404211283651119,
-0.0123756783733293));
#34092=CARTESIAN_POINT('Ctrl Pts',(0.00752284458999184,-0.040418089782384,
-0.0124305414650205));
#34093=CARTESIAN_POINT('Ctrl Pts',(0.00750765375979262,-0.0404140515349914,
-0.0125048613369007));
#34094=CARTESIAN_POINT('Ctrl Pts',(0.00750316658639405,-0.0404129762687513,
-0.0125247894159469));
#34095=CARTESIAN_POINT('Ctrl Pts',(0.00749474935935628,-0.0404111433315053,
-0.0125589879895818));
#34096=CARTESIAN_POINT('Ctrl Pts',(0.00749100730240655,-0.0404103799286316,
-0.0125733015119272));
#34097=CARTESIAN_POINT('Ctrl Pts',(0.0074828709071067,-0.0404088196240522,
-0.0126026897296793));
#34098=CARTESIAN_POINT('Ctrl Pts',(0.0074784511532174,-0.0404080236265632,
-0.0126177556362907));
#34099=CARTESIAN_POINT('Ctrl Pts',(0.00746631116520551,-0.0404059634079913,
-0.0126569151840046));
#34100=CARTESIAN_POINT('Ctrl Pts',(0.00745822685667998,-0.0404047107968064,
-0.0126808914083417));
#34101=CARTESIAN_POINT('Ctrl Pts',(0.00740805250009144,-0.0403975576465919,
-0.012818428830889));
#34102=CARTESIAN_POINT('Ctrl Pts',(0.00735330142664926,-0.0403920863542759,
-0.012926913522509));
#34103=CARTESIAN_POINT('Ctrl Pts',(0.00725285110060169,-0.0403836684960879,
-0.0130785770801653));
#34104=CARTESIAN_POINT('Ctrl Pts',(0.00721631094840985,-0.0403808201076095,
-0.0131272379060661));
#34105=CARTESIAN_POINT('Ctrl Pts',(0.00716601669639092,-0.0403769876693734,
-0.0131865671440192));
#34106=CARTESIAN_POINT('Ctrl Pts',(0.00715482184829609,-0.0403761395138823,
-0.0131993394338739));
#34107=CARTESIAN_POINT('Ctrl Pts',(0.00713715072272266,-0.0403748035501098,
-0.0132188414827236));
#34108=CARTESIAN_POINT('Ctrl Pts',(0.00713082005269487,-0.0403743254874568,
-0.0132257019154294));
#34109=CARTESIAN_POINT('Ctrl Pts',(0.00711873780685018,-0.0403734131778912,
-0.0132385591514045));
#34110=CARTESIAN_POINT('Ctrl Pts',(0.00711299942685477,-0.0403729798366347,
-0.0132445676076484));
#34111=CARTESIAN_POINT('Ctrl Pts',(0.0070985989195325,-0.0403718927614918,
-0.0132594041062761));
#34112=CARTESIAN_POINT('Ctrl Pts',(0.00708987873219968,-0.0403712348863931,
-0.0132681748030421));
#34113=CARTESIAN_POINT('Ctrl Pts',(0.0070566187878232,-0.0403687305111979,
-0.0133008326219144));
#34114=CARTESIAN_POINT('Ctrl Pts',(0.00703139269156884,-0.0403668409588275,
-0.0133240042320652));
#34115=CARTESIAN_POINT('Ctrl Pts',(0.00692010081944446,-0.0403586214392957,
-0.0134196030894155));
#34116=CARTESIAN_POINT('Ctrl Pts',(0.00682702524387715,-0.0403520626058266,
-0.013483343505906));
#34117=CARTESIAN_POINT('Ctrl Pts',(0.00667920837637894,-0.0403426792068573,
-0.0135624199784625));
#34118=CARTESIAN_POINT('Ctrl Pts',(0.00662921079737098,-0.040339655832678,
-0.0135858128318754));
#34119=CARTESIAN_POINT('Ctrl Pts',(0.00655917756140508,-0.0403356350369595,
-0.0136141106948176));
#34120=CARTESIAN_POINT('Ctrl Pts',(0.00654014170196335,-0.0403345627209437,
-0.0136213673512695));
#34121=CARTESIAN_POINT('Ctrl Pts',(0.00650707195655613,-0.0403327343628347,
-0.013633229335486));
#34122=CARTESIAN_POINT('Ctrl Pts',(0.00649310569013887,-0.0403319726169784,
-0.0136380139190129));
#34123=CARTESIAN_POINT('Ctrl Pts',(0.00646417579907839,-0.0403304154388767,
-0.0136474630909198));
#34124=CARTESIAN_POINT('Ctrl Pts',(0.00644920542371297,-0.0403296209134209,
-0.0136521016053768));
#34125=CARTESIAN_POINT('Ctrl Pts',(0.00640993197412165,-0.0403275643903645,
-0.0136636175800836));
#34126=CARTESIAN_POINT('Ctrl Pts',(0.00638552576299623,-0.0403263139982011,
-0.0136701279567808));
#34127=CARTESIAN_POINT('Ctrl Pts',(0.00623320364824762,-0.0403186601895055,
-0.013706779273515));
#34128=CARTESIAN_POINT('Ctrl Pts',(0.00610204122454998,-0.0403127777734839,
-0.0137210736470574));
#34129=CARTESIAN_POINT('Ctrl Pts',(0.00591345249454654,-0.0403040111900056,
-0.0137174860241215));
#34130=CARTESIAN_POINT('Ctrl Pts',(0.00585636212974602,-0.0403013071018868,
-0.0137132176141899));
#34131=CARTESIAN_POINT('Ctrl Pts',(0.00578588165647265,-0.0402977721336892,
-0.0137039877813217));
#34132=CARTESIAN_POINT('Ctrl Pts',(0.0057721429582911,-0.0402970736313834,
-0.0137019996893812));
#34133=CARTESIAN_POINT('Ctrl Pts',(0.00574987531796092,-0.0402959235191177,
-0.0136984700224787));
#34134=CARTESIAN_POINT('Ctrl Pts',(0.0057413289620749,-0.0402954777799242,
-0.0136970414307356));
#34135=CARTESIAN_POINT('Ctrl Pts',(0.0057251653300398,-0.0402946258109353,
-0.0136941993997607));
#34136=CARTESIAN_POINT('Ctrl Pts',(0.00571754579026297,-0.0402942204276567,
-0.0136928004279197));
#34137=CARTESIAN_POINT('Ctrl Pts',(0.00569662647892313,-0.0402930977046662,
-0.0136887965024294));
#34138=CARTESIAN_POINT('Ctrl Pts',(0.00568335025939411,-0.0402923743131018,
-0.0136860736630137));
#34139=CARTESIAN_POINT('Ctrl Pts',(0.00562415315508727,-0.0402891053116787,
-0.0136731179736892));
#34140=CARTESIAN_POINT('Ctrl Pts',(0.00557868142717328,-0.0402864773429017,
-0.0136609635241214));
#34141=CARTESIAN_POINT('Ctrl Pts',(0.00543821427708631,-0.0402781281298423,
-0.0136164463705754));
#34142=CARTESIAN_POINT('Ctrl Pts',(0.00534576417179183,-0.0402723104351218,
-0.0135768847893157));
#34143=CARTESIAN_POINT('Ctrl Pts',(0.00521155400225171,-0.04026375968715,
-0.0135032512796518));
#34144=CARTESIAN_POINT('Ctrl Pts',(0.00516662819587161,-0.0402608731294837,
-0.0134755166229041));
#34145=CARTESIAN_POINT('Ctrl Pts',(0.00510667925255735,-0.0402569977364808,
-0.013434118176001));
#34146=CARTESIAN_POINT('Ctrl Pts',(0.00509037432770296,-0.0402559409159203,
-0.0134223819368332));
#34147=CARTESIAN_POINT('Ctrl Pts',(0.0050625381934056,-0.0402541310681055,
-0.0134015084539686));
#34148=CARTESIAN_POINT('Ctrl Pts',(0.00505090015735443,-0.0402533726133902,
-0.0133925187033156));
#34149=CARTESIAN_POINT('Ctrl Pts',(0.00502707169803573,-0.0402518153237023,
-0.0133735625070618));
#34150=CARTESIAN_POINT('Ctrl Pts',(0.0050149017174851,-0.0402510175137377,
-0.0133635730575938));
#34151=CARTESIAN_POINT('Ctrl Pts',(0.00498328798146628,-0.0402489370394154,
-0.0133368034064114));
#34152=CARTESIAN_POINT('Ctrl Pts',(0.00496410625415742,-0.0402476665561709,
-0.0133197207388894));
#34153=CARTESIAN_POINT('Ctrl Pts',(0.00486887362719248,-0.0402412991041479,
-0.0132305482003861));
#34154=CARTESIAN_POINT('Ctrl Pts',(0.00479988196266337,-0.0402365091211676,
-0.0131513258032048));
#34155=CARTESIAN_POINT('Ctrl Pts',(0.00469250865091143,-0.0402279443321174,
-0.0129992244577492));
#34156=CARTESIAN_POINT('Ctrl Pts',(0.0046509079311341,-0.0402241865076432,
-0.0129291273235219));
#34157=CARTESIAN_POINT('Ctrl Pts',(0.00460859068870627,-0.0402194246455536,
-0.0128429684761729));
#34158=CARTESIAN_POINT('Ctrl Pts',(0.00460233529864465,-0.040218690819738,
-0.0128297614618998));
#34159=CARTESIAN_POINT('Ctrl Pts',(0.00459260879323672,-0.0402174973655215,
-0.0128084484958542));
#34160=CARTESIAN_POINT('Ctrl Pts',(0.00458901782168303,-0.0402170444771133,
-0.0128003979150007));
#34161=CARTESIAN_POINT('Ctrl Pts',(0.0045820272196626,-0.0402161371802396,
-0.012784357667434));
#34162=CARTESIAN_POINT('Ctrl Pts',(0.00457862566748462,-0.0402156828997755,
-0.0127763692196311));
#34163=CARTESIAN_POINT('Ctrl Pts',(0.0045699320362051,-0.0402144886410961,
-0.012755464747554));
#34164=CARTESIAN_POINT('Ctrl Pts',(0.00456474756445648,-0.0402137428537678,
-0.0127425050729073));
#34165=CARTESIAN_POINT('Ctrl Pts',(0.00453997078154124,-0.0402100132472505,
-0.01267804794355));
#34166=CARTESIAN_POINT('Ctrl Pts',(0.00452297206170388,-0.0402069161419197,
-0.0126256002669764));
#34167=CARTESIAN_POINT('Ctrl Pts',(0.00448478516591968,-0.0401984585186114,
-0.0124819869868053));
#34168=CARTESIAN_POINT('Ctrl Pts',(0.00446901849805195,-0.0401930544215412,
-0.0123896088971841));
#34169=CARTESIAN_POINT('Ctrl Pts',(0.00445857228063263,-0.0401855955796433,
-0.0122562726149411));
#34170=CARTESIAN_POINT('Ctrl Pts',(0.00445700000019507,-0.0401833878786776,
-0.0122160697976288));
#34171=CARTESIAN_POINT('Ctrl Pts',(0.004457,-0.0401812248373849,-0.0121758532940426));
#34172=CARTESIAN_POINT('Ctrl Pts',(0.00510755223020394,-0.0408418305049472,
-0.0112835843270982));
#34173=CARTESIAN_POINT('Ctrl Pts',(0.00540310700475264,-0.0408154711366772,
-0.0109879656812376));
#34174=CARTESIAN_POINT('Ctrl Pts',(0.0063059411121766,-0.0407627550577508,
-0.0107184895915512));
#34175=CARTESIAN_POINT('Ctrl Pts',(0.00739033724866104,-0.0406836822681679,
-0.0116385674487439));
#34176=CARTESIAN_POINT('Ctrl Pts',(0.00720783737929209,-0.0406046121361985,
-0.0130470858798218));
#34177=CARTESIAN_POINT('Ctrl Pts',(0.00592950186608492,-0.0405255420042292,
-0.0136637827569462));
#34178=CARTESIAN_POINT('Ctrl Pts',(0.00471435818957979,-0.0404464718722598,
-0.0129284907266282));
#34179=CARTESIAN_POINT('Ctrl Pts',(0.00466790546059575,-0.0403674017402905,
-0.0115092477749536));
#34180=CARTESIAN_POINT('Ctrl Pts',(0.00583168420583166,-0.0402883316083211,
-0.0106957608437662));
#34181=CARTESIAN_POINT('Ctrl Pts',(0.00714852543999728,-0.0402092614763518,
-0.0112272060724861));
#34182=CARTESIAN_POINT('Ctrl Pts',(0.00742165614668327,-0.0401301913443825,
-0.0126206807356106));
#34183=CARTESIAN_POINT('Ctrl Pts',(0.00640297533227296,-0.0400511212124132,
-0.0136099434274877));
#34184=CARTESIAN_POINT('Ctrl Pts',(0.00501810018683856,-0.0399720510804438,
-0.0132960670082253));
#34185=CARTESIAN_POINT('Ctrl Pts',(0.00452547350724074,-0.0398929809484745,
-0.0119642651766415));
#34186=CARTESIAN_POINT('Ctrl Pts',(0.00537272725475431,-0.0398139108165052,
-0.0108247312644503));
#34187=CARTESIAN_POINT('Ctrl Pts',(0.0067899782676088,-0.0397348406845358,
-0.0109129454936839));
#34188=CARTESIAN_POINT('Ctrl Pts',(0.00748938447730575,-0.0396557705525665,
-0.0121487489266506));
#34189=CARTESIAN_POINT('Ctrl Pts',(0.00683540547876292,-0.0395767004205972,
-0.0134091817184311));
#34190=CARTESIAN_POINT('Ctrl Pts',(0.00542230329908635,-0.0394976302886279,
-0.013548903831367));
#34191=CARTESIAN_POINT('Ctrl Pts',(0.00453414730039512,-0.0394185601566585,
-0.0124409514268199));
#34192=CARTESIAN_POINT('Ctrl Pts',(0.00497799393576915,-0.0393394900246892,
-0.0110921075389659));
#34193=CARTESIAN_POINT('Ctrl Pts',(0.00635052521873909,-0.0392604198927198,
-0.0107280503657344));
#34194=CARTESIAN_POINT('Ctrl Pts',(0.00740453843513532,-0.0391813497607505,
-0.0116795942838205));
#34195=CARTESIAN_POINT('Ctrl Pts',(0.0071822644889926,-0.0391022796287812,
-0.0130820827843013));
#34196=CARTESIAN_POINT('Ctrl Pts',(0.00588568102543133,-0.0390232094968118,
-0.0136610914472305));
#34197=CARTESIAN_POINT('Ctrl Pts',(0.00469297784078796,-0.0389441393648425,
-0.0128904820682789));
#34198=CARTESIAN_POINT('Ctrl Pts',(0.00468794996067798,-0.0388650692328732,
-0.0114704981162847));
#34199=CARTESIAN_POINT('Ctrl Pts',(0.00587516616144298,-0.0387859991009039,
-0.0106914619181288));
#34200=CARTESIAN_POINT('Ctrl Pts',(0.00717581736826139,-0.0387069289689345,
-0.0112612742922497));
#34201=CARTESIAN_POINT('Ctrl Pts',(0.00740801748443278,-0.0386278588369652,
-0.0126621535902753));
#34202=CARTESIAN_POINT('Ctrl Pts',(0.00636076905686384,-0.0385487887049958,
-0.0136211376572347));
#34203=CARTESIAN_POINT('Ctrl Pts',(0.00498569413162669,-0.0384697185730265,
-0.0132668092063614));
#34204=CARTESIAN_POINT('Ctrl Pts',(0.00453230673704881,-0.0383906484410572,
-0.0119211422494873));
#34205=CARTESIAN_POINT('Ctrl Pts',(0.00541259455569142,-0.0383115783090878,
-0.0108069281298219));
#34206=CARTESIAN_POINT('Ctrl Pts',(0.00682665061441721,-0.0382325081771185,
-0.0109366398575666));
#34207=CARTESIAN_POINT('Ctrl Pts',(0.00748953924320393,-0.0381534380451492,
-0.0121924098502718));
#34208=CARTESIAN_POINT('Ctrl Pts',(0.00679890142091577,-0.0380743679131799,
-0.0134331352177383));
#34209=CARTESIAN_POINT('Ctrl Pts',(0.00538231162445055,-0.0379952977812105,
-0.0135313833814939));
#34210=CARTESIAN_POINT('Ctrl Pts',(0.00452700756245122,-0.0379162276492412,
-0.0123978781399435));
#34211=CARTESIAN_POINT('Ctrl Pts',(0.00501019450630097,-0.0378371575172719,
-0.0110626206513034));
#34212=CARTESIAN_POINT('Ctrl Pts',(0.0063928048011601,-0.0377580873853025,
-0.0107389460890354));
#34213=CARTESIAN_POINT('Ctrl Pts',(0.00741848003443745,-0.0376790172533332,
-0.0117209682272295));
#34214=CARTESIAN_POINT('Ctrl Pts',(0.00715519574970712,-0.0375999471213639,
-0.0131163459396875));
#34215=CARTESIAN_POINT('Ctrl Pts',(0.00584220638794218,-0.0375208769893944,
-0.0136570956147497));
#34216=CARTESIAN_POINT('Ctrl Pts',(0.00467258771297713,-0.0374418068574252,
-0.0128518849746824));
#34217=CARTESIAN_POINT('Ctrl Pts',(0.00470920090848562,-0.0373627367254559,
-0.0114323201325417));
#34218=CARTESIAN_POINT('Ctrl Pts',(0.00591869234964484,-0.0372836665934865,
-0.0106884972982332));
#34219=CARTESIAN_POINT('Ctrl Pts',(0.00720217534268384,-0.0372045964615172,
-0.0112960166958557));
#34220=CARTESIAN_POINT('Ctrl Pts',(0.00739304429033509,-0.0371255263295479,
-0.0127034247991513));
#34221=CARTESIAN_POINT('Ctrl Pts',(0.0063184850578249,-0.0370464561975785,
-0.0136306675820344));
#34222=CARTESIAN_POINT('Ctrl Pts',(0.00495370982778676,-0.0369673860656093,
-0.0132374514271274));
#34223=CARTESIAN_POINT('Ctrl Pts',(0.00454129505257269,-0.0368883158002724,
-0.0118764800191924));
#34224=CARTESIAN_POINT('Ctrl Pts',(0.00514779084977581,-0.0368356022455921,
-0.0111555318307725));
#34225=CARTESIAN_POINT('Ctrl Pts',(0.00553656972522908,-0.0368092454015681,
-0.0110020392895787));
#34226=CARTESIAN_POINT('Ctrl Pts',(0.00504057926485683,-0.0408965082243162,
-0.011216624780417));
#34227=CARTESIAN_POINT('Ctrl Pts',(0.00535831368996204,-0.0408701488560462,
-0.0108988216908329));
#34228=CARTESIAN_POINT('Ctrl Pts',(0.00632890019639147,-0.0408174327771198,
-0.0106091230027746));
#34229=CARTESIAN_POINT('Ctrl Pts',(0.00749467389616782,-0.0407383599875368,
-0.0115982473011506));
#34230=CARTESIAN_POINT('Ctrl Pts',(0.00729847848310348,-0.0406592898555674,
-0.0131124667707295));
#34231=CARTESIAN_POINT('Ctrl Pts',(0.00592421139504614,-0.0405802197235982,
-0.0137754431277062));
#34232=CARTESIAN_POINT('Ctrl Pts',(0.00461787832002084,-0.0405011495916288,
-0.0129849717475897));
#34233=CARTESIAN_POINT('Ctrl Pts',(0.0045679395864617,-0.0404220794596595,
-0.0114592229451094));
#34234=CARTESIAN_POINT('Ctrl Pts',(0.00581905309370203,-0.0403430093276902,
-0.0105846885959143));
#34235=CARTESIAN_POINT('Ctrl Pts',(0.00723471553099929,-0.0402639391957208,
-0.0111560156688065));
#34236=CARTESIAN_POINT('Ctrl Pts',(0.00752834309360578,-0.0401848690637515,
-0.0126540624239728));
#34237=CARTESIAN_POINT('Ctrl Pts',(0.00643321626499464,-0.0401057989317822,
-0.0137175634726755));
#34238=CARTESIAN_POINT('Ctrl Pts',(0.00494441437083125,-0.0400267287998128,
-0.0133801324709917));
#34239=CARTESIAN_POINT('Ctrl Pts',(0.00441481895125976,-0.0399476586678434,
-0.0119483867312771));
#34240=CARTESIAN_POINT('Ctrl Pts',(0.00532565411809312,-0.0398685885358742,
-0.0107233374894542));
#34241=CARTESIAN_POINT('Ctrl Pts',(0.00684926149843999,-0.0397895184039048,
-0.0108181716786648));
#34242=CARTESIAN_POINT('Ctrl Pts',(0.00760115403779219,-0.0397104482719355,
-0.0121467149035757));
#34243=CARTESIAN_POINT('Ctrl Pts',(0.0068980977550771,-0.0396313781399662,
-0.0135017357760746));
#34244=CARTESIAN_POINT('Ctrl Pts',(0.00537895055347951,-0.0395523080079968,
-0.0136519432132442));
#34245=CARTESIAN_POINT('Ctrl Pts',(0.00442414366166439,-0.0394732378760275,
-0.0124608454857914));
#34246=CARTESIAN_POINT('Ctrl Pts',(0.0049012983810927,-0.0393941677440582,
-0.0110107787835418));
#34247=CARTESIAN_POINT('Ctrl Pts',(0.00637683007838732,-0.0393150976120888,
-0.0106194012569266));
#34248=CARTESIAN_POINT('Ctrl Pts',(0.00750994079830842,-0.0392360274801195,
-0.0116423529593213));
#34249=CARTESIAN_POINT('Ctrl Pts',(0.00727098649753159,-0.0391569573481502,
-0.0131500899874149));
#34250=CARTESIAN_POINT('Ctrl Pts',(0.00587710205758417,-0.0390778872161808,
-0.0137725498509977));
#34251=CARTESIAN_POINT('Ctrl Pts',(0.00459489350158125,-0.0389988170842115,
-0.0129441107625892));
#34252=CARTESIAN_POINT('Ctrl Pts',(0.0045894883085889,-0.0389197469522422,
-0.0114175653520659));
#34253=CARTESIAN_POINT('Ctrl Pts',(0.00586579811478878,-0.0388406768202728,
-0.0105800670611478));
#34254=CARTESIAN_POINT('Ctrl Pts',(0.00726405555824212,-0.0387616066883035,
-0.0111926405084406));
#34255=CARTESIAN_POINT('Ctrl Pts',(0.00751368092982937,-0.0386825365563341,
-0.0126986475728829));
#34256=CARTESIAN_POINT('Ctrl Pts',(0.00638784265641935,-0.0386034664243649,
-0.013729597763641));
#34257=CARTESIAN_POINT('Ctrl Pts',(0.00490957643143956,-0.0385243962923955,
-0.0133486790428774));
#34258=CARTESIAN_POINT('Ctrl Pts',(0.00442216497484537,-0.0384453261604262,
-0.0119020276816251));
#34259=CARTESIAN_POINT('Ctrl Pts',(0.00536851322589506,-0.0383662560284569,
-0.0107041983340985));
#34260=CARTESIAN_POINT('Ctrl Pts',(0.00688868588956419,-0.0382871858964875,
-0.0108436441654417));
#34261=CARTESIAN_POINT('Ctrl Pts',(0.00760132041796233,-0.0382081157645182,
-0.0121936523231709));
#34262=CARTESIAN_POINT('Ctrl Pts',(0.00685885428201276,-0.0381290456325488,
-0.013527486844868));
#34263=CARTESIAN_POINT('Ctrl Pts',(0.00533595773846292,-0.0380499755005795,
-0.0136331079564748));
#34264=CARTESIAN_POINT('Ctrl Pts',(0.00441646812830693,-0.0379709053686102,
-0.0124145398016286));
#34265=CARTESIAN_POINT('Ctrl Pts',(0.00493591541538556,-0.0378918352366409,
-0.0109790790780847));
#34266=CARTESIAN_POINT('Ctrl Pts',(0.00642228249523544,-0.0378127651046715,
-0.01063111464029));
#34267=CARTESIAN_POINT('Ctrl Pts',(0.00752492863278372,-0.0377336949727022,
-0.0116868317742668));
#34268=CARTESIAN_POINT('Ctrl Pts',(0.00724188640828986,-0.0376546248407329,
-0.0131869243914458));
#34269=CARTESIAN_POINT('Ctrl Pts',(0.0058303649038016,-0.0375755547087635,
-0.0137682541547496));
#34270=CARTESIAN_POINT('Ctrl Pts',(0.00457297321439364,-0.0374964845767942,
-0.0129026171837311));
#34271=CARTESIAN_POINT('Ctrl Pts',(0.00461233401526018,-0.0374174144448248,
-0.011376522334795));
#34272=CARTESIAN_POINT('Ctrl Pts',(0.00591259068786246,-0.0373383443128556,
-0.010576879963935));
#34273=CARTESIAN_POINT('Ctrl Pts',(0.00729239154389094,-0.0372592741808862,
-0.0112299901254563));
#34274=CARTESIAN_POINT('Ctrl Pts',(0.00749758408542575,-0.0371802040489169,
-0.0127430159436719));
#34275=CARTESIAN_POINT('Ctrl Pts',(0.00634238549151208,-0.0371011339169475,
-0.0137398428533443));
#34276=CARTESIAN_POINT('Ctrl Pts',(0.004875191893384,-0.0370220637849782,
-0.0133171181346785));
#34277=CARTESIAN_POINT('Ctrl Pts',(0.00443182781067669,-0.0369429935196414,
-0.0118540138131692));
#34278=CARTESIAN_POINT('Ctrl Pts',(0.00508383755657679,-0.0368902799649611,
-0.011078962696069));
#34279=CARTESIAN_POINT('Ctrl Pts',(0.00550179200401839,-0.0368639231209372,
-0.0109139514408505));
#34280=CARTESIAN_POINT('Ctrl Pts',(0.0049736062995096,-0.0409511859436854,
-0.0111496652337357));
#34281=CARTESIAN_POINT('Ctrl Pts',(0.00531352037517144,-0.0409248265754152,
-0.0108096777004281));
#34282=CARTESIAN_POINT('Ctrl Pts',(0.00635185928060625,-0.0408721104964888,
-0.0104997564139979));
#34283=CARTESIAN_POINT('Ctrl Pts',(0.00759901054367472,-0.0407930377069059,
-0.0115579271535574));
#34284=CARTESIAN_POINT('Ctrl Pts',(0.00738911958691479,-0.0407139675749367,
-0.0131778476616374));
#34285=CARTESIAN_POINT('Ctrl Pts',(0.00591892092400736,-0.0406348974429673,
-0.0138871034984661));
#34286=CARTESIAN_POINT('Ctrl Pts',(0.0045213984504619,-0.040555827310998,
-0.0130414527685509));
#34287=CARTESIAN_POINT('Ctrl Pts',(0.00446797371232754,-0.0404767571790286,
-0.0114091981152651));
#34288=CARTESIAN_POINT('Ctrl Pts',(0.00580642198157228,-0.0403976870470593,
-0.0104736163480623));
#34289=CARTESIAN_POINT('Ctrl Pts',(0.00732090562200129,-0.0403186169150899,
-0.011084825265127));
#34290=CARTESIAN_POINT('Ctrl Pts',(0.0076350300405283,-0.0402395467831207,
-0.0126874441123349));
#34291=CARTESIAN_POINT('Ctrl Pts',(0.00646345719771645,-0.0401604766511513,
-0.0138251835178632));
#34292=CARTESIAN_POINT('Ctrl Pts',(0.00487072855482406,-0.040081406519182,
-0.0134641979337579));
#34293=CARTESIAN_POINT('Ctrl Pts',(0.00430416439527867,-0.0400023363872126,
-0.0119325082859126));
#34294=CARTESIAN_POINT('Ctrl Pts',(0.00527858098143203,-0.0399232662552434,
-0.0106219437144581));
#34295=CARTESIAN_POINT('Ctrl Pts',(0.00690854472927117,-0.039844196123274,
-0.0107233978636457));
#34296=CARTESIAN_POINT('Ctrl Pts',(0.00771292359827863,-0.0397651259913046,
-0.0121446808805009));
#34297=CARTESIAN_POINT('Ctrl Pts',(0.0069607900313913,-0.0396860558593353,
-0.0135942898337181));
#34298=CARTESIAN_POINT('Ctrl Pts',(0.00533559780787254,-0.039606985727366,
-0.0137549825951213));
#34299=CARTESIAN_POINT('Ctrl Pts',(0.00431414002293365,-0.0395279155953967,
-0.012480739544763));
#34300=CARTESIAN_POINT('Ctrl Pts',(0.00482460282641615,-0.0394488454634273,
-0.0109294500281175));
#34301=CARTESIAN_POINT('Ctrl Pts',(0.00640313493803564,-0.039369775331458,
-0.0105107521481187));
#34302=CARTESIAN_POINT('Ctrl Pts',(0.0076153431614815,-0.0392907051994886,
-0.0116051116348221));
#34303=CARTESIAN_POINT('Ctrl Pts',(0.00735970850607058,-0.0392116350675194,
-0.0132180971905287));
#34304=CARTESIAN_POINT('Ctrl Pts',(0.00586852308973702,-0.03913256493555,
-0.0138840082547647));
#34305=CARTESIAN_POINT('Ctrl Pts',(0.00449680916237462,-0.0390534948035806,
-0.0129977394568994));
#34306=CARTESIAN_POINT('Ctrl Pts',(0.00449102665649993,-0.0389744246716113,
-0.0113646325878472));
#34307=CARTESIAN_POINT('Ctrl Pts',(0.00585643006813467,-0.0388953545396419,
-0.0104686722041668));
#34308=CARTESIAN_POINT('Ctrl Pts',(0.00735229374822285,-0.0388162844076727,
-0.0111240067246316));
#34309=CARTESIAN_POINT('Ctrl Pts',(0.00761934437522596,-0.0387372142757033,
-0.0127351415554907));
#34310=CARTESIAN_POINT('Ctrl Pts',(0.00641491625597485,-0.038658144143734,
-0.0138380578700472));
#34311=CARTESIAN_POINT('Ctrl Pts',(0.00483345873125242,-0.0385790740117646,
-0.0134305488793935));
#34312=CARTESIAN_POINT('Ctrl Pts',(0.00431202321264183,-0.0385000038797954,
-0.0118829131137628));
#34313=CARTESIAN_POINT('Ctrl Pts',(0.00532443189609871,-0.038420933747826,
-0.0106014685383751));
#34314=CARTESIAN_POINT('Ctrl Pts',(0.00695072116471118,-0.0383418636158567,
-0.0107506484733166));
#34315=CARTESIAN_POINT('Ctrl Pts',(0.00771310159272074,-0.0382627934838874,
-0.01219489479607));
#34316=CARTESIAN_POINT('Ctrl Pts',(0.00691880714310953,-0.038183723351918,
-0.0136218384719977));
#34317=CARTESIAN_POINT('Ctrl Pts',(0.00528960385247539,-0.0381046532199487,
-0.0137348325314557));
#34318=CARTESIAN_POINT('Ctrl Pts',(0.00430592869416266,-0.0380255830879794,
-0.0124312014633137));
#34319=CARTESIAN_POINT('Ctrl Pts',(0.00486163632447015,-0.03794651295601,
-0.0108955375048661));
#34320=CARTESIAN_POINT('Ctrl Pts',(0.0064517601893108,-0.0378674428240407,
-0.0105232831915444));
#34321=CARTESIAN_POINT('Ctrl Pts',(0.00763137723112998,-0.0377883726920714,
-0.0116526953213039));
#34322=CARTESIAN_POINT('Ctrl Pts',(0.0073285770668726,-0.037709302560102,
-0.013257502843204));
#34323=CARTESIAN_POINT('Ctrl Pts',(0.00581852341966102,-0.0376302324281327,
-0.0138794126947496));
#34324=CARTESIAN_POINT('Ctrl Pts',(0.00447335871581017,-0.0375511622961633,
-0.0129533493927798));
#34325=CARTESIAN_POINT('Ctrl Pts',(0.00451546712203466,-0.0374720921641941,
-0.0113207245370486));
#34326=CARTESIAN_POINT('Ctrl Pts',(0.00590648902608009,-0.0373930220322247,
-0.0104652626296369));
#34327=CARTESIAN_POINT('Ctrl Pts',(0.00738260774509806,-0.0373139519002554,
-0.0111639635550568));
#34328=CARTESIAN_POINT('Ctrl Pts',(0.00760212388051653,-0.037234881768286,
-0.0127826070881925));
#34329=CARTESIAN_POINT('Ctrl Pts',(0.00636628592519926,-0.0371558116363166,
-0.0138490181246544));
#34330=CARTESIAN_POINT('Ctrl Pts',(0.00479667395898134,-0.0370767415043474,
-0.0133967848422295));
#34331=CARTESIAN_POINT('Ctrl Pts',(0.00432236056878079,-0.0369976712390105,
-0.011831547607146));
#34332=CARTESIAN_POINT('Ctrl Pts',(0.00501988426337788,-0.0369449576843301,
-0.0110023935613656));
#34333=CARTESIAN_POINT('Ctrl Pts',(0.0054670142828077,-0.0369186008403063,
-0.010825863592122));
#34334=CARTESIAN_POINT('Ctrl Pts',(0.0049066333341625,-0.0410058636630544,
-0.0110827056870545));
#34335=CARTESIAN_POINT('Ctrl Pts',(0.00526872706038073,-0.0409795042947844,
-0.0107205337100233));
#34336=CARTESIAN_POINT('Ctrl Pts',(0.00637481836482103,-0.0409267882158579,
-0.0103903898252213));
#34337=CARTESIAN_POINT('Ctrl Pts',(0.00770334719118149,-0.040847715426275,
-0.0115176070059642));
#34338=CARTESIAN_POINT('Ctrl Pts',(0.00747976069072619,-0.0407686452943056,
-0.0132432285525452));
#34339=CARTESIAN_POINT('Ctrl Pts',(0.00591363045296858,-0.0406895751623363,
-0.0139987638692261));
#34340=CARTESIAN_POINT('Ctrl Pts',(0.00442491858090285,-0.040610505030367,
-0.0130979337895123));
#34341=CARTESIAN_POINT('Ctrl Pts',(0.0043680078381935,-0.0405314348983977,
-0.0113591732854209));
#34342=CARTESIAN_POINT('Ctrl Pts',(0.00579379086944254,-0.0404523647664283,
-0.0103625441002104));
#34343=CARTESIAN_POINT('Ctrl Pts',(0.0074070957130034,-0.0403732946344591,
-0.0110136348614473));
#34344=CARTESIAN_POINT('Ctrl Pts',(0.00774171698745092,-0.0402942245024896,
-0.0127208258006971));
#34345=CARTESIAN_POINT('Ctrl Pts',(0.00649369813043813,-0.0402151543705203,
-0.013932803563051));
#34346=CARTESIAN_POINT('Ctrl Pts',(0.00479704273881685,-0.0401360842385509,
-0.0135482633965242));
#34347=CARTESIAN_POINT('Ctrl Pts',(0.00419350983929769,-0.0400570141065816,
-0.0119166298405482));
#34348=CARTESIAN_POINT('Ctrl Pts',(0.00523150784477083,-0.0399779439746123,
-0.0105205499394621));
#34349=CARTESIAN_POINT('Ctrl Pts',(0.00696782796010235,-0.0398988738426429,
-0.0106286240486267));
#34350=CARTESIAN_POINT('Ctrl Pts',(0.00782469315876507,-0.0398198037106736,
-0.0121426468574261));
#34351=CARTESIAN_POINT('Ctrl Pts',(0.00702348230770549,-0.0397407335787043,
-0.0136868438913615));
#34352=CARTESIAN_POINT('Ctrl Pts',(0.00529224506226558,-0.039661663446735,
-0.0138580219769984));
#34353=CARTESIAN_POINT('Ctrl Pts',(0.00420413638420291,-0.0395825933147656,
-0.0125006336037345));
#34354=CARTESIAN_POINT('Ctrl Pts',(0.0047479072717396,-0.0395035231827963,
-0.0108481212726933));
#34355=CARTESIAN_POINT('Ctrl Pts',(0.00642943979768396,-0.0394244530508269,
-0.0104021030393109));
#34356=CARTESIAN_POINT('Ctrl Pts',(0.0077207455246546,-0.0393453829188576,
-0.011567870310323));
#34357=CARTESIAN_POINT('Ctrl Pts',(0.00744843051460957,-0.0392663127868883,
-0.0132861043936424));
#34358=CARTESIAN_POINT('Ctrl Pts',(0.00585994412188996,-0.039187242654919,
-0.0139954666585319));
#34359=CARTESIAN_POINT('Ctrl Pts',(0.00439872482316802,-0.0391081725229496,
-0.0130513681512097));
#34360=CARTESIAN_POINT('Ctrl Pts',(0.00439256500441095,-0.0390291023909803,
-0.0113116998236284));
#34361=CARTESIAN_POINT('Ctrl Pts',(0.00584706202148047,-0.038950032259011,
-0.0103572773471858));
#34362=CARTESIAN_POINT('Ctrl Pts',(0.00744053193820359,-0.0388709621270416,
-0.0110553729408225));
#34363=CARTESIAN_POINT('Ctrl Pts',(0.00772500782062244,-0.0387918919950723,
-0.0127716355380983));
#34364=CARTESIAN_POINT('Ctrl Pts',(0.00644198985553047,-0.038712821863103,
-0.0139465179764535));
#34365=CARTESIAN_POINT('Ctrl Pts',(0.00475734103106529,-0.0386337517311336,
-0.0135124187159094));
#34366=CARTESIAN_POINT('Ctrl Pts',(0.0042018814504384,-0.0385546815991643,
-0.0118637985459005));
#34367=CARTESIAN_POINT('Ctrl Pts',(0.00528035056630226,-0.038475611467195,
-0.0104987387426518));
#34368=CARTESIAN_POINT('Ctrl Pts',(0.00701275643985817,-0.0383965413352256,
-0.0106576527811916));
#34369=CARTESIAN_POINT('Ctrl Pts',(0.00782488276747915,-0.0383174712032563,
-0.0121961372689691));
#34370=CARTESIAN_POINT('Ctrl Pts',(0.00697876000420641,-0.038238401071287,
-0.0137161900991274));
#34371=CARTESIAN_POINT('Ctrl Pts',(0.00524324996648776,-0.0381593309393176,
-0.0138365571064366));
#34372=CARTESIAN_POINT('Ctrl Pts',(0.00419538926001839,-0.0380802608073483,
-0.0124478631249988));
#34373=CARTESIAN_POINT('Ctrl Pts',(0.00478735723355475,-0.038001190675379,
-0.0108119959316474));
#34374=CARTESIAN_POINT('Ctrl Pts',(0.00648123788338614,-0.0379221205434096,
-0.010415451742799));
#34375=CARTESIAN_POINT('Ctrl Pts',(0.00773782582947614,-0.0378430504114403,
-0.0116185588683412));
#34376=CARTESIAN_POINT('Ctrl Pts',(0.00741526772545535,-0.037763980279471,
-0.0133280812949623));
#34377=CARTESIAN_POINT('Ctrl Pts',(0.00580668193552033,-0.0376849101475016,
-0.0139905712347495));
#34378=CARTESIAN_POINT('Ctrl Pts',(0.00437374421722668,-0.0376058400155324,
-0.0130040816018285));
#34379=CARTESIAN_POINT('Ctrl Pts',(0.00441860022880923,-0.037526769883563,
-0.0112649267393021));
#34380=CARTESIAN_POINT('Ctrl Pts',(0.00590038736429771,-0.0374476997515936,
-0.0103536452953387));
#34381=CARTESIAN_POINT('Ctrl Pts',(0.00747282394630516,-0.0373686296196243,
-0.0110979369846573));
#34382=CARTESIAN_POINT('Ctrl Pts',(0.0077066636756073,-0.037289559487655,
-0.0128221982327131));
#34383=CARTESIAN_POINT('Ctrl Pts',(0.00639018635888645,-0.0372104893556857,
-0.0139581933959644));
#34384=CARTESIAN_POINT('Ctrl Pts',(0.00471815602457857,-0.0371314192237164,
-0.0134764515497806));
#34385=CARTESIAN_POINT('Ctrl Pts',(0.00421289332688479,-0.0370523489583796,
-0.0118090814011229));
#34386=CARTESIAN_POINT('Ctrl Pts',(0.00495593097017897,-0.0369996354036992,
-0.0109258244266621));
#34387=CARTESIAN_POINT('Ctrl Pts',(0.00543223656159701,-0.0369732785596753,
-0.0107377757433937));
#34388=CARTESIAN_POINT('',(0.00445700003781045,-0.0405679514195094,-0.0121755116975483));
#34389=CARTESIAN_POINT('Ctrl Pts',(0.00445700003781045,-0.0405679514195094,
-0.0121755116975483));
#34390=CARTESIAN_POINT('Ctrl Pts',(0.00445700301761374,-0.0405672476957248,
-0.0121620515561686));
#34391=CARTESIAN_POINT('Ctrl Pts',(0.00445718212343988,-0.0405665385763963,
-0.0121485923059843));
#34392=CARTESIAN_POINT('Ctrl Pts',(0.00445802931760553,-0.0405648343653531,
-0.0121164975946681));
#34393=CARTESIAN_POINT('Ctrl Pts',(0.00445885916667054,-0.0405638345050433,
-0.0120978688272803));
#34394=CARTESIAN_POINT('Ctrl Pts',(0.00446660927761155,-0.0405571317217464,
-0.0119743096298569));
#34395=CARTESIAN_POINT('Ctrl Pts',(0.00448390293192045,-0.0405511225439535,
-0.0118703186347209));
#34396=CARTESIAN_POINT('Ctrl Pts',(0.00452569449924638,-0.0405420351721237,
-0.0117174689997002));
#34397=CARTESIAN_POINT('Ctrl Pts',(0.00454241680909747,-0.0405389832279566,
-0.0116667908739223));
#34398=CARTESIAN_POINT('Ctrl Pts',(0.00457283306441903,-0.0405342953142253,
-0.0115885002902892));
#34399=CARTESIAN_POINT('Ctrl Pts',(0.0045847859545511,-0.0405326102753515,
-0.0115602572874876));
#34400=CARTESIAN_POINT('Ctrl Pts',(0.00460233303742628,-0.0405303548848834,
-0.0115220135971565));
#34401=CARTESIAN_POINT('Ctrl Pts',(0.00460720800297794,-0.0405297489031321,
-0.0115116923528811));
#34402=CARTESIAN_POINT('Ctrl Pts',(0.00461571486029345,-0.0405287269962117,
-0.0114941873700126));
#34403=CARTESIAN_POINT('Ctrl Pts',(0.00461928918985885,-0.0405283077731754,
-0.0114869763462131));
#34404=CARTESIAN_POINT('Ctrl Pts',(0.0046270987701427,-0.0405274136454441,
-0.0114715259314694));
#34405=CARTESIAN_POINT('Ctrl Pts',(0.00463135201963233,-0.0405269398170757,
-0.0114632962542935));
#34406=CARTESIAN_POINT('Ctrl Pts',(0.00464364934464731,-0.040525605133667,
-0.0114400183630903));
#34407=CARTESIAN_POINT('Ctrl Pts',(0.00465186946591345,-0.0405247543672459,
-0.0114250642069838));
#34408=CARTESIAN_POINT('Ctrl Pts',(0.00469296533736947,-0.0405206812399618,
-0.0113531541550091));
#34409=CARTESIAN_POINT('Ctrl Pts',(0.00472921379575197,-0.0405176221086522,
-0.0112981988720777));
#34410=CARTESIAN_POINT('Ctrl Pts',(0.00481868615956656,-0.0405107910158406,
-0.0111797717459593));
#34411=CARTESIAN_POINT('Ctrl Pts',(0.00487372973224963,-0.0405070438407399,
-0.0111179327794487));
#34412=CARTESIAN_POINT('Ctrl Pts',(0.0049682166488859,-0.0405008789541652,
-0.011027556517288));
#34413=CARTESIAN_POINT('Ctrl Pts',(0.0050045073728012,-0.0404985657521315,
-0.0109959565641567));
#34414=CARTESIAN_POINT('Ctrl Pts',(0.00505724066377667,-0.0404952359539612,
-0.010954206350628));
#34415=CARTESIAN_POINT('Ctrl Pts',(0.00507248857654536,-0.04049427673922,
-0.0109425897621374));
#34416=CARTESIAN_POINT('Ctrl Pts',(0.00509940407724372,-0.0404925875743147,
-0.0109228657824191));
#34417=CARTESIAN_POINT('Ctrl Pts',(0.00511097472269373,-0.0404918626853937,
-0.0109146297772545));
#34418=CARTESIAN_POINT('Ctrl Pts',(0.00513527106277933,-0.0404903423847992,
-0.0108978360752631));
#34419=CARTESIAN_POINT('Ctrl Pts',(0.00514801390652434,-0.0404895460433777,
-0.0108893060463693));
#34420=CARTESIAN_POINT('Ctrl Pts',(0.00518205914660631,-0.0404874203061145,
-0.0108672438743938));
#34421=CARTESIAN_POINT('Ctrl Pts',(0.00520356940942222,-0.0404860790587345,
-0.0108540423893678));
#34422=CARTESIAN_POINT('Ctrl Pts',(0.00533579934686101,-0.0404778423415594,
-0.0107772886264239));
#34423=CARTESIAN_POINT('Ctrl Pts',(0.00545371997776377,-0.040470473157869,
-0.0107271592989575));
#34424=CARTESIAN_POINT('Ctrl Pts',(0.00563634119169197,-0.0404596098027992,
-0.0106750261729495));
#34425=CARTESIAN_POINT('Ctrl Pts',(0.00569722955898793,-0.0404560839389985,
-0.0106615676297317));
#34426=CARTESIAN_POINT('Ctrl Pts',(0.005772470192972,-0.0404519653661404,
-0.0106496581444446));
#34427=CARTESIAN_POINT('Ctrl Pts',(0.00578620044358163,-0.0404512234567575,
-0.0106476742392438));
#34428=CARTESIAN_POINT('Ctrl Pts',(0.00580837411008537,-0.0404500428994715,
-0.010644775041075));
#34429=CARTESIAN_POINT('Ctrl Pts',(0.00581680132489728,-0.040449598302531,
-0.0106437438493416));
#34430=CARTESIAN_POINT('Ctrl Pts',(0.00583360070876016,-0.0404487207200846,
-0.0106418287953362));
#34431=CARTESIAN_POINT('Ctrl Pts',(0.00584197242801135,-0.0404482876957185,
-0.0106409437922207));
#34432=CARTESIAN_POINT('Ctrl Pts',(0.00586383724602124,-0.0404471670186347,
-0.0106388131743079));
#34433=CARTESIAN_POINT('Ctrl Pts',(0.00587734051983284,-0.0404464851002116,
-0.010637676678446));
#34434=CARTESIAN_POINT('Ctrl Pts',(0.00594227547400257,-0.0404432474614542,
-0.0106330720357617));
#34435=CARTESIAN_POINT('Ctrl Pts',(0.00599384813652307,-0.0404408006717884,
-0.0106320044958175));
#34436=CARTESIAN_POINT('Ctrl Pts',(0.00614361500215606,-0.0404338229875484,
-0.0106364111776378));
#34437=CARTESIAN_POINT('Ctrl Pts',(0.00624134770538443,-0.0404294158626033,
-0.0106486796896947));
#34438=CARTESIAN_POINT('Ctrl Pts',(0.00638823661725556,-0.0404223508074989,
-0.0106815804683772));
#34439=CARTESIAN_POINT('Ctrl Pts',(0.0064386054520579,-0.0404198483817655,
-0.0106955818395151));
#34440=CARTESIAN_POINT('Ctrl Pts',(0.00650681854332323,-0.0404162939743058,
-0.0107183311998621));
#34441=CARTESIAN_POINT('Ctrl Pts',(0.00652535120527398,-0.0404153111816445,
-0.0107249081682775));
#34442=CARTESIAN_POINT('Ctrl Pts',(0.00655710121066071,-0.0404135954396204,
-0.0107368638176332));
#34443=CARTESIAN_POINT('Ctrl Pts',(0.00657037915965547,-0.0404128680815828,
-0.0107420750446032));
#34444=CARTESIAN_POINT('Ctrl Pts',(0.00659758083910213,-0.0404113568610635,
-0.0107531886044942));
#34445=CARTESIAN_POINT('Ctrl Pts',(0.00661149382758474,-0.0404105723150985,
-0.0107591130372277));
#34446=CARTESIAN_POINT('Ctrl Pts',(0.00664747666319189,-0.0404085121191546,
-0.0107750640417832));
#34447=CARTESIAN_POINT('Ctrl Pts',(0.00666940069386643,-0.0404072258642573,
-0.0107854076169645));
#34448=CARTESIAN_POINT('Ctrl Pts',(0.00679577104057577,-0.0403996267428555,
-0.0108487096745987));
#34449=CARTESIAN_POINT('Ctrl Pts',(0.00689414695991099,-0.0403929195475568,
-0.0109128982910897));
#34450=CARTESIAN_POINT('Ctrl Pts',(0.00702318350109659,-0.0403833073684436,
-0.0110197851465529));
#34451=CARTESIAN_POINT('Ctrl Pts',(0.00706046201418208,-0.0403804216564015,
-0.0110538823623851));
#34452=CARTESIAN_POINT('Ctrl Pts',(0.00711687587008837,-0.04037595238858,
-0.0111108102703621));
#34453=CARTESIAN_POINT('Ctrl Pts',(0.00713713856100051,-0.0403743240875982,
-0.0111324720352807));
#34454=CARTESIAN_POINT('Ctrl Pts',(0.00716421219055398,-0.0403721320234571,
-0.0111631412882262));
#34455=CARTESIAN_POINT('Ctrl Pts',(0.00717156666670154,-0.0403715347956552,
-0.0111716584965681));
#34456=CARTESIAN_POINT('Ctrl Pts',(0.00718399166949294,-0.0403705239276032,
-0.0111863701978207));
#34457=CARTESIAN_POINT('Ctrl Pts',(0.00718910825526529,-0.0403701071261388,
-0.0111925249469508));
#34458=CARTESIAN_POINT('Ctrl Pts',(0.00720006800680869,-0.0403692134634119,
-0.0112059191055391));
#34459=CARTESIAN_POINT('Ctrl Pts',(0.00720589390455731,-0.0403687377556948,
-0.011213171908399));
#34460=CARTESIAN_POINT('Ctrl Pts',(0.00722235105476872,-0.0403673906434058,
-0.0112340436578774));
#34461=CARTESIAN_POINT('Ctrl Pts',(0.00723281992394978,-0.0403665296495844,
-0.011247789410233));
#34462=CARTESIAN_POINT('Ctrl Pts',(0.0072842819686224,-0.0403622606215341,
-0.0113177676206833));
#34463=CARTESIAN_POINT('Ctrl Pts',(0.00732167195999868,-0.0403590357549089,
-0.0113765560972033));
#34464=CARTESIAN_POINT('Ctrl Pts',(0.00738531630127132,-0.0403529227231774,
-0.0114933783939187));
#34465=CARTESIAN_POINT('Ctrl Pts',(0.00741220053659239,-0.0403500354241956,
-0.0115509030932052));
#34466=CARTESIAN_POINT('Ctrl Pts',(0.00745748577726506,-0.0403442809440113,
-0.0116657668982553));
#34467=CARTESIAN_POINT('Ctrl Pts',(0.00747622470702912,-0.0403414259387455,
-0.0117228492555738));
#34468=CARTESIAN_POINT('Ctrl Pts',(0.0074968372540085,-0.0403374541892639,
-0.0118006900942998));
#34469=CARTESIAN_POINT('Ctrl Pts',(0.00750168891075866,-0.0403364315077939,
-0.0118206075240896));
#34470=CARTESIAN_POINT('Ctrl Pts',(0.00750927442345102,-0.0403346681066388,
-0.0118546873591697));
#34471=CARTESIAN_POINT('Ctrl Pts',(0.00751220918272555,-0.0403339338421727,
-0.0118688024639827));
#34472=CARTESIAN_POINT('Ctrl Pts',(0.007517439300735,-0.0403325184288825,
-0.0118958541084151));
#34473=CARTESIAN_POINT('Ctrl Pts',(0.00751976807005864,-0.0403318384098902,
-0.0119087829395005));
#34474=CARTESIAN_POINT('Ctrl Pts',(0.00752546818548569,-0.0403300329188543,
-0.0119429219400548));
#34475=CARTESIAN_POINT('Ctrl Pts',(0.00752856220884581,-0.04032889888979,
-0.011964174971697));
#34476=CARTESIAN_POINT('Ctrl Pts',(0.00753907045443044,-0.040324347603729,
-0.012048697164316));
#34477=CARTESIAN_POINT('Ctrl Pts',(0.00754300673222017,-0.0403208263147395,
-0.0121123289554273));
#34478=CARTESIAN_POINT('Ctrl Pts',(0.00754299363468279,-0.0403138357438406,
-0.0122360752528632));
#34479=CARTESIAN_POINT('Ctrl Pts',(0.00753948075027893,-0.040310381362184,
-0.0122960806343023));
#34480=CARTESIAN_POINT('Ctrl Pts',(0.00752464214422209,-0.0403030819248212,
-0.0124225025366504));
#34481=CARTESIAN_POINT('Ctrl Pts',(0.00751244756973687,-0.040299246965904,
-0.012488700055835));
#34482=CARTESIAN_POINT('Ctrl Pts',(0.007491777459145,-0.0402946442035614,
-0.0125704951364037));
#34483=CARTESIAN_POINT('Ctrl Pts',(0.00748730619594309,-0.0402937213372485,
-0.0125870253956281));
#34484=CARTESIAN_POINT('Ctrl Pts',(0.00747999081126814,-0.0402923203577272,
-0.0126123875631331));
#34485=CARTESIAN_POINT('Ctrl Pts',(0.00747734077131737,-0.0402918323652687,
-0.0126212735712009));
#34486=CARTESIAN_POINT('Ctrl Pts',(0.00747224957979907,-0.0402909308680515,
-0.0126377997031975));
#34487=CARTESIAN_POINT('Ctrl Pts',(0.00746982875414881,-0.040290516320024,
-0.012645445398858));
#34488=CARTESIAN_POINT('Ctrl Pts',(0.00746384371102012,-0.0402895241320731,
-0.0126638481598918));
#34489=CARTESIAN_POINT('Ctrl Pts',(0.0074602203541576,-0.0402889498051573,
-0.0126745856179936));
#34490=CARTESIAN_POINT('Ctrl Pts',(0.00744650860343296,-0.0402868665418217,
-0.0127137880749279));
#34491=CARTESIAN_POINT('Ctrl Pts',(0.00743570298600019,-0.040285393932746,
-0.0127419964834778));
#34492=CARTESIAN_POINT('Ctrl Pts',(0.00740405424159433,-0.0402814606177515,
-0.0128178699894255));
#34493=CARTESIAN_POINT('Ctrl Pts',(0.00738161775109788,-0.040279056021971,
-0.01286482836826));
#34494=CARTESIAN_POINT('Ctrl Pts',(0.00730257127607069,-0.0402714295646993,
-0.0130108097373296));
#34495=CARTESIAN_POINT('Ctrl Pts',(0.00723735442326272,-0.0402662609593681,
-0.0131047217027002));
#34496=CARTESIAN_POINT('Ctrl Pts',(0.00714619465120043,-0.0402594895565454,
-0.0132091457545853));
#34497=CARTESIAN_POINT('Ctrl Pts',(0.00712955750886972,-0.0402582704283589,
-0.0132273071629746));
#34498=CARTESIAN_POINT('Ctrl Pts',(0.00710195540869737,-0.0402562692446052,
-0.0132560266751178));
#34499=CARTESIAN_POINT('Ctrl Pts',(0.00709125614038842,-0.0402554984815776,
-0.0132668346278284));
#34500=CARTESIAN_POINT('Ctrl Pts',(0.00707023003018678,-0.0402539922359212,
-0.0132874555334687));
#34501=CARTESIAN_POINT('Ctrl Pts',(0.00705992358778738,-0.0402532576882166,
-0.0132972871200758));
#34502=CARTESIAN_POINT('Ctrl Pts',(0.00703520729260259,-0.0402515042566375,
-0.0133202195228351));
#34503=CARTESIAN_POINT('Ctrl Pts',(0.00702068285259519,-0.0402504801701176,
-0.0133331927741724));
#34504=CARTESIAN_POINT('Ctrl Pts',(0.00696757253860754,-0.0402467563739465,
-0.0133788534799981));
#34505=CARTESIAN_POINT('Ctrl Pts',(0.00692763372871506,-0.0402439932862024,
-0.0134099120365688));
#34506=CARTESIAN_POINT('Ctrl Pts',(0.0068114018217784,-0.0402360697866959,
-0.0134914654130546));
#34507=CARTESIAN_POINT('Ctrl Pts',(0.00673204235351503,-0.0402307818460033,
-0.0135372202990062));
#34508=CARTESIAN_POINT('Ctrl Pts',(0.00659482577633572,-0.0402221378613781,
-0.0136008485070819));
#34509=CARTESIAN_POINT('Ctrl Pts',(0.0065391212700711,-0.0402187567995619,
-0.013622842736316));
#34510=CARTESIAN_POINT('Ctrl Pts',(0.00646903628206338,-0.040214767076841,
-0.0136459037082862));
#34511=CARTESIAN_POINT('Ctrl Pts',(0.00645573742270655,-0.0402140215003565,
-0.0136500807806306));
#34512=CARTESIAN_POINT('Ctrl Pts',(0.00643423630405216,-0.0402128365602255,
-0.0136565153516891));
#34513=CARTESIAN_POINT('Ctrl Pts',(0.00642606905079611,-0.0402123911736499,
-0.0136588861552256));
#34514=CARTESIAN_POINT('Ctrl Pts',(0.00640978564714478,-0.0402115131379154,
-0.0136634673057992));
#34515=CARTESIAN_POINT('Ctrl Pts',(0.00640167022233017,-0.0402110804315408,
-0.0136656790430655));
#34516=CARTESIAN_POINT('Ctrl Pts',(0.0063804829877849,-0.0402099625236005,
-0.0136712675964416));
#34517=CARTESIAN_POINT('Ctrl Pts',(0.00636738396481212,-0.0402092829928113,
-0.0136745394805046));
#34518=CARTESIAN_POINT('Ctrl Pts',(0.00630120246256232,-0.0402059004767904,
-0.0136901504627736));
#34519=CARTESIAN_POINT('Ctrl Pts',(0.00624753154893221,-0.040203320313985,
-0.0136998440837757));
#34520=CARTESIAN_POINT('Ctrl Pts',(0.00607883964329059,-0.0401954181763324,
-0.0137211623565376));
#34521=CARTESIAN_POINT('Ctrl Pts',(0.00596296217540964,-0.0401902583719616,
-0.0137227290113307));
#34522=CARTESIAN_POINT('Ctrl Pts',(0.0058105679022793,-0.0401829425867689,
-0.0137076427269774));
#34523=CARTESIAN_POINT('Ctrl Pts',(0.00577329221115343,-0.0401811136345478,
-0.0137025709165474));
#34524=CARTESIAN_POINT('Ctrl Pts',(0.00571887632306444,-0.0401783665276171,
-0.0136931301472994));
#34525=CARTESIAN_POINT('Ctrl Pts',(0.00570156540977394,-0.0401774810805772,
-0.0136898203790236));
#34526=CARTESIAN_POINT('Ctrl Pts',(0.00567059380385307,-0.04017587450769,
-0.0136833469236624));
#34527=CARTESIAN_POINT('Ctrl Pts',(0.00565691222451923,-0.040175156898776,
-0.0136802921418639));
#34528=CARTESIAN_POINT('Ctrl Pts',(0.00562757210221092,-0.0401736002078394,
-0.0136733201300485));
#34529=CARTESIAN_POINT('Ctrl Pts',(0.00561192968306698,-0.0401727592769231,
-0.013669342787428));
#34530=CARTESIAN_POINT('Ctrl Pts',(0.00556803411134551,-0.0401703674623307,
-0.0136574454497776));
#34531=CARTESIAN_POINT('Ctrl Pts',(0.00553994140173687,-0.0401687989056851,
-0.0136489642117284));
#34532=CARTESIAN_POINT('Ctrl Pts',(0.00544037245825868,-0.0401631021784236,
-0.0136157782047824));
#34533=CARTESIAN_POINT('Ctrl Pts',(0.00537049787839429,-0.0401588405396027,
-0.0135866302939539));
#34534=CARTESIAN_POINT('Ctrl Pts',(0.00521523389267398,-0.0401488866767666,
-0.0135080240204686));
#34535=CARTESIAN_POINT('Ctrl Pts',(0.00513187306148297,-0.0401431681972347,
-0.0134552647863316));
#34536=CARTESIAN_POINT('Ctrl Pts',(0.00503938843387431,-0.0401367626469985,
-0.0133835044565315));
#34537=CARTESIAN_POINT('Ctrl Pts',(0.00502487997886895,-0.0401357563713039,
-0.0133718202311756));
#34538=CARTESIAN_POINT('Ctrl Pts',(0.00500332313841348,-0.0401342636271399,
-0.0133538065192534));
#34539=CARTESIAN_POINT('Ctrl Pts',(0.00499611603124252,-0.0401337649755924,
-0.0133476704954765));
#34540=CARTESIAN_POINT('Ctrl Pts',(0.00498354693693273,-0.0401328967934447,
-0.0133367682809583));
#34541=CARTESIAN_POINT('Ctrl Pts',(0.00497816125846767,-0.0401325253300547,
-0.0133320306267527));
#34542=CARTESIAN_POINT('Ctrl Pts',(0.00496500621493986,-0.0401316190870195,
-0.0133202947181631));
#34543=CARTESIAN_POINT('Ctrl Pts',(0.00495727467599045,-0.0401310873409846,
-0.0133132548144854));
#34544=CARTESIAN_POINT('Ctrl Pts',(0.00493187871816833,-0.0401293413109231,
-0.0132896540688937));
#34545=CARTESIAN_POINT('Ctrl Pts',(0.00491453188351238,-0.0401281496542151,
-0.0132727554418182));
#34546=CARTESIAN_POINT('Ctrl Pts',(0.00487176531018632,-0.0401251926184072,
-0.0132290853135259));
#34547=CARTESIAN_POINT('Ctrl Pts',(0.00484689467674212,-0.0401234547917817,
-0.0132017965503136));
#34548=CARTESIAN_POINT('Ctrl Pts',(0.00474878601273222,-0.0401164029261517,
-0.0130860691439521));
#34549=CARTESIAN_POINT('Ctrl Pts',(0.00468455339088075,-0.0401112747257682,
-0.0129904882228372));
#34550=CARTESIAN_POINT('Ctrl Pts',(0.00461386333023939,-0.0401039707727769,
-0.0128547747284036));
#34551=CARTESIAN_POINT('Ctrl Pts',(0.00459747652041293,-0.0401021137308062,
-0.0128202419913573));
#34552=CARTESIAN_POINT('Ctrl Pts',(0.004575390220447,-0.0400993324930915,
-0.0127688542346881));
#34553=CARTESIAN_POINT('Ctrl Pts',(0.00456867273681648,-0.0400984422383127,
-0.012752451397434));
#34554=CARTESIAN_POINT('Ctrl Pts',(0.00455714755953665,-0.0400968304100547,
-0.0127228657341133));
#34555=CARTESIAN_POINT('Ctrl Pts',(0.00455223425630502,-0.0400961124515623,
-0.0127097260402703));
#34556=CARTESIAN_POINT('Ctrl Pts',(0.0045420764996996,-0.040094558898561,
-0.0126813891200141));
#34557=CARTESIAN_POINT('Ctrl Pts',(0.00453688905817036,-0.0400937215260027,
-0.0126661733427898));
#34558=CARTESIAN_POINT('Ctrl Pts',(0.00452301252276451,-0.0400913516626143,
-0.0126232881858243));
#34559=CARTESIAN_POINT('Ctrl Pts',(0.00451486468955921,-0.0400898020214516,
-0.0125954518525099));
#34560=CARTESIAN_POINT('Ctrl Pts',(0.00448662158125346,-0.040083764457735,
-0.0124877960722624));
#34561=CARTESIAN_POINT('Ctrl Pts',(0.00447214163801477,-0.0400791119384198,
-0.0124066534941163));
#34562=CARTESIAN_POINT('Ctrl Pts',(0.00445940319010193,-0.0400715496481565,
-0.0122752641998871));
#34563=CARTESIAN_POINT('Ctrl Pts',(0.00445699999999992,-0.04006868578093,
-0.0122255734026042));
#34564=CARTESIAN_POINT('Ctrl Pts',(0.004457,-0.0400658559061629,-0.0121758532865556));
#34565=CARTESIAN_POINT('Ctrl Pts',(0.004457,-0.0405679692773165,-0.012175853286558));
#34566=CARTESIAN_POINT('Ctrl Pts',(0.004457,-0.0405679633251033,-0.0121757394235622));
#34567=CARTESIAN_POINT('Ctrl Pts',(0.00445700001260348,-0.040567957372501,
-0.0121756255605583));
#34568=CARTESIAN_POINT('Ctrl Pts',(0.00445700003781045,-0.0405679514195094,
-0.0121755116975483));
#34569=CARTESIAN_POINT('Ctrl Pts',(0.00517003826372136,-0.0368388088258703,
-0.0112226527283813));
#34570=CARTESIAN_POINT('Ctrl Pts',(0.00496318803061621,-0.0368566041514186,
-0.0114031443924197));
#34571=CARTESIAN_POINT('Ctrl Pts',(0.00481517121886622,-0.0368716613977715,
-0.0116537046307317));
#34572=CARTESIAN_POINT('Ctrl Pts',(0.00476045244943773,-0.0368890231487594,
-0.0119228284334495));
#34573=CARTESIAN_POINT('Ctrl Pts',(0.00475804259485334,-0.0368897877729577,
-0.011934680842349));
#34574=CARTESIAN_POINT('Ctrl Pts',(0.00475581169755592,-0.0368905568669409,
-0.0119465719172147));
#34575=CARTESIAN_POINT('Ctrl Pts',(0.00475375746819469,-0.0368913308614504,
-0.0119584969221675));
#34576=CARTESIAN_POINT('Ctrl Pts',(0.00472994900992145,-0.0369003014351997,
-0.0120967073811281));
#34577=CARTESIAN_POINT('Ctrl Pts',(0.00472969925662481,-0.0369100660923477,
-0.0122383423209631));
#34578=CARTESIAN_POINT('Ctrl Pts',(0.00475183331331961,-0.0369192107959462,
-0.0123755348980974));
#34579=CARTESIAN_POINT('Ctrl Pts',(0.00479405294068054,-0.0369366538694675,
-0.0126372230090101));
#34580=CARTESIAN_POINT('Ctrl Pts',(0.00492069786421945,-0.0369513027772182,
-0.0128890197323158));
#34581=CARTESIAN_POINT('Ctrl Pts',(0.00511161730525771,-0.036968058701728,
-0.0130769904122617));
#34582=CARTESIAN_POINT('Ctrl Pts',(0.00512542591996926,-0.0369692706061021,
-0.0130905857521723));
#34583=CARTESIAN_POINT('Ctrl Pts',(0.00513957437411001,-0.0369704935326665,
-0.013103852713356));
#34584=CARTESIAN_POINT('Ctrl Pts',(0.0051540427324716,-0.0369717293358099,
-0.0131167880484792));
#34585=CARTESIAN_POINT('Ctrl Pts',(0.00525891627092471,-0.0369806870243903,
-0.0132105495058292));
#34586=CARTESIAN_POINT('Ctrl Pts',(0.00537951599478848,-0.0369904541203737,
-0.0132863860868721));
#34587=CARTESIAN_POINT('Ctrl Pts',(0.00550872901378148,-0.0369996339059789,
-0.0133406619611183));
#34588=CARTESIAN_POINT('Origin',(0.006,-0.0418165664398416,-0.0121758532865581));
#34589=CARTESIAN_POINT('Origin',(0.0078,-0.0299787743898723,-0.00817585328655812));
#34590=CARTESIAN_POINT('Origin',(-0.0125,-0.0298787743898723,-0.0121758532865581));
#34591=CARTESIAN_POINT('',(-0.0137645000000023,-0.03021427438987,-0.0121758532865581));
#34592=CARTESIAN_POINT('Origin',(-0.01249999999999,-0.0302142743898623,
-0.0121758532865681));
#34593=CARTESIAN_POINT('',(-0.0141,-0.0298787743898723,-0.0121758532865581));
#34594=CARTESIAN_POINT('Origin',(-0.01249999999999,-0.0302142743898623,
-0.0121758532865681));
#34595=CARTESIAN_POINT('Origin',(-0.0148,-0.0299787743898723,-0.0161758532865581));
#34596=CARTESIAN_POINT('Origin',(-0.0125,-0.0302142743898723,-0.0121758532865581));
#34597=CARTESIAN_POINT('Origin',(0.006,-0.0418165664398416,-0.0121758532865581));
#34598=CARTESIAN_POINT('',(0.00753652184170541,-0.0364251782306474,-0.0123170964455508));
#34599=CARTESIAN_POINT('Origin',(0.00600000000001,-0.036425178177226,-0.0121758532865681));
#34600=CARTESIAN_POINT('Ctrl Pts',(0.00753652184170541,-0.0364251782306474,
-0.0123170964455508));
#34601=CARTESIAN_POINT('Ctrl Pts',(0.00756822434111586,-0.0364430425111789,
-0.0119722189794262));
#34602=CARTESIAN_POINT('Ctrl Pts',(0.00747951616489019,-0.0364609067917104,
-0.0116174390738647));
#34603=CARTESIAN_POINT('Ctrl Pts',(0.00728922782690805,-0.0364787710722419,
-0.0113280675764132));
#34604=CARTESIAN_POINT('Ctrl Pts',(0.0072673963600219,-0.0364808206116566,
-0.0112948684622089));
#34605=CARTESIAN_POINT('Ctrl Pts',(0.00724428189505873,-0.0364828701510714,
-0.0112625130653046));
#34606=CARTESIAN_POINT('Ctrl Pts',(0.00721995334505698,-0.0364849196904862,
-0.0112310978494823));
#34607=CARTESIAN_POINT('Origin',(0.006,-0.036425178177236,-0.0121758532865581));
#34608=CARTESIAN_POINT('Origin',(0.0064207661241384,-0.0364251781806992,
-0.0121386924149705));
#34609=CARTESIAN_POINT('Ctrl Pts',(0.0072199533450484,-0.0364849196904962,
-0.0112310978494712));
#34610=CARTESIAN_POINT('Ctrl Pts',(0.0074098002074744,-0.0364689287443744,
-0.0114762452238835));
#34611=CARTESIAN_POINT('Ctrl Pts',(0.0076367749937228,-0.0364369468521306,
-0.0120839293008583));
#34612=CARTESIAN_POINT('Ctrl Pts',(0.0074792699890148,-0.0364049649598869,
-0.0127132063976075));
#34613=CARTESIAN_POINT('Ctrl Pts',(0.0073180661489925,-0.036388974013765,
-0.0129780693589976));
#34614=CARTESIAN_POINT('Ctrl Pts',(0.00714655018737591,-0.0365385211752087,
-0.0112879426727523));
#34615=CARTESIAN_POINT('Ctrl Pts',(0.00732497418741711,-0.0365225302290869,
-0.0115183398180267));
#34616=CARTESIAN_POINT('Ctrl Pts',(0.00753829216778011,-0.0364905483368431,
-0.0120894602589426));
#34617=CARTESIAN_POINT('Ctrl Pts',(0.00739026405392343,-0.0364585664445993,
-0.012680874493034));
#34618=CARTESIAN_POINT('Ctrl Pts',(0.00723875965932221,-0.0364425754984775,
-0.0129298009616103));
#34619=CARTESIAN_POINT('Ctrl Pts',(0.0070731470297034,-0.0365921226599213,
-0.0113447874960334));
#34620=CARTESIAN_POINT('Ctrl Pts',(0.00724014816735991,-0.0365761317137994,
-0.0115604344121699));
#34621=CARTESIAN_POINT('Ctrl Pts',(0.00743980934183733,-0.0365441498215557,
-0.0120949912170268));
#34622=CARTESIAN_POINT('Ctrl Pts',(0.00730125811883206,-0.036512167929312,
-0.0126485425884606));
#34623=CARTESIAN_POINT('Ctrl Pts',(0.00715945316965194,-0.0364961769831901,
-0.0128815325642231));
#34624=CARTESIAN_POINT('Ctrl Pts',(0.0069997438720308,-0.0366457241446337,
-0.0114016323193146));
#34625=CARTESIAN_POINT('Ctrl Pts',(0.00715532214730263,-0.0366297331985119,
-0.0116025290063132));
#34626=CARTESIAN_POINT('Ctrl Pts',(0.00734132651589453,-0.0365977513062682,
-0.0121005221751111));
#34627=CARTESIAN_POINT('Ctrl Pts',(0.0072122521837407,-0.0365657694140244,
-0.0126162106838871));
#34628=CARTESIAN_POINT('Ctrl Pts',(0.00708014667998167,-0.0365497784679025,
-0.0128332641668358));
#34629=CARTESIAN_POINT('Ctrl Pts',(0.00708453011998519,-0.0366362514743427,
-0.0115256574169581));
#34630=CARTESIAN_POINT('Ctrl Pts',(0.00723825165049006,-0.0366174374253146,
-0.0117820657359241));
#34631=CARTESIAN_POINT('Ctrl Pts',(0.00729678566547772,-0.0365986233762864,
-0.0120941053643385));
#34632=CARTESIAN_POINT('Ctrl Pts',(0.00724644164534432,-0.0365798093272583,
-0.0123887933597039));
#34633=CARTESIAN_POINT('Ctrl Pts',(0.00722898096775414,-0.0365732841025469,
-0.0124909991840131));
#34634=CARTESIAN_POINT('Ctrl Pts',(0.00719888732060191,-0.0365667588778354,
-0.0125910404109786));
#34635=CARTESIAN_POINT('Ctrl Pts',(0.00715706304473573,-0.036560233653124,
-0.0126859173614613));
#34636=CARTESIAN_POINT('Origin',(0.006,-0.0412787743898723,-0.0121758532865581));
#34637=CARTESIAN_POINT('Ctrl Pts',(0.0071049221523962,-0.036616763538703,
-0.0127891486670682));
#34638=CARTESIAN_POINT('Ctrl Pts',(0.00722758846935883,-0.0366330987428971,
-0.0125677025948817));
#34639=CARTESIAN_POINT('Ctrl Pts',(0.00728449242226235,-0.0366477660520011,
-0.01230803163059));
#34640=CARTESIAN_POINT('Ctrl Pts',(0.00726021773649979,-0.0366635671619898,
-0.0120563276956654));
#34641=CARTESIAN_POINT('Ctrl Pts',(0.00725576839945219,-0.0366664633668987,
-0.0120101925714606));
#34642=CARTESIAN_POINT('Ctrl Pts',(0.00724860265255448,-0.0366693976626142,
-0.0119643005706726));
#34643=CARTESIAN_POINT('Ctrl Pts',(0.00723890064348258,-0.0366723873013995,
-0.0119188749448376));
#34644=CARTESIAN_POINT('Ctrl Pts',(0.00719971714612425,-0.0366844615535031,
-0.011735414501056));
#34645=CARTESIAN_POINT('Ctrl Pts',(0.00711972216632024,-0.0366973265713535,
-0.0115610957458025));
#34646=CARTESIAN_POINT('Ctrl Pts',(0.00700648721588952,-0.0367089394431721,
-0.0114117479980388));
#34647=CARTESIAN_POINT('Ctrl Pts',(0.00658722785536586,-0.036742294363837,
-0.0110560653534979));
#34648=CARTESIAN_POINT('Ctrl Pts',(0.00695797246101722,-0.0367159475964203,
-0.0112504847865641));
#34649=CARTESIAN_POINT('Ctrl Pts',(0.00748293891467684,-0.0366632540613929,
-0.0120352036662368));
#34650=CARTESIAN_POINT('Ctrl Pts',(0.00711485957225081,-0.0366105605263656,
-0.012904623644283));
#34651=CARTESIAN_POINT('Ctrl Pts',(0.00678727634316453,-0.0365842137587548,
-0.0131652761125726));
#34652=CARTESIAN_POINT('Ctrl Pts',(0.00663053159797881,-0.0367961275404045,
-0.010973489215477));
#34653=CARTESIAN_POINT('Ctrl Pts',(0.00702861589610487,-0.0367697807729879,
-0.0111822456542074));
#34654=CARTESIAN_POINT('Ctrl Pts',(0.00759229477115595,-0.0367170872379605,
-0.0120248317894578));
#34655=CARTESIAN_POINT('Ctrl Pts',(0.00719707227984838,-0.0366643937029331,
-0.0129583651071692));
#34656=CARTESIAN_POINT('Ctrl Pts',(0.00684533219289669,-0.0366380469353223,
-0.0132382387811545));
#34657=CARTESIAN_POINT('Ctrl Pts',(0.00667383534059177,-0.0368499607169721,
-0.0108909130774562));
#34658=CARTESIAN_POINT('Ctrl Pts',(0.00709925933119253,-0.0368236139495555,
-0.0111140065218506));
#34659=CARTESIAN_POINT('Ctrl Pts',(0.00770165062763507,-0.0367709204145281,
-0.0120144599126789));
#34660=CARTESIAN_POINT('Ctrl Pts',(0.00727928498744596,-0.0367182268795007,
-0.0130121065700554));
#34661=CARTESIAN_POINT('Ctrl Pts',(0.00690338804262885,-0.0366918801118899,
-0.0133112014497364));
#34662=CARTESIAN_POINT('Ctrl Pts',(0.00671713908320482,-0.0369037938935395,
-0.0108083369394354));
#34663=CARTESIAN_POINT('Ctrl Pts',(0.00716990276628018,-0.0368774471261231,
-0.0110457673894939));
#34664=CARTESIAN_POINT('Ctrl Pts',(0.00781100648411419,-0.0368247535910955,
-0.0120040880358999));
#34665=CARTESIAN_POINT('Ctrl Pts',(0.00736149769504353,-0.0367720600560681,
-0.0130658480329415));
#34666=CARTESIAN_POINT('Ctrl Pts',(0.00696144389236101,-0.0367457132884574,
-0.0133841641183183));
#34667=CARTESIAN_POINT('Ctrl Pts',(0.00671669833492856,-0.0369031264224378,
-0.0108094007638883));
#34668=CARTESIAN_POINT('Ctrl Pts',(0.00701188501977547,-0.0368859357702769,
-0.0109642248810918));
#34669=CARTESIAN_POINT('Ctrl Pts',(0.0072554276123368,-0.036868745118116,
-0.0112188246564027));
#34670=CARTESIAN_POINT('Ctrl Pts',(0.00747237848207918,-0.0368424001339865,
-0.0116814132518847));
#34671=CARTESIAN_POINT('Ctrl Pts',(0.00751947603869318,-0.0368332458020179,
-0.0118548192245139));
#34672=CARTESIAN_POINT('Ctrl Pts',(0.00756733595801313,-0.0368069008178862,
-0.0123594301513162));
#34673=CARTESIAN_POINT('Ctrl Pts',(0.0074885971694383,-0.036789710165723,
-0.0127017865636874));
#34674=CARTESIAN_POINT('Ctrl Pts',(0.00721964017367036,-0.0367633651813997,
-0.0131376204535356));
#34675=CARTESIAN_POINT('Ctrl Pts',(0.00709970046774227,-0.0367542108492395,
-0.0132726735662828));
#34676=CARTESIAN_POINT('Ctrl Pts',(0.00696081100483646,-0.0367450565170793,
-0.0133832021230528));
#34677=CARTESIAN_POINT('Origin',(0.006,-0.0418165664398416,-0.0121758532865581));
#34678=CARTESIAN_POINT('Origin',(0.006,-0.0412787743898723,-0.0121758532865581));
#34679=CARTESIAN_POINT('Ctrl Pts',(0.0053235011610246,-0.0369233529358344,
-0.0132441741984872));
#34680=CARTESIAN_POINT('Ctrl Pts',(0.00523505662430941,-0.0369167648474377,
-0.0131881679687734));
#34681=CARTESIAN_POINT('Ctrl Pts',(0.00515392214402666,-0.0369097144759522,
-0.0131214057275732));
#34682=CARTESIAN_POINT('Ctrl Pts',(0.00500976886549827,-0.0368958757947603,
-0.0129692115297485));
#34683=CARTESIAN_POINT('Ctrl Pts',(0.00494735345119867,-0.0368891524433538,
-0.0128843145970702));
#34684=CARTESIAN_POINT('Ctrl Pts',(0.00481584137034549,-0.0368726379308069,
-0.0126489587493082));
#34685=CARTESIAN_POINT('Ctrl Pts',(0.00476439120123418,-0.0368635400229235,
-0.0124909884384143));
#34686=CARTESIAN_POINT('Ctrl Pts',(0.00472487521828434,-0.0368427862176367,
-0.0121641285889202));
#34687=CARTESIAN_POINT('Ctrl Pts',(0.00473723272218724,-0.0368312891618365,
-0.0119983443282033));
#34688=CARTESIAN_POINT('Ctrl Pts',(0.00480893333673192,-0.0368138833665868,
-0.0117384487674225));
#34689=CARTESIAN_POINT('Ctrl Pts',(0.00484930331121405,-0.0368074684757722,
-0.011641189466955));
#34690=CARTESIAN_POINT('Ctrl Pts',(0.00495301550513732,-0.0367949520902989,
-0.0114591025077254));
#34691=CARTESIAN_POINT('Ctrl Pts',(0.00501587895403898,-0.0367888825209941,
-0.0113749731264201));
#34692=CARTESIAN_POINT('Ctrl Pts',(0.00508837275135261,-0.0367823435972233,
-0.0112995565277352));
#34693=CARTESIAN_POINT('Ctrl Pts',(0.0051742753449155,-0.0367620604347684,
-0.0134803778190167));
#34694=CARTESIAN_POINT('Ctrl Pts',(0.00478645345963078,-0.0367384031130101,
-0.0132349052736592));
#34695=CARTESIAN_POINT('Ctrl Pts',(0.00424919073978731,-0.0366910919663293,
-0.0123774938115404));
#34696=CARTESIAN_POINT('Ctrl Pts',(0.00457748608479308,-0.0366437808196484,
-0.0114204297049166));
#34697=CARTESIAN_POINT('Ctrl Pts',(0.00489928336256372,-0.0366201269947257,
-0.0110932507042787));
#34698=CARTESIAN_POINT('Ctrl Pts',(0.0052243777953317,-0.0368161458631363,
-0.0134012232542332));
#34699=CARTESIAN_POINT('Ctrl Pts',(0.00486008775768916,-0.0367924885413782,
-0.0131706452332872));
#34700=CARTESIAN_POINT('Ctrl Pts',(0.00435542449895617,-0.0367451773946972,
-0.0123652588802681));
#34701=CARTESIAN_POINT('Ctrl Pts',(0.00466379988499779,-0.0366978662480164,
-0.0114662665008865));
#34702=CARTESIAN_POINT('Ctrl Pts',(0.00496607148667975,-0.0366742124230938,
-0.0111589397228459));
#34703=CARTESIAN_POINT('Ctrl Pts',(0.00527448024574789,-0.0368702312915042,
-0.0133220686894497));
#34704=CARTESIAN_POINT('Ctrl Pts',(0.00493372205574744,-0.036846573969746,
-0.0131063851929151));
#34705=CARTESIAN_POINT('Ctrl Pts',(0.00446165825812503,-0.0367992628230653,
-0.0123530239489957));
#34706=CARTESIAN_POINT('Ctrl Pts',(0.00475011368520242,-0.0367519516763844,
-0.0115121032968564));
#34707=CARTESIAN_POINT('Ctrl Pts',(0.00503285961079578,-0.0367282978514617,
-0.0112246287414129));
#34708=CARTESIAN_POINT('Ctrl Pts',(0.00532458269616408,-0.0369243167198722,
-0.0132429141246661));
#34709=CARTESIAN_POINT('Ctrl Pts',(0.00500735635380582,-0.036900659398114,
-0.0130421251525431));
#34710=CARTESIAN_POINT('Ctrl Pts',(0.0045678920172939,-0.0368533482514331,
-0.0123407890177234));
#34711=CARTESIAN_POINT('Ctrl Pts',(0.00483642748540704,-0.0368060371047523,
-0.0115579400928262));
#34712=CARTESIAN_POINT('Ctrl Pts',(0.00509964773491181,-0.0367823832798296,
-0.0112903177599799));
#34713=CARTESIAN_POINT('Ctrl Pts',(0.00489985734136315,-0.0366206471528947,
-0.0110939405679678));
#34714=CARTESIAN_POINT('Ctrl Pts',(0.00466420781315652,-0.0366379795411557,
-0.0113335607277211));
#34715=CARTESIAN_POINT('Ctrl Pts',(0.00450992989288636,-0.0366553119294167,
-0.0116531134538887));
#34716=CARTESIAN_POINT('Ctrl Pts',(0.00446868682950251,-0.0366726443176777,
-0.0119863038896692));
#34717=CARTESIAN_POINT('Ctrl Pts',(0.00445672246310587,-0.0366776723400085,
-0.0120829604453774));
#34718=CARTESIAN_POINT('Ctrl Pts',(0.004453955327891,-0.0366827003623392,
-0.0121806314281746));
#34719=CARTESIAN_POINT('Ctrl Pts',(0.00446035287725328,-0.03668772838467,
-0.012277518115372));
#34720=CARTESIAN_POINT('Ctrl Pts',(0.00448240549051054,-0.0367050601824617,
-0.0126114904728402));
#34721=CARTESIAN_POINT('Ctrl Pts',(0.00461749012905982,-0.0367223919802533,
-0.0129392208664159));
#34722=CARTESIAN_POINT('Ctrl Pts',(0.00483915438748629,-0.036739723778045,
-0.0131923602781266));
#34723=CARTESIAN_POINT('Ctrl Pts',(0.00490339558020791,-0.0367447467590616,
-0.0132657233807241));
#34724=CARTESIAN_POINT('Ctrl Pts',(0.00497459353102844,-0.0367497697400783,
-0.0133329516444489));
#34725=CARTESIAN_POINT('Ctrl Pts',(0.00505141064578676,-0.0367547927210949,
-0.013392827911221));
#34726=CARTESIAN_POINT('Origin',(0.006,-0.0418165664398416,-0.0121758532865581));
#34727=CARTESIAN_POINT('Ctrl Pts',(0.00490822568141441,-0.036629014744178,
-0.0132662100342682));
#34728=CARTESIAN_POINT('Ctrl Pts',(0.00466938135519506,-0.0366115831763784,
-0.0130270551869636));
#34729=CARTESIAN_POINT('Ctrl Pts',(0.00451241393214875,-0.0365941516085787,
-0.0127067464029452));
#34730=CARTESIAN_POINT('Ctrl Pts',(0.00446454380236732,-0.0365747000596988,
-0.012333183817743));
#34731=CARTESIAN_POINT('Ctrl Pts',(0.00446105042715403,-0.0365726800786186,
-0.0122942175049728));
#34732=CARTESIAN_POINT('Ctrl Pts',(0.00444170231516779,-0.0365532285297388,
-0.0119184373241344));
#34733=CARTESIAN_POINT('Ctrl Pts',(0.00453897781770981,-0.0365357969619391,
-0.0115753543699202));
#34734=CARTESIAN_POINT('Ctrl Pts',(0.00475379842566362,-0.0365163454130592,
-0.0112651579623936));
#34735=CARTESIAN_POINT('Ctrl Pts',(0.00477733077671506,-0.0365143254319789,
-0.0112338007169063));
#34736=CARTESIAN_POINT('Ctrl Pts',(0.00480201558775486,-0.0365123054508986,
-0.0112033912831782));
#34737=CARTESIAN_POINT('Ctrl Pts',(0.00509572370535752,-0.0364760372027012,
-0.013078987754096));
#34738=CARTESIAN_POINT('Ctrl Pts',(0.004874960106594,-0.0364565851795555,
-0.0128579454042039));
#34739=CARTESIAN_POINT('Ctrl Pts',(0.0046039989248781,-0.0364176811332647,
-0.012247730374574));
#34740=CARTESIAN_POINT('Ctrl Pts',(0.00481085609633788,-0.0363787770869738,
-0.0116129135072826));
#34741=CARTESIAN_POINT('Ctrl Pts',(0.00500775049564412,-0.0363593250638284,
-0.0113703668468132));
#34742=CARTESIAN_POINT('Ctrl Pts',(0.00503316372018776,-0.036527084977588,
-0.0131414687449504));
#34743=CARTESIAN_POINT('Ctrl Pts',(0.00479712717050601,-0.0365076329544425,
-0.0129051341594739));
#34744=CARTESIAN_POINT('Ctrl Pts',(0.0045074202496723,-0.0364687289081516,
-0.0122527030025053));
#34745=CARTESIAN_POINT('Ctrl Pts',(0.00472858829232875,-0.0364298248618607,
-0.0115739679942225));
#34746=CARTESIAN_POINT('Ctrl Pts',(0.00493910431455436,-0.0364103728387155,
-0.0113146413788082));
#34747=CARTESIAN_POINT('Ctrl Pts',(0.004970603735018,-0.0365781327524749,
-0.013203949735805));
#34748=CARTESIAN_POINT('Ctrl Pts',(0.00471929423441792,-0.0365586807293294,
-0.0129523229147439));
#34749=CARTESIAN_POINT('Ctrl Pts',(0.00441084157446649,-0.0365197766830385,
-0.0122576756304366));
#34750=CARTESIAN_POINT('Ctrl Pts',(0.00464632048831952,-0.0364808726367475,
-0.0115350224811624));
#34751=CARTESIAN_POINT('Ctrl Pts',(0.00487045813346461,-0.0364614206136023,
-0.0112589159108031));
#34752=CARTESIAN_POINT('Ctrl Pts',(0.00490804374984815,-0.0366291805273617,
-0.0132664307266594));
#34753=CARTESIAN_POINT('Ctrl Pts',(0.00464146129832983,-0.0366097285042163,
-0.0129995116700138));
#34754=CARTESIAN_POINT('Ctrl Pts',(0.0043142628992607,-0.0365708244579254,
-0.0122626482583679));
#34755=CARTESIAN_POINT('Ctrl Pts',(0.00456405268431038,-0.0365319204116345,
-0.0114960769681023));
#34756=CARTESIAN_POINT('Ctrl Pts',(0.00480181195237485,-0.0365124683884891,
-0.0112031904427979));
#34757=CARTESIAN_POINT('Ctrl Pts',(0.00473550000001001,-0.036425178177236,
-0.0117172854002574));
#34758=CARTESIAN_POINT('Ctrl Pts',(0.00470881837868537,-0.036425178177236,
-0.0118237756649726));
#34759=CARTESIAN_POINT('Ctrl Pts',(0.0046949074287484,-0.0364251781770394,
-0.0119335309693111));
#34760=CARTESIAN_POINT('Ctrl Pts',(0.00469488166357817,-0.0364251781770394,
-0.0121504784412239));
#34761=CARTESIAN_POINT('Ctrl Pts',(0.00470813137606538,-0.036425178177236,
-0.012256680250331));
#34762=CARTESIAN_POINT('Ctrl Pts',(0.00473547236319308,-0.036425178177236,
-0.0123610727438316));
#34763=CARTESIAN_POINT('Origin',(0.006,-0.036425178177236,-0.0121758532865581));
#34764=CARTESIAN_POINT('Origin',(1.7347234759768E-18,-0.0304787743898723,
-0.0121758532865581));
#50048=UNCERTAINTY_MEASURE_WITH_UNIT(LENGTH_MEASURE(1.E-5),#50082,
'DISTANCE_ACCURACY_VALUE',
'Maximum model space distance between geometric entities at asserted c
onnectivities');
#50059=UNCERTAINTY_MEASURE_WITH_UNIT(LENGTH_MEASURE(1.E-5),#50082,
'DISTANCE_ACCURACY_VALUE',
'Maximum model space distance between geometric entities at asserted c
onnectivities');
#50070=(
GEOMETRIC_REPRESENTATION_CONTEXT(3)
GLOBAL_UNCERTAINTY_ASSIGNED_CONTEXT((#50048))
GLOBAL_UNIT_ASSIGNED_CONTEXT((#50082,#50083,#50084))
REPRESENTATION_CONTEXT('','3D')
);
#50081=(
GEOMETRIC_REPRESENTATION_CONTEXT(3)
GLOBAL_UNCERTAINTY_ASSIGNED_CONTEXT((#50059))
GLOBAL_UNIT_ASSIGNED_CONTEXT((#50082,#50083,#50084))
REPRESENTATION_CONTEXT('','3D')
);
#50082=(
LENGTH_UNIT()
NAMED_UNIT(*)
SI_UNIT($,.METRE.)
);
#50083=(
NAMED_UNIT(*)
PLANE_ANGLE_UNIT()
SI_UNIT($,.RADIAN.)
);
#50084=(
NAMED_UNIT(*)
SI_UNIT($,.STERADIAN.)
SOLID_ANGLE_UNIT()
);
#50095=SHAPE_DEFINITION_REPRESENTATION(#50116,#50157);
#50116=PRODUCT_DEFINITION_SHAPE('',$,#50179);
#50157=SHAPE_REPRESENTATION('',(#10466),#50070);
#50168=PRODUCT_DEFINITION_CONTEXT('part definition',#50233,'design');
#50179=PRODUCT_DEFINITION('Aluminum Thermal Heater Block',
'Aluminum Thermal Heater Block',#50200,#50168);
#50200=PRODUCT_DEFINITION_FORMATION('',$,#50245);
#50233=APPLICATION_CONTEXT('Managed model based 3d engineering');
#50234=PRODUCT_CONTEXT('part definition',#50233,'mechanical');
#50245=PRODUCT('Aluminum Thermal Heater Block',
'Aluminum Thermal Heater Block',
'LEGAL AND USAGE DISCLAIMER: this Data/Model is provided \X2\201C\X0\A
S IS\X2\201D\X0\ for informational and representational only. It is a 
geometric approximation and is NOT engineered, certified, or guarantee
d for dimensional accuracy, exact tolerances, or production-level prec
ision. Vendor disclaims all implied warranties including fitness for a
 particular purpose. DO NOT USE FOR DIRECT PHYSICAL MANUFACTURING, AUT
OMATED PRODUCTION, OR SAFETY-CRITICAL SYSTEMS without independent engi
neering verification and resolution of any design discrepancies.',(#50234));
#50259=PRESENTATION_STYLE_ASSIGNMENT((#50266));
#50266=SURFACE_STYLE_USAGE(.BOTH.,#50273);
#50273=SURFACE_SIDE_STYLE('',(#50280));
#50280=SURFACE_STYLE_FILL_AREA(#50287);
#50287=FILL_AREA_STYLE('Opaque(246,246,243)',(#50294));
#50294=FILL_AREA_STYLE_COLOUR('Opaque(246,246,243)',#50301);
#50301=COLOUR_RGB('Opaque(246,246,243)',0.964705882352941,0.964705882352941,
0.952941176470588);
ENDSEC;
END-ISO-10303-21;
